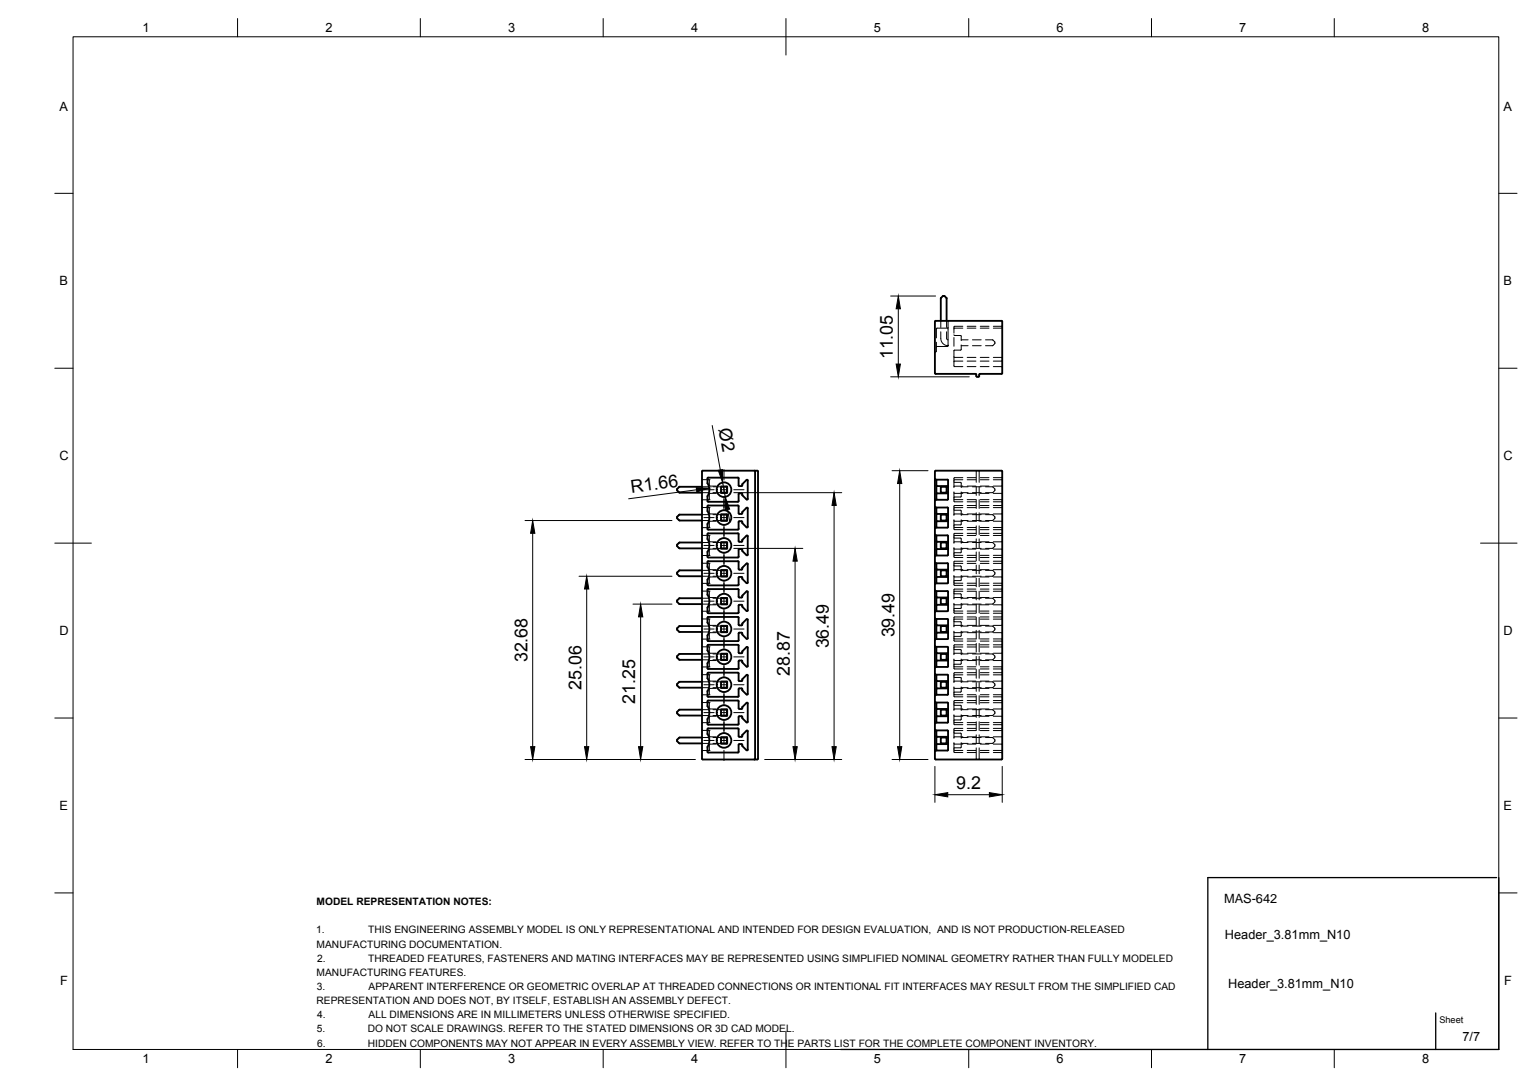
ISO-10303-21;
HEADER;
FILE_DESCRIPTION((''),'2;1');
FILE_NAME('Header_3.81mm_N10.step','2026-10-09T09:51:33-07:00',(''),(''),'','','');
FILE_SCHEMA (('AUTOMOTIVE_DESIGN { 1 0 10303 214 3 1 1 }'));
ENDSEC;
DATA;
#10=MECHANICAL_DESIGN_GEOMETRIC_PRESENTATION_REPRESENTATION('',(#1939,#1940,#1941,#1942,#1943,#1944,#1945,#1946,#1947,#1948,#1949,#1950,#1951,#1952,#1953,#1954,#1955,#1956,#1957,#1958,#1959,#1960,#1961,#1962,#1963,#1964,#1965,#1966,#1967,#1968,#1969,#1970,#1971,#1972,#1973,#1974,#1975,#1976,#1977,#1978,#1979,#1980,#1981,#1982,#1983,#1984,#1985,#1986,#1987,#1988,#1989,#1990,#1991,#1992,#1993,#1994,#1995,#1996,#1997,#1998,#1999,#2000,#2001,#2002,#2003,#2004,#2005,#2006,#2007,#2008,#2009,#2010,#2011,#2012,#2013,#2014,#2015,#2016,#2017,#2018,#2019,#2020,#2021,#2022,#2023,#2024,#2025,#2026,#2027,#2028,#2029,#2030,#2031,#2032,#2033,#2034,#2035,#2036,#2037,#2038,#2039,#2040,#2041,#2042,#2043,#2044,#2045,#2046,#2047,#2048,#2049,#2050,#2051,#2052,#2053,#2054,#2055,#2056,#2057,#2058,#2059,#2060,#2061,#2062,#2063,#2064,#2065,#2066,#2067,#2068,#2069,#2070,#2071,#2072,#2073,#2074,#2075,#2076,#2077,#2078,#2079,#2080,#2081,#2082,#2083,#2084,#2085,#2086,#2087,#2088,#2089,#2090,#2091,#2092,#2093,#2094,#2095,#2096,#2097,#2098,#2099,#2100,#2101,#2102,#2103,#2104,#2105,#2106,#2107,#2108,#2109,#2110,#2111,#2112,#2113,#2114,#2115,#2116,#2117,#2118,#2119,#2120,#2121,#2122,#2123,#2124,#2125,#2126,#2127,#2128,#2129,#2130,#2131,#2132,#2133,#2134,#2135,#2136,#2137,#2138,#2139,#2140,#2141,#2142,#2143,#2144,#2145,#2146,#2147,#2148,#2149,#2150,#2151,#2152,#2153,#2154,#2155,#2156,#2157,#2158,#2159,#2160,#2161,#2162,#2163,#2164,#2165,#2166,#2167,#2168,#2169,#2170,#2171,#2172,#2173,#2174,#2175,#2176,#2177,#2178,#2179,#2180,#2181,#2182,#2183,#2184,#2185,#2186,#2187,#2188,#2189,#2190,#2191,#2192,#2193,#2194,#2195,#2196,#2197,#2198,#2199,#2200,#2201,#2202,#2203,#2204,#2205,#2206,#2207,#2208,#2209,#2210,#2211,#2212,#2213,#2214,#2215,#2216,#2217,#2218,#2219,#2220,#2221,#2222,#2223,#2224,#2225,#2226,#2227,#2228,#2229,#2230,#2231,#2232,#2233,#2234,#2235,#2236,#2237,#2238,#2239,#2240,#2241,#2242,#2243,#2244,#2245,#2246,#2247,#2248,#2249,#2250,#2251,#2252,#2253,#2254,#2255,#2256,#2257,#2258,#2259,#2260,#2261,#2262,#2263,#2264,#2265,#2266,#2267,#2268,#2269,#2270,#2271,#2272,#2273,#2274,#2275,#2276,#2277,#2278,#2279,#2280,#2281,#2282,#2283,#2284,#2285,#2286,#2287,#2288,#2289,#2290,#2291,#2292,#2293,#2294,#2295,#2296,#2297,#2298,#2299,#2300,#2301,#2302,#2303,#2304,#2305,#2306,#2307,#2308,#2309,#2310,#2311,#2312,#2313,#2314,#2315,#2316,#2317,#2318,#2319,#2320,#2321,#2322,#2323,#2324,#2325,#2326,#2327,#2328,#2329,#2330,#2331,#2332,#2333,#2334,#2335,#2336,#2337,#2338,#2339,#2340,#2341,#2342,#2343,#2344,#2345,#2346,#2347,#2348,#2349,#2350,#2351,#2352,#2353,#2354,#2355,#2356,#2357,#2358,#2359,#2360,#2361,#2362,#2363,#2364,#2365,#2366,#2367,#2368,#2369,#2370,#2371,#2372,#2373,#2374,#2375,#2376,#2377,#2378,#2379,#2380,#2381,#2382,#2383,#2384,#2385,#2386,#2387,#2388,#2389,#2390,#2391,#2392,#2393,#2394,#2395,#2396,#2397,#2398,#2399,#2400,#2401,#2402,#2403,#2404,#2405,#2406,#2407,#2408,#2409,#2410,#2411,#2412,#2413,#2414,#2415,#2416,#2417,#2418,#2419,#2420,#2421,#2422,#2423,#2424,#2425,#2426,#2427,#2428,#2429,#2430,#2431,#2432,#2433,#2434,#2435,#2436,#2437,#2438,#2439,#2440,#2441,#2442,#2443,#2444,#2445,#2446,#2447,#2448,#2449,#2450,#2451,#2452,#2453,#2454,#2455,#2456,#2457,#2458,#2459,#2460,#2461,#2462,#2463,#2464,#2465,#2466,#2467,#2468,#2469,#2470,#2471,#2472,#2473,#2474,#2475,#2476,#2477,#2478,#2479,#2480,#2481,#2482,#2483,#2484,#2485,#2486,#2487,#2488,#2489,#2490,#2491,#2492,#2493,#2494,#2495,#2496,#2497,#2498,#2499,#2500,#2501,#2502,#2503,#2504,#2505,#2506,#2507,#2508,#2509,#2510,#2511,#2512,#2513,#2514,#2515,#2516,#2517,#2518,#2519,#2520,#2521,#2522,#2523,#2524,#2525,#2526,#2527,#2528,#2529,#2530,#2531,#2532,#2533,#2534,#2535,#2536,#2537,#2538,#2539,#2540,#2541,#2542,#2543,#2544,#2545,#2546,#2547,#2548,#2549,#2550,#2551,#2552,#2553,#2554,#2555,#2556,#2557,#2558,#2559,#2560,#2561,#2562,#2563,#2564,#2565,#2566,#2567,#2568,#2569,#2570,#2571,#2572,#2573,#2574,#2575,#2576,#2577,#2578,#2579,#2580,#2581,#2582,#2583,#2584,#2585,#2586,#2587,#2588,#2589,#2590,#2591,#2592,#2593,#2594,#2595,#2596,#2597,#2598,#2599,#2600,#2601,#2602,#2603,#2604,#2605,#2606,#2607,#2608,#2609,#2610,#2611,#2612,#2613,#2614,#2615,#2616,#2617,#2618,#2619,#2620,#2621,#2622,#2623,#2624,#2625,#2626,#2627,#2628,#2629,#2630,#2631,#2632,#2633,#2634,#2635,#2636,#2637,#2638,#2639,#2640,#2641,#2642,#2643,#2644,#2645,#2646,#2647,#2648,#2649,#2650,#2651,#2652,#2653,#2654,#2655,#2656,#2657,#2658,#2659,#2660,#2661,#2662,#2663,#2664,#2665,#2666,#2667,#2668,#2669,#2670,#2671,#2672,#2673,#2674,#2675,#2676,#2677,#2678,#2679,#2680,#2681,#2682,#2683,#2684,#2685,#2686,#2687,#2688,#2689,#2690,#2691,#2692,#2693,#2694,#2695,#2696,#2697,#2698,#2699,#2700,#2701,#2702,#2703,#2704,#2705,#2706,#2707,#2708,#2709,#2710,#2711,#2712,#2713,#2714,#2715,#2716,#2717,#2718,#2719,#2720,#2721,#2722,#2723,#2724,#2725,#2726,#2727,#2728,#2729,#2730,#2731,#2732,#2733,#2734,#2735,#2736,#2737,#2738,#2739,#2740,#2741,#2742,#2743,#2744,#2745,#2746,#2747,#2748,#2749,#2750,#2751,#2752,#2753,#2754,#2755,#2756,#2757,#2758,#2759,#2760,#2761,#2762,#2763,#2764,#2765,#2766,#2767,#2768,#2769,#2770,#2771,#2772,#2773,#2774,#2775,#2776,#2777,#2778,#2779,#2780,#2781,#2782,#2783,#2784,#2785,#2786,#2787,#2788,#2789,#2790,#2791,#2792,#2793,#2794,#2795,#2796,#2797,#2798,#2799,#2800,#2801,#2802,#2803,#2804,#2805,#2806,#2807,#2808,#2809,#2810,#2811,#2812,#2813,#2814,#2815,#2816,#2817,#2818,#2819,#2820,#2821,#2822,#2823,#2824,#2825,#2826,#2827,#2828,#2829,#2830,#2831,#2832,#2833,#2834,#2835,#2836,#2837,#2838,#2839,#2840,#2841,#2842,#2843,#2844,#2845,#2846,#2847,#2848,#2849,#2850,#2851,#2852,#2853,#2854,#2855,#2856,#2857,#2858,#2859,#2860,#2861,#2862,#2863,#2864,#2865,#2866,#2867,#2868,#2869,#2870,#2871,#2872,#2873,#2874,#2875,#2876,#2877,#2878,#2879,#2880,#2881,#2882,#2883,#2884,#2885,#2886,#2887,#2888,#2889,#2890,#2891,#2892,#2893,#2894,#2895,#2896,#2897,#2898,#2899,#2900,#2901,#2902,#2903,#2904,#2905,#2906,#2907,#2908,#2909,#2910,#2911,#2912,#2913,#2914,#2915,#2916,#2917,#2918,#2919,#2920,#2921,#2922,#2923,#2924,#2925,#2926,#2927,#2928,#2929,#2930,#2931,#2932,#2933,#2934,#2935,#2936,#2937,#2938,#2939,#2940,#2941,#2942,#2943,#2944,#2945,#2946,#2947,#2948,#2949,#2950,#2951,#2952,#2953,#2954,#2955,#2956,#2957,#2958,#2959,#2960,#2961,#2962,#2963,#2964,#2965,#2966,#2967,#2968,#2969,#2970,#2971,#2972,#2973,#2974,#2975,#2976,#2977,#2978,#2979,#2980,#2981,#2982,#2983,#2984,#2985,#2986,#2987,#2988,#2989,#2990,#2991,#2992,#2993,#2994,#2995,#2996,#2997,#2998,#2999,#3000,#3001,#3002,#3003,#3004,#3005,#3006,#3007,#3008,#3009,#3010,#3011,#3012,#3013,#3014,#3015,#3016,#3017,#3018,#3019,#3020,#3021,#3022,#3023,#3024,#3025,#3026,#3027,#3028,#3029,#3030,#3031,#3032,#3033,#3034,#3035,#3036,#3037,#3038,#3039,#3040,#3041,#3042,#3043,#3044,#3045,#3046,#3047,#3048,#3049,#3050,#3051,#3052,#3053,#3054,#3055,#3056,#3057,#3058,#3059,#3060,#3061,#3062,#3063,#3064,#3065,#3066,#3067,#3068,#3069,#3070,#3071,#3072,#3073,#3074,#3075,#3076,#3077,#3078,#3079,#3080,#3081,#3082,#3083,#3084,#3085,#3086,#3087,#3088,#3089,#3090,#3091,#3092,#3093,#3094,#3095,#3096,#3097,#3098,#3099,#3100,#3101,#3102,#3103,#3104,#3105,#3106,#3107,#3108,#3109,#3110,#3111,#3112,#3113,#3114,#3115,#3116,#3117,#3118,#3119,#3120,#3121,#3122,#3123,#3124,#3125,#3126,#3127,#3128,#3129,#3130,#3131,#3132,#3133,#3134,#3135,#3136,#3137,#3138,#3139,#3140,#3141,#3142,#3143,#3144,#3145,#3146,#3147,#3148,#3149,#3150,#3151,#3152,#3153,#3154,#3155,#3156,#3157,#3158,#3159,#3160,#3161,#3162,#3163,#3164,#3165,#3166,#3167,#3168,#3169,#3170,#3171,#3172,#3173,#3174,#3175,#3176,#3177,#3178,#3179,#3180,#3181,#3182,#3183,#3184,#3185,#3186,#3187,#3188,#3189,#3190,#3191,#3192,#3193,#3194,#3195,#3196,#3197,#3198,#3199,#3200,#3201,#3202,#3203,#3204,#3205,#3206,#3207,#3208,#3209,#3210,#3211,#3212,#3213,#3214,#3215,#3216,#3217,#3218,#3219,#3220,#3221,#3222,#3223,#3224,#3225,#3226,#3227,#3228,#3229,#3230,#3231,#3232,#3233,#3234,#3235,#3236,#3237,#3238,#3239,#3240,#3241,#3242,#3243,#3244,#3245,#3246,#3247,#3248,#3249,#3250,#3251,#3252,#3253,#3254,#3255,#3256,#3257,#3258,#3259,#3260,#3261,#3262,#3263,#3264,#3265,#3266,#3267,#3268,#3269,#3270,#3271,#3272,#3273,#3274,#3275,#3276,#3277,#3278,#3279,#3280,#3281,#3282,#3283,#3284,#3285,#3286,#3287,#3288,#3289,#3290,#3291,#3292,#3293,#3294,#3295,#3296,#3297,#3298,#3299,#3300,#3301,#3302,#3303,#3304,#3305,#3306,#3307,#3308,#3309,#3310,#3311,#3312,#3313,#3314,#3315,#3316,#3317,#3318,#3319,#3320,#3321,#3322,#3323,#3324,#3325,#3326,#3327,#3328,#3329,#3330,#3331,#3332,#3333,#3334,#3335,#3336,#3337,#3338,#3339,#3340,#3341,#3342,#3343,#3344,#3345,#3346,#3347,#3348,#3349,#3350,#3351,#3352,#3353,#3354,#3355,#3356,#3357,#3358,#3359,#3360,#3361,#3362,#3363,#3364,#3365,#3366,#3367,#3368,#3369,#3370,#3371,#3372,#3373,#3374,#3375,#3376,#3377,#3378,#3379,#3380,#3381,#3382,#3383,#3384,#3385,#3386,#3387,#3388,#3389,#3390,#3391,#3392,#3393,#3394,#3395,#3396,#3397,#3398,#3399,#3400,#3401,#3402,#3403,#3404,#3405,#3406,#3407,#3408,#3409,#3410,#3411,#3412,#3413,#3414,#3415,#3416,#3417,#3418,#3419,#3420,#3421,#3422,#3423,#3424,#3425,#3426,#3427,#3428,#3429,#3430,#3431,#3432,#3433,#3434,#3435,#3436,#3437,#3438,#3439,#3440,#3441,#3442,#3443,#3444,#3445,#3446,#3447,#3448,#3449,#3450,#3451,#3452,#3453,#3454,#3455,#3456,#3457,#3458,#3459,#3460,#3461,#3462,#3463,#3464,#3465,#3466,#3467,#3468,#3469,#3470,#3471,#3472,#3473,#3474,#3475,#3476,#3477,#3478,#3479,#3480,#3481,#3482,#3483,#3484,#3485,#3486,#3487,#3488,#3489,#3490,#3491,#3492,#3493,#3494,#3495,#3496,#3497,#3498,#3499,#3500,#3501,#3502,#3503,#3504,#3505,#3506,#3507,#3508,#3509,#3510,#3511,#3512,#3513,#3514,#3515,#3516,#3517,#3518,#3519,#3520,#3521,#3522,#3523,#3524,#3525,#3526,#3527,#3528,#3529,#3530,#3531,#3532,#3533,#3534,#3535,#3536,#3537,#3538,#3539,#3540,#3541,#3542,#3543,#3544,#3545,#3546,#3547,#3548,#3549,#3550,#3551,#3552,#3553,#3554,#3555,#3556,#3557,#3558,#3559,#3560,#3561,#3562,#3563,#3564,#3565,#3566,#3567,#3568,#3569,#3570,#3571,#3572,#3573,#3574,#3575,#3576,#3577,#3578,#3579,#3580,#3581,#3582,#3583,#3584,#3585,#3586,#3587,#3588,#3589,#3590,#3591,#3592,#3593,#3594,#3595,#3596,#3597,#3598,#3599,#3600,#3601,#3602,#3603,#3604,#3605,#3606,#3607,#3608,#3609,#3610,#3611,#3612,#3613,#3614,#3615,#3616,#3617,#3618,#3619,#3620,#3621,#3622,#3623,#3624,#3625,#3626,#3627,#3628,#3629,#3630,#3631,#3632,#3633,#3634,#3635,#3636,#3637,#3638,#3639,#3640,#3641,#3642,#3643,#3644,#3645,#3646,#3647,#3648,#3649,#3650,#3651,#3652,#3653,#3654,#3655,#3656,#3657,#3658,#3659,#3660,#3661,#3662,#3663,#3664,#3665,#3666,#3667,#3668,#3669,#3670,#3671,#3672,#3673,#3674,#3675,#3676,#3677,#3678,#3679,#3680,#3681,#3682,#3683,#3684,#3685,#3686,#3687,#3688,#3689,#3690,#3691,#3692,#3693,#3694,#3695,#3696,#3697,#3698,#3699,#3700,#3701,#3702,#3703,#3704,#3705,#3706,#3707,#3708,#3709,#3710,#3711,#3712,#3713,#3714,#3715,#3716,#3717,#3718,#3719,#3720,#3721,#3722,#3723,#3724,#3725,#3726,#3727,#3728,#3729,#3730,#3731,#3732,#3733,#3734,#3735,#3736,#3737,#3738,#3739,#3740,#3741,#3742,#3743,#3744,#3745,#3746,#3747,#3748,#3749,#3750,#3751,#3752,#3753,#3754,#3755,#3756,#3757,#3758,#3759,#3760,#3761,#3762,#3763,#3764,#3765,#3766,#3767,#3768,#3769,#3770,#3771,#3772,#3773,#3774,#3775,#3776,#3777,#3778,#3779,#3780,#3781,#3782,#3783,#3784,#3785,#3786,#3787,#3788,#3789,#3790,#3791,#3792,#3793,#3794,#3795,#3796,#3797,#3798,#3799,#3800,#3801,#3802,#3803,#3804,#3805,#3806,#3807,#3808,#3809,#3810,#3811,#3812,#3813,#3814,#3815,#3816,#3817,#3818,#3819,#3820,#3821,#3822,#3823,#3824,#3825,#3826,#3827,#3828,#3829,#3830,#3831,#3832,#3833,#3834,#3835,#3836,#3837,#3838,#3839,#3840,#3841,#3842,#3843,#3844,#3845,#3846,#3847,#3848,#3849,#3850,#3851,#3852,#3853,#3854,#3855,#3856,#3857,#3858,#3859,#3860,#3861,#3862,#3863,#3864,#3865,#3866,#3867,#3868,#3869,#3870,#3871,#3872,#3873,#3874,#3875,#3876,#3877,#3878,#3879,#3880,#3881,#3882,#3883,#3884,#3885,#3886,#3887,#3888,#3889,#3890,#3891,#3892,#3893,#3894,#3895,#3896,#3897,#3898,#3899,#3900,#3901,#3902,#3903,#3904,#3905,#3906,#3907,#3908,#3909,#3910,#3911,#3912,#3913,#3914,#3915,#3916,#3917,#3918,#3919,#3920,#3921,#3922,#3923,#3924,#3925,#3926,#3927,#3928,#3929,#3930,#3931,#3932,#3933,#3934,#3935,#3936,#3937,#3938,#3939,#3940,#3941,#3942,#3943,#3944,#3945,#3946,#3947,#3948,#3949,#3950,#3951,#3952,#3953,#3954,#3955,#3956,#3957,#3958,#3959,#3960,#3961,#3962,#3963,#3964,#3965,#3966,#3967,#3968,#3969,#3970,#3971,#3972,#3973,#3974,#3975,#3976,#3977,#3978,#3979,#3980,#3981,#3982,#3983,#3984,#3985,#3986,#3987,#3988,#3989,#3990,#3991,#3992,#3993,#3994,#3995,#3996,#3997,#3998,#3999,#4000,#4001,#4002,#4003,#4004,#4005,#4006,#4007,#4008,#4009,#4010,#4011,#4012,#4013,#4014,#4015,#4016,#4017,#4018,#4019,#4020,#4021,#4022,#4023,#4024,#4025,#4026,#4027,#4028,#4029,#4030,#4031,#4032,#4033,#4034,#4035,#4036,#4037,#4038,#4039,#4040,#4041,#4042,#4043,#4044,#4045,#4046,#4047,#4048,#4049,#4050,#4051,#4052,#4053,#4054,#4055,#4056,#4057,#4058,#4059,#4060,#4061,#4062,#4063,#4064,#4065,#4066,#4067,#4068,#4069,#4070,#4071,#4072,#4073,#4074,#4075,#4076,#4077,#4078,#4079,#4080,#4081,#4082,#4083,#4084,#4085,#4086,#4087,#4088,#4089,#4090,#4091,#4092,#4093,#4094,#4095,#4096,#4097,#4098,#4099,#4100,#4101,#4102,#4103,#4104,#4105,#4106,#4107,#4108,#4109,#4110,#4111,#4112,#4113,#4114,#4115,#4116,#4117,#4118,#4119,#4120,#4121,#4122,#4123,#4124,#4125,#4126,#4127,#4128,#4129,#4130,#4131,#4132,#4133,#4134,#4135,#4136,#4137,#4138,#4139,#4140,#4141,#4142,#4143,#4144,#4145,#4146,#4147,#4148,#4149,#4150,#4151,#4152,#4153,#4154,#4155,#4156,#4157,#4158,#4159,#4160,#4161,#4162,#4163,#4164,#4165,#4166,#4167,#4168,#4169),#126571);
#290=B_SPLINE_CURVE_WITH_KNOTS('',3,(#113894,#113895,#113896,#113897,#113898,
#113899,#113900,#113901),.UNSPECIFIED.,.F.,.F.,(4,2,2,4),(-0.0212593174733862,
-0.0176486602253693,-0.0143243289552082,-0.0134403252720105),
 .UNSPECIFIED.) ;
#291=B_SPLINE_CURVE_WITH_KNOTS('',3,(#113937,#113938,#113939,#113940,#113941,
#113942,#113943,#113944),.UNSPECIFIED.,.F.,.F.,(4,2,2,4),(-0.021259317482921,
-0.0176486602328459,-0.0143243289609224,-0.0134403252772803),
 .UNSPECIFIED.) ;
#292=B_SPLINE_CURVE_WITH_KNOTS('',3,(#113980,#113981,#113982,#113983,#113984,
#113985,#113986,#113987),.UNSPECIFIED.,.F.,.F.,(4,2,2,4),(-0.0212593174877944,
-0.0176486602368674,-0.0143243289641644,-0.0134403252803157),
 .UNSPECIFIED.) ;
#293=B_SPLINE_CURVE_WITH_KNOTS('',3,(#114023,#114024,#114025,#114026,#114027,
#114028,#114029,#114030),.UNSPECIFIED.,.F.,.F.,(4,2,2,4),(-0.0212593174829433,
-0.0176486602328601,-0.014324328960934,-0.0134403252772914),
 .UNSPECIFIED.) ;
#294=B_SPLINE_CURVE_WITH_KNOTS('',3,(#114066,#114067,#114068,#114069,#114070,
#114071,#114072,#114073),.UNSPECIFIED.,.F.,.F.,(4,2,2,4),(-0.0212593174732112,
-0.0176486602254681,-0.0143243289554829,-0.0134403252723181),
 .UNSPECIFIED.) ;
#295=B_SPLINE_CURVE_WITH_KNOTS('',3,(#114109,#114110,#114111,#114112,#114113,
#114114,#114115,#114116),.UNSPECIFIED.,.F.,.F.,(4,2,2,4),(-0.0212593174781932,
-0.0176486602293651,-0.0143243289584549,-0.0134403252750573),
 .UNSPECIFIED.) ;
#296=B_SPLINE_CURVE_WITH_KNOTS('',3,(#114152,#114153,#114154,#114155,#114156,
#114157,#114158,#114159),.UNSPECIFIED.,.F.,.F.,(4,2,2,4),(-0.0212593174830444,
-0.0176486602331658,-0.0143243289613579,-0.0134403252777338),
 .UNSPECIFIED.) ;
#297=B_SPLINE_CURVE_WITH_KNOTS('',3,(#114195,#114196,#114197,#114198,#114199,
#114200,#114201,#114202),.UNSPECIFIED.,.F.,.F.,(4,2,2,4),(-0.021259317485983,
-0.017648660235379,-0.0143243289629727,-0.0134403252792024),
 .UNSPECIFIED.) ;
#298=B_SPLINE_CURVE_WITH_KNOTS('',3,(#114319,#114320,#114321,#114322,#114323,
#114324,#114325,#114326),.UNSPECIFIED.,.F.,.F.,(4,2,2,4),(-0.0212593174838741,
-0.0176486602337396,-0.0143243289617316,-0.0134403252780616),
 .UNSPECIFIED.) ;
#299=B_SPLINE_CURVE_WITH_KNOTS('',3,(#114443,#114444,#114445,#114446,#114447,
#114448,#114449,#114450),.UNSPECIFIED.,.F.,.F.,(4,2,2,4),(-0.021259317485706,
-0.0176486602351398,-0.0143243289627718,-0.013440325279013),
 .UNSPECIFIED.) ;
#300=B_SPLINE_CURVE_WITH_KNOTS('',3,(#116047,#116048,#116049,#116050,#116051,
#116052,#116053,#116054),.UNSPECIFIED.,.F.,.F.,(4,2,2,4),(-0.052701717162025,
-0.0518504523811948,-0.0480303917439054,-0.04467544736819),
 .UNSPECIFIED.) ;
#301=B_SPLINE_CURVE_WITH_KNOTS('',3,(#116058,#116059,#116060,#116061,#116062,
#116063,#116064,#116065,#116066,#116067,#116068,#116069,#116070,#116071,
#116072,#116073,#116074,#116075,#116076,#116077,#116078,#116079,#116080,
#116081,#116082,#116083,#116084,#116085,#116086,#116087,#116088),
 .UNSPECIFIED.,.F.,.F.,(4,3,3,3,3,3,3,3,3,3,4),(0.,1.7911486298437E-5,3.35636550441565E-5,
5.14128838689559E-5,6.71346369544057E-5,8.50076921954425E-5,0.000100614915215922,
0.000118595988596762,0.000134133865285036,0.000151845157316713,0.0001565184788544),
 .UNSPECIFIED.) ;
#302=B_SPLINE_CURVE_WITH_KNOTS('',3,(#116090,#116091,#116092,#116093,#116094,
#116095,#116096,#116097,#116098,#116099,#116100,#116101,#116102,#116103,
#116104,#116105,#116106,#116107,#116108,#116109,#116110,#116111),
 .UNSPECIFIED.,.F.,.F.,(4,2,2,2,2,2,2,2,2,2,4),(-0.0842935807175857,-0.0841564124762399,
-0.0836958438579189,-0.0829341784875174,-0.0805923611130053,-0.0773601159115686,
-0.0742136752654363,-0.071123820447877,-0.0675672289498007,-0.0637829215046486,
-0.0629274139192696),.UNSPECIFIED.) ;
#303=B_SPLINE_CURVE_WITH_KNOTS('',3,(#119109,#119110,#119111,#119112,#119113,
#119114,#119115,#119116),.UNSPECIFIED.,.F.,.F.,(4,2,2,4),(-0.0527017171620382,
-0.0518504523812081,-0.0480303917439178,-0.0446754473682008),
 .UNSPECIFIED.) ;
#304=B_SPLINE_CURVE_WITH_KNOTS('',3,(#119120,#119121,#119122,#119123,#119124,
#119125,#119126,#119127,#119128,#119129,#119130,#119131,#119132,#119133,
#119134,#119135,#119136,#119137,#119138,#119139,#119140,#119141,#119142,
#119143,#119144,#119145,#119146,#119147,#119148,#119149,#119150),
 .UNSPECIFIED.,.F.,.F.,(4,3,3,3,3,3,3,3,3,3,4),(0.,1.79114862984415E-5,
3.35636550441565E-5,5.14128838689557E-5,6.7134636954406E-5,8.50076921954395E-5,
0.000100614915215921,0.000118595988596772,0.000134133865285036,0.000151845157316653,
0.0001565184788544),.UNSPECIFIED.) ;
#305=B_SPLINE_CURVE_WITH_KNOTS('',3,(#119152,#119153,#119154,#119155,#119156,
#119157,#119158,#119159,#119160,#119161,#119162,#119163,#119164,#119165,
#119166,#119167,#119168,#119169,#119170,#119171,#119172,#119173),
 .UNSPECIFIED.,.F.,.F.,(4,2,2,2,2,2,2,2,2,2,4),(-0.0842935807153196,-0.0841564124739783,
-0.0836958438556783,-0.0829341784853091,-0.0805923611108952,-0.0773601159095917,
-0.0742136752635866,-0.0711238204461505,-0.0675672289482145,-0.0637829215032092,
-0.062927413917864),.UNSPECIFIED.) ;
#306=B_SPLINE_CURVE_WITH_KNOTS('',3,(#119813,#119814,#119815,#119816,#119817,
#119818,#119819,#119820),.UNSPECIFIED.,.F.,.F.,(4,2,2,4),(-0.0527017171621304,
-0.0518504523813015,-0.0480303917440028,-0.0446754473682719),
 .UNSPECIFIED.) ;
#307=B_SPLINE_CURVE_WITH_KNOTS('',3,(#119824,#119825,#119826,#119827,#119828,
#119829,#119830,#119831,#119832,#119833,#119834,#119835,#119836,#119837,
#119838,#119839,#119840,#119841,#119842,#119843,#119844,#119845,#119846,
#119847,#119848,#119849,#119850,#119851,#119852,#119853,#119854),
 .UNSPECIFIED.,.F.,.F.,(4,3,3,3,3,3,3,3,3,3,4),(0.,1.79114862984384E-5,
3.35636550441566E-5,5.14128838689606E-5,6.7134636954406E-5,8.50076921954722E-5,
0.000100614915215922,0.000118595988596755,0.000134133865285036,0.00015184515731678,
0.0001565184788544),.UNSPECIFIED.) ;
#308=B_SPLINE_CURVE_WITH_KNOTS('',3,(#119856,#119857,#119858,#119859,#119860,
#119861,#119862,#119863,#119864,#119865,#119866,#119867,#119868,#119869,
#119870,#119871,#119872,#119873,#119874,#119875,#119876,#119877),
 .UNSPECIFIED.,.F.,.F.,(4,2,2,2,2,2,2,2,2,2,4),(-0.0842935807419127,-0.0841564125005222,
-0.0836958438819682,-0.082934178511186,-0.0805923611355419,-0.0773601159325885,
-0.0742136752850249,-0.0711238204661043,-0.0675672289665108,-0.0637829215197928,
-0.0629274139340661),.UNSPECIFIED.) ;
#309=B_SPLINE_CURVE_WITH_KNOTS('',3,(#120040,#120041,#120042,#120043,#120044,
#120045,#120046,#120047),.UNSPECIFIED.,.F.,.F.,(4,2,2,4),(-0.0527017171621393,
-0.0518504523813096,-0.0480303917440155,-0.0446754473682944),
 .UNSPECIFIED.) ;
#310=B_SPLINE_CURVE_WITH_KNOTS('',3,(#120051,#120052,#120053,#120054,#120055,
#120056,#120057,#120058,#120059,#120060,#120061,#120062,#120063,#120064,
#120065,#120066,#120067,#120068,#120069,#120070,#120071,#120072,#120073,
#120074,#120075,#120076,#120077,#120078,#120079,#120080,#120081),
 .UNSPECIFIED.,.F.,.F.,(4,3,3,3,3,3,3,3,3,3,4),(0.,1.7911486298444E-5,3.35636550441567E-5,
5.14128838689174E-5,6.71346369544062E-5,8.50076921954515E-5,0.000100614915215921,
0.000118595988596814,0.000134133865285036,0.000151845157316771,0.0001565184788544),
 .UNSPECIFIED.) ;
#311=B_SPLINE_CURVE_WITH_KNOTS('',3,(#120083,#120084,#120085,#120086,#120087,
#120088,#120089,#120090,#120091,#120092,#120093,#120094,#120095,#120096,
#120097,#120098,#120099,#120100,#120101,#120102,#120103,#120104),
 .UNSPECIFIED.,.F.,.F.,(4,2,2,2,2,2,2,2,2,2,4),(-0.0842935808351552,-0.0841564125935704,
-0.0836958439740798,-0.0829341786018125,-0.0805923612217205,-0.077360116012801,
-0.0742136753596006,-0.0711238205353107,-0.0675672290297288,-0.0637829215768355,
-0.0629274139897445),.UNSPECIFIED.) ;
#312=B_SPLINE_CURVE_WITH_KNOTS('',3,(#120267,#120268,#120269,#120270,#120271,
#120272,#120273,#120274),.UNSPECIFIED.,.F.,.F.,(4,2,2,4),(-0.0527017171620452,
-0.0518504523812172,-0.0480303917439374,-0.04467544736823),
 .UNSPECIFIED.) ;
#313=B_SPLINE_CURVE_WITH_KNOTS('',3,(#120278,#120279,#120280,#120281,#120282,
#120283,#120284,#120285,#120286,#120287,#120288,#120289,#120290,#120291,
#120292,#120293,#120294,#120295,#120296,#120297,#120298,#120299,#120300,
#120301,#120302,#120303,#120304,#120305,#120306,#120307,#120308),
 .UNSPECIFIED.,.F.,.F.,(4,3,3,3,3,3,3,3,3,3,4),(0.,1.79114862984569E-5,
3.35636550441567E-5,5.14128838689565E-5,6.71346369544062E-5,8.50076921954284E-5,
0.000100614915215921,0.000118595988596684,0.000134133865285036,0.000151845157316633,
0.0001565184788544),.UNSPECIFIED.) ;
#314=B_SPLINE_CURVE_WITH_KNOTS('',3,(#120310,#120311,#120312,#120313,#120314,
#120315,#120316,#120317,#120318,#120319,#120320,#120321,#120322,#120323,
#120324,#120325,#120326,#120327,#120328,#120329,#120330,#120331),
 .UNSPECIFIED.,.F.,.F.,(4,2,2,2,2,2,2,2,2,2,4),(-0.0842935807861705,-0.0841564125446822,
-0.08369584392567,-0.0829341785541707,-0.0805923611763772,-0.0773601159705437,
-0.0742136753202586,-0.0711238204987475,-0.0675672289962676,-0.0637829215465878,
-0.0629274139602073),.UNSPECIFIED.) ;
#315=B_SPLINE_CURVE_WITH_KNOTS('',3,(#120494,#120495,#120496,#120497,#120498,
#120499,#120500,#120501),.UNSPECIFIED.,.F.,.F.,(4,2,2,4),(-0.0527017171621833,
-0.0518504523813524,-0.0480303917440445,-0.044675447368305),
 .UNSPECIFIED.) ;
#316=B_SPLINE_CURVE_WITH_KNOTS('',3,(#120505,#120506,#120507,#120508,#120509,
#120510,#120511,#120512,#120513,#120514,#120515,#120516,#120517,#120518,
#120519,#120520,#120521,#120522,#120523,#120524,#120525,#120526,#120527,
#120528,#120529,#120530,#120531,#120532,#120533,#120534,#120535),
 .UNSPECIFIED.,.F.,.F.,(4,3,3,3,3,3,3,3,3,3,4),(0.,1.791148629847E-5,3.35636550441561E-5,
5.14128838689644E-5,6.71346369544058E-5,8.50076921954764E-5,0.000100614915215921,
0.000118595988596817,0.000134133865285032,0.000151845157316703,0.000156518478854398),
 .UNSPECIFIED.) ;
#317=B_SPLINE_CURVE_WITH_KNOTS('',3,(#120537,#120538,#120539,#120540,#120541,
#120542,#120543,#120544,#120545,#120546,#120547,#120548,#120549,#120550,
#120551,#120552,#120553,#120554,#120555,#120556,#120557,#120558),
 .UNSPECIFIED.,.F.,.F.,(4,2,2,2,2,2,2,2,2,2,4),(-0.0842935807861705,-0.0841564125446822,
-0.08369584392567,-0.0829341785541707,-0.0805923611763772,-0.0773601159705437,
-0.0742136753202586,-0.0711238204987475,-0.0675672289962676,-0.0637829215465878,
-0.0629274139602073),.UNSPECIFIED.) ;
#318=B_SPLINE_CURVE_WITH_KNOTS('',3,(#120721,#120722,#120723,#120724,#120725,
#120726,#120727,#120728),.UNSPECIFIED.,.F.,.F.,(4,2,2,4),(-0.0527017171619057,
-0.0518504523810739,-0.0480303917437878,-0.0446754473680843),
 .UNSPECIFIED.) ;
#319=B_SPLINE_CURVE_WITH_KNOTS('',3,(#120732,#120733,#120734,#120735,#120736,
#120737,#120738,#120739,#120740,#120741,#120742,#120743,#120744,#120745,
#120746,#120747,#120748,#120749,#120750,#120751,#120752,#120753,#120754,
#120755,#120756,#120757,#120758,#120759,#120760,#120761,#120762),
 .UNSPECIFIED.,.F.,.F.,(4,3,3,3,3,3,3,3,3,3,4),(0.,1.79114862984022E-5,
3.35636550441561E-5,5.14128838690747E-5,6.71346369544058E-5,8.50076921955029E-5,
0.000100614915215921,0.000118595988596949,0.000134133865285032,0.000151845157316721,
0.000156518478854398),.UNSPECIFIED.) ;
#320=B_SPLINE_CURVE_WITH_KNOTS('',3,(#120764,#120765,#120766,#120767,#120768,
#120769,#120770,#120771,#120772,#120773,#120774,#120775,#120776,#120777,
#120778,#120779,#120780,#120781,#120782,#120783,#120784,#120785),
 .UNSPECIFIED.,.F.,.F.,(4,2,2,2,2,2,2,2,2,2,4),(-0.0842935806846017,-0.0841564124433096,
-0.0836958438252493,-0.0829341784552694,-0.0805923610820353,-0.0773601158823278,
-0.0742136752378489,-0.07112382042188,-0.0675672289255957,-0.0637829214823062,
-0.0629274138973503),.UNSPECIFIED.) ;
#321=B_SPLINE_CURVE_WITH_KNOTS('',3,(#120948,#120949,#120950,#120951,#120952,
#120953,#120954,#120955),.UNSPECIFIED.,.F.,.F.,(4,2,2,4),(-0.0527017171620534,
-0.0518504523812236,-0.0480303917439217,-0.0446754473681886),
 .UNSPECIFIED.) ;
#322=B_SPLINE_CURVE_WITH_KNOTS('',3,(#120959,#120960,#120961,#120962,#120963,
#120964,#120965,#120966,#120967,#120968,#120969,#120970,#120971,#120972,
#120973,#120974,#120975,#120976,#120977,#120978,#120979,#120980,#120981,
#120982,#120983,#120984,#120985,#120986,#120987,#120988,#120989),
 .UNSPECIFIED.,.F.,.F.,(4,3,3,3,3,3,3,3,3,3,4),(0.,1.79114862984111E-5,
3.35636550441561E-5,5.1412883869035E-5,6.71346369544058E-5,8.50076921954072E-5,
0.000100614915215921,0.000118595988596959,0.000134133865285032,0.000151845157317271,
0.000156518478854398),.UNSPECIFIED.) ;
#323=B_SPLINE_CURVE_WITH_KNOTS('',3,(#120991,#120992,#120993,#120994,#120995,
#120996,#120997,#120998,#120999,#121000,#121001,#121002,#121003,#121004,
#121005,#121006,#121007,#121008,#121009,#121010,#121011,#121012),
 .UNSPECIFIED.,.F.,.F.,(4,2,2,2,2,2,2,2,2,2,4),(-0.0842935807784001,-0.0841564125369118,
-0.0836958439179285,-0.0829341785465007,-0.080592361168928,-0.0773601159633862,
-0.0742136753133782,-0.071123820492143,-0.0675672289899856,-0.063782921540619,
-0.0629274139542864),.UNSPECIFIED.) ;
#324=B_SPLINE_CURVE_WITH_KNOTS('',3,(#121175,#121176,#121177,#121178,#121179,
#121180,#121181,#121182),.UNSPECIFIED.,.F.,.F.,(4,2,2,4),(-0.0527017171619366,
-0.0518504523811075,-0.0480303917438238,-0.0446754473681228),
 .UNSPECIFIED.) ;
#325=B_SPLINE_CURVE_WITH_KNOTS('',3,(#121186,#121187,#121188,#121189,#121190,
#121191,#121192,#121193,#121194,#121195,#121196,#121197,#121198,#121199,
#121200,#121201,#121202,#121203,#121204,#121205,#121206,#121207,#121208,
#121209,#121210,#121211,#121212,#121213,#121214,#121215,#121216),
 .UNSPECIFIED.,.F.,.F.,(4,3,3,3,3,3,3,3,3,3,4),(0.,1.7911486298388E-5,3.35636550441561E-5,
5.14128838690249E-5,6.71346369544058E-5,8.50076921954834E-5,0.000100614915215921,
0.000118595988596784,0.000134133865285032,0.000151845157317113,0.000156518478854398),
 .UNSPECIFIED.) ;
#326=B_SPLINE_CURVE_WITH_KNOTS('',3,(#121218,#121219,#121220,#121221,#121222,
#121223,#121224,#121225,#121226,#121227,#121228,#121229,#121230,#121231,
#121232,#121233,#121234,#121235,#121236,#121237,#121238,#121239),
 .UNSPECIFIED.,.F.,.F.,(4,2,2,2,2,2,2,2,2,2,4),(-0.0842935807784001,-0.0841564125369118,
-0.0836958439179285,-0.0829341785465007,-0.080592361168928,-0.0773601159633862,
-0.0742136753133782,-0.071123820492143,-0.0675672289899856,-0.063782921540619,
-0.0629274139542864),.UNSPECIFIED.) ;
#327=B_SPLINE_CURVE_WITH_KNOTS('',3,(#121402,#121403,#121404,#121405,#121406,
#121407,#121408,#121409),.UNSPECIFIED.,.F.,.F.,(4,2,2,4),(-0.0527017171617456,
-0.0518504523809185,-0.0480303917436524,-0.0446754473679689),
 .UNSPECIFIED.) ;
#328=B_SPLINE_CURVE_WITH_KNOTS('',3,(#121413,#121414,#121415,#121416,#121417,
#121418,#121419,#121420,#121421,#121422,#121423,#121424,#121425,#121426,
#121427,#121428,#121429,#121430,#121431,#121432,#121433,#121434,#121435,
#121436,#121437,#121438,#121439,#121440,#121441,#121442,#121443),
 .UNSPECIFIED.,.F.,.F.,(4,3,3,3,3,3,3,3,3,3,4),(0.,1.79114862983986E-5,
3.35636550441583E-5,5.14128838688763E-5,6.71346369544075E-5,8.5007692195462E-5,
0.000100614915215918,0.000118595988596873,0.000134133865285036,0.000151845157315814,
0.000156518478854401),.UNSPECIFIED.) ;
#329=B_SPLINE_CURVE_WITH_KNOTS('',3,(#121445,#121446,#121447,#121448,#121449,
#121450,#121451,#121452,#121453,#121454,#121455,#121456,#121457,#121458,
#121459,#121460,#121461,#121462,#121463,#121464,#121465,#121466),
 .UNSPECIFIED.,.F.,.F.,(4,2,2,2,2,2,2,2,2,2,4),(-0.0842935807784001,-0.0841564125369118,
-0.0836958439179285,-0.0829341785465007,-0.080592361168928,-0.0773601159633862,
-0.0742136753133782,-0.071123820492143,-0.0675672289899856,-0.063782921540619,
-0.0629274139542864),.UNSPECIFIED.) ;
#472=SHAPE_REPRESENTATION_RELATIONSHIP('SRR','None',#126602,#478) ;
#478=ADVANCED_BREP_SHAPE_REPRESENTATION('',(#4179),#126568) ;
#1939=STYLED_ITEM('',(#126640),#65362) ;
#1940=STYLED_ITEM('',(#126640),#65363) ;
#1941=STYLED_ITEM('',(#126640),#65364) ;
#1942=STYLED_ITEM('',(#126640),#65365) ;
#1943=STYLED_ITEM('',(#126640),#65366) ;
#1944=STYLED_ITEM('',(#126640),#65367) ;
#1945=STYLED_ITEM('',(#126640),#65368) ;
#1946=STYLED_ITEM('',(#126640),#65369) ;
#1947=STYLED_ITEM('',(#126640),#65370) ;
#1948=STYLED_ITEM('',(#126640),#65371) ;
#1949=STYLED_ITEM('',(#126640),#65372) ;
#1950=STYLED_ITEM('',(#126640),#65373) ;
#1951=STYLED_ITEM('',(#126640),#65374) ;
#1952=STYLED_ITEM('',(#126640),#65375) ;
#1953=STYLED_ITEM('',(#126640),#65376) ;
#1954=STYLED_ITEM('',(#126640),#65377) ;
#1955=STYLED_ITEM('',(#126640),#65378) ;
#1956=STYLED_ITEM('',(#126640),#65379) ;
#1957=STYLED_ITEM('',(#126640),#65380) ;
#1958=STYLED_ITEM('',(#126640),#65381) ;
#1959=STYLED_ITEM('',(#126640),#65382) ;
#1960=STYLED_ITEM('',(#126640),#65383) ;
#1961=STYLED_ITEM('',(#126640),#65384) ;
#1962=STYLED_ITEM('',(#126640),#65385) ;
#1963=STYLED_ITEM('',(#126640),#65386) ;
#1964=STYLED_ITEM('',(#126640),#65387) ;
#1965=STYLED_ITEM('',(#126640),#65388) ;
#1966=STYLED_ITEM('',(#126640),#65389) ;
#1967=STYLED_ITEM('',(#126640),#65390) ;
#1968=STYLED_ITEM('',(#126640),#65391) ;
#1969=STYLED_ITEM('',(#126640),#65392) ;
#1970=STYLED_ITEM('',(#126640),#65393) ;
#1971=STYLED_ITEM('',(#126640),#65394) ;
#1972=STYLED_ITEM('',(#126640),#65395) ;
#1973=STYLED_ITEM('',(#126640),#65396) ;
#1974=STYLED_ITEM('',(#126640),#65397) ;
#1975=STYLED_ITEM('',(#126640),#65398) ;
#1976=STYLED_ITEM('',(#126640),#65399) ;
#1977=STYLED_ITEM('',(#126640),#65400) ;
#1978=STYLED_ITEM('',(#126640),#65401) ;
#1979=STYLED_ITEM('',(#126640),#65402) ;
#1980=STYLED_ITEM('',(#126640),#65403) ;
#1981=STYLED_ITEM('',(#126640),#65404) ;
#1982=STYLED_ITEM('',(#126640),#65405) ;
#1983=STYLED_ITEM('',(#126640),#65406) ;
#1984=STYLED_ITEM('',(#126640),#65407) ;
#1985=STYLED_ITEM('',(#126640),#65408) ;
#1986=STYLED_ITEM('',(#126640),#65409) ;
#1987=STYLED_ITEM('',(#126640),#65410) ;
#1988=STYLED_ITEM('',(#126640),#65411) ;
#1989=STYLED_ITEM('',(#126640),#65412) ;
#1990=STYLED_ITEM('',(#126640),#65413) ;
#1991=STYLED_ITEM('',(#126640),#65414) ;
#1992=STYLED_ITEM('',(#126640),#65415) ;
#1993=STYLED_ITEM('',(#126640),#65416) ;
#1994=STYLED_ITEM('',(#126640),#65417) ;
#1995=STYLED_ITEM('',(#126640),#65418) ;
#1996=STYLED_ITEM('',(#126640),#65419) ;
#1997=STYLED_ITEM('',(#126640),#65420) ;
#1998=STYLED_ITEM('',(#126640),#65421) ;
#1999=STYLED_ITEM('',(#126640),#65422) ;
#2000=STYLED_ITEM('',(#126640),#65423) ;
#2001=STYLED_ITEM('',(#126640),#65424) ;
#2002=STYLED_ITEM('',(#126640),#65425) ;
#2003=STYLED_ITEM('',(#126640),#65426) ;
#2004=STYLED_ITEM('',(#126640),#65427) ;
#2005=STYLED_ITEM('',(#126640),#65428) ;
#2006=STYLED_ITEM('',(#126640),#65429) ;
#2007=STYLED_ITEM('',(#126640),#65430) ;
#2008=STYLED_ITEM('',(#126640),#65431) ;
#2009=STYLED_ITEM('',(#126640),#65432) ;
#2010=STYLED_ITEM('',(#126640),#65433) ;
#2011=STYLED_ITEM('',(#126640),#65434) ;
#2012=STYLED_ITEM('',(#126640),#65435) ;
#2013=STYLED_ITEM('',(#126640),#65436) ;
#2014=STYLED_ITEM('',(#126640),#65437) ;
#2015=STYLED_ITEM('',(#126640),#65438) ;
#2016=STYLED_ITEM('',(#126640),#65439) ;
#2017=STYLED_ITEM('',(#126640),#65440) ;
#2018=STYLED_ITEM('',(#126640),#65441) ;
#2019=STYLED_ITEM('',(#126640),#65442) ;
#2020=STYLED_ITEM('',(#126640),#65443) ;
#2021=STYLED_ITEM('',(#126640),#65444) ;
#2022=STYLED_ITEM('',(#126640),#65445) ;
#2023=STYLED_ITEM('',(#126640),#65446) ;
#2024=STYLED_ITEM('',(#126640),#65447) ;
#2025=STYLED_ITEM('',(#126640),#65448) ;
#2026=STYLED_ITEM('',(#126640),#65449) ;
#2027=STYLED_ITEM('',(#126640),#65450) ;
#2028=STYLED_ITEM('',(#126640),#65451) ;
#2029=STYLED_ITEM('',(#126640),#65452) ;
#2030=STYLED_ITEM('',(#126640),#65453) ;
#2031=STYLED_ITEM('',(#126640),#65454) ;
#2032=STYLED_ITEM('',(#126640),#65455) ;
#2033=STYLED_ITEM('',(#126640),#65456) ;
#2034=STYLED_ITEM('',(#126640),#65457) ;
#2035=STYLED_ITEM('',(#126640),#65458) ;
#2036=STYLED_ITEM('',(#126640),#65459) ;
#2037=STYLED_ITEM('',(#126640),#65460) ;
#2038=STYLED_ITEM('',(#126640),#65461) ;
#2039=STYLED_ITEM('',(#126640),#65462) ;
#2040=STYLED_ITEM('',(#126640),#65463) ;
#2041=STYLED_ITEM('',(#126640),#65464) ;
#2042=STYLED_ITEM('',(#126640),#65465) ;
#2043=STYLED_ITEM('',(#126640),#65466) ;
#2044=STYLED_ITEM('',(#126640),#65467) ;
#2045=STYLED_ITEM('',(#126640),#65468) ;
#2046=STYLED_ITEM('',(#126640),#65469) ;
#2047=STYLED_ITEM('',(#126640),#65470) ;
#2048=STYLED_ITEM('',(#126640),#65471) ;
#2049=STYLED_ITEM('',(#126640),#65472) ;
#2050=STYLED_ITEM('',(#126640),#65473) ;
#2051=STYLED_ITEM('',(#126640),#65474) ;
#2052=STYLED_ITEM('',(#126640),#65475) ;
#2053=STYLED_ITEM('',(#126640),#65476) ;
#2054=STYLED_ITEM('',(#126640),#65477) ;
#2055=STYLED_ITEM('',(#126640),#65478) ;
#2056=STYLED_ITEM('',(#126640),#65479) ;
#2057=STYLED_ITEM('',(#126640),#65480) ;
#2058=STYLED_ITEM('',(#126640),#65481) ;
#2059=STYLED_ITEM('',(#126640),#65482) ;
#2060=STYLED_ITEM('',(#126640),#65483) ;
#2061=STYLED_ITEM('',(#126640),#65484) ;
#2062=STYLED_ITEM('',(#126640),#65485) ;
#2063=STYLED_ITEM('',(#126640),#65486) ;
#2064=STYLED_ITEM('',(#126640),#65487) ;
#2065=STYLED_ITEM('',(#126640),#65488) ;
#2066=STYLED_ITEM('',(#126640),#65489) ;
#2067=STYLED_ITEM('',(#126640),#65490) ;
#2068=STYLED_ITEM('',(#126640),#65491) ;
#2069=STYLED_ITEM('',(#126640),#65492) ;
#2070=STYLED_ITEM('',(#126640),#65493) ;
#2071=STYLED_ITEM('',(#126640),#65494) ;
#2072=STYLED_ITEM('',(#126640),#65495) ;
#2073=STYLED_ITEM('',(#126640),#65496) ;
#2074=STYLED_ITEM('',(#126640),#65497) ;
#2075=STYLED_ITEM('',(#126640),#65498) ;
#2076=STYLED_ITEM('',(#126640),#65499) ;
#2077=STYLED_ITEM('',(#126640),#65500) ;
#2078=STYLED_ITEM('',(#126640),#65501) ;
#2079=STYLED_ITEM('',(#126640),#65502) ;
#2080=STYLED_ITEM('',(#126640),#65503) ;
#2081=STYLED_ITEM('',(#126640),#65504) ;
#2082=STYLED_ITEM('',(#126640),#65505) ;
#2083=STYLED_ITEM('',(#126640),#65506) ;
#2084=STYLED_ITEM('',(#126640),#65507) ;
#2085=STYLED_ITEM('',(#126640),#65508) ;
#2086=STYLED_ITEM('',(#126640),#65509) ;
#2087=STYLED_ITEM('',(#126640),#65510) ;
#2088=STYLED_ITEM('',(#126640),#65511) ;
#2089=STYLED_ITEM('',(#126640),#65512) ;
#2090=STYLED_ITEM('',(#126640),#65513) ;
#2091=STYLED_ITEM('',(#126640),#65514) ;
#2092=STYLED_ITEM('',(#126640),#65515) ;
#2093=STYLED_ITEM('',(#126640),#65516) ;
#2094=STYLED_ITEM('',(#126640),#65517) ;
#2095=STYLED_ITEM('',(#126640),#65518) ;
#2096=STYLED_ITEM('',(#126640),#65519) ;
#2097=STYLED_ITEM('',(#126640),#65520) ;
#2098=STYLED_ITEM('',(#126640),#65521) ;
#2099=STYLED_ITEM('',(#126640),#65522) ;
#2100=STYLED_ITEM('',(#126640),#65523) ;
#2101=STYLED_ITEM('',(#126640),#65524) ;
#2102=STYLED_ITEM('',(#126640),#65525) ;
#2103=STYLED_ITEM('',(#126640),#65526) ;
#2104=STYLED_ITEM('',(#126640),#65527) ;
#2105=STYLED_ITEM('',(#126640),#65528) ;
#2106=STYLED_ITEM('',(#126640),#65529) ;
#2107=STYLED_ITEM('',(#126640),#65530) ;
#2108=STYLED_ITEM('',(#126640),#65531) ;
#2109=STYLED_ITEM('',(#126640),#65532) ;
#2110=STYLED_ITEM('',(#126640),#65533) ;
#2111=STYLED_ITEM('',(#126640),#65534) ;
#2112=STYLED_ITEM('',(#126640),#65535) ;
#2113=STYLED_ITEM('',(#126640),#65536) ;
#2114=STYLED_ITEM('',(#126640),#65537) ;
#2115=STYLED_ITEM('',(#126640),#65538) ;
#2116=STYLED_ITEM('',(#126640),#65539) ;
#2117=STYLED_ITEM('',(#126640),#65540) ;
#2118=STYLED_ITEM('',(#126640),#65541) ;
#2119=STYLED_ITEM('',(#126640),#65542) ;
#2120=STYLED_ITEM('',(#126640),#65543) ;
#2121=STYLED_ITEM('',(#126640),#65544) ;
#2122=STYLED_ITEM('',(#126640),#65545) ;
#2123=STYLED_ITEM('',(#126640),#65546) ;
#2124=STYLED_ITEM('',(#126640),#65547) ;
#2125=STYLED_ITEM('',(#126640),#65548) ;
#2126=STYLED_ITEM('',(#126640),#65549) ;
#2127=STYLED_ITEM('',(#126640),#65550) ;
#2128=STYLED_ITEM('',(#126640),#65551) ;
#2129=STYLED_ITEM('',(#126640),#65552) ;
#2130=STYLED_ITEM('',(#126640),#65553) ;
#2131=STYLED_ITEM('',(#126640),#65554) ;
#2132=STYLED_ITEM('',(#126640),#65555) ;
#2133=STYLED_ITEM('',(#126640),#65556) ;
#2134=STYLED_ITEM('',(#126640),#65557) ;
#2135=STYLED_ITEM('',(#126640),#65558) ;
#2136=STYLED_ITEM('',(#126640),#65559) ;
#2137=STYLED_ITEM('',(#126640),#65560) ;
#2138=STYLED_ITEM('',(#126640),#65561) ;
#2139=STYLED_ITEM('',(#126640),#65562) ;
#2140=STYLED_ITEM('',(#126640),#65563) ;
#2141=STYLED_ITEM('',(#126640),#65564) ;
#2142=STYLED_ITEM('',(#126640),#65565) ;
#2143=STYLED_ITEM('',(#126640),#65566) ;
#2144=STYLED_ITEM('',(#126640),#65567) ;
#2145=STYLED_ITEM('',(#126640),#65568) ;
#2146=STYLED_ITEM('',(#126640),#65569) ;
#2147=STYLED_ITEM('',(#126640),#65570) ;
#2148=STYLED_ITEM('',(#126640),#65571) ;
#2149=STYLED_ITEM('',(#126640),#65572) ;
#2150=STYLED_ITEM('',(#126640),#65573) ;
#2151=STYLED_ITEM('',(#126640),#65574) ;
#2152=STYLED_ITEM('',(#126640),#65575) ;
#2153=STYLED_ITEM('',(#126640),#65576) ;
#2154=STYLED_ITEM('',(#126640),#65577) ;
#2155=STYLED_ITEM('',(#126640),#65578) ;
#2156=STYLED_ITEM('',(#126640),#65579) ;
#2157=STYLED_ITEM('',(#126640),#65580) ;
#2158=STYLED_ITEM('',(#126640),#65581) ;
#2159=STYLED_ITEM('',(#126640),#65582) ;
#2160=STYLED_ITEM('',(#126640),#65583) ;
#2161=STYLED_ITEM('',(#126640),#65584) ;
#2162=STYLED_ITEM('',(#126640),#65585) ;
#2163=STYLED_ITEM('',(#126640),#65586) ;
#2164=STYLED_ITEM('',(#126640),#65587) ;
#2165=STYLED_ITEM('',(#126640),#65588) ;
#2166=STYLED_ITEM('',(#126640),#65589) ;
#2167=STYLED_ITEM('',(#126640),#65590) ;
#2168=STYLED_ITEM('',(#126640),#65591) ;
#2169=STYLED_ITEM('',(#126640),#65592) ;
#2170=STYLED_ITEM('',(#126640),#65593) ;
#2171=STYLED_ITEM('',(#126640),#65594) ;
#2172=STYLED_ITEM('',(#126640),#65595) ;
#2173=STYLED_ITEM('',(#126640),#65596) ;
#2174=STYLED_ITEM('',(#126640),#65597) ;
#2175=STYLED_ITEM('',(#126640),#65598) ;
#2176=STYLED_ITEM('',(#126640),#65599) ;
#2177=STYLED_ITEM('',(#126640),#65600) ;
#2178=STYLED_ITEM('',(#126640),#65601) ;
#2179=STYLED_ITEM('',(#126640),#65602) ;
#2180=STYLED_ITEM('',(#126640),#65603) ;
#2181=STYLED_ITEM('',(#126640),#65604) ;
#2182=STYLED_ITEM('',(#126640),#65605) ;
#2183=STYLED_ITEM('',(#126640),#65606) ;
#2184=STYLED_ITEM('',(#126640),#65607) ;
#2185=STYLED_ITEM('',(#126640),#65608) ;
#2186=STYLED_ITEM('',(#126640),#65609) ;
#2187=STYLED_ITEM('',(#126640),#65610) ;
#2188=STYLED_ITEM('',(#126640),#65611) ;
#2189=STYLED_ITEM('',(#126640),#65612) ;
#2190=STYLED_ITEM('',(#126640),#65613) ;
#2191=STYLED_ITEM('',(#126640),#65614) ;
#2192=STYLED_ITEM('',(#126640),#65615) ;
#2193=STYLED_ITEM('',(#126640),#65616) ;
#2194=STYLED_ITEM('',(#126640),#65617) ;
#2195=STYLED_ITEM('',(#126640),#65618) ;
#2196=STYLED_ITEM('',(#126640),#65619) ;
#2197=STYLED_ITEM('',(#126640),#65620) ;
#2198=STYLED_ITEM('',(#126640),#65621) ;
#2199=STYLED_ITEM('',(#126640),#65622) ;
#2200=STYLED_ITEM('',(#126640),#65623) ;
#2201=STYLED_ITEM('',(#126640),#65624) ;
#2202=STYLED_ITEM('',(#126640),#65625) ;
#2203=STYLED_ITEM('',(#126640),#65626) ;
#2204=STYLED_ITEM('',(#126640),#65627) ;
#2205=STYLED_ITEM('',(#126640),#65628) ;
#2206=STYLED_ITEM('',(#126640),#65629) ;
#2207=STYLED_ITEM('',(#126640),#65630) ;
#2208=STYLED_ITEM('',(#126640),#65631) ;
#2209=STYLED_ITEM('',(#126640),#65632) ;
#2210=STYLED_ITEM('',(#126640),#65633) ;
#2211=STYLED_ITEM('',(#126640),#65634) ;
#2212=STYLED_ITEM('',(#126640),#65635) ;
#2213=STYLED_ITEM('',(#126640),#65636) ;
#2214=STYLED_ITEM('',(#126640),#65637) ;
#2215=STYLED_ITEM('',(#126640),#65638) ;
#2216=STYLED_ITEM('',(#126640),#65639) ;
#2217=STYLED_ITEM('',(#126640),#65640) ;
#2218=STYLED_ITEM('',(#126640),#65641) ;
#2219=STYLED_ITEM('',(#126640),#65642) ;
#2220=STYLED_ITEM('',(#126640),#65643) ;
#2221=STYLED_ITEM('',(#126640),#65644) ;
#2222=STYLED_ITEM('',(#126640),#65645) ;
#2223=STYLED_ITEM('',(#126640),#65646) ;
#2224=STYLED_ITEM('',(#126640),#65647) ;
#2225=STYLED_ITEM('',(#126640),#65648) ;
#2226=STYLED_ITEM('',(#126640),#65649) ;
#2227=STYLED_ITEM('',(#126640),#65650) ;
#2228=STYLED_ITEM('',(#126640),#65651) ;
#2229=STYLED_ITEM('',(#126640),#65652) ;
#2230=STYLED_ITEM('',(#126640),#65653) ;
#2231=STYLED_ITEM('',(#126640),#65654) ;
#2232=STYLED_ITEM('',(#126640),#65655) ;
#2233=STYLED_ITEM('',(#126640),#65656) ;
#2234=STYLED_ITEM('',(#126641),#65657) ;
#2235=STYLED_ITEM('',(#126641),#65658) ;
#2236=STYLED_ITEM('',(#126641),#65659) ;
#2237=STYLED_ITEM('',(#126641),#65660) ;
#2238=STYLED_ITEM('',(#126641),#65661) ;
#2239=STYLED_ITEM('',(#126641),#65662) ;
#2240=STYLED_ITEM('',(#126641),#65663) ;
#2241=STYLED_ITEM('',(#126641),#65664) ;
#2242=STYLED_ITEM('',(#126641),#65665) ;
#2243=STYLED_ITEM('',(#126641),#65666) ;
#2244=STYLED_ITEM('',(#126641),#65667) ;
#2245=STYLED_ITEM('',(#126641),#65668) ;
#2246=STYLED_ITEM('',(#126641),#65669) ;
#2247=STYLED_ITEM('',(#126641),#65670) ;
#2248=STYLED_ITEM('',(#126641),#65671) ;
#2249=STYLED_ITEM('',(#126641),#65672) ;
#2250=STYLED_ITEM('',(#126641),#65673) ;
#2251=STYLED_ITEM('',(#126641),#65674) ;
#2252=STYLED_ITEM('',(#126641),#65675) ;
#2253=STYLED_ITEM('',(#126641),#65676) ;
#2254=STYLED_ITEM('',(#126641),#65677) ;
#2255=STYLED_ITEM('',(#126641),#65678) ;
#2256=STYLED_ITEM('',(#126641),#65679) ;
#2257=STYLED_ITEM('',(#126641),#65680) ;
#2258=STYLED_ITEM('',(#126641),#65681) ;
#2259=STYLED_ITEM('',(#126641),#65682) ;
#2260=STYLED_ITEM('',(#126641),#65683) ;
#2261=STYLED_ITEM('',(#126641),#65684) ;
#2262=STYLED_ITEM('',(#126641),#65685) ;
#2263=STYLED_ITEM('',(#126641),#65686) ;
#2264=STYLED_ITEM('',(#126641),#65687) ;
#2265=STYLED_ITEM('',(#126641),#65688) ;
#2266=STYLED_ITEM('',(#126641),#65689) ;
#2267=STYLED_ITEM('',(#126641),#65690) ;
#2268=STYLED_ITEM('',(#126641),#65691) ;
#2269=STYLED_ITEM('',(#126641),#65692) ;
#2270=STYLED_ITEM('',(#126641),#65693) ;
#2271=STYLED_ITEM('',(#126641),#65694) ;
#2272=STYLED_ITEM('',(#126641),#65695) ;
#2273=STYLED_ITEM('',(#126641),#65696) ;
#2274=STYLED_ITEM('',(#126641),#65697) ;
#2275=STYLED_ITEM('',(#126641),#65698) ;
#2276=STYLED_ITEM('',(#126641),#65699) ;
#2277=STYLED_ITEM('',(#126641),#65700) ;
#2278=STYLED_ITEM('',(#126641),#65701) ;
#2279=STYLED_ITEM('',(#126641),#65702) ;
#2280=STYLED_ITEM('',(#126641),#65703) ;
#2281=STYLED_ITEM('',(#126641),#65704) ;
#2282=STYLED_ITEM('',(#126641),#65705) ;
#2283=STYLED_ITEM('',(#126641),#65706) ;
#2284=STYLED_ITEM('',(#126641),#65707) ;
#2285=STYLED_ITEM('',(#126641),#65708) ;
#2286=STYLED_ITEM('',(#126641),#65709) ;
#2287=STYLED_ITEM('',(#126641),#65710) ;
#2288=STYLED_ITEM('',(#126641),#65711) ;
#2289=STYLED_ITEM('',(#126641),#65712) ;
#2290=STYLED_ITEM('',(#126641),#65713) ;
#2291=STYLED_ITEM('',(#126641),#65714) ;
#2292=STYLED_ITEM('',(#126641),#65715) ;
#2293=STYLED_ITEM('',(#126641),#65716) ;
#2294=STYLED_ITEM('',(#126641),#65717) ;
#2295=STYLED_ITEM('',(#126641),#65718) ;
#2296=STYLED_ITEM('',(#126641),#65719) ;
#2297=STYLED_ITEM('',(#126641),#65720) ;
#2298=STYLED_ITEM('',(#126641),#65721) ;
#2299=STYLED_ITEM('',(#126641),#65722) ;
#2300=STYLED_ITEM('',(#126641),#65723) ;
#2301=STYLED_ITEM('',(#126641),#65724) ;
#2302=STYLED_ITEM('',(#126641),#65725) ;
#2303=STYLED_ITEM('',(#126641),#65726) ;
#2304=STYLED_ITEM('',(#126641),#65727) ;
#2305=STYLED_ITEM('',(#126641),#65728) ;
#2306=STYLED_ITEM('',(#126640),#65729) ;
#2307=STYLED_ITEM('',(#126640),#65730) ;
#2308=STYLED_ITEM('',(#126640),#65731) ;
#2309=STYLED_ITEM('',(#126640),#65732) ;
#2310=STYLED_ITEM('',(#126640),#65733) ;
#2311=STYLED_ITEM('',(#126640),#65734) ;
#2312=STYLED_ITEM('',(#126640),#65735) ;
#2313=STYLED_ITEM('',(#126640),#65736) ;
#2314=STYLED_ITEM('',(#126640),#65737) ;
#2315=STYLED_ITEM('',(#126640),#65738) ;
#2316=STYLED_ITEM('',(#126640),#65739) ;
#2317=STYLED_ITEM('',(#126640),#65740) ;
#2318=STYLED_ITEM('',(#126640),#65741) ;
#2319=STYLED_ITEM('',(#126640),#65742) ;
#2320=STYLED_ITEM('',(#126640),#65743) ;
#2321=STYLED_ITEM('',(#126640),#65744) ;
#2322=STYLED_ITEM('',(#126640),#65745) ;
#2323=STYLED_ITEM('',(#126640),#65746) ;
#2324=STYLED_ITEM('',(#126640),#65747) ;
#2325=STYLED_ITEM('',(#126640),#65748) ;
#2326=STYLED_ITEM('',(#126640),#65749) ;
#2327=STYLED_ITEM('',(#126640),#65750) ;
#2328=STYLED_ITEM('',(#126640),#65751) ;
#2329=STYLED_ITEM('',(#126640),#65752) ;
#2330=STYLED_ITEM('',(#126640),#65753) ;
#2331=STYLED_ITEM('',(#126640),#65754) ;
#2332=STYLED_ITEM('',(#126640),#65755) ;
#2333=STYLED_ITEM('',(#126640),#65756) ;
#2334=STYLED_ITEM('',(#126640),#65757) ;
#2335=STYLED_ITEM('',(#126640),#65758) ;
#2336=STYLED_ITEM('',(#126640),#65759) ;
#2337=STYLED_ITEM('',(#126640),#65760) ;
#2338=STYLED_ITEM('',(#126640),#65761) ;
#2339=STYLED_ITEM('',(#126640),#65762) ;
#2340=STYLED_ITEM('',(#126640),#65763) ;
#2341=STYLED_ITEM('',(#126640),#65764) ;
#2342=STYLED_ITEM('',(#126640),#65765) ;
#2343=STYLED_ITEM('',(#126640),#65766) ;
#2344=STYLED_ITEM('',(#126640),#65767) ;
#2345=STYLED_ITEM('',(#126640),#65768) ;
#2346=STYLED_ITEM('',(#126640),#65769) ;
#2347=STYLED_ITEM('',(#126640),#65770) ;
#2348=STYLED_ITEM('',(#126640),#65771) ;
#2349=STYLED_ITEM('',(#126640),#65772) ;
#2350=STYLED_ITEM('',(#126640),#65773) ;
#2351=STYLED_ITEM('',(#126640),#65774) ;
#2352=STYLED_ITEM('',(#126640),#65775) ;
#2353=STYLED_ITEM('',(#126640),#65776) ;
#2354=STYLED_ITEM('',(#126640),#65777) ;
#2355=STYLED_ITEM('',(#126640),#65778) ;
#2356=STYLED_ITEM('',(#126640),#65779) ;
#2357=STYLED_ITEM('',(#126640),#65780) ;
#2358=STYLED_ITEM('',(#126640),#65781) ;
#2359=STYLED_ITEM('',(#126640),#65782) ;
#2360=STYLED_ITEM('',(#126640),#65783) ;
#2361=STYLED_ITEM('',(#126640),#65784) ;
#2362=STYLED_ITEM('',(#126640),#65785) ;
#2363=STYLED_ITEM('',(#126640),#65786) ;
#2364=STYLED_ITEM('',(#126640),#65787) ;
#2365=STYLED_ITEM('',(#126640),#65788) ;
#2366=STYLED_ITEM('',(#126640),#65789) ;
#2367=STYLED_ITEM('',(#126640),#65790) ;
#2368=STYLED_ITEM('',(#126640),#65791) ;
#2369=STYLED_ITEM('',(#126640),#65792) ;
#2370=STYLED_ITEM('',(#126640),#65793) ;
#2371=STYLED_ITEM('',(#126640),#65794) ;
#2372=STYLED_ITEM('',(#126640),#65795) ;
#2373=STYLED_ITEM('',(#126640),#65796) ;
#2374=STYLED_ITEM('',(#126640),#65797) ;
#2375=STYLED_ITEM('',(#126640),#65798) ;
#2376=STYLED_ITEM('',(#126640),#65799) ;
#2377=STYLED_ITEM('',(#126640),#65800) ;
#2378=STYLED_ITEM('',(#126640),#65801) ;
#2379=STYLED_ITEM('',(#126640),#65802) ;
#2380=STYLED_ITEM('',(#126640),#65803) ;
#2381=STYLED_ITEM('',(#126640),#65804) ;
#2382=STYLED_ITEM('',(#126640),#65805) ;
#2383=STYLED_ITEM('',(#126640),#65806) ;
#2384=STYLED_ITEM('',(#126640),#65807) ;
#2385=STYLED_ITEM('',(#126640),#65808) ;
#2386=STYLED_ITEM('',(#126640),#65809) ;
#2387=STYLED_ITEM('',(#126640),#65810) ;
#2388=STYLED_ITEM('',(#126640),#65811) ;
#2389=STYLED_ITEM('',(#126640),#65812) ;
#2390=STYLED_ITEM('',(#126640),#65813) ;
#2391=STYLED_ITEM('',(#126640),#65814) ;
#2392=STYLED_ITEM('',(#126640),#65815) ;
#2393=STYLED_ITEM('',(#126640),#65816) ;
#2394=STYLED_ITEM('',(#126640),#65817) ;
#2395=STYLED_ITEM('',(#126640),#65818) ;
#2396=STYLED_ITEM('',(#126640),#65819) ;
#2397=STYLED_ITEM('',(#126640),#65820) ;
#2398=STYLED_ITEM('',(#126640),#65821) ;
#2399=STYLED_ITEM('',(#126640),#65822) ;
#2400=STYLED_ITEM('',(#126640),#65823) ;
#2401=STYLED_ITEM('',(#126640),#65824) ;
#2402=STYLED_ITEM('',(#126640),#65825) ;
#2403=STYLED_ITEM('',(#126640),#65826) ;
#2404=STYLED_ITEM('',(#126640),#65827) ;
#2405=STYLED_ITEM('',(#126640),#65828) ;
#2406=STYLED_ITEM('',(#126640),#65829) ;
#2407=STYLED_ITEM('',(#126640),#65830) ;
#2408=STYLED_ITEM('',(#126640),#65831) ;
#2409=STYLED_ITEM('',(#126640),#65832) ;
#2410=STYLED_ITEM('',(#126640),#65833) ;
#2411=STYLED_ITEM('',(#126640),#65834) ;
#2412=STYLED_ITEM('',(#126640),#65835) ;
#2413=STYLED_ITEM('',(#126640),#65836) ;
#2414=STYLED_ITEM('',(#126640),#65837) ;
#2415=STYLED_ITEM('',(#126640),#65838) ;
#2416=STYLED_ITEM('',(#126640),#65839) ;
#2417=STYLED_ITEM('',(#126640),#65840) ;
#2418=STYLED_ITEM('',(#126640),#65841) ;
#2419=STYLED_ITEM('',(#126640),#65842) ;
#2420=STYLED_ITEM('',(#126640),#65843) ;
#2421=STYLED_ITEM('',(#126640),#65844) ;
#2422=STYLED_ITEM('',(#126640),#65845) ;
#2423=STYLED_ITEM('',(#126640),#65846) ;
#2424=STYLED_ITEM('',(#126640),#65847) ;
#2425=STYLED_ITEM('',(#126640),#65848) ;
#2426=STYLED_ITEM('',(#126640),#65849) ;
#2427=STYLED_ITEM('',(#126640),#65850) ;
#2428=STYLED_ITEM('',(#126640),#65851) ;
#2429=STYLED_ITEM('',(#126640),#65852) ;
#2430=STYLED_ITEM('',(#126640),#65853) ;
#2431=STYLED_ITEM('',(#126640),#65854) ;
#2432=STYLED_ITEM('',(#126640),#65855) ;
#2433=STYLED_ITEM('',(#126640),#65856) ;
#2434=STYLED_ITEM('',(#126640),#65857) ;
#2435=STYLED_ITEM('',(#126640),#65858) ;
#2436=STYLED_ITEM('',(#126640),#65859) ;
#2437=STYLED_ITEM('',(#126640),#65860) ;
#2438=STYLED_ITEM('',(#126640),#65861) ;
#2439=STYLED_ITEM('',(#126640),#65862) ;
#2440=STYLED_ITEM('',(#126640),#65863) ;
#2441=STYLED_ITEM('',(#126640),#65864) ;
#2442=STYLED_ITEM('',(#126640),#65865) ;
#2443=STYLED_ITEM('',(#126640),#65866) ;
#2444=STYLED_ITEM('',(#126640),#65867) ;
#2445=STYLED_ITEM('',(#126640),#65868) ;
#2446=STYLED_ITEM('',(#126640),#65869) ;
#2447=STYLED_ITEM('',(#126640),#65870) ;
#2448=STYLED_ITEM('',(#126640),#65871) ;
#2449=STYLED_ITEM('',(#126640),#65872) ;
#2450=STYLED_ITEM('',(#126640),#65873) ;
#2451=STYLED_ITEM('',(#126640),#65874) ;
#2452=STYLED_ITEM('',(#126640),#65875) ;
#2453=STYLED_ITEM('',(#126640),#65876) ;
#2454=STYLED_ITEM('',(#126640),#65877) ;
#2455=STYLED_ITEM('',(#126640),#65878) ;
#2456=STYLED_ITEM('',(#126640),#65879) ;
#2457=STYLED_ITEM('',(#126640),#65880) ;
#2458=STYLED_ITEM('',(#126640),#65881) ;
#2459=STYLED_ITEM('',(#126640),#65882) ;
#2460=STYLED_ITEM('',(#126640),#65883) ;
#2461=STYLED_ITEM('',(#126640),#65884) ;
#2462=STYLED_ITEM('',(#126640),#65885) ;
#2463=STYLED_ITEM('',(#126640),#65886) ;
#2464=STYLED_ITEM('',(#126640),#65887) ;
#2465=STYLED_ITEM('',(#126640),#65888) ;
#2466=STYLED_ITEM('',(#126640),#65889) ;
#2467=STYLED_ITEM('',(#126640),#65890) ;
#2468=STYLED_ITEM('',(#126640),#65891) ;
#2469=STYLED_ITEM('',(#126640),#65892) ;
#2470=STYLED_ITEM('',(#126640),#65893) ;
#2471=STYLED_ITEM('',(#126640),#65894) ;
#2472=STYLED_ITEM('',(#126640),#65895) ;
#2473=STYLED_ITEM('',(#126640),#65896) ;
#2474=STYLED_ITEM('',(#126640),#65897) ;
#2475=STYLED_ITEM('',(#126640),#65898) ;
#2476=STYLED_ITEM('',(#126640),#65899) ;
#2477=STYLED_ITEM('',(#126640),#65900) ;
#2478=STYLED_ITEM('',(#126640),#65901) ;
#2479=STYLED_ITEM('',(#126640),#65902) ;
#2480=STYLED_ITEM('',(#126640),#65903) ;
#2481=STYLED_ITEM('',(#126640),#65904) ;
#2482=STYLED_ITEM('',(#126640),#65905) ;
#2483=STYLED_ITEM('',(#126640),#65906) ;
#2484=STYLED_ITEM('',(#126640),#65907) ;
#2485=STYLED_ITEM('',(#126640),#65908) ;
#2486=STYLED_ITEM('',(#126640),#65909) ;
#2487=STYLED_ITEM('',(#126640),#65910) ;
#2488=STYLED_ITEM('',(#126640),#65911) ;
#2489=STYLED_ITEM('',(#126640),#65912) ;
#2490=STYLED_ITEM('',(#126640),#65913) ;
#2491=STYLED_ITEM('',(#126640),#65914) ;
#2492=STYLED_ITEM('',(#126640),#65915) ;
#2493=STYLED_ITEM('',(#126640),#65916) ;
#2494=STYLED_ITEM('',(#126640),#65917) ;
#2495=STYLED_ITEM('',(#126640),#65918) ;
#2496=STYLED_ITEM('',(#126640),#65919) ;
#2497=STYLED_ITEM('',(#126640),#65920) ;
#2498=STYLED_ITEM('',(#126640),#65921) ;
#2499=STYLED_ITEM('',(#126640),#65922) ;
#2500=STYLED_ITEM('',(#126640),#65923) ;
#2501=STYLED_ITEM('',(#126640),#65924) ;
#2502=STYLED_ITEM('',(#126640),#65925) ;
#2503=STYLED_ITEM('',(#126640),#65926) ;
#2504=STYLED_ITEM('',(#126640),#65927) ;
#2505=STYLED_ITEM('',(#126640),#65928) ;
#2506=STYLED_ITEM('',(#126640),#65929) ;
#2507=STYLED_ITEM('',(#126640),#65930) ;
#2508=STYLED_ITEM('',(#126640),#65931) ;
#2509=STYLED_ITEM('',(#126640),#65932) ;
#2510=STYLED_ITEM('',(#126640),#65933) ;
#2511=STYLED_ITEM('',(#126640),#65934) ;
#2512=STYLED_ITEM('',(#126640),#65935) ;
#2513=STYLED_ITEM('',(#126640),#65936) ;
#2514=STYLED_ITEM('',(#126640),#65937) ;
#2515=STYLED_ITEM('',(#126640),#65938) ;
#2516=STYLED_ITEM('',(#126640),#65939) ;
#2517=STYLED_ITEM('',(#126640),#65940) ;
#2518=STYLED_ITEM('',(#126640),#65941) ;
#2519=STYLED_ITEM('',(#126640),#65942) ;
#2520=STYLED_ITEM('',(#126640),#65943) ;
#2521=STYLED_ITEM('',(#126640),#65944) ;
#2522=STYLED_ITEM('',(#126640),#65945) ;
#2523=STYLED_ITEM('',(#126640),#65946) ;
#2524=STYLED_ITEM('',(#126640),#65947) ;
#2525=STYLED_ITEM('',(#126640),#65948) ;
#2526=STYLED_ITEM('',(#126640),#65949) ;
#2527=STYLED_ITEM('',(#126640),#65950) ;
#2528=STYLED_ITEM('',(#126640),#65951) ;
#2529=STYLED_ITEM('',(#126640),#65952) ;
#2530=STYLED_ITEM('',(#126640),#65953) ;
#2531=STYLED_ITEM('',(#126640),#65954) ;
#2532=STYLED_ITEM('',(#126640),#65955) ;
#2533=STYLED_ITEM('',(#126640),#65956) ;
#2534=STYLED_ITEM('',(#126640),#65957) ;
#2535=STYLED_ITEM('',(#126640),#65958) ;
#2536=STYLED_ITEM('',(#126640),#65959) ;
#2537=STYLED_ITEM('',(#126640),#65960) ;
#2538=STYLED_ITEM('',(#126640),#65961) ;
#2539=STYLED_ITEM('',(#126640),#65962) ;
#2540=STYLED_ITEM('',(#126640),#65963) ;
#2541=STYLED_ITEM('',(#126640),#65964) ;
#2542=STYLED_ITEM('',(#126640),#65965) ;
#2543=STYLED_ITEM('',(#126640),#65966) ;
#2544=STYLED_ITEM('',(#126640),#65967) ;
#2545=STYLED_ITEM('',(#126640),#65968) ;
#2546=STYLED_ITEM('',(#126640),#65969) ;
#2547=STYLED_ITEM('',(#126640),#65970) ;
#2548=STYLED_ITEM('',(#126640),#65971) ;
#2549=STYLED_ITEM('',(#126640),#65972) ;
#2550=STYLED_ITEM('',(#126640),#65973) ;
#2551=STYLED_ITEM('',(#126640),#65974) ;
#2552=STYLED_ITEM('',(#126640),#65975) ;
#2553=STYLED_ITEM('',(#126640),#65976) ;
#2554=STYLED_ITEM('',(#126640),#65977) ;
#2555=STYLED_ITEM('',(#126640),#65978) ;
#2556=STYLED_ITEM('',(#126640),#65979) ;
#2557=STYLED_ITEM('',(#126640),#65980) ;
#2558=STYLED_ITEM('',(#126640),#65981) ;
#2559=STYLED_ITEM('',(#126640),#65982) ;
#2560=STYLED_ITEM('',(#126640),#65983) ;
#2561=STYLED_ITEM('',(#126640),#65984) ;
#2562=STYLED_ITEM('',(#126640),#65985) ;
#2563=STYLED_ITEM('',(#126640),#65986) ;
#2564=STYLED_ITEM('',(#126640),#65987) ;
#2565=STYLED_ITEM('',(#126640),#65988) ;
#2566=STYLED_ITEM('',(#126640),#65989) ;
#2567=STYLED_ITEM('',(#126640),#65990) ;
#2568=STYLED_ITEM('',(#126640),#65991) ;
#2569=STYLED_ITEM('',(#126640),#65992) ;
#2570=STYLED_ITEM('',(#126640),#65993) ;
#2571=STYLED_ITEM('',(#126640),#65994) ;
#2572=STYLED_ITEM('',(#126640),#65995) ;
#2573=STYLED_ITEM('',(#126640),#65996) ;
#2574=STYLED_ITEM('',(#126640),#65997) ;
#2575=STYLED_ITEM('',(#126640),#65998) ;
#2576=STYLED_ITEM('',(#126640),#65999) ;
#2577=STYLED_ITEM('',(#126640),#66000) ;
#2578=STYLED_ITEM('',(#126640),#66001) ;
#2579=STYLED_ITEM('',(#126640),#66002) ;
#2580=STYLED_ITEM('',(#126640),#66003) ;
#2581=STYLED_ITEM('',(#126640),#66004) ;
#2582=STYLED_ITEM('',(#126640),#66005) ;
#2583=STYLED_ITEM('',(#126640),#66006) ;
#2584=STYLED_ITEM('',(#126640),#66007) ;
#2585=STYLED_ITEM('',(#126640),#66008) ;
#2586=STYLED_ITEM('',(#126640),#66009) ;
#2587=STYLED_ITEM('',(#126640),#66010) ;
#2588=STYLED_ITEM('',(#126640),#66011) ;
#2589=STYLED_ITEM('',(#126640),#66012) ;
#2590=STYLED_ITEM('',(#126640),#66013) ;
#2591=STYLED_ITEM('',(#126640),#66014) ;
#2592=STYLED_ITEM('',(#126640),#66015) ;
#2593=STYLED_ITEM('',(#126640),#66016) ;
#2594=STYLED_ITEM('',(#126640),#66017) ;
#2595=STYLED_ITEM('',(#126640),#66018) ;
#2596=STYLED_ITEM('',(#126640),#66019) ;
#2597=STYLED_ITEM('',(#126640),#66020) ;
#2598=STYLED_ITEM('',(#126640),#66021) ;
#2599=STYLED_ITEM('',(#126640),#66022) ;
#2600=STYLED_ITEM('',(#126640),#66023) ;
#2601=STYLED_ITEM('',(#126640),#66024) ;
#2602=STYLED_ITEM('',(#126640),#66025) ;
#2603=STYLED_ITEM('',(#126640),#66026) ;
#2604=STYLED_ITEM('',(#126640),#66027) ;
#2605=STYLED_ITEM('',(#126640),#66028) ;
#2606=STYLED_ITEM('',(#126640),#66029) ;
#2607=STYLED_ITEM('',(#126640),#66030) ;
#2608=STYLED_ITEM('',(#126640),#66031) ;
#2609=STYLED_ITEM('',(#126640),#66032) ;
#2610=STYLED_ITEM('',(#126640),#66033) ;
#2611=STYLED_ITEM('',(#126640),#66034) ;
#2612=STYLED_ITEM('',(#126640),#66035) ;
#2613=STYLED_ITEM('',(#126640),#66036) ;
#2614=STYLED_ITEM('',(#126640),#66037) ;
#2615=STYLED_ITEM('',(#126640),#66038) ;
#2616=STYLED_ITEM('',(#126640),#66039) ;
#2617=STYLED_ITEM('',(#126640),#66040) ;
#2618=STYLED_ITEM('',(#126640),#66041) ;
#2619=STYLED_ITEM('',(#126640),#66042) ;
#2620=STYLED_ITEM('',(#126640),#66043) ;
#2621=STYLED_ITEM('',(#126640),#66044) ;
#2622=STYLED_ITEM('',(#126640),#66045) ;
#2623=STYLED_ITEM('',(#126640),#66046) ;
#2624=STYLED_ITEM('',(#126640),#66047) ;
#2625=STYLED_ITEM('',(#126640),#66048) ;
#2626=STYLED_ITEM('',(#126640),#66049) ;
#2627=STYLED_ITEM('',(#126640),#66050) ;
#2628=STYLED_ITEM('',(#126640),#66051) ;
#2629=STYLED_ITEM('',(#126640),#66052) ;
#2630=STYLED_ITEM('',(#126640),#66053) ;
#2631=STYLED_ITEM('',(#126640),#66054) ;
#2632=STYLED_ITEM('',(#126640),#66055) ;
#2633=STYLED_ITEM('',(#126640),#66056) ;
#2634=STYLED_ITEM('',(#126640),#66057) ;
#2635=STYLED_ITEM('',(#126640),#66058) ;
#2636=STYLED_ITEM('',(#126640),#66059) ;
#2637=STYLED_ITEM('',(#126640),#66060) ;
#2638=STYLED_ITEM('',(#126640),#66061) ;
#2639=STYLED_ITEM('',(#126640),#66062) ;
#2640=STYLED_ITEM('',(#126640),#66063) ;
#2641=STYLED_ITEM('',(#126640),#66064) ;
#2642=STYLED_ITEM('',(#126640),#66065) ;
#2643=STYLED_ITEM('',(#126640),#66066) ;
#2644=STYLED_ITEM('',(#126640),#66067) ;
#2645=STYLED_ITEM('',(#126640),#66068) ;
#2646=STYLED_ITEM('',(#126640),#66069) ;
#2647=STYLED_ITEM('',(#126640),#66070) ;
#2648=STYLED_ITEM('',(#126640),#66071) ;
#2649=STYLED_ITEM('',(#126640),#66072) ;
#2650=STYLED_ITEM('',(#126640),#66073) ;
#2651=STYLED_ITEM('',(#126640),#66074) ;
#2652=STYLED_ITEM('',(#126640),#66075) ;
#2653=STYLED_ITEM('',(#126640),#66076) ;
#2654=STYLED_ITEM('',(#126640),#66077) ;
#2655=STYLED_ITEM('',(#126640),#66078) ;
#2656=STYLED_ITEM('',(#126640),#66079) ;
#2657=STYLED_ITEM('',(#126640),#66080) ;
#2658=STYLED_ITEM('',(#126640),#66081) ;
#2659=STYLED_ITEM('',(#126640),#66082) ;
#2660=STYLED_ITEM('',(#126640),#66083) ;
#2661=STYLED_ITEM('',(#126640),#66084) ;
#2662=STYLED_ITEM('',(#126640),#66085) ;
#2663=STYLED_ITEM('',(#126640),#66086) ;
#2664=STYLED_ITEM('',(#126640),#66087) ;
#2665=STYLED_ITEM('',(#126640),#66088) ;
#2666=STYLED_ITEM('',(#126640),#66089) ;
#2667=STYLED_ITEM('',(#126640),#66090) ;
#2668=STYLED_ITEM('',(#126640),#66091) ;
#2669=STYLED_ITEM('',(#126640),#66092) ;
#2670=STYLED_ITEM('',(#126640),#66093) ;
#2671=STYLED_ITEM('',(#126640),#66094) ;
#2672=STYLED_ITEM('',(#126640),#66095) ;
#2673=STYLED_ITEM('',(#126640),#66096) ;
#2674=STYLED_ITEM('',(#126640),#66097) ;
#2675=STYLED_ITEM('',(#126640),#66098) ;
#2676=STYLED_ITEM('',(#126640),#66099) ;
#2677=STYLED_ITEM('',(#126640),#66100) ;
#2678=STYLED_ITEM('',(#126640),#66101) ;
#2679=STYLED_ITEM('',(#126640),#66102) ;
#2680=STYLED_ITEM('',(#126640),#66103) ;
#2681=STYLED_ITEM('',(#126640),#66104) ;
#2682=STYLED_ITEM('',(#126640),#66105) ;
#2683=STYLED_ITEM('',(#126640),#66106) ;
#2684=STYLED_ITEM('',(#126640),#66107) ;
#2685=STYLED_ITEM('',(#126640),#66108) ;
#2686=STYLED_ITEM('',(#126640),#66109) ;
#2687=STYLED_ITEM('',(#126640),#66110) ;
#2688=STYLED_ITEM('',(#126640),#66111) ;
#2689=STYLED_ITEM('',(#126640),#66112) ;
#2690=STYLED_ITEM('',(#126640),#66113) ;
#2691=STYLED_ITEM('',(#126640),#66114) ;
#2692=STYLED_ITEM('',(#126640),#66115) ;
#2693=STYLED_ITEM('',(#126640),#66116) ;
#2694=STYLED_ITEM('',(#126640),#66117) ;
#2695=STYLED_ITEM('',(#126640),#66118) ;
#2696=STYLED_ITEM('',(#126640),#66119) ;
#2697=STYLED_ITEM('',(#126640),#66120) ;
#2698=STYLED_ITEM('',(#126640),#66121) ;
#2699=STYLED_ITEM('',(#126640),#66122) ;
#2700=STYLED_ITEM('',(#126640),#66123) ;
#2701=STYLED_ITEM('',(#126640),#66124) ;
#2702=STYLED_ITEM('',(#126640),#66125) ;
#2703=STYLED_ITEM('',(#126640),#66126) ;
#2704=STYLED_ITEM('',(#126640),#66127) ;
#2705=STYLED_ITEM('',(#126640),#66128) ;
#2706=STYLED_ITEM('',(#126640),#66129) ;
#2707=STYLED_ITEM('',(#126640),#66130) ;
#2708=STYLED_ITEM('',(#126640),#66131) ;
#2709=STYLED_ITEM('',(#126640),#66132) ;
#2710=STYLED_ITEM('',(#126640),#66133) ;
#2711=STYLED_ITEM('',(#126640),#66134) ;
#2712=STYLED_ITEM('',(#126640),#66135) ;
#2713=STYLED_ITEM('',(#126640),#66136) ;
#2714=STYLED_ITEM('',(#126640),#66137) ;
#2715=STYLED_ITEM('',(#126640),#66138) ;
#2716=STYLED_ITEM('',(#126640),#66139) ;
#2717=STYLED_ITEM('',(#126640),#66140) ;
#2718=STYLED_ITEM('',(#126640),#66141) ;
#2719=STYLED_ITEM('',(#126640),#66142) ;
#2720=STYLED_ITEM('',(#126640),#66143) ;
#2721=STYLED_ITEM('',(#126640),#66144) ;
#2722=STYLED_ITEM('',(#126640),#66145) ;
#2723=STYLED_ITEM('',(#126640),#66146) ;
#2724=STYLED_ITEM('',(#126640),#66147) ;
#2725=STYLED_ITEM('',(#126640),#66148) ;
#2726=STYLED_ITEM('',(#126640),#66149) ;
#2727=STYLED_ITEM('',(#126640),#66150) ;
#2728=STYLED_ITEM('',(#126640),#66151) ;
#2729=STYLED_ITEM('',(#126640),#66152) ;
#2730=STYLED_ITEM('',(#126640),#66153) ;
#2731=STYLED_ITEM('',(#126640),#66154) ;
#2732=STYLED_ITEM('',(#126640),#66155) ;
#2733=STYLED_ITEM('',(#126640),#66156) ;
#2734=STYLED_ITEM('',(#126640),#66157) ;
#2735=STYLED_ITEM('',(#126640),#66158) ;
#2736=STYLED_ITEM('',(#126640),#66159) ;
#2737=STYLED_ITEM('',(#126640),#66160) ;
#2738=STYLED_ITEM('',(#126640),#66161) ;
#2739=STYLED_ITEM('',(#126640),#66162) ;
#2740=STYLED_ITEM('',(#126640),#66163) ;
#2741=STYLED_ITEM('',(#126640),#66164) ;
#2742=STYLED_ITEM('',(#126640),#66165) ;
#2743=STYLED_ITEM('',(#126640),#66166) ;
#2744=STYLED_ITEM('',(#126640),#66167) ;
#2745=STYLED_ITEM('',(#126640),#66168) ;
#2746=STYLED_ITEM('',(#126640),#66169) ;
#2747=STYLED_ITEM('',(#126640),#66170) ;
#2748=STYLED_ITEM('',(#126640),#66171) ;
#2749=STYLED_ITEM('',(#126640),#66172) ;
#2750=STYLED_ITEM('',(#126640),#66173) ;
#2751=STYLED_ITEM('',(#126640),#66174) ;
#2752=STYLED_ITEM('',(#126640),#66175) ;
#2753=STYLED_ITEM('',(#126640),#66176) ;
#2754=STYLED_ITEM('',(#126640),#66177) ;
#2755=STYLED_ITEM('',(#126640),#66178) ;
#2756=STYLED_ITEM('',(#126640),#66179) ;
#2757=STYLED_ITEM('',(#126640),#66180) ;
#2758=STYLED_ITEM('',(#126640),#66181) ;
#2759=STYLED_ITEM('',(#126640),#66182) ;
#2760=STYLED_ITEM('',(#126640),#66183) ;
#2761=STYLED_ITEM('',(#126640),#66184) ;
#2762=STYLED_ITEM('',(#126640),#66185) ;
#2763=STYLED_ITEM('',(#126640),#66186) ;
#2764=STYLED_ITEM('',(#126640),#66187) ;
#2765=STYLED_ITEM('',(#126640),#66188) ;
#2766=STYLED_ITEM('',(#126640),#66189) ;
#2767=STYLED_ITEM('',(#126640),#66190) ;
#2768=STYLED_ITEM('',(#126640),#66191) ;
#2769=STYLED_ITEM('',(#126640),#66192) ;
#2770=STYLED_ITEM('',(#126640),#66193) ;
#2771=STYLED_ITEM('',(#126640),#66194) ;
#2772=STYLED_ITEM('',(#126640),#66195) ;
#2773=STYLED_ITEM('',(#126640),#66196) ;
#2774=STYLED_ITEM('',(#126640),#66197) ;
#2775=STYLED_ITEM('',(#126640),#66198) ;
#2776=STYLED_ITEM('',(#126640),#66199) ;
#2777=STYLED_ITEM('',(#126640),#66200) ;
#2778=STYLED_ITEM('',(#126640),#66201) ;
#2779=STYLED_ITEM('',(#126640),#66202) ;
#2780=STYLED_ITEM('',(#126640),#66203) ;
#2781=STYLED_ITEM('',(#126640),#66204) ;
#2782=STYLED_ITEM('',(#126640),#66205) ;
#2783=STYLED_ITEM('',(#126640),#66206) ;
#2784=STYLED_ITEM('',(#126640),#66207) ;
#2785=STYLED_ITEM('',(#126640),#66208) ;
#2786=STYLED_ITEM('',(#126640),#66209) ;
#2787=STYLED_ITEM('',(#126640),#66210) ;
#2788=STYLED_ITEM('',(#126640),#66211) ;
#2789=STYLED_ITEM('',(#126640),#66212) ;
#2790=STYLED_ITEM('',(#126640),#66213) ;
#2791=STYLED_ITEM('',(#126640),#66214) ;
#2792=STYLED_ITEM('',(#126640),#66215) ;
#2793=STYLED_ITEM('',(#126640),#66216) ;
#2794=STYLED_ITEM('',(#126640),#66217) ;
#2795=STYLED_ITEM('',(#126640),#66218) ;
#2796=STYLED_ITEM('',(#126640),#66219) ;
#2797=STYLED_ITEM('',(#126640),#66220) ;
#2798=STYLED_ITEM('',(#126640),#66221) ;
#2799=STYLED_ITEM('',(#126640),#66222) ;
#2800=STYLED_ITEM('',(#126640),#66223) ;
#2801=STYLED_ITEM('',(#126640),#66224) ;
#2802=STYLED_ITEM('',(#126640),#66225) ;
#2803=STYLED_ITEM('',(#126640),#66226) ;
#2804=STYLED_ITEM('',(#126640),#66227) ;
#2805=STYLED_ITEM('',(#126640),#66228) ;
#2806=STYLED_ITEM('',(#126640),#66229) ;
#2807=STYLED_ITEM('',(#126640),#66230) ;
#2808=STYLED_ITEM('',(#126640),#66231) ;
#2809=STYLED_ITEM('',(#126640),#66232) ;
#2810=STYLED_ITEM('',(#126640),#66233) ;
#2811=STYLED_ITEM('',(#126640),#66234) ;
#2812=STYLED_ITEM('',(#126640),#66235) ;
#2813=STYLED_ITEM('',(#126640),#66236) ;
#2814=STYLED_ITEM('',(#126640),#66237) ;
#2815=STYLED_ITEM('',(#126640),#66238) ;
#2816=STYLED_ITEM('',(#126640),#66239) ;
#2817=STYLED_ITEM('',(#126640),#66240) ;
#2818=STYLED_ITEM('',(#126640),#66241) ;
#2819=STYLED_ITEM('',(#126640),#66242) ;
#2820=STYLED_ITEM('',(#126640),#66243) ;
#2821=STYLED_ITEM('',(#126640),#66244) ;
#2822=STYLED_ITEM('',(#126640),#66245) ;
#2823=STYLED_ITEM('',(#126640),#66246) ;
#2824=STYLED_ITEM('',(#126640),#66247) ;
#2825=STYLED_ITEM('',(#126640),#66248) ;
#2826=STYLED_ITEM('',(#126640),#66249) ;
#2827=STYLED_ITEM('',(#126640),#66250) ;
#2828=STYLED_ITEM('',(#126640),#66251) ;
#2829=STYLED_ITEM('',(#126640),#66252) ;
#2830=STYLED_ITEM('',(#126640),#66253) ;
#2831=STYLED_ITEM('',(#126640),#66254) ;
#2832=STYLED_ITEM('',(#126640),#66255) ;
#2833=STYLED_ITEM('',(#126640),#66256) ;
#2834=STYLED_ITEM('',(#126640),#66257) ;
#2835=STYLED_ITEM('',(#126640),#66258) ;
#2836=STYLED_ITEM('',(#126640),#66259) ;
#2837=STYLED_ITEM('',(#126640),#66260) ;
#2838=STYLED_ITEM('',(#126640),#66261) ;
#2839=STYLED_ITEM('',(#126640),#66262) ;
#2840=STYLED_ITEM('',(#126640),#66263) ;
#2841=STYLED_ITEM('',(#126640),#66264) ;
#2842=STYLED_ITEM('',(#126640),#66265) ;
#2843=STYLED_ITEM('',(#126640),#66266) ;
#2844=STYLED_ITEM('',(#126640),#66267) ;
#2845=STYLED_ITEM('',(#126640),#66268) ;
#2846=STYLED_ITEM('',(#126640),#66269) ;
#2847=STYLED_ITEM('',(#126640),#66270) ;
#2848=STYLED_ITEM('',(#126640),#66271) ;
#2849=STYLED_ITEM('',(#126640),#66272) ;
#2850=STYLED_ITEM('',(#126640),#66273) ;
#2851=STYLED_ITEM('',(#126640),#66274) ;
#2852=STYLED_ITEM('',(#126640),#66275) ;
#2853=STYLED_ITEM('',(#126640),#66276) ;
#2854=STYLED_ITEM('',(#126640),#66277) ;
#2855=STYLED_ITEM('',(#126640),#66278) ;
#2856=STYLED_ITEM('',(#126640),#66279) ;
#2857=STYLED_ITEM('',(#126640),#66280) ;
#2858=STYLED_ITEM('',(#126640),#66281) ;
#2859=STYLED_ITEM('',(#126640),#66282) ;
#2860=STYLED_ITEM('',(#126640),#66283) ;
#2861=STYLED_ITEM('',(#126640),#66284) ;
#2862=STYLED_ITEM('',(#126640),#66285) ;
#2863=STYLED_ITEM('',(#126640),#66286) ;
#2864=STYLED_ITEM('',(#126640),#66287) ;
#2865=STYLED_ITEM('',(#126640),#66288) ;
#2866=STYLED_ITEM('',(#126640),#66289) ;
#2867=STYLED_ITEM('',(#126640),#66290) ;
#2868=STYLED_ITEM('',(#126640),#66291) ;
#2869=STYLED_ITEM('',(#126640),#66292) ;
#2870=STYLED_ITEM('',(#126640),#66293) ;
#2871=STYLED_ITEM('',(#126640),#66294) ;
#2872=STYLED_ITEM('',(#126640),#66295) ;
#2873=STYLED_ITEM('',(#126640),#66296) ;
#2874=STYLED_ITEM('',(#126640),#66297) ;
#2875=STYLED_ITEM('',(#126640),#66298) ;
#2876=STYLED_ITEM('',(#126640),#66299) ;
#2877=STYLED_ITEM('',(#126640),#66300) ;
#2878=STYLED_ITEM('',(#126640),#66301) ;
#2879=STYLED_ITEM('',(#126640),#66302) ;
#2880=STYLED_ITEM('',(#126640),#66303) ;
#2881=STYLED_ITEM('',(#126640),#66304) ;
#2882=STYLED_ITEM('',(#126640),#66305) ;
#2883=STYLED_ITEM('',(#126640),#66306) ;
#2884=STYLED_ITEM('',(#126640),#66307) ;
#2885=STYLED_ITEM('',(#126640),#66308) ;
#2886=STYLED_ITEM('',(#126640),#66309) ;
#2887=STYLED_ITEM('',(#126640),#66310) ;
#2888=STYLED_ITEM('',(#126640),#66311) ;
#2889=STYLED_ITEM('',(#126640),#66312) ;
#2890=STYLED_ITEM('',(#126640),#66313) ;
#2891=STYLED_ITEM('',(#126640),#66314) ;
#2892=STYLED_ITEM('',(#126640),#66315) ;
#2893=STYLED_ITEM('',(#126640),#66316) ;
#2894=STYLED_ITEM('',(#126640),#66317) ;
#2895=STYLED_ITEM('',(#126640),#66318) ;
#2896=STYLED_ITEM('',(#126640),#66319) ;
#2897=STYLED_ITEM('',(#126640),#66320) ;
#2898=STYLED_ITEM('',(#126640),#66321) ;
#2899=STYLED_ITEM('',(#126640),#66322) ;
#2900=STYLED_ITEM('',(#126640),#66323) ;
#2901=STYLED_ITEM('',(#126640),#66324) ;
#2902=STYLED_ITEM('',(#126640),#66325) ;
#2903=STYLED_ITEM('',(#126640),#66326) ;
#2904=STYLED_ITEM('',(#126640),#66327) ;
#2905=STYLED_ITEM('',(#126640),#66328) ;
#2906=STYLED_ITEM('',(#126640),#66329) ;
#2907=STYLED_ITEM('',(#126640),#66330) ;
#2908=STYLED_ITEM('',(#126640),#66331) ;
#2909=STYLED_ITEM('',(#126640),#66332) ;
#2910=STYLED_ITEM('',(#126640),#66333) ;
#2911=STYLED_ITEM('',(#126640),#66334) ;
#2912=STYLED_ITEM('',(#126640),#66335) ;
#2913=STYLED_ITEM('',(#126640),#66336) ;
#2914=STYLED_ITEM('',(#126640),#66337) ;
#2915=STYLED_ITEM('',(#126640),#66338) ;
#2916=STYLED_ITEM('',(#126640),#66339) ;
#2917=STYLED_ITEM('',(#126640),#66340) ;
#2918=STYLED_ITEM('',(#126640),#66341) ;
#2919=STYLED_ITEM('',(#126640),#66342) ;
#2920=STYLED_ITEM('',(#126640),#66343) ;
#2921=STYLED_ITEM('',(#126640),#66344) ;
#2922=STYLED_ITEM('',(#126640),#66345) ;
#2923=STYLED_ITEM('',(#126640),#66346) ;
#2924=STYLED_ITEM('',(#126640),#66347) ;
#2925=STYLED_ITEM('',(#126640),#66348) ;
#2926=STYLED_ITEM('',(#126640),#66349) ;
#2927=STYLED_ITEM('',(#126640),#66350) ;
#2928=STYLED_ITEM('',(#126640),#66351) ;
#2929=STYLED_ITEM('',(#126640),#66352) ;
#2930=STYLED_ITEM('',(#126640),#66353) ;
#2931=STYLED_ITEM('',(#126640),#66354) ;
#2932=STYLED_ITEM('',(#126640),#66355) ;
#2933=STYLED_ITEM('',(#126640),#66356) ;
#2934=STYLED_ITEM('',(#126640),#66357) ;
#2935=STYLED_ITEM('',(#126640),#66358) ;
#2936=STYLED_ITEM('',(#126640),#66359) ;
#2937=STYLED_ITEM('',(#126640),#66360) ;
#2938=STYLED_ITEM('',(#126640),#66361) ;
#2939=STYLED_ITEM('',(#126640),#66362) ;
#2940=STYLED_ITEM('',(#126640),#66363) ;
#2941=STYLED_ITEM('',(#126640),#66364) ;
#2942=STYLED_ITEM('',(#126640),#66365) ;
#2943=STYLED_ITEM('',(#126640),#66366) ;
#2944=STYLED_ITEM('',(#126640),#66367) ;
#2945=STYLED_ITEM('',(#126640),#66368) ;
#2946=STYLED_ITEM('',(#126640),#66369) ;
#2947=STYLED_ITEM('',(#126640),#66370) ;
#2948=STYLED_ITEM('',(#126640),#66371) ;
#2949=STYLED_ITEM('',(#126640),#66372) ;
#2950=STYLED_ITEM('',(#126640),#66373) ;
#2951=STYLED_ITEM('',(#126640),#66374) ;
#2952=STYLED_ITEM('',(#126640),#66375) ;
#2953=STYLED_ITEM('',(#126640),#66376) ;
#2954=STYLED_ITEM('',(#126640),#66377) ;
#2955=STYLED_ITEM('',(#126640),#66378) ;
#2956=STYLED_ITEM('',(#126640),#66379) ;
#2957=STYLED_ITEM('',(#126640),#66380) ;
#2958=STYLED_ITEM('',(#126640),#66381) ;
#2959=STYLED_ITEM('',(#126640),#66382) ;
#2960=STYLED_ITEM('',(#126640),#66383) ;
#2961=STYLED_ITEM('',(#126640),#66384) ;
#2962=STYLED_ITEM('',(#126640),#66385) ;
#2963=STYLED_ITEM('',(#126640),#66386) ;
#2964=STYLED_ITEM('',(#126640),#66387) ;
#2965=STYLED_ITEM('',(#126640),#66388) ;
#2966=STYLED_ITEM('',(#126640),#66389) ;
#2967=STYLED_ITEM('',(#126640),#66390) ;
#2968=STYLED_ITEM('',(#126640),#66391) ;
#2969=STYLED_ITEM('',(#126640),#66392) ;
#2970=STYLED_ITEM('',(#126640),#66393) ;
#2971=STYLED_ITEM('',(#126640),#66394) ;
#2972=STYLED_ITEM('',(#126640),#66395) ;
#2973=STYLED_ITEM('',(#126640),#66396) ;
#2974=STYLED_ITEM('',(#126640),#66397) ;
#2975=STYLED_ITEM('',(#126640),#66398) ;
#2976=STYLED_ITEM('',(#126640),#66399) ;
#2977=STYLED_ITEM('',(#126640),#66400) ;
#2978=STYLED_ITEM('',(#126640),#66401) ;
#2979=STYLED_ITEM('',(#126640),#66402) ;
#2980=STYLED_ITEM('',(#126640),#66403) ;
#2981=STYLED_ITEM('',(#126640),#66404) ;
#2982=STYLED_ITEM('',(#126640),#66405) ;
#2983=STYLED_ITEM('',(#126640),#66406) ;
#2984=STYLED_ITEM('',(#126640),#66407) ;
#2985=STYLED_ITEM('',(#126640),#66408) ;
#2986=STYLED_ITEM('',(#126640),#66409) ;
#2987=STYLED_ITEM('',(#126640),#66410) ;
#2988=STYLED_ITEM('',(#126640),#66411) ;
#2989=STYLED_ITEM('',(#126640),#66412) ;
#2990=STYLED_ITEM('',(#126640),#66413) ;
#2991=STYLED_ITEM('',(#126640),#66414) ;
#2992=STYLED_ITEM('',(#126640),#66415) ;
#2993=STYLED_ITEM('',(#126640),#66416) ;
#2994=STYLED_ITEM('',(#126640),#66417) ;
#2995=STYLED_ITEM('',(#126640),#66418) ;
#2996=STYLED_ITEM('',(#126640),#66419) ;
#2997=STYLED_ITEM('',(#126640),#66420) ;
#2998=STYLED_ITEM('',(#126640),#66421) ;
#2999=STYLED_ITEM('',(#126640),#66422) ;
#3000=STYLED_ITEM('',(#126640),#66423) ;
#3001=STYLED_ITEM('',(#126640),#66424) ;
#3002=STYLED_ITEM('',(#126640),#66425) ;
#3003=STYLED_ITEM('',(#126640),#66426) ;
#3004=STYLED_ITEM('',(#126640),#66427) ;
#3005=STYLED_ITEM('',(#126640),#66428) ;
#3006=STYLED_ITEM('',(#126640),#66429) ;
#3007=STYLED_ITEM('',(#126640),#66430) ;
#3008=STYLED_ITEM('',(#126640),#66431) ;
#3009=STYLED_ITEM('',(#126640),#66432) ;
#3010=STYLED_ITEM('',(#126640),#66433) ;
#3011=STYLED_ITEM('',(#126640),#66434) ;
#3012=STYLED_ITEM('',(#126640),#66435) ;
#3013=STYLED_ITEM('',(#126640),#66436) ;
#3014=STYLED_ITEM('',(#126640),#66437) ;
#3015=STYLED_ITEM('',(#126640),#66438) ;
#3016=STYLED_ITEM('',(#126640),#66439) ;
#3017=STYLED_ITEM('',(#126640),#66440) ;
#3018=STYLED_ITEM('',(#126640),#66441) ;
#3019=STYLED_ITEM('',(#126640),#66442) ;
#3020=STYLED_ITEM('',(#126640),#66443) ;
#3021=STYLED_ITEM('',(#126640),#66444) ;
#3022=STYLED_ITEM('',(#126640),#66445) ;
#3023=STYLED_ITEM('',(#126640),#66446) ;
#3024=STYLED_ITEM('',(#126640),#66447) ;
#3025=STYLED_ITEM('',(#126640),#66448) ;
#3026=STYLED_ITEM('',(#126640),#66449) ;
#3027=STYLED_ITEM('',(#126640),#66450) ;
#3028=STYLED_ITEM('',(#126640),#66451) ;
#3029=STYLED_ITEM('',(#126640),#66452) ;
#3030=STYLED_ITEM('',(#126640),#66453) ;
#3031=STYLED_ITEM('',(#126640),#66454) ;
#3032=STYLED_ITEM('',(#126640),#66455) ;
#3033=STYLED_ITEM('',(#126640),#66456) ;
#3034=STYLED_ITEM('',(#126640),#66457) ;
#3035=STYLED_ITEM('',(#126640),#66458) ;
#3036=STYLED_ITEM('',(#126640),#66459) ;
#3037=STYLED_ITEM('',(#126640),#66460) ;
#3038=STYLED_ITEM('',(#126640),#66461) ;
#3039=STYLED_ITEM('',(#126640),#66462) ;
#3040=STYLED_ITEM('',(#126640),#66463) ;
#3041=STYLED_ITEM('',(#126640),#66464) ;
#3042=STYLED_ITEM('',(#126640),#66465) ;
#3043=STYLED_ITEM('',(#126640),#66466) ;
#3044=STYLED_ITEM('',(#126640),#66467) ;
#3045=STYLED_ITEM('',(#126640),#66468) ;
#3046=STYLED_ITEM('',(#126640),#66469) ;
#3047=STYLED_ITEM('',(#126640),#66470) ;
#3048=STYLED_ITEM('',(#126640),#66471) ;
#3049=STYLED_ITEM('',(#126640),#66472) ;
#3050=STYLED_ITEM('',(#126640),#66473) ;
#3051=STYLED_ITEM('',(#126640),#66474) ;
#3052=STYLED_ITEM('',(#126640),#66475) ;
#3053=STYLED_ITEM('',(#126640),#66476) ;
#3054=STYLED_ITEM('',(#126640),#66477) ;
#3055=STYLED_ITEM('',(#126640),#66478) ;
#3056=STYLED_ITEM('',(#126640),#66479) ;
#3057=STYLED_ITEM('',(#126640),#66480) ;
#3058=STYLED_ITEM('',(#126640),#66481) ;
#3059=STYLED_ITEM('',(#126640),#66482) ;
#3060=STYLED_ITEM('',(#126640),#66483) ;
#3061=STYLED_ITEM('',(#126640),#66484) ;
#3062=STYLED_ITEM('',(#126640),#66485) ;
#3063=STYLED_ITEM('',(#126640),#66486) ;
#3064=STYLED_ITEM('',(#126640),#66487) ;
#3065=STYLED_ITEM('',(#126640),#66488) ;
#3066=STYLED_ITEM('',(#126640),#66489) ;
#3067=STYLED_ITEM('',(#126640),#66490) ;
#3068=STYLED_ITEM('',(#126640),#66491) ;
#3069=STYLED_ITEM('',(#126640),#66492) ;
#3070=STYLED_ITEM('',(#126640),#66493) ;
#3071=STYLED_ITEM('',(#126640),#66494) ;
#3072=STYLED_ITEM('',(#126640),#66495) ;
#3073=STYLED_ITEM('',(#126640),#66496) ;
#3074=STYLED_ITEM('',(#126640),#66497) ;
#3075=STYLED_ITEM('',(#126640),#66498) ;
#3076=STYLED_ITEM('',(#126640),#66499) ;
#3077=STYLED_ITEM('',(#126640),#66500) ;
#3078=STYLED_ITEM('',(#126640),#66501) ;
#3079=STYLED_ITEM('',(#126640),#66502) ;
#3080=STYLED_ITEM('',(#126640),#66503) ;
#3081=STYLED_ITEM('',(#126640),#66504) ;
#3082=STYLED_ITEM('',(#126640),#66505) ;
#3083=STYLED_ITEM('',(#126640),#66506) ;
#3084=STYLED_ITEM('',(#126640),#66507) ;
#3085=STYLED_ITEM('',(#126640),#66508) ;
#3086=STYLED_ITEM('',(#126640),#66509) ;
#3087=STYLED_ITEM('',(#126640),#66510) ;
#3088=STYLED_ITEM('',(#126640),#66511) ;
#3089=STYLED_ITEM('',(#126640),#66512) ;
#3090=STYLED_ITEM('',(#126640),#66513) ;
#3091=STYLED_ITEM('',(#126640),#66514) ;
#3092=STYLED_ITEM('',(#126640),#66515) ;
#3093=STYLED_ITEM('',(#126640),#66516) ;
#3094=STYLED_ITEM('',(#126640),#66517) ;
#3095=STYLED_ITEM('',(#126640),#66518) ;
#3096=STYLED_ITEM('',(#126640),#66519) ;
#3097=STYLED_ITEM('',(#126640),#66520) ;
#3098=STYLED_ITEM('',(#126640),#66521) ;
#3099=STYLED_ITEM('',(#126640),#66522) ;
#3100=STYLED_ITEM('',(#126640),#66523) ;
#3101=STYLED_ITEM('',(#126640),#66524) ;
#3102=STYLED_ITEM('',(#126640),#66525) ;
#3103=STYLED_ITEM('',(#126640),#66526) ;
#3104=STYLED_ITEM('',(#126640),#66527) ;
#3105=STYLED_ITEM('',(#126640),#66528) ;
#3106=STYLED_ITEM('',(#126640),#66529) ;
#3107=STYLED_ITEM('',(#126640),#66530) ;
#3108=STYLED_ITEM('',(#126640),#66531) ;
#3109=STYLED_ITEM('',(#126640),#66532) ;
#3110=STYLED_ITEM('',(#126640),#66533) ;
#3111=STYLED_ITEM('',(#126640),#66534) ;
#3112=STYLED_ITEM('',(#126640),#66535) ;
#3113=STYLED_ITEM('',(#126640),#66536) ;
#3114=STYLED_ITEM('',(#126640),#66537) ;
#3115=STYLED_ITEM('',(#126640),#66538) ;
#3116=STYLED_ITEM('',(#126640),#66539) ;
#3117=STYLED_ITEM('',(#126640),#66540) ;
#3118=STYLED_ITEM('',(#126640),#66541) ;
#3119=STYLED_ITEM('',(#126640),#66542) ;
#3120=STYLED_ITEM('',(#126640),#66543) ;
#3121=STYLED_ITEM('',(#126640),#66544) ;
#3122=STYLED_ITEM('',(#126640),#66545) ;
#3123=STYLED_ITEM('',(#126640),#66546) ;
#3124=STYLED_ITEM('',(#126640),#66547) ;
#3125=STYLED_ITEM('',(#126640),#66548) ;
#3126=STYLED_ITEM('',(#126640),#66549) ;
#3127=STYLED_ITEM('',(#126640),#66550) ;
#3128=STYLED_ITEM('',(#126640),#66551) ;
#3129=STYLED_ITEM('',(#126640),#66552) ;
#3130=STYLED_ITEM('',(#126640),#66553) ;
#3131=STYLED_ITEM('',(#126640),#66554) ;
#3132=STYLED_ITEM('',(#126640),#66555) ;
#3133=STYLED_ITEM('',(#126640),#66556) ;
#3134=STYLED_ITEM('',(#126640),#66557) ;
#3135=STYLED_ITEM('',(#126640),#66558) ;
#3136=STYLED_ITEM('',(#126640),#66559) ;
#3137=STYLED_ITEM('',(#126640),#66560) ;
#3138=STYLED_ITEM('',(#126640),#66561) ;
#3139=STYLED_ITEM('',(#126640),#66562) ;
#3140=STYLED_ITEM('',(#126640),#66563) ;
#3141=STYLED_ITEM('',(#126640),#66564) ;
#3142=STYLED_ITEM('',(#126640),#66565) ;
#3143=STYLED_ITEM('',(#126640),#66566) ;
#3144=STYLED_ITEM('',(#126640),#66567) ;
#3145=STYLED_ITEM('',(#126640),#66568) ;
#3146=STYLED_ITEM('',(#126640),#66569) ;
#3147=STYLED_ITEM('',(#126640),#66570) ;
#3148=STYLED_ITEM('',(#126640),#66571) ;
#3149=STYLED_ITEM('',(#126640),#66572) ;
#3150=STYLED_ITEM('',(#126640),#66573) ;
#3151=STYLED_ITEM('',(#126640),#66574) ;
#3152=STYLED_ITEM('',(#126640),#66575) ;
#3153=STYLED_ITEM('',(#126640),#66576) ;
#3154=STYLED_ITEM('',(#126640),#66577) ;
#3155=STYLED_ITEM('',(#126640),#66578) ;
#3156=STYLED_ITEM('',(#126640),#66579) ;
#3157=STYLED_ITEM('',(#126640),#66580) ;
#3158=STYLED_ITEM('',(#126640),#66581) ;
#3159=STYLED_ITEM('',(#126640),#66582) ;
#3160=STYLED_ITEM('',(#126640),#66583) ;
#3161=STYLED_ITEM('',(#126640),#66584) ;
#3162=STYLED_ITEM('',(#126640),#66585) ;
#3163=STYLED_ITEM('',(#126640),#66586) ;
#3164=STYLED_ITEM('',(#126640),#66587) ;
#3165=STYLED_ITEM('',(#126640),#66588) ;
#3166=STYLED_ITEM('',(#126640),#66589) ;
#3167=STYLED_ITEM('',(#126640),#66590) ;
#3168=STYLED_ITEM('',(#126640),#66591) ;
#3169=STYLED_ITEM('',(#126640),#66592) ;
#3170=STYLED_ITEM('',(#126640),#66593) ;
#3171=STYLED_ITEM('',(#126640),#66594) ;
#3172=STYLED_ITEM('',(#126640),#66595) ;
#3173=STYLED_ITEM('',(#126640),#66596) ;
#3174=STYLED_ITEM('',(#126640),#66597) ;
#3175=STYLED_ITEM('',(#126640),#66598) ;
#3176=STYLED_ITEM('',(#126640),#66599) ;
#3177=STYLED_ITEM('',(#126640),#66600) ;
#3178=STYLED_ITEM('',(#126640),#66601) ;
#3179=STYLED_ITEM('',(#126640),#66602) ;
#3180=STYLED_ITEM('',(#126640),#66603) ;
#3181=STYLED_ITEM('',(#126640),#66604) ;
#3182=STYLED_ITEM('',(#126640),#66605) ;
#3183=STYLED_ITEM('',(#126640),#66606) ;
#3184=STYLED_ITEM('',(#126640),#66607) ;
#3185=STYLED_ITEM('',(#126640),#66608) ;
#3186=STYLED_ITEM('',(#126640),#66609) ;
#3187=STYLED_ITEM('',(#126640),#66610) ;
#3188=STYLED_ITEM('',(#126640),#66611) ;
#3189=STYLED_ITEM('',(#126640),#66612) ;
#3190=STYLED_ITEM('',(#126640),#66613) ;
#3191=STYLED_ITEM('',(#126640),#66614) ;
#3192=STYLED_ITEM('',(#126640),#66615) ;
#3193=STYLED_ITEM('',(#126640),#66616) ;
#3194=STYLED_ITEM('',(#126640),#66617) ;
#3195=STYLED_ITEM('',(#126640),#66618) ;
#3196=STYLED_ITEM('',(#126640),#66619) ;
#3197=STYLED_ITEM('',(#126640),#66620) ;
#3198=STYLED_ITEM('',(#126640),#66621) ;
#3199=STYLED_ITEM('',(#126640),#66622) ;
#3200=STYLED_ITEM('',(#126640),#66623) ;
#3201=STYLED_ITEM('',(#126640),#66624) ;
#3202=STYLED_ITEM('',(#126640),#66625) ;
#3203=STYLED_ITEM('',(#126640),#66626) ;
#3204=STYLED_ITEM('',(#126640),#66627) ;
#3205=STYLED_ITEM('',(#126640),#66628) ;
#3206=STYLED_ITEM('',(#126640),#66629) ;
#3207=STYLED_ITEM('',(#126640),#66630) ;
#3208=STYLED_ITEM('',(#126640),#66631) ;
#3209=STYLED_ITEM('',(#126640),#66632) ;
#3210=STYLED_ITEM('',(#126640),#66633) ;
#3211=STYLED_ITEM('',(#126640),#66634) ;
#3212=STYLED_ITEM('',(#126640),#66635) ;
#3213=STYLED_ITEM('',(#126640),#66636) ;
#3214=STYLED_ITEM('',(#126640),#66637) ;
#3215=STYLED_ITEM('',(#126640),#66638) ;
#3216=STYLED_ITEM('',(#126640),#66639) ;
#3217=STYLED_ITEM('',(#126640),#66640) ;
#3218=STYLED_ITEM('',(#126640),#66641) ;
#3219=STYLED_ITEM('',(#126640),#66642) ;
#3220=STYLED_ITEM('',(#126640),#66643) ;
#3221=STYLED_ITEM('',(#126640),#66644) ;
#3222=STYLED_ITEM('',(#126640),#66645) ;
#3223=STYLED_ITEM('',(#126640),#66646) ;
#3224=STYLED_ITEM('',(#126640),#66647) ;
#3225=STYLED_ITEM('',(#126640),#66648) ;
#3226=STYLED_ITEM('',(#126640),#66649) ;
#3227=STYLED_ITEM('',(#126640),#66650) ;
#3228=STYLED_ITEM('',(#126640),#66651) ;
#3229=STYLED_ITEM('',(#126640),#66652) ;
#3230=STYLED_ITEM('',(#126640),#66653) ;
#3231=STYLED_ITEM('',(#126640),#66654) ;
#3232=STYLED_ITEM('',(#126640),#66655) ;
#3233=STYLED_ITEM('',(#126640),#66656) ;
#3234=STYLED_ITEM('',(#126640),#66657) ;
#3235=STYLED_ITEM('',(#126640),#66658) ;
#3236=STYLED_ITEM('',(#126640),#66659) ;
#3237=STYLED_ITEM('',(#126640),#66660) ;
#3238=STYLED_ITEM('',(#126640),#66661) ;
#3239=STYLED_ITEM('',(#126640),#66662) ;
#3240=STYLED_ITEM('',(#126640),#66663) ;
#3241=STYLED_ITEM('',(#126640),#66664) ;
#3242=STYLED_ITEM('',(#126640),#66665) ;
#3243=STYLED_ITEM('',(#126640),#66666) ;
#3244=STYLED_ITEM('',(#126640),#66667) ;
#3245=STYLED_ITEM('',(#126640),#66668) ;
#3246=STYLED_ITEM('',(#126640),#66669) ;
#3247=STYLED_ITEM('',(#126640),#66670) ;
#3248=STYLED_ITEM('',(#126640),#66671) ;
#3249=STYLED_ITEM('',(#126640),#66672) ;
#3250=STYLED_ITEM('',(#126640),#66673) ;
#3251=STYLED_ITEM('',(#126640),#66674) ;
#3252=STYLED_ITEM('',(#126640),#66675) ;
#3253=STYLED_ITEM('',(#126640),#66676) ;
#3254=STYLED_ITEM('',(#126640),#66677) ;
#3255=STYLED_ITEM('',(#126640),#66678) ;
#3256=STYLED_ITEM('',(#126640),#66679) ;
#3257=STYLED_ITEM('',(#126640),#66680) ;
#3258=STYLED_ITEM('',(#126640),#66681) ;
#3259=STYLED_ITEM('',(#126640),#66682) ;
#3260=STYLED_ITEM('',(#126640),#66683) ;
#3261=STYLED_ITEM('',(#126640),#66684) ;
#3262=STYLED_ITEM('',(#126640),#66685) ;
#3263=STYLED_ITEM('',(#126640),#66686) ;
#3264=STYLED_ITEM('',(#126640),#66687) ;
#3265=STYLED_ITEM('',(#126640),#66688) ;
#3266=STYLED_ITEM('',(#126640),#66689) ;
#3267=STYLED_ITEM('',(#126640),#66690) ;
#3268=STYLED_ITEM('',(#126640),#66691) ;
#3269=STYLED_ITEM('',(#126640),#66692) ;
#3270=STYLED_ITEM('',(#126640),#66693) ;
#3271=STYLED_ITEM('',(#126640),#66694) ;
#3272=STYLED_ITEM('',(#126640),#66695) ;
#3273=STYLED_ITEM('',(#126640),#66696) ;
#3274=STYLED_ITEM('',(#126640),#66697) ;
#3275=STYLED_ITEM('',(#126640),#66698) ;
#3276=STYLED_ITEM('',(#126640),#66699) ;
#3277=STYLED_ITEM('',(#126640),#66700) ;
#3278=STYLED_ITEM('',(#126640),#66701) ;
#3279=STYLED_ITEM('',(#126640),#66702) ;
#3280=STYLED_ITEM('',(#126640),#66703) ;
#3281=STYLED_ITEM('',(#126640),#66704) ;
#3282=STYLED_ITEM('',(#126640),#66705) ;
#3283=STYLED_ITEM('',(#126640),#66706) ;
#3284=STYLED_ITEM('',(#126640),#66707) ;
#3285=STYLED_ITEM('',(#126640),#66708) ;
#3286=STYLED_ITEM('',(#126640),#66709) ;
#3287=STYLED_ITEM('',(#126640),#66710) ;
#3288=STYLED_ITEM('',(#126640),#66711) ;
#3289=STYLED_ITEM('',(#126640),#66712) ;
#3290=STYLED_ITEM('',(#126640),#66713) ;
#3291=STYLED_ITEM('',(#126640),#66714) ;
#3292=STYLED_ITEM('',(#126640),#66715) ;
#3293=STYLED_ITEM('',(#126640),#66716) ;
#3294=STYLED_ITEM('',(#126640),#66717) ;
#3295=STYLED_ITEM('',(#126640),#66718) ;
#3296=STYLED_ITEM('',(#126640),#66719) ;
#3297=STYLED_ITEM('',(#126640),#66720) ;
#3298=STYLED_ITEM('',(#126640),#66721) ;
#3299=STYLED_ITEM('',(#126640),#66722) ;
#3300=STYLED_ITEM('',(#126640),#66723) ;
#3301=STYLED_ITEM('',(#126640),#66724) ;
#3302=STYLED_ITEM('',(#126640),#66725) ;
#3303=STYLED_ITEM('',(#126640),#66726) ;
#3304=STYLED_ITEM('',(#126640),#66727) ;
#3305=STYLED_ITEM('',(#126640),#66728) ;
#3306=STYLED_ITEM('',(#126640),#66729) ;
#3307=STYLED_ITEM('',(#126640),#66730) ;
#3308=STYLED_ITEM('',(#126640),#66731) ;
#3309=STYLED_ITEM('',(#126640),#66732) ;
#3310=STYLED_ITEM('',(#126640),#66733) ;
#3311=STYLED_ITEM('',(#126640),#66734) ;
#3312=STYLED_ITEM('',(#126640),#66735) ;
#3313=STYLED_ITEM('',(#126640),#66736) ;
#3314=STYLED_ITEM('',(#126640),#66737) ;
#3315=STYLED_ITEM('',(#126640),#66738) ;
#3316=STYLED_ITEM('',(#126640),#66739) ;
#3317=STYLED_ITEM('',(#126640),#66740) ;
#3318=STYLED_ITEM('',(#126640),#66741) ;
#3319=STYLED_ITEM('',(#126640),#66742) ;
#3320=STYLED_ITEM('',(#126640),#66743) ;
#3321=STYLED_ITEM('',(#126640),#66744) ;
#3322=STYLED_ITEM('',(#126640),#66745) ;
#3323=STYLED_ITEM('',(#126640),#66746) ;
#3324=STYLED_ITEM('',(#126640),#66747) ;
#3325=STYLED_ITEM('',(#126640),#66748) ;
#3326=STYLED_ITEM('',(#126640),#66749) ;
#3327=STYLED_ITEM('',(#126640),#66750) ;
#3328=STYLED_ITEM('',(#126640),#66751) ;
#3329=STYLED_ITEM('',(#126640),#66752) ;
#3330=STYLED_ITEM('',(#126640),#66753) ;
#3331=STYLED_ITEM('',(#126640),#66754) ;
#3332=STYLED_ITEM('',(#126640),#66755) ;
#3333=STYLED_ITEM('',(#126640),#66756) ;
#3334=STYLED_ITEM('',(#126640),#66757) ;
#3335=STYLED_ITEM('',(#126640),#66758) ;
#3336=STYLED_ITEM('',(#126640),#66759) ;
#3337=STYLED_ITEM('',(#126640),#66760) ;
#3338=STYLED_ITEM('',(#126640),#66761) ;
#3339=STYLED_ITEM('',(#126640),#66762) ;
#3340=STYLED_ITEM('',(#126640),#66763) ;
#3341=STYLED_ITEM('',(#126640),#66764) ;
#3342=STYLED_ITEM('',(#126640),#66765) ;
#3343=STYLED_ITEM('',(#126640),#66766) ;
#3344=STYLED_ITEM('',(#126640),#66767) ;
#3345=STYLED_ITEM('',(#126640),#66768) ;
#3346=STYLED_ITEM('',(#126640),#66769) ;
#3347=STYLED_ITEM('',(#126640),#66770) ;
#3348=STYLED_ITEM('',(#126640),#66771) ;
#3349=STYLED_ITEM('',(#126640),#66772) ;
#3350=STYLED_ITEM('',(#126640),#66773) ;
#3351=STYLED_ITEM('',(#126640),#66774) ;
#3352=STYLED_ITEM('',(#126640),#66775) ;
#3353=STYLED_ITEM('',(#126640),#66776) ;
#3354=STYLED_ITEM('',(#126640),#66777) ;
#3355=STYLED_ITEM('',(#126640),#66778) ;
#3356=STYLED_ITEM('',(#126640),#66779) ;
#3357=STYLED_ITEM('',(#126640),#66780) ;
#3358=STYLED_ITEM('',(#126640),#66781) ;
#3359=STYLED_ITEM('',(#126640),#66782) ;
#3360=STYLED_ITEM('',(#126640),#66783) ;
#3361=STYLED_ITEM('',(#126640),#66784) ;
#3362=STYLED_ITEM('',(#126640),#66785) ;
#3363=STYLED_ITEM('',(#126640),#66786) ;
#3364=STYLED_ITEM('',(#126640),#66787) ;
#3365=STYLED_ITEM('',(#126640),#66788) ;
#3366=STYLED_ITEM('',(#126640),#66789) ;
#3367=STYLED_ITEM('',(#126640),#66790) ;
#3368=STYLED_ITEM('',(#126640),#66791) ;
#3369=STYLED_ITEM('',(#126640),#66792) ;
#3370=STYLED_ITEM('',(#126640),#66793) ;
#3371=STYLED_ITEM('',(#126640),#66794) ;
#3372=STYLED_ITEM('',(#126640),#66795) ;
#3373=STYLED_ITEM('',(#126640),#66796) ;
#3374=STYLED_ITEM('',(#126640),#66797) ;
#3375=STYLED_ITEM('',(#126640),#66798) ;
#3376=STYLED_ITEM('',(#126640),#66799) ;
#3377=STYLED_ITEM('',(#126640),#66800) ;
#3378=STYLED_ITEM('',(#126640),#66801) ;
#3379=STYLED_ITEM('',(#126640),#66802) ;
#3380=STYLED_ITEM('',(#126640),#66803) ;
#3381=STYLED_ITEM('',(#126640),#66804) ;
#3382=STYLED_ITEM('',(#126640),#66805) ;
#3383=STYLED_ITEM('',(#126640),#66806) ;
#3384=STYLED_ITEM('',(#126640),#66807) ;
#3385=STYLED_ITEM('',(#126640),#66808) ;
#3386=STYLED_ITEM('',(#126640),#66809) ;
#3387=STYLED_ITEM('',(#126640),#66810) ;
#3388=STYLED_ITEM('',(#126640),#66811) ;
#3389=STYLED_ITEM('',(#126640),#66812) ;
#3390=STYLED_ITEM('',(#126640),#66813) ;
#3391=STYLED_ITEM('',(#126640),#66814) ;
#3392=STYLED_ITEM('',(#126640),#66815) ;
#3393=STYLED_ITEM('',(#126640),#66816) ;
#3394=STYLED_ITEM('',(#126640),#66817) ;
#3395=STYLED_ITEM('',(#126640),#66818) ;
#3396=STYLED_ITEM('',(#126640),#66819) ;
#3397=STYLED_ITEM('',(#126640),#66820) ;
#3398=STYLED_ITEM('',(#126640),#66821) ;
#3399=STYLED_ITEM('',(#126640),#66822) ;
#3400=STYLED_ITEM('',(#126640),#66823) ;
#3401=STYLED_ITEM('',(#126640),#66824) ;
#3402=STYLED_ITEM('',(#126640),#66825) ;
#3403=STYLED_ITEM('',(#126640),#66826) ;
#3404=STYLED_ITEM('',(#126640),#66827) ;
#3405=STYLED_ITEM('',(#126640),#66828) ;
#3406=STYLED_ITEM('',(#126640),#66829) ;
#3407=STYLED_ITEM('',(#126640),#66830) ;
#3408=STYLED_ITEM('',(#126640),#66831) ;
#3409=STYLED_ITEM('',(#126640),#66832) ;
#3410=STYLED_ITEM('',(#126640),#66833) ;
#3411=STYLED_ITEM('',(#126640),#66834) ;
#3412=STYLED_ITEM('',(#126640),#66835) ;
#3413=STYLED_ITEM('',(#126640),#66836) ;
#3414=STYLED_ITEM('',(#126640),#66837) ;
#3415=STYLED_ITEM('',(#126640),#66838) ;
#3416=STYLED_ITEM('',(#126640),#66839) ;
#3417=STYLED_ITEM('',(#126640),#66840) ;
#3418=STYLED_ITEM('',(#126640),#66841) ;
#3419=STYLED_ITEM('',(#126640),#66842) ;
#3420=STYLED_ITEM('',(#126640),#66843) ;
#3421=STYLED_ITEM('',(#126640),#66844) ;
#3422=STYLED_ITEM('',(#126640),#66845) ;
#3423=STYLED_ITEM('',(#126640),#66846) ;
#3424=STYLED_ITEM('',(#126640),#66847) ;
#3425=STYLED_ITEM('',(#126640),#66848) ;
#3426=STYLED_ITEM('',(#126640),#66849) ;
#3427=STYLED_ITEM('',(#126640),#66850) ;
#3428=STYLED_ITEM('',(#126640),#66851) ;
#3429=STYLED_ITEM('',(#126640),#66852) ;
#3430=STYLED_ITEM('',(#126640),#66853) ;
#3431=STYLED_ITEM('',(#126640),#66854) ;
#3432=STYLED_ITEM('',(#126640),#66855) ;
#3433=STYLED_ITEM('',(#126640),#66856) ;
#3434=STYLED_ITEM('',(#126640),#66857) ;
#3435=STYLED_ITEM('',(#126640),#66858) ;
#3436=STYLED_ITEM('',(#126640),#66859) ;
#3437=STYLED_ITEM('',(#126640),#66860) ;
#3438=STYLED_ITEM('',(#126640),#66861) ;
#3439=STYLED_ITEM('',(#126640),#66862) ;
#3440=STYLED_ITEM('',(#126640),#66863) ;
#3441=STYLED_ITEM('',(#126640),#66864) ;
#3442=STYLED_ITEM('',(#126640),#66865) ;
#3443=STYLED_ITEM('',(#126640),#66866) ;
#3444=STYLED_ITEM('',(#126640),#66867) ;
#3445=STYLED_ITEM('',(#126640),#66868) ;
#3446=STYLED_ITEM('',(#126640),#66869) ;
#3447=STYLED_ITEM('',(#126640),#66870) ;
#3448=STYLED_ITEM('',(#126640),#66871) ;
#3449=STYLED_ITEM('',(#126640),#66872) ;
#3450=STYLED_ITEM('',(#126640),#66873) ;
#3451=STYLED_ITEM('',(#126640),#66874) ;
#3452=STYLED_ITEM('',(#126640),#66875) ;
#3453=STYLED_ITEM('',(#126640),#66876) ;
#3454=STYLED_ITEM('',(#126640),#66877) ;
#3455=STYLED_ITEM('',(#126640),#66878) ;
#3456=STYLED_ITEM('',(#126640),#66879) ;
#3457=STYLED_ITEM('',(#126640),#66880) ;
#3458=STYLED_ITEM('',(#126640),#66881) ;
#3459=STYLED_ITEM('',(#126640),#66882) ;
#3460=STYLED_ITEM('',(#126640),#66883) ;
#3461=STYLED_ITEM('',(#126640),#66884) ;
#3462=STYLED_ITEM('',(#126640),#66885) ;
#3463=STYLED_ITEM('',(#126640),#66886) ;
#3464=STYLED_ITEM('',(#126640),#66887) ;
#3465=STYLED_ITEM('',(#126640),#66888) ;
#3466=STYLED_ITEM('',(#126640),#66889) ;
#3467=STYLED_ITEM('',(#126640),#66890) ;
#3468=STYLED_ITEM('',(#126640),#66891) ;
#3469=STYLED_ITEM('',(#126640),#66892) ;
#3470=STYLED_ITEM('',(#126640),#66893) ;
#3471=STYLED_ITEM('',(#126640),#66894) ;
#3472=STYLED_ITEM('',(#126640),#66895) ;
#3473=STYLED_ITEM('',(#126640),#66896) ;
#3474=STYLED_ITEM('',(#126640),#66897) ;
#3475=STYLED_ITEM('',(#126640),#66898) ;
#3476=STYLED_ITEM('',(#126640),#66899) ;
#3477=STYLED_ITEM('',(#126640),#66900) ;
#3478=STYLED_ITEM('',(#126640),#66901) ;
#3479=STYLED_ITEM('',(#126640),#66902) ;
#3480=STYLED_ITEM('',(#126640),#66903) ;
#3481=STYLED_ITEM('',(#126640),#66904) ;
#3482=STYLED_ITEM('',(#126640),#66905) ;
#3483=STYLED_ITEM('',(#126640),#66906) ;
#3484=STYLED_ITEM('',(#126640),#66907) ;
#3485=STYLED_ITEM('',(#126640),#66908) ;
#3486=STYLED_ITEM('',(#126640),#66909) ;
#3487=STYLED_ITEM('',(#126640),#66910) ;
#3488=STYLED_ITEM('',(#126640),#66911) ;
#3489=STYLED_ITEM('',(#126640),#66912) ;
#3490=STYLED_ITEM('',(#126640),#66913) ;
#3491=STYLED_ITEM('',(#126640),#66914) ;
#3492=STYLED_ITEM('',(#126640),#66915) ;
#3493=STYLED_ITEM('',(#126640),#66916) ;
#3494=STYLED_ITEM('',(#126640),#66917) ;
#3495=STYLED_ITEM('',(#126640),#66918) ;
#3496=STYLED_ITEM('',(#126640),#66919) ;
#3497=STYLED_ITEM('',(#126640),#66920) ;
#3498=STYLED_ITEM('',(#126640),#66921) ;
#3499=STYLED_ITEM('',(#126640),#66922) ;
#3500=STYLED_ITEM('',(#126640),#66923) ;
#3501=STYLED_ITEM('',(#126640),#66924) ;
#3502=STYLED_ITEM('',(#126640),#66925) ;
#3503=STYLED_ITEM('',(#126640),#66926) ;
#3504=STYLED_ITEM('',(#126640),#66927) ;
#3505=STYLED_ITEM('',(#126640),#66928) ;
#3506=STYLED_ITEM('',(#126640),#66929) ;
#3507=STYLED_ITEM('',(#126640),#66930) ;
#3508=STYLED_ITEM('',(#126640),#66931) ;
#3509=STYLED_ITEM('',(#126640),#66932) ;
#3510=STYLED_ITEM('',(#126640),#66933) ;
#3511=STYLED_ITEM('',(#126640),#66934) ;
#3512=STYLED_ITEM('',(#126640),#66935) ;
#3513=STYLED_ITEM('',(#126640),#66936) ;
#3514=STYLED_ITEM('',(#126640),#66937) ;
#3515=STYLED_ITEM('',(#126640),#66938) ;
#3516=STYLED_ITEM('',(#126640),#66939) ;
#3517=STYLED_ITEM('',(#126640),#66940) ;
#3518=STYLED_ITEM('',(#126640),#66941) ;
#3519=STYLED_ITEM('',(#126640),#66942) ;
#3520=STYLED_ITEM('',(#126640),#66943) ;
#3521=STYLED_ITEM('',(#126641),#66944) ;
#3522=STYLED_ITEM('',(#126641),#66945) ;
#3523=STYLED_ITEM('',(#126641),#66946) ;
#3524=STYLED_ITEM('',(#126641),#66947) ;
#3525=STYLED_ITEM('',(#126641),#66948) ;
#3526=STYLED_ITEM('',(#126641),#66949) ;
#3527=STYLED_ITEM('',(#126641),#66950) ;
#3528=STYLED_ITEM('',(#126641),#66951) ;
#3529=STYLED_ITEM('',(#126641),#66952) ;
#3530=STYLED_ITEM('',(#126641),#66953) ;
#3531=STYLED_ITEM('',(#126641),#66954) ;
#3532=STYLED_ITEM('',(#126641),#66955) ;
#3533=STYLED_ITEM('',(#126641),#66956) ;
#3534=STYLED_ITEM('',(#126641),#66957) ;
#3535=STYLED_ITEM('',(#126641),#66958) ;
#3536=STYLED_ITEM('',(#126641),#66959) ;
#3537=STYLED_ITEM('',(#126641),#66960) ;
#3538=STYLED_ITEM('',(#126641),#66961) ;
#3539=STYLED_ITEM('',(#126641),#66962) ;
#3540=STYLED_ITEM('',(#126641),#66963) ;
#3541=STYLED_ITEM('',(#126641),#66964) ;
#3542=STYLED_ITEM('',(#126641),#66965) ;
#3543=STYLED_ITEM('',(#126641),#66966) ;
#3544=STYLED_ITEM('',(#126641),#66967) ;
#3545=STYLED_ITEM('',(#126641),#66968) ;
#3546=STYLED_ITEM('',(#126641),#66969) ;
#3547=STYLED_ITEM('',(#126641),#66970) ;
#3548=STYLED_ITEM('',(#126641),#66971) ;
#3549=STYLED_ITEM('',(#126641),#66972) ;
#3550=STYLED_ITEM('',(#126641),#66973) ;
#3551=STYLED_ITEM('',(#126641),#66974) ;
#3552=STYLED_ITEM('',(#126641),#66975) ;
#3553=STYLED_ITEM('',(#126641),#66976) ;
#3554=STYLED_ITEM('',(#126641),#66977) ;
#3555=STYLED_ITEM('',(#126641),#66978) ;
#3556=STYLED_ITEM('',(#126641),#66979) ;
#3557=STYLED_ITEM('',(#126641),#66980) ;
#3558=STYLED_ITEM('',(#126641),#66981) ;
#3559=STYLED_ITEM('',(#126641),#66982) ;
#3560=STYLED_ITEM('',(#126641),#66983) ;
#3561=STYLED_ITEM('',(#126641),#66984) ;
#3562=STYLED_ITEM('',(#126641),#66985) ;
#3563=STYLED_ITEM('',(#126641),#66986) ;
#3564=STYLED_ITEM('',(#126641),#66987) ;
#3565=STYLED_ITEM('',(#126641),#66988) ;
#3566=STYLED_ITEM('',(#126641),#66989) ;
#3567=STYLED_ITEM('',(#126641),#66990) ;
#3568=STYLED_ITEM('',(#126641),#66991) ;
#3569=STYLED_ITEM('',(#126641),#66992) ;
#3570=STYLED_ITEM('',(#126641),#66993) ;
#3571=STYLED_ITEM('',(#126641),#66994) ;
#3572=STYLED_ITEM('',(#126641),#66995) ;
#3573=STYLED_ITEM('',(#126641),#66996) ;
#3574=STYLED_ITEM('',(#126641),#66997) ;
#3575=STYLED_ITEM('',(#126641),#66998) ;
#3576=STYLED_ITEM('',(#126641),#66999) ;
#3577=STYLED_ITEM('',(#126641),#67000) ;
#3578=STYLED_ITEM('',(#126641),#67001) ;
#3579=STYLED_ITEM('',(#126641),#67002) ;
#3580=STYLED_ITEM('',(#126641),#67003) ;
#3581=STYLED_ITEM('',(#126641),#67004) ;
#3582=STYLED_ITEM('',(#126641),#67005) ;
#3583=STYLED_ITEM('',(#126641),#67006) ;
#3584=STYLED_ITEM('',(#126641),#67007) ;
#3585=STYLED_ITEM('',(#126641),#67008) ;
#3586=STYLED_ITEM('',(#126641),#67009) ;
#3587=STYLED_ITEM('',(#126641),#67010) ;
#3588=STYLED_ITEM('',(#126641),#67011) ;
#3589=STYLED_ITEM('',(#126641),#67012) ;
#3590=STYLED_ITEM('',(#126641),#67013) ;
#3591=STYLED_ITEM('',(#126641),#67014) ;
#3592=STYLED_ITEM('',(#126641),#67015) ;
#3593=STYLED_ITEM('',(#126641),#67016) ;
#3594=STYLED_ITEM('',(#126641),#67017) ;
#3595=STYLED_ITEM('',(#126641),#67018) ;
#3596=STYLED_ITEM('',(#126641),#67019) ;
#3597=STYLED_ITEM('',(#126641),#67020) ;
#3598=STYLED_ITEM('',(#126641),#67021) ;
#3599=STYLED_ITEM('',(#126641),#67022) ;
#3600=STYLED_ITEM('',(#126641),#67023) ;
#3601=STYLED_ITEM('',(#126641),#67024) ;
#3602=STYLED_ITEM('',(#126641),#67025) ;
#3603=STYLED_ITEM('',(#126641),#67026) ;
#3604=STYLED_ITEM('',(#126641),#67027) ;
#3605=STYLED_ITEM('',(#126641),#67028) ;
#3606=STYLED_ITEM('',(#126641),#67029) ;
#3607=STYLED_ITEM('',(#126641),#67030) ;
#3608=STYLED_ITEM('',(#126641),#67031) ;
#3609=STYLED_ITEM('',(#126641),#67032) ;
#3610=STYLED_ITEM('',(#126641),#67033) ;
#3611=STYLED_ITEM('',(#126641),#67034) ;
#3612=STYLED_ITEM('',(#126641),#67035) ;
#3613=STYLED_ITEM('',(#126641),#67036) ;
#3614=STYLED_ITEM('',(#126641),#67037) ;
#3615=STYLED_ITEM('',(#126641),#67038) ;
#3616=STYLED_ITEM('',(#126641),#67039) ;
#3617=STYLED_ITEM('',(#126641),#67040) ;
#3618=STYLED_ITEM('',(#126641),#67041) ;
#3619=STYLED_ITEM('',(#126641),#67042) ;
#3620=STYLED_ITEM('',(#126641),#67043) ;
#3621=STYLED_ITEM('',(#126641),#67044) ;
#3622=STYLED_ITEM('',(#126641),#67045) ;
#3623=STYLED_ITEM('',(#126641),#67046) ;
#3624=STYLED_ITEM('',(#126641),#67047) ;
#3625=STYLED_ITEM('',(#126641),#67048) ;
#3626=STYLED_ITEM('',(#126641),#67049) ;
#3627=STYLED_ITEM('',(#126641),#67050) ;
#3628=STYLED_ITEM('',(#126641),#67051) ;
#3629=STYLED_ITEM('',(#126641),#67052) ;
#3630=STYLED_ITEM('',(#126641),#67053) ;
#3631=STYLED_ITEM('',(#126641),#67054) ;
#3632=STYLED_ITEM('',(#126641),#67055) ;
#3633=STYLED_ITEM('',(#126641),#67056) ;
#3634=STYLED_ITEM('',(#126641),#67057) ;
#3635=STYLED_ITEM('',(#126641),#67058) ;
#3636=STYLED_ITEM('',(#126641),#67059) ;
#3637=STYLED_ITEM('',(#126641),#67060) ;
#3638=STYLED_ITEM('',(#126641),#67061) ;
#3639=STYLED_ITEM('',(#126641),#67062) ;
#3640=STYLED_ITEM('',(#126641),#67063) ;
#3641=STYLED_ITEM('',(#126641),#67064) ;
#3642=STYLED_ITEM('',(#126641),#67065) ;
#3643=STYLED_ITEM('',(#126641),#67066) ;
#3644=STYLED_ITEM('',(#126641),#67067) ;
#3645=STYLED_ITEM('',(#126641),#67068) ;
#3646=STYLED_ITEM('',(#126641),#67069) ;
#3647=STYLED_ITEM('',(#126641),#67070) ;
#3648=STYLED_ITEM('',(#126641),#67071) ;
#3649=STYLED_ITEM('',(#126641),#67072) ;
#3650=STYLED_ITEM('',(#126641),#67073) ;
#3651=STYLED_ITEM('',(#126641),#67074) ;
#3652=STYLED_ITEM('',(#126641),#67075) ;
#3653=STYLED_ITEM('',(#126641),#67076) ;
#3654=STYLED_ITEM('',(#126641),#67077) ;
#3655=STYLED_ITEM('',(#126641),#67078) ;
#3656=STYLED_ITEM('',(#126641),#67079) ;
#3657=STYLED_ITEM('',(#126641),#67080) ;
#3658=STYLED_ITEM('',(#126641),#67081) ;
#3659=STYLED_ITEM('',(#126641),#67082) ;
#3660=STYLED_ITEM('',(#126641),#67083) ;
#3661=STYLED_ITEM('',(#126641),#67084) ;
#3662=STYLED_ITEM('',(#126641),#67085) ;
#3663=STYLED_ITEM('',(#126641),#67086) ;
#3664=STYLED_ITEM('',(#126641),#67087) ;
#3665=STYLED_ITEM('',(#126641),#67088) ;
#3666=STYLED_ITEM('',(#126641),#67089) ;
#3667=STYLED_ITEM('',(#126641),#67090) ;
#3668=STYLED_ITEM('',(#126641),#67091) ;
#3669=STYLED_ITEM('',(#126641),#67092) ;
#3670=STYLED_ITEM('',(#126641),#67093) ;
#3671=STYLED_ITEM('',(#126641),#67094) ;
#3672=STYLED_ITEM('',(#126641),#67095) ;
#3673=STYLED_ITEM('',(#126641),#67096) ;
#3674=STYLED_ITEM('',(#126641),#67097) ;
#3675=STYLED_ITEM('',(#126641),#67098) ;
#3676=STYLED_ITEM('',(#126641),#67099) ;
#3677=STYLED_ITEM('',(#126641),#67100) ;
#3678=STYLED_ITEM('',(#126641),#67101) ;
#3679=STYLED_ITEM('',(#126641),#67102) ;
#3680=STYLED_ITEM('',(#126641),#67103) ;
#3681=STYLED_ITEM('',(#126641),#67104) ;
#3682=STYLED_ITEM('',(#126641),#67105) ;
#3683=STYLED_ITEM('',(#126641),#67106) ;
#3684=STYLED_ITEM('',(#126641),#67107) ;
#3685=STYLED_ITEM('',(#126641),#67108) ;
#3686=STYLED_ITEM('',(#126641),#67109) ;
#3687=STYLED_ITEM('',(#126641),#67110) ;
#3688=STYLED_ITEM('',(#126641),#67111) ;
#3689=STYLED_ITEM('',(#126641),#67112) ;
#3690=STYLED_ITEM('',(#126641),#67113) ;
#3691=STYLED_ITEM('',(#126641),#67114) ;
#3692=STYLED_ITEM('',(#126641),#67115) ;
#3693=STYLED_ITEM('',(#126641),#67116) ;
#3694=STYLED_ITEM('',(#126641),#67117) ;
#3695=STYLED_ITEM('',(#126641),#67118) ;
#3696=STYLED_ITEM('',(#126641),#67119) ;
#3697=STYLED_ITEM('',(#126641),#67120) ;
#3698=STYLED_ITEM('',(#126641),#67121) ;
#3699=STYLED_ITEM('',(#126641),#67122) ;
#3700=STYLED_ITEM('',(#126641),#67123) ;
#3701=STYLED_ITEM('',(#126641),#67124) ;
#3702=STYLED_ITEM('',(#126641),#67125) ;
#3703=STYLED_ITEM('',(#126641),#67126) ;
#3704=STYLED_ITEM('',(#126641),#67127) ;
#3705=STYLED_ITEM('',(#126641),#67128) ;
#3706=STYLED_ITEM('',(#126641),#67129) ;
#3707=STYLED_ITEM('',(#126641),#67130) ;
#3708=STYLED_ITEM('',(#126641),#67131) ;
#3709=STYLED_ITEM('',(#126641),#67132) ;
#3710=STYLED_ITEM('',(#126641),#67133) ;
#3711=STYLED_ITEM('',(#126641),#67134) ;
#3712=STYLED_ITEM('',(#126641),#67135) ;
#3713=STYLED_ITEM('',(#126641),#67136) ;
#3714=STYLED_ITEM('',(#126641),#67137) ;
#3715=STYLED_ITEM('',(#126641),#67138) ;
#3716=STYLED_ITEM('',(#126641),#67139) ;
#3717=STYLED_ITEM('',(#126641),#67140) ;
#3718=STYLED_ITEM('',(#126641),#67141) ;
#3719=STYLED_ITEM('',(#126641),#67142) ;
#3720=STYLED_ITEM('',(#126641),#67143) ;
#3721=STYLED_ITEM('',(#126641),#67144) ;
#3722=STYLED_ITEM('',(#126641),#67145) ;
#3723=STYLED_ITEM('',(#126641),#67146) ;
#3724=STYLED_ITEM('',(#126641),#67147) ;
#3725=STYLED_ITEM('',(#126641),#67148) ;
#3726=STYLED_ITEM('',(#126641),#67149) ;
#3727=STYLED_ITEM('',(#126641),#67150) ;
#3728=STYLED_ITEM('',(#126641),#67151) ;
#3729=STYLED_ITEM('',(#126641),#67152) ;
#3730=STYLED_ITEM('',(#126641),#67153) ;
#3731=STYLED_ITEM('',(#126641),#67154) ;
#3732=STYLED_ITEM('',(#126641),#67155) ;
#3733=STYLED_ITEM('',(#126641),#67156) ;
#3734=STYLED_ITEM('',(#126641),#67157) ;
#3735=STYLED_ITEM('',(#126641),#67158) ;
#3736=STYLED_ITEM('',(#126641),#67159) ;
#3737=STYLED_ITEM('',(#126641),#67160) ;
#3738=STYLED_ITEM('',(#126641),#67161) ;
#3739=STYLED_ITEM('',(#126641),#67162) ;
#3740=STYLED_ITEM('',(#126641),#67163) ;
#3741=STYLED_ITEM('',(#126641),#67164) ;
#3742=STYLED_ITEM('',(#126641),#67165) ;
#3743=STYLED_ITEM('',(#126641),#67166) ;
#3744=STYLED_ITEM('',(#126641),#67167) ;
#3745=STYLED_ITEM('',(#126641),#67168) ;
#3746=STYLED_ITEM('',(#126641),#67169) ;
#3747=STYLED_ITEM('',(#126641),#67170) ;
#3748=STYLED_ITEM('',(#126641),#67171) ;
#3749=STYLED_ITEM('',(#126641),#67172) ;
#3750=STYLED_ITEM('',(#126641),#67173) ;
#3751=STYLED_ITEM('',(#126641),#67174) ;
#3752=STYLED_ITEM('',(#126641),#67175) ;
#3753=STYLED_ITEM('',(#126641),#67176) ;
#3754=STYLED_ITEM('',(#126641),#67177) ;
#3755=STYLED_ITEM('',(#126641),#67178) ;
#3756=STYLED_ITEM('',(#126641),#67179) ;
#3757=STYLED_ITEM('',(#126641),#67180) ;
#3758=STYLED_ITEM('',(#126641),#67181) ;
#3759=STYLED_ITEM('',(#126641),#67182) ;
#3760=STYLED_ITEM('',(#126641),#67183) ;
#3761=STYLED_ITEM('',(#126641),#67184) ;
#3762=STYLED_ITEM('',(#126641),#67185) ;
#3763=STYLED_ITEM('',(#126641),#67186) ;
#3764=STYLED_ITEM('',(#126641),#67187) ;
#3765=STYLED_ITEM('',(#126641),#67188) ;
#3766=STYLED_ITEM('',(#126641),#67189) ;
#3767=STYLED_ITEM('',(#126641),#67190) ;
#3768=STYLED_ITEM('',(#126641),#67191) ;
#3769=STYLED_ITEM('',(#126641),#67192) ;
#3770=STYLED_ITEM('',(#126641),#67193) ;
#3771=STYLED_ITEM('',(#126641),#67194) ;
#3772=STYLED_ITEM('',(#126641),#67195) ;
#3773=STYLED_ITEM('',(#126641),#67196) ;
#3774=STYLED_ITEM('',(#126641),#67197) ;
#3775=STYLED_ITEM('',(#126641),#67198) ;
#3776=STYLED_ITEM('',(#126641),#67199) ;
#3777=STYLED_ITEM('',(#126641),#67200) ;
#3778=STYLED_ITEM('',(#126641),#67201) ;
#3779=STYLED_ITEM('',(#126641),#67202) ;
#3780=STYLED_ITEM('',(#126641),#67203) ;
#3781=STYLED_ITEM('',(#126641),#67204) ;
#3782=STYLED_ITEM('',(#126641),#67205) ;
#3783=STYLED_ITEM('',(#126641),#67206) ;
#3784=STYLED_ITEM('',(#126641),#67207) ;
#3785=STYLED_ITEM('',(#126641),#67208) ;
#3786=STYLED_ITEM('',(#126641),#67209) ;
#3787=STYLED_ITEM('',(#126641),#67210) ;
#3788=STYLED_ITEM('',(#126641),#67211) ;
#3789=STYLED_ITEM('',(#126641),#67212) ;
#3790=STYLED_ITEM('',(#126641),#67213) ;
#3791=STYLED_ITEM('',(#126641),#67214) ;
#3792=STYLED_ITEM('',(#126641),#67215) ;
#3793=STYLED_ITEM('',(#126641),#67216) ;
#3794=STYLED_ITEM('',(#126641),#67217) ;
#3795=STYLED_ITEM('',(#126641),#67218) ;
#3796=STYLED_ITEM('',(#126641),#67219) ;
#3797=STYLED_ITEM('',(#126641),#67220) ;
#3798=STYLED_ITEM('',(#126641),#67221) ;
#3799=STYLED_ITEM('',(#126641),#67222) ;
#3800=STYLED_ITEM('',(#126641),#67223) ;
#3801=STYLED_ITEM('',(#126641),#67224) ;
#3802=STYLED_ITEM('',(#126641),#67225) ;
#3803=STYLED_ITEM('',(#126641),#67226) ;
#3804=STYLED_ITEM('',(#126641),#67227) ;
#3805=STYLED_ITEM('',(#126641),#67228) ;
#3806=STYLED_ITEM('',(#126641),#67229) ;
#3807=STYLED_ITEM('',(#126641),#67230) ;
#3808=STYLED_ITEM('',(#126641),#67231) ;
#3809=STYLED_ITEM('',(#126641),#67232) ;
#3810=STYLED_ITEM('',(#126641),#67233) ;
#3811=STYLED_ITEM('',(#126641),#67234) ;
#3812=STYLED_ITEM('',(#126641),#67235) ;
#3813=STYLED_ITEM('',(#126641),#67236) ;
#3814=STYLED_ITEM('',(#126641),#67237) ;
#3815=STYLED_ITEM('',(#126641),#67238) ;
#3816=STYLED_ITEM('',(#126641),#67239) ;
#3817=STYLED_ITEM('',(#126641),#67240) ;
#3818=STYLED_ITEM('',(#126641),#67241) ;
#3819=STYLED_ITEM('',(#126641),#67242) ;
#3820=STYLED_ITEM('',(#126641),#67243) ;
#3821=STYLED_ITEM('',(#126641),#67244) ;
#3822=STYLED_ITEM('',(#126641),#67245) ;
#3823=STYLED_ITEM('',(#126641),#67246) ;
#3824=STYLED_ITEM('',(#126641),#67247) ;
#3825=STYLED_ITEM('',(#126641),#67248) ;
#3826=STYLED_ITEM('',(#126641),#67249) ;
#3827=STYLED_ITEM('',(#126641),#67250) ;
#3828=STYLED_ITEM('',(#126641),#67251) ;
#3829=STYLED_ITEM('',(#126641),#67252) ;
#3830=STYLED_ITEM('',(#126641),#67253) ;
#3831=STYLED_ITEM('',(#126641),#67254) ;
#3832=STYLED_ITEM('',(#126641),#67255) ;
#3833=STYLED_ITEM('',(#126641),#67256) ;
#3834=STYLED_ITEM('',(#126641),#67257) ;
#3835=STYLED_ITEM('',(#126641),#67258) ;
#3836=STYLED_ITEM('',(#126641),#67259) ;
#3837=STYLED_ITEM('',(#126641),#67260) ;
#3838=STYLED_ITEM('',(#126641),#67261) ;
#3839=STYLED_ITEM('',(#126641),#67262) ;
#3840=STYLED_ITEM('',(#126641),#67263) ;
#3841=STYLED_ITEM('',(#126641),#67264) ;
#3842=STYLED_ITEM('',(#126641),#67265) ;
#3843=STYLED_ITEM('',(#126641),#67266) ;
#3844=STYLED_ITEM('',(#126641),#67267) ;
#3845=STYLED_ITEM('',(#126641),#67268) ;
#3846=STYLED_ITEM('',(#126641),#67269) ;
#3847=STYLED_ITEM('',(#126641),#67270) ;
#3848=STYLED_ITEM('',(#126641),#67271) ;
#3849=STYLED_ITEM('',(#126641),#67272) ;
#3850=STYLED_ITEM('',(#126641),#67273) ;
#3851=STYLED_ITEM('',(#126641),#67274) ;
#3852=STYLED_ITEM('',(#126641),#67275) ;
#3853=STYLED_ITEM('',(#126641),#67276) ;
#3854=STYLED_ITEM('',(#126641),#67277) ;
#3855=STYLED_ITEM('',(#126641),#67278) ;
#3856=STYLED_ITEM('',(#126641),#67279) ;
#3857=STYLED_ITEM('',(#126641),#67280) ;
#3858=STYLED_ITEM('',(#126641),#67281) ;
#3859=STYLED_ITEM('',(#126641),#67282) ;
#3860=STYLED_ITEM('',(#126641),#67283) ;
#3861=STYLED_ITEM('',(#126641),#67284) ;
#3862=STYLED_ITEM('',(#126641),#67285) ;
#3863=STYLED_ITEM('',(#126641),#67286) ;
#3864=STYLED_ITEM('',(#126641),#67287) ;
#3865=STYLED_ITEM('',(#126641),#67288) ;
#3866=STYLED_ITEM('',(#126641),#67289) ;
#3867=STYLED_ITEM('',(#126641),#67290) ;
#3868=STYLED_ITEM('',(#126641),#67291) ;
#3869=STYLED_ITEM('',(#126641),#67292) ;
#3870=STYLED_ITEM('',(#126641),#67293) ;
#3871=STYLED_ITEM('',(#126641),#67294) ;
#3872=STYLED_ITEM('',(#126641),#67295) ;
#3873=STYLED_ITEM('',(#126641),#67296) ;
#3874=STYLED_ITEM('',(#126641),#67297) ;
#3875=STYLED_ITEM('',(#126641),#67298) ;
#3876=STYLED_ITEM('',(#126641),#67299) ;
#3877=STYLED_ITEM('',(#126641),#67300) ;
#3878=STYLED_ITEM('',(#126641),#67301) ;
#3879=STYLED_ITEM('',(#126641),#67302) ;
#3880=STYLED_ITEM('',(#126641),#67303) ;
#3881=STYLED_ITEM('',(#126641),#67304) ;
#3882=STYLED_ITEM('',(#126641),#67305) ;
#3883=STYLED_ITEM('',(#126641),#67306) ;
#3884=STYLED_ITEM('',(#126641),#67307) ;
#3885=STYLED_ITEM('',(#126641),#67308) ;
#3886=STYLED_ITEM('',(#126641),#67309) ;
#3887=STYLED_ITEM('',(#126641),#67310) ;
#3888=STYLED_ITEM('',(#126641),#67311) ;
#3889=STYLED_ITEM('',(#126641),#67312) ;
#3890=STYLED_ITEM('',(#126641),#67313) ;
#3891=STYLED_ITEM('',(#126641),#67314) ;
#3892=STYLED_ITEM('',(#126641),#67315) ;
#3893=STYLED_ITEM('',(#126641),#67316) ;
#3894=STYLED_ITEM('',(#126641),#67317) ;
#3895=STYLED_ITEM('',(#126641),#67318) ;
#3896=STYLED_ITEM('',(#126641),#67319) ;
#3897=STYLED_ITEM('',(#126641),#67320) ;
#3898=STYLED_ITEM('',(#126641),#67321) ;
#3899=STYLED_ITEM('',(#126641),#67322) ;
#3900=STYLED_ITEM('',(#126641),#67323) ;
#3901=STYLED_ITEM('',(#126641),#67324) ;
#3902=STYLED_ITEM('',(#126641),#67325) ;
#3903=STYLED_ITEM('',(#126641),#67326) ;
#3904=STYLED_ITEM('',(#126641),#67327) ;
#3905=STYLED_ITEM('',(#126641),#67328) ;
#3906=STYLED_ITEM('',(#126641),#67329) ;
#3907=STYLED_ITEM('',(#126641),#67330) ;
#3908=STYLED_ITEM('',(#126641),#67331) ;
#3909=STYLED_ITEM('',(#126641),#67332) ;
#3910=STYLED_ITEM('',(#126641),#67333) ;
#3911=STYLED_ITEM('',(#126641),#67334) ;
#3912=STYLED_ITEM('',(#126641),#67335) ;
#3913=STYLED_ITEM('',(#126641),#67336) ;
#3914=STYLED_ITEM('',(#126641),#67337) ;
#3915=STYLED_ITEM('',(#126641),#67338) ;
#3916=STYLED_ITEM('',(#126641),#67339) ;
#3917=STYLED_ITEM('',(#126641),#67340) ;
#3918=STYLED_ITEM('',(#126641),#67341) ;
#3919=STYLED_ITEM('',(#126641),#67342) ;
#3920=STYLED_ITEM('',(#126641),#67343) ;
#3921=STYLED_ITEM('',(#126641),#67344) ;
#3922=STYLED_ITEM('',(#126641),#67345) ;
#3923=STYLED_ITEM('',(#126641),#67346) ;
#3924=STYLED_ITEM('',(#126641),#67347) ;
#3925=STYLED_ITEM('',(#126641),#67348) ;
#3926=STYLED_ITEM('',(#126641),#67349) ;
#3927=STYLED_ITEM('',(#126641),#67350) ;
#3928=STYLED_ITEM('',(#126641),#67351) ;
#3929=STYLED_ITEM('',(#126641),#67352) ;
#3930=STYLED_ITEM('',(#126641),#67353) ;
#3931=STYLED_ITEM('',(#126641),#67354) ;
#3932=STYLED_ITEM('',(#126641),#67355) ;
#3933=STYLED_ITEM('',(#126641),#67356) ;
#3934=STYLED_ITEM('',(#126641),#67357) ;
#3935=STYLED_ITEM('',(#126641),#67358) ;
#3936=STYLED_ITEM('',(#126641),#67359) ;
#3937=STYLED_ITEM('',(#126641),#67360) ;
#3938=STYLED_ITEM('',(#126641),#67361) ;
#3939=STYLED_ITEM('',(#126641),#67362) ;
#3940=STYLED_ITEM('',(#126641),#67363) ;
#3941=STYLED_ITEM('',(#126641),#67364) ;
#3942=STYLED_ITEM('',(#126641),#67365) ;
#3943=STYLED_ITEM('',(#126641),#67366) ;
#3944=STYLED_ITEM('',(#126641),#67367) ;
#3945=STYLED_ITEM('',(#126641),#67368) ;
#3946=STYLED_ITEM('',(#126641),#67369) ;
#3947=STYLED_ITEM('',(#126641),#67370) ;
#3948=STYLED_ITEM('',(#126641),#67371) ;
#3949=STYLED_ITEM('',(#126641),#67372) ;
#3950=STYLED_ITEM('',(#126641),#67373) ;
#3951=STYLED_ITEM('',(#126641),#67374) ;
#3952=STYLED_ITEM('',(#126641),#67375) ;
#3953=STYLED_ITEM('',(#126641),#67376) ;
#3954=STYLED_ITEM('',(#126641),#67377) ;
#3955=STYLED_ITEM('',(#126641),#67378) ;
#3956=STYLED_ITEM('',(#126641),#67379) ;
#3957=STYLED_ITEM('',(#126641),#67380) ;
#3958=STYLED_ITEM('',(#126641),#67381) ;
#3959=STYLED_ITEM('',(#126641),#67382) ;
#3960=STYLED_ITEM('',(#126641),#67383) ;
#3961=STYLED_ITEM('',(#126641),#67384) ;
#3962=STYLED_ITEM('',(#126641),#67385) ;
#3963=STYLED_ITEM('',(#126641),#67386) ;
#3964=STYLED_ITEM('',(#126641),#67387) ;
#3965=STYLED_ITEM('',(#126641),#67388) ;
#3966=STYLED_ITEM('',(#126641),#67389) ;
#3967=STYLED_ITEM('',(#126641),#67390) ;
#3968=STYLED_ITEM('',(#126641),#67391) ;
#3969=STYLED_ITEM('',(#126641),#67392) ;
#3970=STYLED_ITEM('',(#126641),#67393) ;
#3971=STYLED_ITEM('',(#126641),#67394) ;
#3972=STYLED_ITEM('',(#126641),#67395) ;
#3973=STYLED_ITEM('',(#126641),#67396) ;
#3974=STYLED_ITEM('',(#126641),#67397) ;
#3975=STYLED_ITEM('',(#126641),#67398) ;
#3976=STYLED_ITEM('',(#126641),#67399) ;
#3977=STYLED_ITEM('',(#126641),#67400) ;
#3978=STYLED_ITEM('',(#126641),#67401) ;
#3979=STYLED_ITEM('',(#126641),#67402) ;
#3980=STYLED_ITEM('',(#126641),#67403) ;
#3981=STYLED_ITEM('',(#126641),#67404) ;
#3982=STYLED_ITEM('',(#126641),#67405) ;
#3983=STYLED_ITEM('',(#126641),#67406) ;
#3984=STYLED_ITEM('',(#126641),#67407) ;
#3985=STYLED_ITEM('',(#126641),#67408) ;
#3986=STYLED_ITEM('',(#126641),#67409) ;
#3987=STYLED_ITEM('',(#126641),#67410) ;
#3988=STYLED_ITEM('',(#126641),#67411) ;
#3989=STYLED_ITEM('',(#126641),#67412) ;
#3990=STYLED_ITEM('',(#126641),#67413) ;
#3991=STYLED_ITEM('',(#126641),#67414) ;
#3992=STYLED_ITEM('',(#126641),#67415) ;
#3993=STYLED_ITEM('',(#126641),#67416) ;
#3994=STYLED_ITEM('',(#126641),#67417) ;
#3995=STYLED_ITEM('',(#126641),#67418) ;
#3996=STYLED_ITEM('',(#126641),#67419) ;
#3997=STYLED_ITEM('',(#126641),#67420) ;
#3998=STYLED_ITEM('',(#126641),#67421) ;
#3999=STYLED_ITEM('',(#126641),#67422) ;
#4000=STYLED_ITEM('',(#126641),#67423) ;
#4001=STYLED_ITEM('',(#126641),#67424) ;
#4002=STYLED_ITEM('',(#126641),#67425) ;
#4003=STYLED_ITEM('',(#126641),#67426) ;
#4004=STYLED_ITEM('',(#126641),#67427) ;
#4005=STYLED_ITEM('',(#126641),#67428) ;
#4006=STYLED_ITEM('',(#126641),#67429) ;
#4007=STYLED_ITEM('',(#126641),#67430) ;
#4008=STYLED_ITEM('',(#126641),#67431) ;
#4009=STYLED_ITEM('',(#126641),#67432) ;
#4010=STYLED_ITEM('',(#126641),#67433) ;
#4011=STYLED_ITEM('',(#126641),#67434) ;
#4012=STYLED_ITEM('',(#126641),#67435) ;
#4013=STYLED_ITEM('',(#126641),#67436) ;
#4014=STYLED_ITEM('',(#126641),#67437) ;
#4015=STYLED_ITEM('',(#126641),#67438) ;
#4016=STYLED_ITEM('',(#126641),#67439) ;
#4017=STYLED_ITEM('',(#126641),#67440) ;
#4018=STYLED_ITEM('',(#126641),#67441) ;
#4019=STYLED_ITEM('',(#126641),#67442) ;
#4020=STYLED_ITEM('',(#126641),#67443) ;
#4021=STYLED_ITEM('',(#126641),#67444) ;
#4022=STYLED_ITEM('',(#126641),#67445) ;
#4023=STYLED_ITEM('',(#126641),#67446) ;
#4024=STYLED_ITEM('',(#126641),#67447) ;
#4025=STYLED_ITEM('',(#126641),#67448) ;
#4026=STYLED_ITEM('',(#126641),#67449) ;
#4027=STYLED_ITEM('',(#126641),#67450) ;
#4028=STYLED_ITEM('',(#126641),#67451) ;
#4029=STYLED_ITEM('',(#126641),#67452) ;
#4030=STYLED_ITEM('',(#126641),#67453) ;
#4031=STYLED_ITEM('',(#126641),#67454) ;
#4032=STYLED_ITEM('',(#126641),#67455) ;
#4033=STYLED_ITEM('',(#126641),#67456) ;
#4034=STYLED_ITEM('',(#126641),#67457) ;
#4035=STYLED_ITEM('',(#126641),#67458) ;
#4036=STYLED_ITEM('',(#126641),#67459) ;
#4037=STYLED_ITEM('',(#126641),#67460) ;
#4038=STYLED_ITEM('',(#126641),#67461) ;
#4039=STYLED_ITEM('',(#126641),#67462) ;
#4040=STYLED_ITEM('',(#126641),#67463) ;
#4041=STYLED_ITEM('',(#126641),#67464) ;
#4042=STYLED_ITEM('',(#126641),#67465) ;
#4043=STYLED_ITEM('',(#126641),#67466) ;
#4044=STYLED_ITEM('',(#126641),#67467) ;
#4045=STYLED_ITEM('',(#126641),#67468) ;
#4046=STYLED_ITEM('',(#126641),#67469) ;
#4047=STYLED_ITEM('',(#126641),#67470) ;
#4048=STYLED_ITEM('',(#126641),#67471) ;
#4049=STYLED_ITEM('',(#126641),#67472) ;
#4050=STYLED_ITEM('',(#126641),#67473) ;
#4051=STYLED_ITEM('',(#126641),#67474) ;
#4052=STYLED_ITEM('',(#126641),#67475) ;
#4053=STYLED_ITEM('',(#126641),#67476) ;
#4054=STYLED_ITEM('',(#126641),#67477) ;
#4055=STYLED_ITEM('',(#126641),#67478) ;
#4056=STYLED_ITEM('',(#126641),#67479) ;
#4057=STYLED_ITEM('',(#126641),#67480) ;
#4058=STYLED_ITEM('',(#126641),#67481) ;
#4059=STYLED_ITEM('',(#126641),#67482) ;
#4060=STYLED_ITEM('',(#126641),#67483) ;
#4061=STYLED_ITEM('',(#126641),#67484) ;
#4062=STYLED_ITEM('',(#126641),#67485) ;
#4063=STYLED_ITEM('',(#126641),#67486) ;
#4064=STYLED_ITEM('',(#126641),#67487) ;
#4065=STYLED_ITEM('',(#126641),#67488) ;
#4066=STYLED_ITEM('',(#126641),#67489) ;
#4067=STYLED_ITEM('',(#126641),#67490) ;
#4068=STYLED_ITEM('',(#126641),#67491) ;
#4069=STYLED_ITEM('',(#126641),#67492) ;
#4070=STYLED_ITEM('',(#126641),#67493) ;
#4071=STYLED_ITEM('',(#126641),#67494) ;
#4072=STYLED_ITEM('',(#126641),#67495) ;
#4073=STYLED_ITEM('',(#126641),#67496) ;
#4074=STYLED_ITEM('',(#126641),#67497) ;
#4075=STYLED_ITEM('',(#126641),#67498) ;
#4076=STYLED_ITEM('',(#126641),#67499) ;
#4077=STYLED_ITEM('',(#126641),#67500) ;
#4078=STYLED_ITEM('',(#126641),#67501) ;
#4079=STYLED_ITEM('',(#126641),#67502) ;
#4080=STYLED_ITEM('',(#126641),#67503) ;
#4081=STYLED_ITEM('',(#126641),#67504) ;
#4082=STYLED_ITEM('',(#126641),#67505) ;
#4083=STYLED_ITEM('',(#126641),#67506) ;
#4084=STYLED_ITEM('',(#126641),#67507) ;
#4085=STYLED_ITEM('',(#126641),#67508) ;
#4086=STYLED_ITEM('',(#126641),#67509) ;
#4087=STYLED_ITEM('',(#126641),#67510) ;
#4088=STYLED_ITEM('',(#126641),#67511) ;
#4089=STYLED_ITEM('',(#126641),#67512) ;
#4090=STYLED_ITEM('',(#126641),#67513) ;
#4091=STYLED_ITEM('',(#126641),#67514) ;
#4092=STYLED_ITEM('',(#126641),#67515) ;
#4093=STYLED_ITEM('',(#126641),#67516) ;
#4094=STYLED_ITEM('',(#126641),#67517) ;
#4095=STYLED_ITEM('',(#126641),#67518) ;
#4096=STYLED_ITEM('',(#126641),#67519) ;
#4097=STYLED_ITEM('',(#126641),#67520) ;
#4098=STYLED_ITEM('',(#126641),#67521) ;
#4099=STYLED_ITEM('',(#126641),#67522) ;
#4100=STYLED_ITEM('',(#126641),#67523) ;
#4101=STYLED_ITEM('',(#126641),#67524) ;
#4102=STYLED_ITEM('',(#126641),#67525) ;
#4103=STYLED_ITEM('',(#126641),#67526) ;
#4104=STYLED_ITEM('',(#126641),#67527) ;
#4105=STYLED_ITEM('',(#126641),#67528) ;
#4106=STYLED_ITEM('',(#126641),#67529) ;
#4107=STYLED_ITEM('',(#126641),#67530) ;
#4108=STYLED_ITEM('',(#126641),#67531) ;
#4109=STYLED_ITEM('',(#126641),#67532) ;
#4110=STYLED_ITEM('',(#126641),#67533) ;
#4111=STYLED_ITEM('',(#126641),#67534) ;
#4112=STYLED_ITEM('',(#126641),#67535) ;
#4113=STYLED_ITEM('',(#126641),#67536) ;
#4114=STYLED_ITEM('',(#126641),#67537) ;
#4115=STYLED_ITEM('',(#126641),#67538) ;
#4116=STYLED_ITEM('',(#126641),#67539) ;
#4117=STYLED_ITEM('',(#126641),#67540) ;
#4118=STYLED_ITEM('',(#126641),#67541) ;
#4119=STYLED_ITEM('',(#126641),#67542) ;
#4120=STYLED_ITEM('',(#126641),#67543) ;
#4121=STYLED_ITEM('',(#126641),#67544) ;
#4122=STYLED_ITEM('',(#126641),#67545) ;
#4123=STYLED_ITEM('',(#126641),#67546) ;
#4124=STYLED_ITEM('',(#126641),#67547) ;
#4125=STYLED_ITEM('',(#126641),#67548) ;
#4126=STYLED_ITEM('',(#126641),#67549) ;
#4127=STYLED_ITEM('',(#126641),#67550) ;
#4128=STYLED_ITEM('',(#126641),#67551) ;
#4129=STYLED_ITEM('',(#126641),#67552) ;
#4130=STYLED_ITEM('',(#126641),#67553) ;
#4131=STYLED_ITEM('',(#126641),#67554) ;
#4132=STYLED_ITEM('',(#126641),#67555) ;
#4133=STYLED_ITEM('',(#126641),#67556) ;
#4134=STYLED_ITEM('',(#126641),#67557) ;
#4135=STYLED_ITEM('',(#126641),#67558) ;
#4136=STYLED_ITEM('',(#126641),#67559) ;
#4137=STYLED_ITEM('',(#126641),#67560) ;
#4138=STYLED_ITEM('',(#126641),#67561) ;
#4139=STYLED_ITEM('',(#126641),#67562) ;
#4140=STYLED_ITEM('',(#126641),#67563) ;
#4141=STYLED_ITEM('',(#126641),#67564) ;
#4142=STYLED_ITEM('',(#126641),#67565) ;
#4143=STYLED_ITEM('',(#126641),#67566) ;
#4144=STYLED_ITEM('',(#126641),#67567) ;
#4145=STYLED_ITEM('',(#126641),#67568) ;
#4146=STYLED_ITEM('',(#126641),#67569) ;
#4147=STYLED_ITEM('',(#126641),#67570) ;
#4148=STYLED_ITEM('',(#126641),#67571) ;
#4149=STYLED_ITEM('',(#126641),#67572) ;
#4150=STYLED_ITEM('',(#126641),#67573) ;
#4151=STYLED_ITEM('',(#126641),#67574) ;
#4152=STYLED_ITEM('',(#126641),#67575) ;
#4153=STYLED_ITEM('',(#126641),#67576) ;
#4154=STYLED_ITEM('',(#126641),#67577) ;
#4155=STYLED_ITEM('',(#126641),#67578) ;
#4156=STYLED_ITEM('',(#126641),#67579) ;
#4157=STYLED_ITEM('',(#126641),#67580) ;
#4158=STYLED_ITEM('',(#126641),#67581) ;
#4159=STYLED_ITEM('',(#126641),#67582) ;
#4160=STYLED_ITEM('',(#126641),#67583) ;
#4161=STYLED_ITEM('',(#126641),#67584) ;
#4162=STYLED_ITEM('',(#126641),#67585) ;
#4163=STYLED_ITEM('',(#126641),#67586) ;
#4164=STYLED_ITEM('',(#126641),#67587) ;
#4165=STYLED_ITEM('',(#126641),#67588) ;
#4166=STYLED_ITEM('',(#126641),#67589) ;
#4167=STYLED_ITEM('',(#126641),#67590) ;
#4168=STYLED_ITEM('',(#126641),#67591) ;
#4169=STYLED_ITEM('',(#126639),#4179) ;
#4179=MANIFOLD_SOLID_BREP('Body1',#67693) ;
#4427=SPHERICAL_SURFACE('',#71876,0.1) ;
#4428=SPHERICAL_SURFACE('',#71893,0.1) ;
#4429=SPHERICAL_SURFACE('',#71910,0.1) ;
#4430=SPHERICAL_SURFACE('',#71927,0.1) ;
#4431=SPHERICAL_SURFACE('',#71944,0.1) ;
#4432=SPHERICAL_SURFACE('',#71961,0.1) ;
#4433=SPHERICAL_SURFACE('',#71978,0.1) ;
#4434=SPHERICAL_SURFACE('',#71995,0.1) ;
#4435=SPHERICAL_SURFACE('',#72057,0.1) ;
#4436=SPHERICAL_SURFACE('',#72106,0.1) ;
#4437=SPHERICAL_SURFACE('',#72494,0.1) ;
#4438=SPHERICAL_SURFACE('',#72497,0.1) ;
#4439=SPHERICAL_SURFACE('',#72515,0.1) ;
#4440=SPHERICAL_SURFACE('',#72536,0.1) ;
#4441=SPHERICAL_SURFACE('',#72538,0.1) ;
#4442=SPHERICAL_SURFACE('',#72543,0.1) ;
#4443=SPHERICAL_SURFACE('',#72546,0.1) ;
#4444=SPHERICAL_SURFACE('',#72563,0.1) ;
#4445=SPHERICAL_SURFACE('',#72569,0.1) ;
#4446=SPHERICAL_SURFACE('',#72587,0.1) ;
#4447=SPHERICAL_SURFACE('',#72588,0.1) ;
#4448=SPHERICAL_SURFACE('',#72597,0.1) ;
#4449=SPHERICAL_SURFACE('',#72603,0.1) ;
#4450=SPHERICAL_SURFACE('',#72611,0.1) ;
#4451=SPHERICAL_SURFACE('',#72613,0.1) ;
#4452=SPHERICAL_SURFACE('',#72619,0.1) ;
#4453=SPHERICAL_SURFACE('',#72620,0.1) ;
#4454=SPHERICAL_SURFACE('',#72629,0.1) ;
#4455=SPHERICAL_SURFACE('',#72635,0.1) ;
#4456=SPHERICAL_SURFACE('',#72643,0.1) ;
#4457=SPHERICAL_SURFACE('',#72645,0.1) ;
#4458=SPHERICAL_SURFACE('',#72651,0.1) ;
#4459=SPHERICAL_SURFACE('',#72657,0.1) ;
#4460=SPHERICAL_SURFACE('',#72665,0.1) ;
#4461=SPHERICAL_SURFACE('',#72671,0.1) ;
#4462=SPHERICAL_SURFACE('',#72673,0.1) ;
#4463=SPHERICAL_SURFACE('',#72679,0.1) ;
#4464=SPHERICAL_SURFACE('',#72681,0.1) ;
#4465=SPHERICAL_SURFACE('',#72686,0.1) ;
#4466=SPHERICAL_SURFACE('',#72692,0.1) ;
#4467=SPHERICAL_SURFACE('',#72694,0.1) ;
#4468=SPHERICAL_SURFACE('',#72708,0.1) ;
#4469=SPHERICAL_SURFACE('',#72710,0.1) ;
#4470=SPHERICAL_SURFACE('',#72745,0.1) ;
#4471=SPHERICAL_SURFACE('',#72753,0.1) ;
#4472=SPHERICAL_SURFACE('',#72792,0.1) ;
#4473=SPHERICAL_SURFACE('',#72802,0.1) ;
#4474=SPHERICAL_SURFACE('',#72804,0.1) ;
#4475=SPHERICAL_SURFACE('',#72813,0.1) ;
#4476=SPHERICAL_SURFACE('',#72826,0.1) ;
#4477=SPHERICAL_SURFACE('',#72836,0.1) ;
#4478=SPHERICAL_SURFACE('',#72838,0.1) ;
#4479=SPHERICAL_SURFACE('',#72847,0.1) ;
#4480=SPHERICAL_SURFACE('',#72858,0.1) ;
#4481=SPHERICAL_SURFACE('',#72862,0.1) ;
#4482=SPHERICAL_SURFACE('',#72871,0.1) ;
#4483=SPHERICAL_SURFACE('',#72875,0.1) ;
#4484=SPHERICAL_SURFACE('',#72882,0.1) ;
#4485=SPHERICAL_SURFACE('',#72886,0.1) ;
#4486=SPHERICAL_SURFACE('',#72891,0.1) ;
#4487=SPHERICAL_SURFACE('',#72897,0.1) ;
#4488=SPHERICAL_SURFACE('',#73561,0.1) ;
#4489=SPHERICAL_SURFACE('',#73564,0.1) ;
#4490=SPHERICAL_SURFACE('',#73582,0.1) ;
#4491=SPHERICAL_SURFACE('',#73603,0.1) ;
#4492=SPHERICAL_SURFACE('',#73605,0.1) ;
#4493=SPHERICAL_SURFACE('',#73610,0.1) ;
#4494=SPHERICAL_SURFACE('',#73613,0.1) ;
#4495=SPHERICAL_SURFACE('',#73630,0.1) ;
#4496=SPHERICAL_SURFACE('',#73636,0.1) ;
#4497=SPHERICAL_SURFACE('',#73654,0.1) ;
#4498=SPHERICAL_SURFACE('',#73660,0.1) ;
#4499=SPHERICAL_SURFACE('',#73668,0.1) ;
#4500=SPHERICAL_SURFACE('',#73674,0.1) ;
#4501=SPHERICAL_SURFACE('',#73676,0.1) ;
#4502=SPHERICAL_SURFACE('',#73682,0.1) ;
#4503=SPHERICAL_SURFACE('',#73684,0.1) ;
#4504=SPHERICAL_SURFACE('',#73689,0.1) ;
#4505=SPHERICAL_SURFACE('',#73695,0.1) ;
#4506=SPHERICAL_SURFACE('',#73697,0.1) ;
#4507=SPHERICAL_SURFACE('',#73711,0.1) ;
#4508=SPHERICAL_SURFACE('',#73713,0.1) ;
#4509=SPHERICAL_SURFACE('',#73748,0.1) ;
#4510=SPHERICAL_SURFACE('',#73756,0.1) ;
#4511=SPHERICAL_SURFACE('',#73764,0.1) ;
#4512=SPHERICAL_SURFACE('',#73766,0.1) ;
#4513=SPHERICAL_SURFACE('',#73801,0.1) ;
#4514=SPHERICAL_SURFACE('',#73809,0.1) ;
#4515=SPHERICAL_SURFACE('',#73817,0.1) ;
#4516=SPHERICAL_SURFACE('',#73819,0.1) ;
#4517=SPHERICAL_SURFACE('',#73854,0.1) ;
#4518=SPHERICAL_SURFACE('',#73862,0.1) ;
#4519=SPHERICAL_SURFACE('',#73870,0.1) ;
#4520=SPHERICAL_SURFACE('',#73872,0.1) ;
#4521=SPHERICAL_SURFACE('',#73907,0.1) ;
#4522=SPHERICAL_SURFACE('',#73915,0.1) ;
#4523=SPHERICAL_SURFACE('',#73923,0.1) ;
#4524=SPHERICAL_SURFACE('',#73925,0.1) ;
#4525=SPHERICAL_SURFACE('',#73960,0.1) ;
#4526=SPHERICAL_SURFACE('',#73968,0.1) ;
#4527=SPHERICAL_SURFACE('',#73976,0.1) ;
#4528=SPHERICAL_SURFACE('',#73978,0.1) ;
#4529=SPHERICAL_SURFACE('',#74013,0.1) ;
#4530=SPHERICAL_SURFACE('',#74021,0.1) ;
#4531=SPHERICAL_SURFACE('',#74029,0.1) ;
#4532=SPHERICAL_SURFACE('',#74031,0.1) ;
#4533=SPHERICAL_SURFACE('',#74066,0.1) ;
#4534=SPHERICAL_SURFACE('',#74074,0.1) ;
#4535=SPHERICAL_SURFACE('',#74082,0.1) ;
#4536=SPHERICAL_SURFACE('',#74084,0.1) ;
#4537=SPHERICAL_SURFACE('',#74119,0.1) ;
#4538=SPHERICAL_SURFACE('',#74127,0.1) ;
#4539=SPHERICAL_SURFACE('',#74135,0.1) ;
#4540=SPHERICAL_SURFACE('',#74137,0.1) ;
#4541=SPHERICAL_SURFACE('',#74172,0.1) ;
#4542=SPHERICAL_SURFACE('',#74180,0.1) ;
#4543=SPHERICAL_SURFACE('',#74191,0.1) ;
#4544=SPHERICAL_SURFACE('',#74194,0.1) ;
#4545=SPHERICAL_SURFACE('',#74212,0.1) ;
#4546=SPHERICAL_SURFACE('',#74233,0.1) ;
#4547=SPHERICAL_SURFACE('',#74235,0.1) ;
#4548=SPHERICAL_SURFACE('',#74240,0.1) ;
#4549=SPHERICAL_SURFACE('',#74243,0.1) ;
#4550=SPHERICAL_SURFACE('',#74260,0.1) ;
#4551=SPHERICAL_SURFACE('',#74266,0.1) ;
#4552=SPHERICAL_SURFACE('',#74284,0.1) ;
#4553=SPHERICAL_SURFACE('',#74290,0.1) ;
#4554=SPHERICAL_SURFACE('',#74298,0.1) ;
#4555=SPHERICAL_SURFACE('',#74304,0.1) ;
#4556=SPHERICAL_SURFACE('',#74306,0.1) ;
#4557=SPHERICAL_SURFACE('',#74312,0.1) ;
#4558=SPHERICAL_SURFACE('',#74314,0.1) ;
#4559=SPHERICAL_SURFACE('',#74319,0.1) ;
#4560=SPHERICAL_SURFACE('',#74325,0.1) ;
#4561=SPHERICAL_SURFACE('',#74327,0.1) ;
#4562=SPHERICAL_SURFACE('',#74344,0.1) ;
#4563=SPHERICAL_SURFACE('',#74347,0.1) ;
#4564=SPHERICAL_SURFACE('',#74365,0.1) ;
#4565=SPHERICAL_SURFACE('',#74386,0.1) ;
#4566=SPHERICAL_SURFACE('',#74388,0.1) ;
#4567=SPHERICAL_SURFACE('',#74393,0.1) ;
#4568=SPHERICAL_SURFACE('',#74396,0.1) ;
#4569=SPHERICAL_SURFACE('',#74413,0.1) ;
#4570=SPHERICAL_SURFACE('',#74419,0.1) ;
#4571=SPHERICAL_SURFACE('',#74437,0.1) ;
#4572=SPHERICAL_SURFACE('',#74443,0.1) ;
#4573=SPHERICAL_SURFACE('',#74451,0.1) ;
#4574=SPHERICAL_SURFACE('',#74457,0.1) ;
#4575=SPHERICAL_SURFACE('',#74459,0.1) ;
#4576=SPHERICAL_SURFACE('',#74465,0.1) ;
#4577=SPHERICAL_SURFACE('',#74467,0.1) ;
#4578=SPHERICAL_SURFACE('',#74472,0.1) ;
#4579=SPHERICAL_SURFACE('',#74478,0.1) ;
#4580=SPHERICAL_SURFACE('',#74480,0.1) ;
#4581=SPHERICAL_SURFACE('',#74497,0.1) ;
#4582=SPHERICAL_SURFACE('',#74500,0.1) ;
#4583=SPHERICAL_SURFACE('',#74518,0.1) ;
#4584=SPHERICAL_SURFACE('',#74539,0.1) ;
#4585=SPHERICAL_SURFACE('',#74541,0.1) ;
#4586=SPHERICAL_SURFACE('',#74546,0.1) ;
#4587=SPHERICAL_SURFACE('',#74549,0.1) ;
#4588=SPHERICAL_SURFACE('',#74566,0.1) ;
#4589=SPHERICAL_SURFACE('',#74572,0.1) ;
#4590=SPHERICAL_SURFACE('',#74590,0.1) ;
#4591=SPHERICAL_SURFACE('',#74596,0.1) ;
#4592=SPHERICAL_SURFACE('',#74604,0.1) ;
#4593=SPHERICAL_SURFACE('',#74610,0.1) ;
#4594=SPHERICAL_SURFACE('',#74612,0.1) ;
#4595=SPHERICAL_SURFACE('',#74618,0.1) ;
#4596=SPHERICAL_SURFACE('',#74620,0.1) ;
#4597=SPHERICAL_SURFACE('',#74625,0.1) ;
#4598=SPHERICAL_SURFACE('',#74631,0.1) ;
#4599=SPHERICAL_SURFACE('',#74633,0.1) ;
#4600=SPHERICAL_SURFACE('',#74650,0.1) ;
#4601=SPHERICAL_SURFACE('',#74653,0.1) ;
#4602=SPHERICAL_SURFACE('',#74671,0.1) ;
#4603=SPHERICAL_SURFACE('',#74692,0.1) ;
#4604=SPHERICAL_SURFACE('',#74694,0.1) ;
#4605=SPHERICAL_SURFACE('',#74699,0.1) ;
#4606=SPHERICAL_SURFACE('',#74702,0.1) ;
#4607=SPHERICAL_SURFACE('',#74719,0.1) ;
#4608=SPHERICAL_SURFACE('',#74725,0.1) ;
#4609=SPHERICAL_SURFACE('',#74743,0.1) ;
#4610=SPHERICAL_SURFACE('',#74749,0.1) ;
#4611=SPHERICAL_SURFACE('',#74757,0.1) ;
#4612=SPHERICAL_SURFACE('',#74763,0.1) ;
#4613=SPHERICAL_SURFACE('',#74765,0.1) ;
#4614=SPHERICAL_SURFACE('',#74771,0.1) ;
#4615=SPHERICAL_SURFACE('',#74773,0.1) ;
#4616=SPHERICAL_SURFACE('',#74778,0.1) ;
#4617=SPHERICAL_SURFACE('',#74784,0.1) ;
#4618=SPHERICAL_SURFACE('',#74786,0.1) ;
#4619=SPHERICAL_SURFACE('',#74803,0.1) ;
#4620=SPHERICAL_SURFACE('',#74806,0.1) ;
#4621=SPHERICAL_SURFACE('',#74824,0.1) ;
#4622=SPHERICAL_SURFACE('',#74845,0.1) ;
#4623=SPHERICAL_SURFACE('',#74847,0.1) ;
#4624=SPHERICAL_SURFACE('',#74852,0.1) ;
#4625=SPHERICAL_SURFACE('',#74855,0.1) ;
#4626=SPHERICAL_SURFACE('',#74872,0.1) ;
#4627=SPHERICAL_SURFACE('',#74878,0.1) ;
#4628=SPHERICAL_SURFACE('',#74896,0.1) ;
#4629=SPHERICAL_SURFACE('',#74902,0.1) ;
#4630=SPHERICAL_SURFACE('',#74910,0.1) ;
#4631=SPHERICAL_SURFACE('',#74916,0.1) ;
#4632=SPHERICAL_SURFACE('',#74918,0.1) ;
#4633=SPHERICAL_SURFACE('',#74924,0.1) ;
#4634=SPHERICAL_SURFACE('',#74926,0.1) ;
#4635=SPHERICAL_SURFACE('',#74931,0.1) ;
#4636=SPHERICAL_SURFACE('',#74937,0.1) ;
#4637=SPHERICAL_SURFACE('',#74939,0.1) ;
#4638=SPHERICAL_SURFACE('',#74956,0.1) ;
#4639=SPHERICAL_SURFACE('',#74959,0.1) ;
#4640=SPHERICAL_SURFACE('',#74977,0.1) ;
#4641=SPHERICAL_SURFACE('',#74998,0.1) ;
#4642=SPHERICAL_SURFACE('',#75000,0.1) ;
#4643=SPHERICAL_SURFACE('',#75005,0.1) ;
#4644=SPHERICAL_SURFACE('',#75008,0.1) ;
#4645=SPHERICAL_SURFACE('',#75025,0.1) ;
#4646=SPHERICAL_SURFACE('',#75031,0.1) ;
#4647=SPHERICAL_SURFACE('',#75049,0.1) ;
#4648=SPHERICAL_SURFACE('',#75055,0.1) ;
#4649=SPHERICAL_SURFACE('',#75063,0.1) ;
#4650=SPHERICAL_SURFACE('',#75069,0.1) ;
#4651=SPHERICAL_SURFACE('',#75071,0.1) ;
#4652=SPHERICAL_SURFACE('',#75077,0.1) ;
#4653=SPHERICAL_SURFACE('',#75079,0.1) ;
#4654=SPHERICAL_SURFACE('',#75084,0.1) ;
#4655=SPHERICAL_SURFACE('',#75090,0.1) ;
#4656=SPHERICAL_SURFACE('',#75092,0.1) ;
#4657=SPHERICAL_SURFACE('',#75109,0.1) ;
#4658=SPHERICAL_SURFACE('',#75112,0.1) ;
#4659=SPHERICAL_SURFACE('',#75130,0.1) ;
#4660=SPHERICAL_SURFACE('',#75151,0.1) ;
#4661=SPHERICAL_SURFACE('',#75153,0.1) ;
#4662=SPHERICAL_SURFACE('',#75158,0.1) ;
#4663=SPHERICAL_SURFACE('',#75161,0.1) ;
#4664=SPHERICAL_SURFACE('',#75178,0.1) ;
#4665=SPHERICAL_SURFACE('',#75184,0.1) ;
#4666=SPHERICAL_SURFACE('',#75202,0.1) ;
#4667=SPHERICAL_SURFACE('',#75208,0.1) ;
#4668=SPHERICAL_SURFACE('',#75216,0.1) ;
#4669=SPHERICAL_SURFACE('',#75222,0.1) ;
#4670=SPHERICAL_SURFACE('',#75224,0.1) ;
#4671=SPHERICAL_SURFACE('',#75230,0.1) ;
#4672=SPHERICAL_SURFACE('',#75232,0.1) ;
#4673=SPHERICAL_SURFACE('',#75237,0.1) ;
#4674=SPHERICAL_SURFACE('',#75243,0.1) ;
#4675=SPHERICAL_SURFACE('',#75245,0.1) ;
#4676=SPHERICAL_SURFACE('',#75262,0.1) ;
#4677=SPHERICAL_SURFACE('',#75265,0.1) ;
#4678=SPHERICAL_SURFACE('',#75283,0.1) ;
#4679=SPHERICAL_SURFACE('',#75304,0.1) ;
#4680=SPHERICAL_SURFACE('',#75306,0.1) ;
#4681=SPHERICAL_SURFACE('',#75311,0.1) ;
#4682=SPHERICAL_SURFACE('',#75314,0.1) ;
#4683=SPHERICAL_SURFACE('',#75331,0.1) ;
#4684=SPHERICAL_SURFACE('',#75337,0.1) ;
#4685=SPHERICAL_SURFACE('',#75355,0.1) ;
#4686=SPHERICAL_SURFACE('',#75361,0.1) ;
#4687=SPHERICAL_SURFACE('',#75369,0.1) ;
#4688=SPHERICAL_SURFACE('',#75375,0.1) ;
#4689=SPHERICAL_SURFACE('',#75377,0.1) ;
#4690=SPHERICAL_SURFACE('',#75383,0.1) ;
#4691=SPHERICAL_SURFACE('',#75385,0.1) ;
#4692=SPHERICAL_SURFACE('',#75390,0.1) ;
#4693=SPHERICAL_SURFACE('',#75396,0.1) ;
#4694=SPHERICAL_SURFACE('',#75398,0.1) ;
#4695=SPHERICAL_SURFACE('',#75667,0.1) ;
#4696=SPHERICAL_SURFACE('',#75677,0.1) ;
#4697=SPHERICAL_SURFACE('',#75679,0.1) ;
#4698=SPHERICAL_SURFACE('',#75688,0.1) ;
#4699=SPHERICAL_SURFACE('',#75701,0.1) ;
#4700=SPHERICAL_SURFACE('',#75711,0.1) ;
#4701=SPHERICAL_SURFACE('',#75713,0.1) ;
#4702=SPHERICAL_SURFACE('',#75722,0.1) ;
#4703=SPHERICAL_SURFACE('',#75735,0.1) ;
#4704=SPHERICAL_SURFACE('',#75745,0.1) ;
#4705=SPHERICAL_SURFACE('',#75747,0.1) ;
#4706=SPHERICAL_SURFACE('',#75756,0.1) ;
#4707=SPHERICAL_SURFACE('',#75769,0.1) ;
#4708=SPHERICAL_SURFACE('',#75779,0.1) ;
#4709=SPHERICAL_SURFACE('',#75781,0.1) ;
#4710=SPHERICAL_SURFACE('',#75790,0.1) ;
#4711=SPHERICAL_SURFACE('',#75803,0.1) ;
#4712=SPHERICAL_SURFACE('',#75813,0.1) ;
#4713=SPHERICAL_SURFACE('',#75815,0.1) ;
#4714=SPHERICAL_SURFACE('',#75824,0.1) ;
#4715=SPHERICAL_SURFACE('',#75837,0.1) ;
#4716=SPHERICAL_SURFACE('',#75847,0.1) ;
#4717=SPHERICAL_SURFACE('',#75849,0.1) ;
#4718=SPHERICAL_SURFACE('',#75858,0.1) ;
#4719=SPHERICAL_SURFACE('',#75871,0.1) ;
#4720=SPHERICAL_SURFACE('',#75881,0.1) ;
#4721=SPHERICAL_SURFACE('',#75883,0.1) ;
#4722=SPHERICAL_SURFACE('',#75892,0.1) ;
#4723=SPHERICAL_SURFACE('',#75905,0.1) ;
#4724=SPHERICAL_SURFACE('',#75915,0.1) ;
#4725=SPHERICAL_SURFACE('',#75917,0.1) ;
#4726=SPHERICAL_SURFACE('',#75926,0.1) ;
#4727=SPHERICAL_SURFACE('',#75939,0.1) ;
#4728=SPHERICAL_SURFACE('',#75949,0.1) ;
#4729=SPHERICAL_SURFACE('',#75951,0.1) ;
#4730=SPHERICAL_SURFACE('',#75960,0.1) ;
#4731=SPHERICAL_SURFACE('',#75973,0.1) ;
#4732=SPHERICAL_SURFACE('',#75983,0.1) ;
#4733=SPHERICAL_SURFACE('',#75985,0.1) ;
#4734=SPHERICAL_SURFACE('',#75994,0.1) ;
#4735=SPHERICAL_SURFACE('',#76007,0.1) ;
#4736=SPHERICAL_SURFACE('',#76017,0.1) ;
#4737=SPHERICAL_SURFACE('',#76019,0.1) ;
#4738=SPHERICAL_SURFACE('',#76028,0.1) ;
#4739=SPHERICAL_SURFACE('',#76041,0.1) ;
#4740=SPHERICAL_SURFACE('',#76051,0.1) ;
#4741=SPHERICAL_SURFACE('',#76053,0.1) ;
#4742=SPHERICAL_SURFACE('',#76062,0.1) ;
#4743=SPHERICAL_SURFACE('',#76075,0.1) ;
#4744=SPHERICAL_SURFACE('',#76085,0.1) ;
#4745=SPHERICAL_SURFACE('',#76087,0.1) ;
#4746=SPHERICAL_SURFACE('',#76096,0.1) ;
#4747=SPHERICAL_SURFACE('',#76109,0.1) ;
#4748=SPHERICAL_SURFACE('',#76119,0.1) ;
#4749=SPHERICAL_SURFACE('',#76121,0.1) ;
#4750=SPHERICAL_SURFACE('',#76130,0.1) ;
#4751=SPHERICAL_SURFACE('',#76143,0.1) ;
#4752=SPHERICAL_SURFACE('',#76153,0.1) ;
#4753=SPHERICAL_SURFACE('',#76155,0.1) ;
#4754=SPHERICAL_SURFACE('',#76164,0.1) ;
#4755=SPHERICAL_SURFACE('',#76177,0.1) ;
#4756=SPHERICAL_SURFACE('',#76187,0.1) ;
#4757=SPHERICAL_SURFACE('',#76189,0.1) ;
#4758=SPHERICAL_SURFACE('',#76198,0.1) ;
#4759=SPHERICAL_SURFACE('',#76211,0.1) ;
#4760=SPHERICAL_SURFACE('',#76221,0.1) ;
#4761=SPHERICAL_SURFACE('',#76223,0.1) ;
#4762=SPHERICAL_SURFACE('',#76232,0.1) ;
#4763=SPHERICAL_SURFACE('',#76245,0.1) ;
#4764=SPHERICAL_SURFACE('',#76255,0.1) ;
#4765=SPHERICAL_SURFACE('',#76257,0.1) ;
#4766=SPHERICAL_SURFACE('',#76266,0.1) ;
#4767=SPHERICAL_SURFACE('',#76277,0.1) ;
#4768=SPHERICAL_SURFACE('',#76281,0.1) ;
#4769=SPHERICAL_SURFACE('',#76290,0.1) ;
#4770=SPHERICAL_SURFACE('',#76294,0.1) ;
#4771=SPHERICAL_SURFACE('',#76301,0.1) ;
#4772=SPHERICAL_SURFACE('',#76305,0.1) ;
#4773=SPHERICAL_SURFACE('',#76310,0.1) ;
#4774=SPHERICAL_SURFACE('',#76316,0.1) ;
#4775=SPHERICAL_SURFACE('',#76321,0.1) ;
#4776=SPHERICAL_SURFACE('',#76325,0.1) ;
#4777=SPHERICAL_SURFACE('',#76334,0.1) ;
#4778=SPHERICAL_SURFACE('',#76338,0.1) ;
#4779=SPHERICAL_SURFACE('',#76345,0.1) ;
#4780=SPHERICAL_SURFACE('',#76349,0.1) ;
#4781=SPHERICAL_SURFACE('',#76354,0.1) ;
#4782=SPHERICAL_SURFACE('',#76360,0.1) ;
#4783=SPHERICAL_SURFACE('',#76365,0.1) ;
#4784=SPHERICAL_SURFACE('',#76369,0.1) ;
#4785=SPHERICAL_SURFACE('',#76378,0.1) ;
#4786=SPHERICAL_SURFACE('',#76382,0.1) ;
#4787=SPHERICAL_SURFACE('',#76389,0.1) ;
#4788=SPHERICAL_SURFACE('',#76393,0.1) ;
#4789=SPHERICAL_SURFACE('',#76398,0.1) ;
#4790=SPHERICAL_SURFACE('',#76404,0.1) ;
#4791=SPHERICAL_SURFACE('',#76409,0.1) ;
#4792=SPHERICAL_SURFACE('',#76413,0.1) ;
#4793=SPHERICAL_SURFACE('',#76422,0.1) ;
#4794=SPHERICAL_SURFACE('',#76426,0.1) ;
#4795=SPHERICAL_SURFACE('',#76433,0.1) ;
#4796=SPHERICAL_SURFACE('',#76437,0.1) ;
#4797=SPHERICAL_SURFACE('',#76442,0.1) ;
#4798=SPHERICAL_SURFACE('',#76448,0.1) ;
#4799=SPHERICAL_SURFACE('',#76453,0.1) ;
#4800=SPHERICAL_SURFACE('',#76457,0.1) ;
#4801=SPHERICAL_SURFACE('',#76466,0.1) ;
#4802=SPHERICAL_SURFACE('',#76470,0.1) ;
#4803=SPHERICAL_SURFACE('',#76477,0.1) ;
#4804=SPHERICAL_SURFACE('',#76481,0.1) ;
#4805=SPHERICAL_SURFACE('',#76486,0.1) ;
#4806=SPHERICAL_SURFACE('',#76492,0.1) ;
#4807=SPHERICAL_SURFACE('',#76497,0.1) ;
#4808=SPHERICAL_SURFACE('',#76501,0.1) ;
#4809=SPHERICAL_SURFACE('',#76510,0.1) ;
#4810=SPHERICAL_SURFACE('',#76514,0.1) ;
#4811=SPHERICAL_SURFACE('',#76521,0.1) ;
#4812=SPHERICAL_SURFACE('',#76525,0.1) ;
#4813=SPHERICAL_SURFACE('',#76530,0.1) ;
#4814=SPHERICAL_SURFACE('',#76536,0.1) ;
#4815=SPHERICAL_SURFACE('',#76541,0.1) ;
#4816=SPHERICAL_SURFACE('',#76545,0.1) ;
#4817=SPHERICAL_SURFACE('',#76554,0.1) ;
#4818=SPHERICAL_SURFACE('',#76558,0.1) ;
#4819=SPHERICAL_SURFACE('',#76565,0.1) ;
#4820=SPHERICAL_SURFACE('',#76569,0.1) ;
#4821=SPHERICAL_SURFACE('',#76574,0.1) ;
#4822=SPHERICAL_SURFACE('',#76580,0.1) ;
#4823=SPHERICAL_SURFACE('',#76585,0.1) ;
#4824=SPHERICAL_SURFACE('',#76589,0.1) ;
#4825=SPHERICAL_SURFACE('',#76598,0.1) ;
#4826=SPHERICAL_SURFACE('',#76602,0.1) ;
#4827=SPHERICAL_SURFACE('',#76609,0.1) ;
#4828=SPHERICAL_SURFACE('',#76613,0.1) ;
#4829=SPHERICAL_SURFACE('',#76618,0.1) ;
#4830=SPHERICAL_SURFACE('',#76624,0.1) ;
#4831=SPHERICAL_SURFACE('',#76629,0.1) ;
#4832=SPHERICAL_SURFACE('',#76633,0.1) ;
#4833=SPHERICAL_SURFACE('',#76642,0.1) ;
#4834=SPHERICAL_SURFACE('',#76646,0.1) ;
#4835=SPHERICAL_SURFACE('',#76653,0.1) ;
#4836=SPHERICAL_SURFACE('',#76657,0.1) ;
#4837=SPHERICAL_SURFACE('',#76662,0.1) ;
#4838=SPHERICAL_SURFACE('',#76668,0.1) ;
#4973=ELLIPSE('',#71881,0.141421356226833,0.0999999999854714) ;
#4974=ELLIPSE('',#71898,0.141421356205715,0.0999999999561054) ;
#4975=ELLIPSE('',#71915,0.141421356206211,0.0999999999568741) ;
#4976=ELLIPSE('',#71932,0.14142135619891,0.0999999999469108) ;
#4977=ELLIPSE('',#71949,0.14142135620716,0.0999999999583245) ;
#4978=ELLIPSE('',#71966,0.141421356264666,0.100000000037862) ;
#4979=ELLIPSE('',#71983,0.141421356235352,0.0999999999972513) ;
#4980=ELLIPSE('',#72000,0.141421356240128,0.100000000003844) ;
#4981=ELLIPSE('',#72062,0.141421356242718,0.100000000007393) ;
#4982=ELLIPSE('',#72111,0.141421356244824,0.100000000010334) ;
#5031=FACE_BOUND('',#22487,.T.) ;
#5032=FACE_BOUND('',#22488,.T.) ;
#5033=FACE_BOUND('',#22489,.T.) ;
#5034=FACE_BOUND('',#22490,.T.) ;
#5035=FACE_BOUND('',#22491,.T.) ;
#5036=FACE_BOUND('',#22492,.T.) ;
#5037=FACE_BOUND('',#22493,.T.) ;
#5038=FACE_BOUND('',#22494,.T.) ;
#5039=FACE_BOUND('',#22495,.T.) ;
#5040=FACE_BOUND('',#22496,.T.) ;
#5041=FACE_BOUND('',#22533,.T.) ;
#5042=FACE_BOUND('',#22535,.T.) ;
#5043=FACE_BOUND('',#22822,.T.) ;
#5044=FACE_BOUND('',#22851,.T.) ;
#5045=FACE_BOUND('',#22880,.T.) ;
#5046=FACE_BOUND('',#22909,.T.) ;
#5047=FACE_BOUND('',#22938,.T.) ;
#5048=FACE_BOUND('',#22967,.T.) ;
#5049=FACE_BOUND('',#22996,.T.) ;
#5050=FACE_BOUND('',#23025,.T.) ;
#5051=FACE_BOUND('',#23054,.T.) ;
#5052=FACE_BOUND('',#23056,.T.) ;
#5053=FACE_BOUND('',#23058,.T.) ;
#5054=FACE_BOUND('',#23060,.T.) ;
#5055=FACE_BOUND('',#23062,.T.) ;
#5056=FACE_BOUND('',#23064,.T.) ;
#5057=FACE_BOUND('',#23066,.T.) ;
#5058=FACE_BOUND('',#23068,.T.) ;
#5059=FACE_BOUND('',#23070,.T.) ;
#5060=FACE_BOUND('',#23072,.T.) ;
#5483=PLANE('',#72117) ;
#5484=PLANE('',#72122) ;
#5485=PLANE('',#72127) ;
#5486=PLANE('',#72132) ;
#5487=PLANE('',#72137) ;
#5488=PLANE('',#72142) ;
#5489=PLANE('',#72147) ;
#5490=PLANE('',#72152) ;
#5491=PLANE('',#72157) ;
#5492=PLANE('',#72162) ;
#5493=PLANE('',#72164) ;
#5494=PLANE('',#72166) ;
#5495=PLANE('',#72168) ;
#5496=PLANE('',#72170) ;
#5497=PLANE('',#72172) ;
#5498=PLANE('',#72174) ;
#5499=PLANE('',#72176) ;
#5500=PLANE('',#72178) ;
#5501=PLANE('',#72180) ;
#5502=PLANE('',#72182) ;
#5503=PLANE('',#72184) ;
#5504=PLANE('',#72186) ;
#5505=PLANE('',#72188) ;
#5506=PLANE('',#72190) ;
#5507=PLANE('',#72192) ;
#5508=PLANE('',#72194) ;
#5509=PLANE('',#72196) ;
#5510=PLANE('',#72225) ;
#5511=PLANE('',#72230) ;
#5512=PLANE('',#72232) ;
#5513=PLANE('',#72240) ;
#5514=PLANE('',#72264) ;
#5515=PLANE('',#72288) ;
#5516=PLANE('',#72292) ;
#5517=PLANE('',#72296) ;
#5518=PLANE('',#72300) ;
#5519=PLANE('',#72304) ;
#5520=PLANE('',#72308) ;
#5521=PLANE('',#72409) ;
#5522=PLANE('',#72412) ;
#5523=PLANE('',#72415) ;
#5524=PLANE('',#72418) ;
#5525=PLANE('',#72419) ;
#5526=PLANE('',#72420) ;
#5527=PLANE('',#72421) ;
#5528=PLANE('',#72422) ;
#5529=PLANE('',#72426) ;
#5530=PLANE('',#72430) ;
#5531=PLANE('',#72434) ;
#5532=PLANE('',#72437) ;
#5533=PLANE('',#72438) ;
#5534=PLANE('',#72442) ;
#5535=PLANE('',#72446) ;
#5536=PLANE('',#72450) ;
#5537=PLANE('',#72454) ;
#5538=PLANE('',#72458) ;
#5539=PLANE('',#72468) ;
#5540=PLANE('',#72472) ;
#5541=PLANE('',#72476) ;
#5542=PLANE('',#72477) ;
#5543=PLANE('',#72483) ;
#5544=PLANE('',#72758) ;
#5545=PLANE('',#72759) ;
#5546=PLANE('',#72760) ;
#5547=PLANE('',#72761) ;
#5548=PLANE('',#72762) ;
#5549=PLANE('',#72763) ;
#5550=PLANE('',#72766) ;
#5551=PLANE('',#72775) ;
#5552=PLANE('',#72776) ;
#5553=PLANE('',#72777) ;
#5554=PLANE('',#72778) ;
#5555=PLANE('',#72779) ;
#5556=PLANE('',#72780) ;
#5557=PLANE('',#72781) ;
#5558=PLANE('',#72782) ;
#5559=PLANE('',#72783) ;
#5560=PLANE('',#72784) ;
#5561=PLANE('',#72785) ;
#5562=PLANE('',#72898) ;
#5563=PLANE('',#72901) ;
#5564=PLANE('',#72904) ;
#5565=PLANE('',#72907) ;
#5566=PLANE('',#72910) ;
#5567=PLANE('',#72913) ;
#5568=PLANE('',#72916) ;
#5569=PLANE('',#72919) ;
#5570=PLANE('',#72922) ;
#5571=PLANE('',#72925) ;
#5572=PLANE('',#72926) ;
#5573=PLANE('',#72927) ;
#5574=PLANE('',#72928) ;
#5575=PLANE('',#72929) ;
#5576=PLANE('',#72930) ;
#5577=PLANE('',#72931) ;
#5578=PLANE('',#72932) ;
#5579=PLANE('',#72933) ;
#5580=PLANE('',#72934) ;
#5581=PLANE('',#72935) ;
#5582=PLANE('',#72936) ;
#5583=PLANE('',#72937) ;
#5584=PLANE('',#72938) ;
#5585=PLANE('',#72939) ;
#5586=PLANE('',#72940) ;
#5587=PLANE('',#72941) ;
#5588=PLANE('',#72942) ;
#5589=PLANE('',#72943) ;
#5590=PLANE('',#72944) ;
#5591=PLANE('',#72945) ;
#5592=PLANE('',#72946) ;
#5593=PLANE('',#72947) ;
#5594=PLANE('',#72948) ;
#5595=PLANE('',#72949) ;
#5596=PLANE('',#72950) ;
#5597=PLANE('',#72951) ;
#5598=PLANE('',#72952) ;
#5599=PLANE('',#72953) ;
#5600=PLANE('',#72954) ;
#5601=PLANE('',#72955) ;
#5602=PLANE('',#72956) ;
#5603=PLANE('',#72957) ;
#5604=PLANE('',#72958) ;
#5605=PLANE('',#72959) ;
#5606=PLANE('',#72960) ;
#5607=PLANE('',#72961) ;
#5608=PLANE('',#72962) ;
#5609=PLANE('',#72963) ;
#5610=PLANE('',#72964) ;
#5611=PLANE('',#72965) ;
#5612=PLANE('',#72966) ;
#5613=PLANE('',#72967) ;
#5614=PLANE('',#72968) ;
#5615=PLANE('',#72969) ;
#5616=PLANE('',#72973) ;
#5617=PLANE('',#72977) ;
#5618=PLANE('',#72981) ;
#5619=PLANE('',#72984) ;
#5620=PLANE('',#72985) ;
#5621=PLANE('',#72989) ;
#5622=PLANE('',#72993) ;
#5623=PLANE('',#72997) ;
#5624=PLANE('',#73001) ;
#5625=PLANE('',#73005) ;
#5626=PLANE('',#73015) ;
#5627=PLANE('',#73019) ;
#5628=PLANE('',#73023) ;
#5629=PLANE('',#73024) ;
#5630=PLANE('',#73033) ;
#5631=PLANE('',#73037) ;
#5632=PLANE('',#73041) ;
#5633=PLANE('',#73044) ;
#5634=PLANE('',#73045) ;
#5635=PLANE('',#73049) ;
#5636=PLANE('',#73053) ;
#5637=PLANE('',#73057) ;
#5638=PLANE('',#73061) ;
#5639=PLANE('',#73065) ;
#5640=PLANE('',#73075) ;
#5641=PLANE('',#73079) ;
#5642=PLANE('',#73083) ;
#5643=PLANE('',#73084) ;
#5644=PLANE('',#73093) ;
#5645=PLANE('',#73097) ;
#5646=PLANE('',#73101) ;
#5647=PLANE('',#73104) ;
#5648=PLANE('',#73105) ;
#5649=PLANE('',#73109) ;
#5650=PLANE('',#73113) ;
#5651=PLANE('',#73117) ;
#5652=PLANE('',#73121) ;
#5653=PLANE('',#73125) ;
#5654=PLANE('',#73135) ;
#5655=PLANE('',#73139) ;
#5656=PLANE('',#73143) ;
#5657=PLANE('',#73144) ;
#5658=PLANE('',#73153) ;
#5659=PLANE('',#73157) ;
#5660=PLANE('',#73161) ;
#5661=PLANE('',#73164) ;
#5662=PLANE('',#73165) ;
#5663=PLANE('',#73169) ;
#5664=PLANE('',#73173) ;
#5665=PLANE('',#73177) ;
#5666=PLANE('',#73181) ;
#5667=PLANE('',#73185) ;
#5668=PLANE('',#73195) ;
#5669=PLANE('',#73199) ;
#5670=PLANE('',#73203) ;
#5671=PLANE('',#73204) ;
#5672=PLANE('',#73213) ;
#5673=PLANE('',#73217) ;
#5674=PLANE('',#73221) ;
#5675=PLANE('',#73224) ;
#5676=PLANE('',#73225) ;
#5677=PLANE('',#73229) ;
#5678=PLANE('',#73233) ;
#5679=PLANE('',#73237) ;
#5680=PLANE('',#73241) ;
#5681=PLANE('',#73245) ;
#5682=PLANE('',#73255) ;
#5683=PLANE('',#73259) ;
#5684=PLANE('',#73263) ;
#5685=PLANE('',#73264) ;
#5686=PLANE('',#73273) ;
#5687=PLANE('',#73277) ;
#5688=PLANE('',#73281) ;
#5689=PLANE('',#73284) ;
#5690=PLANE('',#73285) ;
#5691=PLANE('',#73289) ;
#5692=PLANE('',#73293) ;
#5693=PLANE('',#73297) ;
#5694=PLANE('',#73301) ;
#5695=PLANE('',#73305) ;
#5696=PLANE('',#73315) ;
#5697=PLANE('',#73319) ;
#5698=PLANE('',#73323) ;
#5699=PLANE('',#73324) ;
#5700=PLANE('',#73333) ;
#5701=PLANE('',#73337) ;
#5702=PLANE('',#73341) ;
#5703=PLANE('',#73344) ;
#5704=PLANE('',#73345) ;
#5705=PLANE('',#73349) ;
#5706=PLANE('',#73353) ;
#5707=PLANE('',#73357) ;
#5708=PLANE('',#73361) ;
#5709=PLANE('',#73365) ;
#5710=PLANE('',#73375) ;
#5711=PLANE('',#73379) ;
#5712=PLANE('',#73383) ;
#5713=PLANE('',#73384) ;
#5714=PLANE('',#73393) ;
#5715=PLANE('',#73397) ;
#5716=PLANE('',#73401) ;
#5717=PLANE('',#73404) ;
#5718=PLANE('',#73405) ;
#5719=PLANE('',#73409) ;
#5720=PLANE('',#73413) ;
#5721=PLANE('',#73417) ;
#5722=PLANE('',#73421) ;
#5723=PLANE('',#73425) ;
#5724=PLANE('',#73435) ;
#5725=PLANE('',#73439) ;
#5726=PLANE('',#73443) ;
#5727=PLANE('',#73444) ;
#5728=PLANE('',#73453) ;
#5729=PLANE('',#73457) ;
#5730=PLANE('',#73461) ;
#5731=PLANE('',#73464) ;
#5732=PLANE('',#73465) ;
#5733=PLANE('',#73469) ;
#5734=PLANE('',#73473) ;
#5735=PLANE('',#73477) ;
#5736=PLANE('',#73481) ;
#5737=PLANE('',#73485) ;
#5738=PLANE('',#73495) ;
#5739=PLANE('',#73499) ;
#5740=PLANE('',#73503) ;
#5741=PLANE('',#73504) ;
#5742=PLANE('',#73510) ;
#5743=PLANE('',#73515) ;
#5744=PLANE('',#73520) ;
#5745=PLANE('',#73525) ;
#5746=PLANE('',#73530) ;
#5747=PLANE('',#73535) ;
#5748=PLANE('',#73540) ;
#5749=PLANE('',#73545) ;
#5750=PLANE('',#73550) ;
#5751=PLANE('',#75409) ;
#5752=PLANE('',#75410) ;
#5753=PLANE('',#75411) ;
#5754=PLANE('',#75412) ;
#5755=PLANE('',#75413) ;
#5756=PLANE('',#75414) ;
#5757=PLANE('',#75417) ;
#5758=PLANE('',#75426) ;
#5759=PLANE('',#75427) ;
#5760=PLANE('',#75428) ;
#5761=PLANE('',#75429) ;
#5762=PLANE('',#75430) ;
#5763=PLANE('',#75431) ;
#5764=PLANE('',#75432) ;
#5765=PLANE('',#75433) ;
#5766=PLANE('',#75434) ;
#5767=PLANE('',#75435) ;
#5768=PLANE('',#75436) ;
#5769=PLANE('',#75437) ;
#5770=PLANE('',#75438) ;
#5771=PLANE('',#75441) ;
#5772=PLANE('',#75450) ;
#5773=PLANE('',#75451) ;
#5774=PLANE('',#75452) ;
#5775=PLANE('',#75453) ;
#5776=PLANE('',#75454) ;
#5777=PLANE('',#75455) ;
#5778=PLANE('',#75456) ;
#5779=PLANE('',#75457) ;
#5780=PLANE('',#75458) ;
#5781=PLANE('',#75459) ;
#5782=PLANE('',#75460) ;
#5783=PLANE('',#75461) ;
#5784=PLANE('',#75462) ;
#5785=PLANE('',#75465) ;
#5786=PLANE('',#75474) ;
#5787=PLANE('',#75475) ;
#5788=PLANE('',#75476) ;
#5789=PLANE('',#75477) ;
#5790=PLANE('',#75478) ;
#5791=PLANE('',#75479) ;
#5792=PLANE('',#75480) ;
#5793=PLANE('',#75481) ;
#5794=PLANE('',#75482) ;
#5795=PLANE('',#75483) ;
#5796=PLANE('',#75484) ;
#5797=PLANE('',#75485) ;
#5798=PLANE('',#75486) ;
#5799=PLANE('',#75489) ;
#5800=PLANE('',#75498) ;
#5801=PLANE('',#75499) ;
#5802=PLANE('',#75500) ;
#5803=PLANE('',#75501) ;
#5804=PLANE('',#75502) ;
#5805=PLANE('',#75503) ;
#5806=PLANE('',#75504) ;
#5807=PLANE('',#75505) ;
#5808=PLANE('',#75506) ;
#5809=PLANE('',#75507) ;
#5810=PLANE('',#75508) ;
#5811=PLANE('',#75509) ;
#5812=PLANE('',#75510) ;
#5813=PLANE('',#75513) ;
#5814=PLANE('',#75522) ;
#5815=PLANE('',#75523) ;
#5816=PLANE('',#75524) ;
#5817=PLANE('',#75525) ;
#5818=PLANE('',#75526) ;
#5819=PLANE('',#75527) ;
#5820=PLANE('',#75528) ;
#5821=PLANE('',#75529) ;
#5822=PLANE('',#75530) ;
#5823=PLANE('',#75531) ;
#5824=PLANE('',#75532) ;
#5825=PLANE('',#75533) ;
#5826=PLANE('',#75534) ;
#5827=PLANE('',#75537) ;
#5828=PLANE('',#75546) ;
#5829=PLANE('',#75547) ;
#5830=PLANE('',#75548) ;
#5831=PLANE('',#75549) ;
#5832=PLANE('',#75550) ;
#5833=PLANE('',#75551) ;
#5834=PLANE('',#75552) ;
#5835=PLANE('',#75553) ;
#5836=PLANE('',#75554) ;
#5837=PLANE('',#75555) ;
#5838=PLANE('',#75556) ;
#5839=PLANE('',#75557) ;
#5840=PLANE('',#75558) ;
#5841=PLANE('',#75561) ;
#5842=PLANE('',#75570) ;
#5843=PLANE('',#75571) ;
#5844=PLANE('',#75572) ;
#5845=PLANE('',#75573) ;
#5846=PLANE('',#75574) ;
#5847=PLANE('',#75575) ;
#5848=PLANE('',#75576) ;
#5849=PLANE('',#75577) ;
#5850=PLANE('',#75578) ;
#5851=PLANE('',#75579) ;
#5852=PLANE('',#75580) ;
#5853=PLANE('',#75581) ;
#5854=PLANE('',#75582) ;
#5855=PLANE('',#75585) ;
#5856=PLANE('',#75594) ;
#5857=PLANE('',#75595) ;
#5858=PLANE('',#75596) ;
#5859=PLANE('',#75597) ;
#5860=PLANE('',#75598) ;
#5861=PLANE('',#75599) ;
#5862=PLANE('',#75600) ;
#5863=PLANE('',#75601) ;
#5864=PLANE('',#75602) ;
#5865=PLANE('',#75603) ;
#5866=PLANE('',#75604) ;
#5867=PLANE('',#75605) ;
#5868=PLANE('',#75606) ;
#5869=PLANE('',#75609) ;
#5870=PLANE('',#75618) ;
#5871=PLANE('',#75619) ;
#5872=PLANE('',#75620) ;
#5873=PLANE('',#75621) ;
#5874=PLANE('',#75622) ;
#5875=PLANE('',#75623) ;
#5876=PLANE('',#75624) ;
#5877=PLANE('',#75625) ;
#5878=PLANE('',#75626) ;
#5879=PLANE('',#75627) ;
#5880=PLANE('',#75628) ;
#5881=PLANE('',#75629) ;
#5882=PLANE('',#75630) ;
#5883=PLANE('',#75631) ;
#5884=PLANE('',#75632) ;
#5885=PLANE('',#75633) ;
#5886=PLANE('',#75634) ;
#5887=PLANE('',#75635) ;
#5888=PLANE('',#75636) ;
#5889=PLANE('',#75637) ;
#5890=PLANE('',#75638) ;
#5891=PLANE('',#75639) ;
#5892=PLANE('',#75640) ;
#5893=PLANE('',#75641) ;
#5894=PLANE('',#75642) ;
#5895=PLANE('',#75643) ;
#5896=PLANE('',#75644) ;
#5897=PLANE('',#75645) ;
#5898=PLANE('',#75646) ;
#5899=PLANE('',#75647) ;
#5900=PLANE('',#75648) ;
#5901=PLANE('',#75649) ;
#5902=PLANE('',#75650) ;
#5903=PLANE('',#75651) ;
#5904=PLANE('',#75652) ;
#5905=PLANE('',#75653) ;
#5906=PLANE('',#75654) ;
#5907=PLANE('',#75655) ;
#5908=PLANE('',#75656) ;
#5909=PLANE('',#75657) ;
#5910=PLANE('',#75658) ;
#5911=PLANE('',#75659) ;
#5912=PLANE('',#75660) ;
#6802=CYLINDRICAL_SURFACE('',#71880,0.1) ;
#6803=CYLINDRICAL_SURFACE('',#71897,0.1) ;
#6804=CYLINDRICAL_SURFACE('',#71914,0.1) ;
#6805=CYLINDRICAL_SURFACE('',#71931,0.1) ;
#6806=CYLINDRICAL_SURFACE('',#71948,0.1) ;
#6807=CYLINDRICAL_SURFACE('',#71965,0.1) ;
#6808=CYLINDRICAL_SURFACE('',#71982,0.1) ;
#6809=CYLINDRICAL_SURFACE('',#71999,0.1) ;
#6810=CYLINDRICAL_SURFACE('',#72061,0.1) ;
#6811=CYLINDRICAL_SURFACE('',#72065,1.) ;
#6812=CYLINDRICAL_SURFACE('',#72066,1.) ;
#6813=CYLINDRICAL_SURFACE('',#72067,1.) ;
#6814=CYLINDRICAL_SURFACE('',#72068,1.) ;
#6815=CYLINDRICAL_SURFACE('',#72069,1.) ;
#6816=CYLINDRICAL_SURFACE('',#72070,0.999999999999999) ;
#6817=CYLINDRICAL_SURFACE('',#72071,0.999999999999999) ;
#6818=CYLINDRICAL_SURFACE('',#72072,1.) ;
#6819=CYLINDRICAL_SURFACE('',#72073,1.) ;
#6820=CYLINDRICAL_SURFACE('',#72074,0.1) ;
#6821=CYLINDRICAL_SURFACE('',#72076,0.100000000000001) ;
#6822=CYLINDRICAL_SURFACE('',#72078,0.100000000000001) ;
#6823=CYLINDRICAL_SURFACE('',#72080,0.0999999999999994) ;
#6824=CYLINDRICAL_SURFACE('',#72082,0.0999999999999994) ;
#6825=CYLINDRICAL_SURFACE('',#72084,0.0999999999999994) ;
#6826=CYLINDRICAL_SURFACE('',#72086,0.0999999999999994) ;
#6827=CYLINDRICAL_SURFACE('',#72088,0.100000000000003) ;
#6828=CYLINDRICAL_SURFACE('',#72090,0.100000000000003) ;
#6829=CYLINDRICAL_SURFACE('',#72110,0.1) ;
#6830=CYLINDRICAL_SURFACE('',#72114,1.) ;
#6831=CYLINDRICAL_SURFACE('',#72115,0.1) ;
#6832=CYLINDRICAL_SURFACE('',#72198,0.1) ;
#6833=CYLINDRICAL_SURFACE('',#72201,0.1) ;
#6834=CYLINDRICAL_SURFACE('',#72204,0.1) ;
#6835=CYLINDRICAL_SURFACE('',#72207,0.1) ;
#6836=CYLINDRICAL_SURFACE('',#72210,0.1) ;
#6837=CYLINDRICAL_SURFACE('',#72213,0.1) ;
#6838=CYLINDRICAL_SURFACE('',#72216,0.1) ;
#6839=CYLINDRICAL_SURFACE('',#72219,0.1) ;
#6840=CYLINDRICAL_SURFACE('',#72222,0.1) ;
#6841=CYLINDRICAL_SURFACE('',#72234,0.1) ;
#6842=CYLINDRICAL_SURFACE('',#72237,0.0999999999999994) ;
#6843=CYLINDRICAL_SURFACE('',#72261,0.1) ;
#6844=CYLINDRICAL_SURFACE('',#72285,0.1) ;
#6845=CYLINDRICAL_SURFACE('',#72289,0.1) ;
#6846=CYLINDRICAL_SURFACE('',#72293,0.1) ;
#6847=CYLINDRICAL_SURFACE('',#72297,0.100000000000001) ;
#6848=CYLINDRICAL_SURFACE('',#72301,0.1) ;
#6849=CYLINDRICAL_SURFACE('',#72305,0.0999999999999994) ;
#6850=CYLINDRICAL_SURFACE('',#72423,0.1) ;
#6851=CYLINDRICAL_SURFACE('',#72427,0.1) ;
#6852=CYLINDRICAL_SURFACE('',#72431,0.0999999999999994) ;
#6853=CYLINDRICAL_SURFACE('',#72435,0.1) ;
#6854=CYLINDRICAL_SURFACE('',#72439,0.1) ;
#6855=CYLINDRICAL_SURFACE('',#72443,0.1) ;
#6856=CYLINDRICAL_SURFACE('',#72447,0.1) ;
#6857=CYLINDRICAL_SURFACE('',#72451,0.1) ;
#6858=CYLINDRICAL_SURFACE('',#72455,0.1) ;
#6859=CYLINDRICAL_SURFACE('',#72459,0.1) ;
#6860=CYLINDRICAL_SURFACE('',#72462,1.65625) ;
#6861=CYLINDRICAL_SURFACE('',#72465,0.1) ;
#6862=CYLINDRICAL_SURFACE('',#72469,0.1) ;
#6863=CYLINDRICAL_SURFACE('',#72473,0.1) ;
#6864=CYLINDRICAL_SURFACE('',#72488,0.1) ;
#6865=CYLINDRICAL_SURFACE('',#72491,0.1) ;
#6866=CYLINDRICAL_SURFACE('',#72502,0.1) ;
#6867=CYLINDRICAL_SURFACE('',#72504,0.1) ;
#6868=CYLINDRICAL_SURFACE('',#72506,0.1) ;
#6869=CYLINDRICAL_SURFACE('',#72508,0.1) ;
#6870=CYLINDRICAL_SURFACE('',#72510,0.1) ;
#6871=CYLINDRICAL_SURFACE('',#72512,0.1) ;
#6872=CYLINDRICAL_SURFACE('',#72523,0.1) ;
#6873=CYLINDRICAL_SURFACE('',#72525,0.0999999999999998) ;
#6874=CYLINDRICAL_SURFACE('',#72527,0.1) ;
#6875=CYLINDRICAL_SURFACE('',#72529,0.1) ;
#6876=CYLINDRICAL_SURFACE('',#72531,0.1) ;
#6877=CYLINDRICAL_SURFACE('',#72541,0.1) ;
#6878=CYLINDRICAL_SURFACE('',#72548,0.1) ;
#6879=CYLINDRICAL_SURFACE('',#72550,0.1) ;
#6880=CYLINDRICAL_SURFACE('',#72552,0.1) ;
#6881=CYLINDRICAL_SURFACE('',#72556,0.1) ;
#6882=CYLINDRICAL_SURFACE('',#72558,0.1) ;
#6883=CYLINDRICAL_SURFACE('',#72560,0.0999999999999998) ;
#6884=CYLINDRICAL_SURFACE('',#72567,0.1) ;
#6885=CYLINDRICAL_SURFACE('',#72574,0.1) ;
#6886=CYLINDRICAL_SURFACE('',#72576,0.1) ;
#6887=CYLINDRICAL_SURFACE('',#72580,0.1) ;
#6888=CYLINDRICAL_SURFACE('',#72583,0.1) ;
#6889=CYLINDRICAL_SURFACE('',#72585,0.1) ;
#6890=CYLINDRICAL_SURFACE('',#72591,0.100000000000003) ;
#6891=CYLINDRICAL_SURFACE('',#72593,0.100000000000003) ;
#6892=CYLINDRICAL_SURFACE('',#72599,0.1) ;
#6893=CYLINDRICAL_SURFACE('',#72601,0.1) ;
#6894=CYLINDRICAL_SURFACE('',#72607,0.1) ;
#6895=CYLINDRICAL_SURFACE('',#72609,0.1) ;
#6896=CYLINDRICAL_SURFACE('',#72615,0.100000000000003) ;
#6897=CYLINDRICAL_SURFACE('',#72617,0.100000000000003) ;
#6898=CYLINDRICAL_SURFACE('',#72623,0.0999999999999998) ;
#6899=CYLINDRICAL_SURFACE('',#72625,0.0999999999999998) ;
#6900=CYLINDRICAL_SURFACE('',#72631,0.1) ;
#6901=CYLINDRICAL_SURFACE('',#72633,0.1) ;
#6902=CYLINDRICAL_SURFACE('',#72639,0.1) ;
#6903=CYLINDRICAL_SURFACE('',#72641,0.1) ;
#6904=CYLINDRICAL_SURFACE('',#72647,0.0999999999999998) ;
#6905=CYLINDRICAL_SURFACE('',#72649,0.0999999999999998) ;
#6906=CYLINDRICAL_SURFACE('',#72652,0.1) ;
#6907=CYLINDRICAL_SURFACE('',#72659,0.1) ;
#6908=CYLINDRICAL_SURFACE('',#72661,0.1) ;
#6909=CYLINDRICAL_SURFACE('',#72667,0.1) ;
#6910=CYLINDRICAL_SURFACE('',#72669,0.1) ;
#6911=CYLINDRICAL_SURFACE('',#72675,0.0999999999999999) ;
#6912=CYLINDRICAL_SURFACE('',#72683,0.1) ;
#6913=CYLINDRICAL_SURFACE('',#72684,0.1) ;
#6914=CYLINDRICAL_SURFACE('',#72688,0.1) ;
#6915=CYLINDRICAL_SURFACE('',#72690,0.1) ;
#6916=CYLINDRICAL_SURFACE('',#72696,0.0999999999999998) ;
#6917=CYLINDRICAL_SURFACE('',#72698,0.1) ;
#6918=CYLINDRICAL_SURFACE('',#72704,0.1) ;
#6919=CYLINDRICAL_SURFACE('',#72705,0.1) ;
#6920=CYLINDRICAL_SURFACE('',#72712,0.0999999999999994) ;
#6921=CYLINDRICAL_SURFACE('',#72714,0.1) ;
#6922=CYLINDRICAL_SURFACE('',#72720,0.1) ;
#6923=CYLINDRICAL_SURFACE('',#72721,0.1) ;
#6924=CYLINDRICAL_SURFACE('',#72725,0.1) ;
#6925=CYLINDRICAL_SURFACE('',#72727,0.0999999999999994) ;
#6926=CYLINDRICAL_SURFACE('',#72733,0.1) ;
#6927=CYLINDRICAL_SURFACE('',#72741,0.0999999999999998) ;
#6928=CYLINDRICAL_SURFACE('',#72743,0.0999999999999994) ;
#6929=CYLINDRICAL_SURFACE('',#72749,0.1) ;
#6930=CYLINDRICAL_SURFACE('',#72751,0.1) ;
#6931=CYLINDRICAL_SURFACE('',#72757,0.1) ;
#6932=CYLINDRICAL_SURFACE('',#72769,1.) ;
#6933=CYLINDRICAL_SURFACE('',#72772,0.2) ;
#6934=CYLINDRICAL_SURFACE('',#72786,0.1) ;
#6935=CYLINDRICAL_SURFACE('',#72789,0.1) ;
#6936=CYLINDRICAL_SURFACE('',#72795,0.1) ;
#6937=CYLINDRICAL_SURFACE('',#72798,0.1) ;
#6938=CYLINDRICAL_SURFACE('',#72800,0.1) ;
#6939=CYLINDRICAL_SURFACE('',#72807,0.1) ;
#6940=CYLINDRICAL_SURFACE('',#72809,0.1) ;
#6941=CYLINDRICAL_SURFACE('',#72811,0.1) ;
#6942=CYLINDRICAL_SURFACE('',#72815,0.1) ;
#6943=CYLINDRICAL_SURFACE('',#72818,0.1) ;
#6944=CYLINDRICAL_SURFACE('',#72820,0.1) ;
#6945=CYLINDRICAL_SURFACE('',#72823,0.1) ;
#6946=CYLINDRICAL_SURFACE('',#72829,0.1) ;
#6947=CYLINDRICAL_SURFACE('',#72832,0.1) ;
#6948=CYLINDRICAL_SURFACE('',#72834,0.1) ;
#6949=CYLINDRICAL_SURFACE('',#72841,0.1) ;
#6950=CYLINDRICAL_SURFACE('',#72843,0.1) ;
#6951=CYLINDRICAL_SURFACE('',#72845,0.1) ;
#6952=CYLINDRICAL_SURFACE('',#72849,0.1) ;
#6953=CYLINDRICAL_SURFACE('',#72852,0.1) ;
#6954=CYLINDRICAL_SURFACE('',#72856,0.1) ;
#6955=CYLINDRICAL_SURFACE('',#72860,0.1) ;
#6956=CYLINDRICAL_SURFACE('',#72864,0.1) ;
#6957=CYLINDRICAL_SURFACE('',#72869,0.1) ;
#6958=CYLINDRICAL_SURFACE('',#72873,0.1) ;
#6959=CYLINDRICAL_SURFACE('',#72877,0.1) ;
#6960=CYLINDRICAL_SURFACE('',#72880,0.1) ;
#6961=CYLINDRICAL_SURFACE('',#72884,0.1) ;
#6962=CYLINDRICAL_SURFACE('',#72888,0.1) ;
#6963=CYLINDRICAL_SURFACE('',#72889,0.1) ;
#6964=CYLINDRICAL_SURFACE('',#72893,0.1) ;
#6965=CYLINDRICAL_SURFACE('',#72895,0.1) ;
#6966=CYLINDRICAL_SURFACE('',#72970,0.100000000000003) ;
#6967=CYLINDRICAL_SURFACE('',#72974,0.100000000000003) ;
#6968=CYLINDRICAL_SURFACE('',#72978,0.0999999999999959) ;
#6969=CYLINDRICAL_SURFACE('',#72982,0.100000000000003) ;
#6970=CYLINDRICAL_SURFACE('',#72986,0.100000000000003) ;
#6971=CYLINDRICAL_SURFACE('',#72990,0.100000000000003) ;
#6972=CYLINDRICAL_SURFACE('',#72994,0.100000000000003) ;
#6973=CYLINDRICAL_SURFACE('',#72998,0.100000000000003) ;
#6974=CYLINDRICAL_SURFACE('',#73002,0.100000000000003) ;
#6975=CYLINDRICAL_SURFACE('',#73006,0.100000000000003) ;
#6976=CYLINDRICAL_SURFACE('',#73009,1.65625) ;
#6977=CYLINDRICAL_SURFACE('',#73012,0.100000000000003) ;
#6978=CYLINDRICAL_SURFACE('',#73016,0.100000000000003) ;
#6979=CYLINDRICAL_SURFACE('',#73020,0.100000000000003) ;
#6980=CYLINDRICAL_SURFACE('',#73030,0.0999999999999994) ;
#6981=CYLINDRICAL_SURFACE('',#73034,0.0999999999999994) ;
#6982=CYLINDRICAL_SURFACE('',#73038,0.0999999999999994) ;
#6983=CYLINDRICAL_SURFACE('',#73042,0.0999999999999994) ;
#6984=CYLINDRICAL_SURFACE('',#73046,0.100000000000003) ;
#6985=CYLINDRICAL_SURFACE('',#73050,0.0999999999999994) ;
#6986=CYLINDRICAL_SURFACE('',#73054,0.0999999999999994) ;
#6987=CYLINDRICAL_SURFACE('',#73058,0.100000000000003) ;
#6988=CYLINDRICAL_SURFACE('',#73062,0.100000000000003) ;
#6989=CYLINDRICAL_SURFACE('',#73066,0.100000000000003) ;
#6990=CYLINDRICAL_SURFACE('',#73069,1.65625) ;
#6991=CYLINDRICAL_SURFACE('',#73072,0.0999999999999994) ;
#6992=CYLINDRICAL_SURFACE('',#73076,0.0999999999999994) ;
#6993=CYLINDRICAL_SURFACE('',#73080,0.0999999999999994) ;
#6994=CYLINDRICAL_SURFACE('',#73090,0.0999999999999994) ;
#6995=CYLINDRICAL_SURFACE('',#73094,0.0999999999999994) ;
#6996=CYLINDRICAL_SURFACE('',#73098,0.0999999999999994) ;
#6997=CYLINDRICAL_SURFACE('',#73102,0.0999999999999994) ;
#6998=CYLINDRICAL_SURFACE('',#73106,0.0999999999999994) ;
#6999=CYLINDRICAL_SURFACE('',#73110,0.0999999999999994) ;
#7000=CYLINDRICAL_SURFACE('',#73114,0.0999999999999994) ;
#7001=CYLINDRICAL_SURFACE('',#73118,0.0999999999999994) ;
#7002=CYLINDRICAL_SURFACE('',#73122,0.0999999999999994) ;
#7003=CYLINDRICAL_SURFACE('',#73126,0.0999999999999994) ;
#7004=CYLINDRICAL_SURFACE('',#73129,1.65625) ;
#7005=CYLINDRICAL_SURFACE('',#73132,0.0999999999999994) ;
#7006=CYLINDRICAL_SURFACE('',#73136,0.0999999999999994) ;
#7007=CYLINDRICAL_SURFACE('',#73140,0.0999999999999994) ;
#7008=CYLINDRICAL_SURFACE('',#73150,0.0999999999999994) ;
#7009=CYLINDRICAL_SURFACE('',#73154,0.0999999999999994) ;
#7010=CYLINDRICAL_SURFACE('',#73158,0.0999999999999994) ;
#7011=CYLINDRICAL_SURFACE('',#73162,0.0999999999999994) ;
#7012=CYLINDRICAL_SURFACE('',#73166,0.0999999999999994) ;
#7013=CYLINDRICAL_SURFACE('',#73170,0.0999999999999994) ;
#7014=CYLINDRICAL_SURFACE('',#73174,0.0999999999999994) ;
#7015=CYLINDRICAL_SURFACE('',#73178,0.0999999999999994) ;
#7016=CYLINDRICAL_SURFACE('',#73182,0.0999999999999994) ;
#7017=CYLINDRICAL_SURFACE('',#73186,0.0999999999999994) ;
#7018=CYLINDRICAL_SURFACE('',#73189,1.65625) ;
#7019=CYLINDRICAL_SURFACE('',#73192,0.0999999999999994) ;
#7020=CYLINDRICAL_SURFACE('',#73196,0.0999999999999994) ;
#7021=CYLINDRICAL_SURFACE('',#73200,0.0999999999999994) ;
#7022=CYLINDRICAL_SURFACE('',#73210,0.0999999999999994) ;
#7023=CYLINDRICAL_SURFACE('',#73214,0.0999999999999994) ;
#7024=CYLINDRICAL_SURFACE('',#73218,0.0999999999999994) ;
#7025=CYLINDRICAL_SURFACE('',#73222,0.0999999999999994) ;
#7026=CYLINDRICAL_SURFACE('',#73226,0.0999999999999994) ;
#7027=CYLINDRICAL_SURFACE('',#73230,0.0999999999999994) ;
#7028=CYLINDRICAL_SURFACE('',#73234,0.0999999999999994) ;
#7029=CYLINDRICAL_SURFACE('',#73238,0.0999999999999994) ;
#7030=CYLINDRICAL_SURFACE('',#73242,0.0999999999999994) ;
#7031=CYLINDRICAL_SURFACE('',#73246,0.0999999999999994) ;
#7032=CYLINDRICAL_SURFACE('',#73249,1.65625) ;
#7033=CYLINDRICAL_SURFACE('',#73252,0.0999999999999994) ;
#7034=CYLINDRICAL_SURFACE('',#73256,0.0999999999999994) ;
#7035=CYLINDRICAL_SURFACE('',#73260,0.0999999999999994) ;
#7036=CYLINDRICAL_SURFACE('',#73270,0.0999999999999994) ;
#7037=CYLINDRICAL_SURFACE('',#73274,0.0999999999999994) ;
#7038=CYLINDRICAL_SURFACE('',#73278,0.0999999999999994) ;
#7039=CYLINDRICAL_SURFACE('',#73282,0.100000000000001) ;
#7040=CYLINDRICAL_SURFACE('',#73286,0.0999999999999994) ;
#7041=CYLINDRICAL_SURFACE('',#73290,0.0999999999999994) ;
#7042=CYLINDRICAL_SURFACE('',#73294,0.0999999999999994) ;
#7043=CYLINDRICAL_SURFACE('',#73298,0.0999999999999994) ;
#7044=CYLINDRICAL_SURFACE('',#73302,0.0999999999999994) ;
#7045=CYLINDRICAL_SURFACE('',#73306,0.0999999999999994) ;
#7046=CYLINDRICAL_SURFACE('',#73309,1.65625) ;
#7047=CYLINDRICAL_SURFACE('',#73312,0.0999999999999994) ;
#7048=CYLINDRICAL_SURFACE('',#73316,0.0999999999999994) ;
#7049=CYLINDRICAL_SURFACE('',#73320,0.0999999999999994) ;
#7050=CYLINDRICAL_SURFACE('',#73330,0.0999999999999994) ;
#7051=CYLINDRICAL_SURFACE('',#73334,0.0999999999999994) ;
#7052=CYLINDRICAL_SURFACE('',#73338,0.0999999999999994) ;
#7053=CYLINDRICAL_SURFACE('',#73342,0.100000000000001) ;
#7054=CYLINDRICAL_SURFACE('',#73346,0.100000000000001) ;
#7055=CYLINDRICAL_SURFACE('',#73350,0.0999999999999994) ;
#7056=CYLINDRICAL_SURFACE('',#73354,0.0999999999999994) ;
#7057=CYLINDRICAL_SURFACE('',#73358,0.0999999999999994) ;
#7058=CYLINDRICAL_SURFACE('',#73362,0.0999999999999994) ;
#7059=CYLINDRICAL_SURFACE('',#73366,0.0999999999999994) ;
#7060=CYLINDRICAL_SURFACE('',#73369,1.65625) ;
#7061=CYLINDRICAL_SURFACE('',#73372,0.0999999999999994) ;
#7062=CYLINDRICAL_SURFACE('',#73376,0.0999999999999994) ;
#7063=CYLINDRICAL_SURFACE('',#73380,0.0999999999999994) ;
#7064=CYLINDRICAL_SURFACE('',#73390,0.1) ;
#7065=CYLINDRICAL_SURFACE('',#73394,0.1) ;
#7066=CYLINDRICAL_SURFACE('',#73398,0.0999999999999994) ;
#7067=CYLINDRICAL_SURFACE('',#73402,0.1) ;
#7068=CYLINDRICAL_SURFACE('',#73406,0.100000000000001) ;
#7069=CYLINDRICAL_SURFACE('',#73410,0.0999999999999994) ;
#7070=CYLINDRICAL_SURFACE('',#73414,0.0999999999999994) ;
#7071=CYLINDRICAL_SURFACE('',#73418,0.0999999999999994) ;
#7072=CYLINDRICAL_SURFACE('',#73422,0.0999999999999994) ;
#7073=CYLINDRICAL_SURFACE('',#73426,0.0999999999999994) ;
#7074=CYLINDRICAL_SURFACE('',#73429,1.65625) ;
#7075=CYLINDRICAL_SURFACE('',#73432,0.1) ;
#7076=CYLINDRICAL_SURFACE('',#73436,0.1) ;
#7077=CYLINDRICAL_SURFACE('',#73440,0.1) ;
#7078=CYLINDRICAL_SURFACE('',#73450,0.0999999999999998) ;
#7079=CYLINDRICAL_SURFACE('',#73454,0.0999999999999998) ;
#7080=CYLINDRICAL_SURFACE('',#73458,0.0999999999999994) ;
#7081=CYLINDRICAL_SURFACE('',#73462,0.100000000000001) ;
#7082=CYLINDRICAL_SURFACE('',#73466,0.1) ;
#7083=CYLINDRICAL_SURFACE('',#73470,0.1) ;
#7084=CYLINDRICAL_SURFACE('',#73474,0.1) ;
#7085=CYLINDRICAL_SURFACE('',#73478,0.1) ;
#7086=CYLINDRICAL_SURFACE('',#73482,0.1) ;
#7087=CYLINDRICAL_SURFACE('',#73486,0.1) ;
#7088=CYLINDRICAL_SURFACE('',#73489,1.65625) ;
#7089=CYLINDRICAL_SURFACE('',#73492,0.0999999999999998) ;
#7090=CYLINDRICAL_SURFACE('',#73496,0.0999999999999998) ;
#7091=CYLINDRICAL_SURFACE('',#73500,0.1) ;
#7092=CYLINDRICAL_SURFACE('',#73555,0.1) ;
#7093=CYLINDRICAL_SURFACE('',#73558,0.1) ;
#7094=CYLINDRICAL_SURFACE('',#73569,0.1) ;
#7095=CYLINDRICAL_SURFACE('',#73571,0.1) ;
#7096=CYLINDRICAL_SURFACE('',#73573,0.1) ;
#7097=CYLINDRICAL_SURFACE('',#73575,0.1) ;
#7098=CYLINDRICAL_SURFACE('',#73577,0.1) ;
#7099=CYLINDRICAL_SURFACE('',#73579,0.1) ;
#7100=CYLINDRICAL_SURFACE('',#73590,0.1) ;
#7101=CYLINDRICAL_SURFACE('',#73592,0.0999999999999998) ;
#7102=CYLINDRICAL_SURFACE('',#73594,0.1) ;
#7103=CYLINDRICAL_SURFACE('',#73596,0.1) ;
#7104=CYLINDRICAL_SURFACE('',#73598,0.1) ;
#7105=CYLINDRICAL_SURFACE('',#73608,0.1) ;
#7106=CYLINDRICAL_SURFACE('',#73615,0.1) ;
#7107=CYLINDRICAL_SURFACE('',#73617,0.1) ;
#7108=CYLINDRICAL_SURFACE('',#73619,0.0999999999999998) ;
#7109=CYLINDRICAL_SURFACE('',#73623,0.1) ;
#7110=CYLINDRICAL_SURFACE('',#73625,0.1) ;
#7111=CYLINDRICAL_SURFACE('',#73627,0.0999999999999998) ;
#7112=CYLINDRICAL_SURFACE('',#73634,0.1) ;
#7113=CYLINDRICAL_SURFACE('',#73641,0.1) ;
#7114=CYLINDRICAL_SURFACE('',#73643,0.1) ;
#7115=CYLINDRICAL_SURFACE('',#73647,0.1) ;
#7116=CYLINDRICAL_SURFACE('',#73650,0.1) ;
#7117=CYLINDRICAL_SURFACE('',#73652,0.1) ;
#7118=CYLINDRICAL_SURFACE('',#73655,0.1) ;
#7119=CYLINDRICAL_SURFACE('',#73662,0.1) ;
#7120=CYLINDRICAL_SURFACE('',#73664,0.1) ;
#7121=CYLINDRICAL_SURFACE('',#73670,0.1) ;
#7122=CYLINDRICAL_SURFACE('',#73672,0.1) ;
#7123=CYLINDRICAL_SURFACE('',#73678,0.1) ;
#7124=CYLINDRICAL_SURFACE('',#73686,0.1) ;
#7125=CYLINDRICAL_SURFACE('',#73687,0.1) ;
#7126=CYLINDRICAL_SURFACE('',#73691,0.1) ;
#7127=CYLINDRICAL_SURFACE('',#73693,0.0999999999999998) ;
#7128=CYLINDRICAL_SURFACE('',#73699,0.0999999999999998) ;
#7129=CYLINDRICAL_SURFACE('',#73701,0.1) ;
#7130=CYLINDRICAL_SURFACE('',#73707,0.0999999999999998) ;
#7131=CYLINDRICAL_SURFACE('',#73708,0.100000000000003) ;
#7132=CYLINDRICAL_SURFACE('',#73715,0.0999999999999994) ;
#7133=CYLINDRICAL_SURFACE('',#73717,0.1) ;
#7134=CYLINDRICAL_SURFACE('',#73723,0.0999999999999989) ;
#7135=CYLINDRICAL_SURFACE('',#73724,0.100000000000003) ;
#7136=CYLINDRICAL_SURFACE('',#73728,0.1) ;
#7137=CYLINDRICAL_SURFACE('',#73730,0.0999999999999994) ;
#7138=CYLINDRICAL_SURFACE('',#73736,0.0999999999999989) ;
#7139=CYLINDRICAL_SURFACE('',#73744,0.0999999999999998) ;
#7140=CYLINDRICAL_SURFACE('',#73746,0.0999999999999994) ;
#7141=CYLINDRICAL_SURFACE('',#73752,0.100000000000003) ;
#7142=CYLINDRICAL_SURFACE('',#73754,0.100000000000003) ;
#7143=CYLINDRICAL_SURFACE('',#73760,0.1) ;
#7144=CYLINDRICAL_SURFACE('',#73761,0.0999999999999994) ;
#7145=CYLINDRICAL_SURFACE('',#73768,0.0999999999999994) ;
#7146=CYLINDRICAL_SURFACE('',#73770,0.1) ;
#7147=CYLINDRICAL_SURFACE('',#73776,0.0999999999999989) ;
#7148=CYLINDRICAL_SURFACE('',#73777,0.100000000000003) ;
#7149=CYLINDRICAL_SURFACE('',#73781,0.1) ;
#7150=CYLINDRICAL_SURFACE('',#73783,0.0999999999999994) ;
#7151=CYLINDRICAL_SURFACE('',#73789,0.0999999999999989) ;
#7152=CYLINDRICAL_SURFACE('',#73797,0.0999999999999998) ;
#7153=CYLINDRICAL_SURFACE('',#73799,0.0999999999999994) ;
#7154=CYLINDRICAL_SURFACE('',#73805,0.0999999999999994) ;
#7155=CYLINDRICAL_SURFACE('',#73807,0.0999999999999994) ;
#7156=CYLINDRICAL_SURFACE('',#73813,0.1) ;
#7157=CYLINDRICAL_SURFACE('',#73814,0.0999999999999994) ;
#7158=CYLINDRICAL_SURFACE('',#73821,0.0999999999999994) ;
#7159=CYLINDRICAL_SURFACE('',#73823,0.1) ;
#7160=CYLINDRICAL_SURFACE('',#73829,0.0999999999999989) ;
#7161=CYLINDRICAL_SURFACE('',#73830,0.0999999999999994) ;
#7162=CYLINDRICAL_SURFACE('',#73834,0.1) ;
#7163=CYLINDRICAL_SURFACE('',#73836,0.0999999999999994) ;
#7164=CYLINDRICAL_SURFACE('',#73842,0.0999999999999989) ;
#7165=CYLINDRICAL_SURFACE('',#73850,0.0999999999999998) ;
#7166=CYLINDRICAL_SURFACE('',#73852,0.0999999999999994) ;
#7167=CYLINDRICAL_SURFACE('',#73858,0.0999999999999994) ;
#7168=CYLINDRICAL_SURFACE('',#73860,0.0999999999999994) ;
#7169=CYLINDRICAL_SURFACE('',#73866,0.1) ;
#7170=CYLINDRICAL_SURFACE('',#73867,0.0999999999999994) ;
#7171=CYLINDRICAL_SURFACE('',#73874,0.0999999999999994) ;
#7172=CYLINDRICAL_SURFACE('',#73876,0.1) ;
#7173=CYLINDRICAL_SURFACE('',#73882,0.0999999999999989) ;
#7174=CYLINDRICAL_SURFACE('',#73883,0.0999999999999994) ;
#7175=CYLINDRICAL_SURFACE('',#73887,0.1) ;
#7176=CYLINDRICAL_SURFACE('',#73889,0.0999999999999994) ;
#7177=CYLINDRICAL_SURFACE('',#73895,0.0999999999999989) ;
#7178=CYLINDRICAL_SURFACE('',#73903,0.0999999999999998) ;
#7179=CYLINDRICAL_SURFACE('',#73905,0.0999999999999994) ;
#7180=CYLINDRICAL_SURFACE('',#73911,0.0999999999999994) ;
#7181=CYLINDRICAL_SURFACE('',#73913,0.0999999999999994) ;
#7182=CYLINDRICAL_SURFACE('',#73919,0.1) ;
#7183=CYLINDRICAL_SURFACE('',#73920,0.0999999999999994) ;
#7184=CYLINDRICAL_SURFACE('',#73927,0.0999999999999994) ;
#7185=CYLINDRICAL_SURFACE('',#73929,0.1) ;
#7186=CYLINDRICAL_SURFACE('',#73935,0.0999999999999989) ;
#7187=CYLINDRICAL_SURFACE('',#73936,0.0999999999999994) ;
#7188=CYLINDRICAL_SURFACE('',#73940,0.1) ;
#7189=CYLINDRICAL_SURFACE('',#73942,0.0999999999999994) ;
#7190=CYLINDRICAL_SURFACE('',#73948,0.0999999999999989) ;
#7191=CYLINDRICAL_SURFACE('',#73956,0.0999999999999998) ;
#7192=CYLINDRICAL_SURFACE('',#73958,0.0999999999999994) ;
#7193=CYLINDRICAL_SURFACE('',#73964,0.0999999999999994) ;
#7194=CYLINDRICAL_SURFACE('',#73966,0.0999999999999994) ;
#7195=CYLINDRICAL_SURFACE('',#73972,0.1) ;
#7196=CYLINDRICAL_SURFACE('',#73973,0.0999999999999994) ;
#7197=CYLINDRICAL_SURFACE('',#73980,0.0999999999999994) ;
#7198=CYLINDRICAL_SURFACE('',#73982,0.1) ;
#7199=CYLINDRICAL_SURFACE('',#73988,0.0999999999999989) ;
#7200=CYLINDRICAL_SURFACE('',#73989,0.0999999999999994) ;
#7201=CYLINDRICAL_SURFACE('',#73993,0.1) ;
#7202=CYLINDRICAL_SURFACE('',#73995,0.0999999999999994) ;
#7203=CYLINDRICAL_SURFACE('',#74001,0.1) ;
#7204=CYLINDRICAL_SURFACE('',#74009,0.0999999999999998) ;
#7205=CYLINDRICAL_SURFACE('',#74011,0.0999999999999994) ;
#7206=CYLINDRICAL_SURFACE('',#74017,0.0999999999999994) ;
#7207=CYLINDRICAL_SURFACE('',#74019,0.0999999999999994) ;
#7208=CYLINDRICAL_SURFACE('',#74025,0.1) ;
#7209=CYLINDRICAL_SURFACE('',#74026,0.0999999999999994) ;
#7210=CYLINDRICAL_SURFACE('',#74033,0.0999999999999994) ;
#7211=CYLINDRICAL_SURFACE('',#74035,0.1) ;
#7212=CYLINDRICAL_SURFACE('',#74041,0.1) ;
#7213=CYLINDRICAL_SURFACE('',#74042,0.0999999999999994) ;
#7214=CYLINDRICAL_SURFACE('',#74046,0.1) ;
#7215=CYLINDRICAL_SURFACE('',#74048,0.0999999999999994) ;
#7216=CYLINDRICAL_SURFACE('',#74054,0.1) ;
#7217=CYLINDRICAL_SURFACE('',#74062,0.0999999999999998) ;
#7218=CYLINDRICAL_SURFACE('',#74064,0.0999999999999994) ;
#7219=CYLINDRICAL_SURFACE('',#74070,0.0999999999999994) ;
#7220=CYLINDRICAL_SURFACE('',#74072,0.0999999999999994) ;
#7221=CYLINDRICAL_SURFACE('',#74078,0.1) ;
#7222=CYLINDRICAL_SURFACE('',#74079,0.0999999999999994) ;
#7223=CYLINDRICAL_SURFACE('',#74086,0.0999999999999994) ;
#7224=CYLINDRICAL_SURFACE('',#74088,0.1) ;
#7225=CYLINDRICAL_SURFACE('',#74094,0.1) ;
#7226=CYLINDRICAL_SURFACE('',#74095,0.0999999999999994) ;
#7227=CYLINDRICAL_SURFACE('',#74099,0.1) ;
#7228=CYLINDRICAL_SURFACE('',#74101,0.0999999999999994) ;
#7229=CYLINDRICAL_SURFACE('',#74107,0.1) ;
#7230=CYLINDRICAL_SURFACE('',#74115,0.0999999999999998) ;
#7231=CYLINDRICAL_SURFACE('',#74117,0.0999999999999994) ;
#7232=CYLINDRICAL_SURFACE('',#74123,0.1) ;
#7233=CYLINDRICAL_SURFACE('',#74125,0.1) ;
#7234=CYLINDRICAL_SURFACE('',#74131,0.1) ;
#7235=CYLINDRICAL_SURFACE('',#74132,0.1) ;
#7236=CYLINDRICAL_SURFACE('',#74139,0.0999999999999994) ;
#7237=CYLINDRICAL_SURFACE('',#74141,0.1) ;
#7238=CYLINDRICAL_SURFACE('',#74147,0.1) ;
#7239=CYLINDRICAL_SURFACE('',#74148,0.1) ;
#7240=CYLINDRICAL_SURFACE('',#74152,0.1) ;
#7241=CYLINDRICAL_SURFACE('',#74154,0.0999999999999994) ;
#7242=CYLINDRICAL_SURFACE('',#74160,0.1) ;
#7243=CYLINDRICAL_SURFACE('',#74168,0.0999999999999998) ;
#7244=CYLINDRICAL_SURFACE('',#74170,0.0999999999999994) ;
#7245=CYLINDRICAL_SURFACE('',#74176,0.0999999999999998) ;
#7246=CYLINDRICAL_SURFACE('',#74178,0.0999999999999998) ;
#7247=CYLINDRICAL_SURFACE('',#74184,0.1) ;
#7248=CYLINDRICAL_SURFACE('',#74185,0.1) ;
#7249=CYLINDRICAL_SURFACE('',#74188,0.1) ;
#7250=CYLINDRICAL_SURFACE('',#74199,0.1) ;
#7251=CYLINDRICAL_SURFACE('',#74201,0.1) ;
#7252=CYLINDRICAL_SURFACE('',#74203,0.1) ;
#7253=CYLINDRICAL_SURFACE('',#74205,0.1) ;
#7254=CYLINDRICAL_SURFACE('',#74207,0.1) ;
#7255=CYLINDRICAL_SURFACE('',#74209,0.1) ;
#7256=CYLINDRICAL_SURFACE('',#74220,0.1) ;
#7257=CYLINDRICAL_SURFACE('',#74222,0.0999999999999998) ;
#7258=CYLINDRICAL_SURFACE('',#74224,0.1) ;
#7259=CYLINDRICAL_SURFACE('',#74226,0.1) ;
#7260=CYLINDRICAL_SURFACE('',#74228,0.1) ;
#7261=CYLINDRICAL_SURFACE('',#74238,0.1) ;
#7262=CYLINDRICAL_SURFACE('',#74245,0.1) ;
#7263=CYLINDRICAL_SURFACE('',#74247,0.1) ;
#7264=CYLINDRICAL_SURFACE('',#74249,0.1) ;
#7265=CYLINDRICAL_SURFACE('',#74253,0.1) ;
#7266=CYLINDRICAL_SURFACE('',#74255,0.1) ;
#7267=CYLINDRICAL_SURFACE('',#74257,0.0999999999999998) ;
#7268=CYLINDRICAL_SURFACE('',#74264,0.1) ;
#7269=CYLINDRICAL_SURFACE('',#74271,0.1) ;
#7270=CYLINDRICAL_SURFACE('',#74273,0.1) ;
#7271=CYLINDRICAL_SURFACE('',#74277,0.1) ;
#7272=CYLINDRICAL_SURFACE('',#74280,0.1) ;
#7273=CYLINDRICAL_SURFACE('',#74282,0.0999999999999994) ;
#7274=CYLINDRICAL_SURFACE('',#74285,0.1) ;
#7275=CYLINDRICAL_SURFACE('',#74292,0.0999999999999994) ;
#7276=CYLINDRICAL_SURFACE('',#74294,0.0999999999999994) ;
#7277=CYLINDRICAL_SURFACE('',#74300,0.1) ;
#7278=CYLINDRICAL_SURFACE('',#74302,0.1) ;
#7279=CYLINDRICAL_SURFACE('',#74308,0.1) ;
#7280=CYLINDRICAL_SURFACE('',#74316,0.1) ;
#7281=CYLINDRICAL_SURFACE('',#74317,0.1) ;
#7282=CYLINDRICAL_SURFACE('',#74321,0.1) ;
#7283=CYLINDRICAL_SURFACE('',#74323,0.1) ;
#7284=CYLINDRICAL_SURFACE('',#74329,0.0999999999999998) ;
#7285=CYLINDRICAL_SURFACE('',#74331,0.1) ;
#7286=CYLINDRICAL_SURFACE('',#74337,0.1) ;
#7287=CYLINDRICAL_SURFACE('',#74338,0.1) ;
#7288=CYLINDRICAL_SURFACE('',#74341,0.1) ;
#7289=CYLINDRICAL_SURFACE('',#74352,0.1) ;
#7290=CYLINDRICAL_SURFACE('',#74354,0.1) ;
#7291=CYLINDRICAL_SURFACE('',#74356,0.1) ;
#7292=CYLINDRICAL_SURFACE('',#74358,0.1) ;
#7293=CYLINDRICAL_SURFACE('',#74360,0.1) ;
#7294=CYLINDRICAL_SURFACE('',#74362,0.1) ;
#7295=CYLINDRICAL_SURFACE('',#74373,0.1) ;
#7296=CYLINDRICAL_SURFACE('',#74375,0.0999999999999998) ;
#7297=CYLINDRICAL_SURFACE('',#74377,0.1) ;
#7298=CYLINDRICAL_SURFACE('',#74379,0.1) ;
#7299=CYLINDRICAL_SURFACE('',#74381,0.1) ;
#7300=CYLINDRICAL_SURFACE('',#74391,0.1) ;
#7301=CYLINDRICAL_SURFACE('',#74398,0.1) ;
#7302=CYLINDRICAL_SURFACE('',#74400,0.1) ;
#7303=CYLINDRICAL_SURFACE('',#74402,0.0999999999999994) ;
#7304=CYLINDRICAL_SURFACE('',#74406,0.1) ;
#7305=CYLINDRICAL_SURFACE('',#74408,0.1) ;
#7306=CYLINDRICAL_SURFACE('',#74410,0.0999999999999998) ;
#7307=CYLINDRICAL_SURFACE('',#74417,0.1) ;
#7308=CYLINDRICAL_SURFACE('',#74424,0.1) ;
#7309=CYLINDRICAL_SURFACE('',#74426,0.1) ;
#7310=CYLINDRICAL_SURFACE('',#74430,0.1) ;
#7311=CYLINDRICAL_SURFACE('',#74433,0.1) ;
#7312=CYLINDRICAL_SURFACE('',#74435,0.0999999999999994) ;
#7313=CYLINDRICAL_SURFACE('',#74438,0.1) ;
#7314=CYLINDRICAL_SURFACE('',#74445,0.0999999999999994) ;
#7315=CYLINDRICAL_SURFACE('',#74447,0.0999999999999994) ;
#7316=CYLINDRICAL_SURFACE('',#74453,0.1) ;
#7317=CYLINDRICAL_SURFACE('',#74455,0.1) ;
#7318=CYLINDRICAL_SURFACE('',#74461,0.1) ;
#7319=CYLINDRICAL_SURFACE('',#74469,0.1) ;
#7320=CYLINDRICAL_SURFACE('',#74470,0.1) ;
#7321=CYLINDRICAL_SURFACE('',#74474,0.1) ;
#7322=CYLINDRICAL_SURFACE('',#74476,0.0999999999999994) ;
#7323=CYLINDRICAL_SURFACE('',#74482,0.0999999999999998) ;
#7324=CYLINDRICAL_SURFACE('',#74484,0.1) ;
#7325=CYLINDRICAL_SURFACE('',#74490,0.0999999999999994) ;
#7326=CYLINDRICAL_SURFACE('',#74491,0.1) ;
#7327=CYLINDRICAL_SURFACE('',#74494,0.1) ;
#7328=CYLINDRICAL_SURFACE('',#74505,0.1) ;
#7329=CYLINDRICAL_SURFACE('',#74507,0.1) ;
#7330=CYLINDRICAL_SURFACE('',#74509,0.1) ;
#7331=CYLINDRICAL_SURFACE('',#74511,0.1) ;
#7332=CYLINDRICAL_SURFACE('',#74513,0.1) ;
#7333=CYLINDRICAL_SURFACE('',#74515,0.1) ;
#7334=CYLINDRICAL_SURFACE('',#74526,0.1) ;
#7335=CYLINDRICAL_SURFACE('',#74528,0.0999999999999998) ;
#7336=CYLINDRICAL_SURFACE('',#74530,0.1) ;
#7337=CYLINDRICAL_SURFACE('',#74532,0.1) ;
#7338=CYLINDRICAL_SURFACE('',#74534,0.1) ;
#7339=CYLINDRICAL_SURFACE('',#74544,0.1) ;
#7340=CYLINDRICAL_SURFACE('',#74551,0.1) ;
#7341=CYLINDRICAL_SURFACE('',#74553,0.1) ;
#7342=CYLINDRICAL_SURFACE('',#74555,0.0999999999999994) ;
#7343=CYLINDRICAL_SURFACE('',#74559,0.1) ;
#7344=CYLINDRICAL_SURFACE('',#74561,0.1) ;
#7345=CYLINDRICAL_SURFACE('',#74563,0.0999999999999998) ;
#7346=CYLINDRICAL_SURFACE('',#74570,0.1) ;
#7347=CYLINDRICAL_SURFACE('',#74577,0.1) ;
#7348=CYLINDRICAL_SURFACE('',#74579,0.1) ;
#7349=CYLINDRICAL_SURFACE('',#74583,0.1) ;
#7350=CYLINDRICAL_SURFACE('',#74586,0.1) ;
#7351=CYLINDRICAL_SURFACE('',#74588,0.0999999999999994) ;
#7352=CYLINDRICAL_SURFACE('',#74591,0.1) ;
#7353=CYLINDRICAL_SURFACE('',#74598,0.0999999999999994) ;
#7354=CYLINDRICAL_SURFACE('',#74600,0.0999999999999994) ;
#7355=CYLINDRICAL_SURFACE('',#74606,0.1) ;
#7356=CYLINDRICAL_SURFACE('',#74608,0.1) ;
#7357=CYLINDRICAL_SURFACE('',#74614,0.1) ;
#7358=CYLINDRICAL_SURFACE('',#74622,0.1) ;
#7359=CYLINDRICAL_SURFACE('',#74623,0.1) ;
#7360=CYLINDRICAL_SURFACE('',#74627,0.1) ;
#7361=CYLINDRICAL_SURFACE('',#74629,0.0999999999999994) ;
#7362=CYLINDRICAL_SURFACE('',#74635,0.0999999999999998) ;
#7363=CYLINDRICAL_SURFACE('',#74637,0.1) ;
#7364=CYLINDRICAL_SURFACE('',#74643,0.0999999999999994) ;
#7365=CYLINDRICAL_SURFACE('',#74644,0.1) ;
#7366=CYLINDRICAL_SURFACE('',#74647,0.1) ;
#7367=CYLINDRICAL_SURFACE('',#74658,0.1) ;
#7368=CYLINDRICAL_SURFACE('',#74660,0.1) ;
#7369=CYLINDRICAL_SURFACE('',#74662,0.1) ;
#7370=CYLINDRICAL_SURFACE('',#74664,0.1) ;
#7371=CYLINDRICAL_SURFACE('',#74666,0.1) ;
#7372=CYLINDRICAL_SURFACE('',#74668,0.1) ;
#7373=CYLINDRICAL_SURFACE('',#74679,0.1) ;
#7374=CYLINDRICAL_SURFACE('',#74681,0.0999999999999998) ;
#7375=CYLINDRICAL_SURFACE('',#74683,0.1) ;
#7376=CYLINDRICAL_SURFACE('',#74685,0.1) ;
#7377=CYLINDRICAL_SURFACE('',#74687,0.1) ;
#7378=CYLINDRICAL_SURFACE('',#74697,0.1) ;
#7379=CYLINDRICAL_SURFACE('',#74704,0.1) ;
#7380=CYLINDRICAL_SURFACE('',#74706,0.1) ;
#7381=CYLINDRICAL_SURFACE('',#74708,0.0999999999999994) ;
#7382=CYLINDRICAL_SURFACE('',#74712,0.1) ;
#7383=CYLINDRICAL_SURFACE('',#74714,0.1) ;
#7384=CYLINDRICAL_SURFACE('',#74716,0.0999999999999998) ;
#7385=CYLINDRICAL_SURFACE('',#74723,0.1) ;
#7386=CYLINDRICAL_SURFACE('',#74730,0.1) ;
#7387=CYLINDRICAL_SURFACE('',#74732,0.1) ;
#7388=CYLINDRICAL_SURFACE('',#74736,0.1) ;
#7389=CYLINDRICAL_SURFACE('',#74739,0.1) ;
#7390=CYLINDRICAL_SURFACE('',#74741,0.0999999999999994) ;
#7391=CYLINDRICAL_SURFACE('',#74744,0.1) ;
#7392=CYLINDRICAL_SURFACE('',#74751,0.0999999999999994) ;
#7393=CYLINDRICAL_SURFACE('',#74753,0.0999999999999994) ;
#7394=CYLINDRICAL_SURFACE('',#74759,0.1) ;
#7395=CYLINDRICAL_SURFACE('',#74761,0.1) ;
#7396=CYLINDRICAL_SURFACE('',#74767,0.0999999999999988) ;
#7397=CYLINDRICAL_SURFACE('',#74775,0.1) ;
#7398=CYLINDRICAL_SURFACE('',#74776,0.1) ;
#7399=CYLINDRICAL_SURFACE('',#74780,0.0999999999999989) ;
#7400=CYLINDRICAL_SURFACE('',#74782,0.0999999999999994) ;
#7401=CYLINDRICAL_SURFACE('',#74788,0.0999999999999998) ;
#7402=CYLINDRICAL_SURFACE('',#74790,0.1) ;
#7403=CYLINDRICAL_SURFACE('',#74796,0.0999999999999994) ;
#7404=CYLINDRICAL_SURFACE('',#74797,0.1) ;
#7405=CYLINDRICAL_SURFACE('',#74800,0.1) ;
#7406=CYLINDRICAL_SURFACE('',#74811,0.1) ;
#7407=CYLINDRICAL_SURFACE('',#74813,0.1) ;
#7408=CYLINDRICAL_SURFACE('',#74815,0.1) ;
#7409=CYLINDRICAL_SURFACE('',#74817,0.1) ;
#7410=CYLINDRICAL_SURFACE('',#74819,0.1) ;
#7411=CYLINDRICAL_SURFACE('',#74821,0.1) ;
#7412=CYLINDRICAL_SURFACE('',#74832,0.1) ;
#7413=CYLINDRICAL_SURFACE('',#74834,0.0999999999999998) ;
#7414=CYLINDRICAL_SURFACE('',#74836,0.1) ;
#7415=CYLINDRICAL_SURFACE('',#74838,0.1) ;
#7416=CYLINDRICAL_SURFACE('',#74840,0.1) ;
#7417=CYLINDRICAL_SURFACE('',#74850,0.1) ;
#7418=CYLINDRICAL_SURFACE('',#74857,0.1) ;
#7419=CYLINDRICAL_SURFACE('',#74859,0.1) ;
#7420=CYLINDRICAL_SURFACE('',#74861,0.0999999999999994) ;
#7421=CYLINDRICAL_SURFACE('',#74865,0.1) ;
#7422=CYLINDRICAL_SURFACE('',#74867,0.1) ;
#7423=CYLINDRICAL_SURFACE('',#74869,0.0999999999999998) ;
#7424=CYLINDRICAL_SURFACE('',#74876,0.1) ;
#7425=CYLINDRICAL_SURFACE('',#74883,0.1) ;
#7426=CYLINDRICAL_SURFACE('',#74885,0.1) ;
#7427=CYLINDRICAL_SURFACE('',#74889,0.1) ;
#7428=CYLINDRICAL_SURFACE('',#74892,0.1) ;
#7429=CYLINDRICAL_SURFACE('',#74894,0.0999999999999994) ;
#7430=CYLINDRICAL_SURFACE('',#74897,0.1) ;
#7431=CYLINDRICAL_SURFACE('',#74904,0.0999999999999994) ;
#7432=CYLINDRICAL_SURFACE('',#74906,0.0999999999999994) ;
#7433=CYLINDRICAL_SURFACE('',#74912,0.1) ;
#7434=CYLINDRICAL_SURFACE('',#74914,0.1) ;
#7435=CYLINDRICAL_SURFACE('',#74920,0.0999999999999988) ;
#7436=CYLINDRICAL_SURFACE('',#74928,0.1) ;
#7437=CYLINDRICAL_SURFACE('',#74929,0.1) ;
#7438=CYLINDRICAL_SURFACE('',#74933,0.0999999999999989) ;
#7439=CYLINDRICAL_SURFACE('',#74935,0.0999999999999994) ;
#7440=CYLINDRICAL_SURFACE('',#74941,0.0999999999999998) ;
#7441=CYLINDRICAL_SURFACE('',#74943,0.1) ;
#7442=CYLINDRICAL_SURFACE('',#74949,0.0999999999999994) ;
#7443=CYLINDRICAL_SURFACE('',#74950,0.1) ;
#7444=CYLINDRICAL_SURFACE('',#74953,0.1) ;
#7445=CYLINDRICAL_SURFACE('',#74964,0.1) ;
#7446=CYLINDRICAL_SURFACE('',#74966,0.1) ;
#7447=CYLINDRICAL_SURFACE('',#74968,0.1) ;
#7448=CYLINDRICAL_SURFACE('',#74970,0.1) ;
#7449=CYLINDRICAL_SURFACE('',#74972,0.1) ;
#7450=CYLINDRICAL_SURFACE('',#74974,0.1) ;
#7451=CYLINDRICAL_SURFACE('',#74985,0.1) ;
#7452=CYLINDRICAL_SURFACE('',#74987,0.0999999999999998) ;
#7453=CYLINDRICAL_SURFACE('',#74989,0.1) ;
#7454=CYLINDRICAL_SURFACE('',#74991,0.1) ;
#7455=CYLINDRICAL_SURFACE('',#74993,0.1) ;
#7456=CYLINDRICAL_SURFACE('',#75003,0.1) ;
#7457=CYLINDRICAL_SURFACE('',#75010,0.1) ;
#7458=CYLINDRICAL_SURFACE('',#75012,0.1) ;
#7459=CYLINDRICAL_SURFACE('',#75014,0.0999999999999994) ;
#7460=CYLINDRICAL_SURFACE('',#75018,0.1) ;
#7461=CYLINDRICAL_SURFACE('',#75020,0.1) ;
#7462=CYLINDRICAL_SURFACE('',#75022,0.0999999999999998) ;
#7463=CYLINDRICAL_SURFACE('',#75029,0.1) ;
#7464=CYLINDRICAL_SURFACE('',#75036,0.1) ;
#7465=CYLINDRICAL_SURFACE('',#75038,0.1) ;
#7466=CYLINDRICAL_SURFACE('',#75042,0.1) ;
#7467=CYLINDRICAL_SURFACE('',#75045,0.1) ;
#7468=CYLINDRICAL_SURFACE('',#75047,0.0999999999999994) ;
#7469=CYLINDRICAL_SURFACE('',#75050,0.1) ;
#7470=CYLINDRICAL_SURFACE('',#75057,0.0999999999999994) ;
#7471=CYLINDRICAL_SURFACE('',#75059,0.0999999999999994) ;
#7472=CYLINDRICAL_SURFACE('',#75065,0.1) ;
#7473=CYLINDRICAL_SURFACE('',#75067,0.1) ;
#7474=CYLINDRICAL_SURFACE('',#75073,0.0999999999999988) ;
#7475=CYLINDRICAL_SURFACE('',#75081,0.1) ;
#7476=CYLINDRICAL_SURFACE('',#75082,0.1) ;
#7477=CYLINDRICAL_SURFACE('',#75086,0.0999999999999989) ;
#7478=CYLINDRICAL_SURFACE('',#75088,0.0999999999999994) ;
#7479=CYLINDRICAL_SURFACE('',#75094,0.0999999999999998) ;
#7480=CYLINDRICAL_SURFACE('',#75096,0.1) ;
#7481=CYLINDRICAL_SURFACE('',#75102,0.0999999999999994) ;
#7482=CYLINDRICAL_SURFACE('',#75103,0.1) ;
#7483=CYLINDRICAL_SURFACE('',#75106,0.1) ;
#7484=CYLINDRICAL_SURFACE('',#75117,0.1) ;
#7485=CYLINDRICAL_SURFACE('',#75119,0.1) ;
#7486=CYLINDRICAL_SURFACE('',#75121,0.1) ;
#7487=CYLINDRICAL_SURFACE('',#75123,0.1) ;
#7488=CYLINDRICAL_SURFACE('',#75125,0.1) ;
#7489=CYLINDRICAL_SURFACE('',#75127,0.1) ;
#7490=CYLINDRICAL_SURFACE('',#75138,0.1) ;
#7491=CYLINDRICAL_SURFACE('',#75140,0.0999999999999998) ;
#7492=CYLINDRICAL_SURFACE('',#75142,0.1) ;
#7493=CYLINDRICAL_SURFACE('',#75144,0.1) ;
#7494=CYLINDRICAL_SURFACE('',#75146,0.1) ;
#7495=CYLINDRICAL_SURFACE('',#75156,0.1) ;
#7496=CYLINDRICAL_SURFACE('',#75163,0.1) ;
#7497=CYLINDRICAL_SURFACE('',#75165,0.1) ;
#7498=CYLINDRICAL_SURFACE('',#75167,0.0999999999999994) ;
#7499=CYLINDRICAL_SURFACE('',#75171,0.1) ;
#7500=CYLINDRICAL_SURFACE('',#75173,0.1) ;
#7501=CYLINDRICAL_SURFACE('',#75175,0.0999999999999998) ;
#7502=CYLINDRICAL_SURFACE('',#75182,0.1) ;
#7503=CYLINDRICAL_SURFACE('',#75189,0.1) ;
#7504=CYLINDRICAL_SURFACE('',#75191,0.1) ;
#7505=CYLINDRICAL_SURFACE('',#75195,0.1) ;
#7506=CYLINDRICAL_SURFACE('',#75198,0.1) ;
#7507=CYLINDRICAL_SURFACE('',#75200,0.100000000000003) ;
#7508=CYLINDRICAL_SURFACE('',#75203,0.1) ;
#7509=CYLINDRICAL_SURFACE('',#75210,0.0999999999999994) ;
#7510=CYLINDRICAL_SURFACE('',#75212,0.100000000000003) ;
#7511=CYLINDRICAL_SURFACE('',#75218,0.1) ;
#7512=CYLINDRICAL_SURFACE('',#75220,0.1) ;
#7513=CYLINDRICAL_SURFACE('',#75226,0.0999999999999988) ;
#7514=CYLINDRICAL_SURFACE('',#75234,0.1) ;
#7515=CYLINDRICAL_SURFACE('',#75235,0.1) ;
#7516=CYLINDRICAL_SURFACE('',#75239,0.0999999999999989) ;
#7517=CYLINDRICAL_SURFACE('',#75241,0.0999999999999994) ;
#7518=CYLINDRICAL_SURFACE('',#75247,0.0999999999999998) ;
#7519=CYLINDRICAL_SURFACE('',#75249,0.1) ;
#7520=CYLINDRICAL_SURFACE('',#75255,0.0999999999999994) ;
#7521=CYLINDRICAL_SURFACE('',#75256,0.1) ;
#7522=CYLINDRICAL_SURFACE('',#75259,0.1) ;
#7523=CYLINDRICAL_SURFACE('',#75270,0.1) ;
#7524=CYLINDRICAL_SURFACE('',#75272,0.1) ;
#7525=CYLINDRICAL_SURFACE('',#75274,0.1) ;
#7526=CYLINDRICAL_SURFACE('',#75276,0.1) ;
#7527=CYLINDRICAL_SURFACE('',#75278,0.1) ;
#7528=CYLINDRICAL_SURFACE('',#75280,0.1) ;
#7529=CYLINDRICAL_SURFACE('',#75291,0.1) ;
#7530=CYLINDRICAL_SURFACE('',#75293,0.0999999999999998) ;
#7531=CYLINDRICAL_SURFACE('',#75295,0.1) ;
#7532=CYLINDRICAL_SURFACE('',#75297,0.1) ;
#7533=CYLINDRICAL_SURFACE('',#75299,0.1) ;
#7534=CYLINDRICAL_SURFACE('',#75309,0.1) ;
#7535=CYLINDRICAL_SURFACE('',#75316,0.1) ;
#7536=CYLINDRICAL_SURFACE('',#75318,0.1) ;
#7537=CYLINDRICAL_SURFACE('',#75320,0.100000000000003) ;
#7538=CYLINDRICAL_SURFACE('',#75324,0.1) ;
#7539=CYLINDRICAL_SURFACE('',#75326,0.1) ;
#7540=CYLINDRICAL_SURFACE('',#75328,0.0999999999999998) ;
#7541=CYLINDRICAL_SURFACE('',#75335,0.1) ;
#7542=CYLINDRICAL_SURFACE('',#75342,0.1) ;
#7543=CYLINDRICAL_SURFACE('',#75344,0.1) ;
#7544=CYLINDRICAL_SURFACE('',#75348,0.1) ;
#7545=CYLINDRICAL_SURFACE('',#75351,0.1) ;
#7546=CYLINDRICAL_SURFACE('',#75353,0.100000000000003) ;
#7547=CYLINDRICAL_SURFACE('',#75356,0.1) ;
#7548=CYLINDRICAL_SURFACE('',#75363,0.100000000000003) ;
#7549=CYLINDRICAL_SURFACE('',#75365,0.100000000000003) ;
#7550=CYLINDRICAL_SURFACE('',#75371,0.1) ;
#7551=CYLINDRICAL_SURFACE('',#75373,0.1) ;
#7552=CYLINDRICAL_SURFACE('',#75379,0.0999999999999988) ;
#7553=CYLINDRICAL_SURFACE('',#75387,0.1) ;
#7554=CYLINDRICAL_SURFACE('',#75388,0.1) ;
#7555=CYLINDRICAL_SURFACE('',#75392,0.0999999999999989) ;
#7556=CYLINDRICAL_SURFACE('',#75394,0.100000000000003) ;
#7557=CYLINDRICAL_SURFACE('',#75400,0.0999999999999998) ;
#7558=CYLINDRICAL_SURFACE('',#75402,0.1) ;
#7559=CYLINDRICAL_SURFACE('',#75408,0.100000000000003) ;
#7560=CYLINDRICAL_SURFACE('',#75420,1.) ;
#7561=CYLINDRICAL_SURFACE('',#75423,0.2) ;
#7562=CYLINDRICAL_SURFACE('',#75444,1.) ;
#7563=CYLINDRICAL_SURFACE('',#75447,0.2) ;
#7564=CYLINDRICAL_SURFACE('',#75468,1.) ;
#7565=CYLINDRICAL_SURFACE('',#75471,0.2) ;
#7566=CYLINDRICAL_SURFACE('',#75492,1.) ;
#7567=CYLINDRICAL_SURFACE('',#75495,0.2) ;
#7568=CYLINDRICAL_SURFACE('',#75516,1.) ;
#7569=CYLINDRICAL_SURFACE('',#75519,0.2) ;
#7570=CYLINDRICAL_SURFACE('',#75540,1.) ;
#7571=CYLINDRICAL_SURFACE('',#75543,0.2) ;
#7572=CYLINDRICAL_SURFACE('',#75564,1.) ;
#7573=CYLINDRICAL_SURFACE('',#75567,0.2) ;
#7574=CYLINDRICAL_SURFACE('',#75588,1.) ;
#7575=CYLINDRICAL_SURFACE('',#75591,0.2) ;
#7576=CYLINDRICAL_SURFACE('',#75612,1.) ;
#7577=CYLINDRICAL_SURFACE('',#75615,0.2) ;
#7578=CYLINDRICAL_SURFACE('',#75661,0.0999999999999999) ;
#7579=CYLINDRICAL_SURFACE('',#75664,0.1) ;
#7580=CYLINDRICAL_SURFACE('',#75670,0.0999999999999999) ;
#7581=CYLINDRICAL_SURFACE('',#75673,0.1) ;
#7582=CYLINDRICAL_SURFACE('',#75675,0.0999999999999998) ;
#7583=CYLINDRICAL_SURFACE('',#75682,0.0999999999999998) ;
#7584=CYLINDRICAL_SURFACE('',#75684,0.1) ;
#7585=CYLINDRICAL_SURFACE('',#75686,0.1) ;
#7586=CYLINDRICAL_SURFACE('',#75690,0.1) ;
#7587=CYLINDRICAL_SURFACE('',#75693,0.0999999999999999) ;
#7588=CYLINDRICAL_SURFACE('',#75695,0.1) ;
#7589=CYLINDRICAL_SURFACE('',#75698,0.1) ;
#7590=CYLINDRICAL_SURFACE('',#75704,0.1) ;
#7591=CYLINDRICAL_SURFACE('',#75707,0.1) ;
#7592=CYLINDRICAL_SURFACE('',#75709,0.0999999999999998) ;
#7593=CYLINDRICAL_SURFACE('',#75716,0.0999999999999998) ;
#7594=CYLINDRICAL_SURFACE('',#75718,0.1) ;
#7595=CYLINDRICAL_SURFACE('',#75720,0.1) ;
#7596=CYLINDRICAL_SURFACE('',#75724,0.1) ;
#7597=CYLINDRICAL_SURFACE('',#75727,0.1) ;
#7598=CYLINDRICAL_SURFACE('',#75729,0.1) ;
#7599=CYLINDRICAL_SURFACE('',#75732,0.1) ;
#7600=CYLINDRICAL_SURFACE('',#75738,0.1) ;
#7601=CYLINDRICAL_SURFACE('',#75741,0.1) ;
#7602=CYLINDRICAL_SURFACE('',#75743,0.1) ;
#7603=CYLINDRICAL_SURFACE('',#75750,0.1) ;
#7604=CYLINDRICAL_SURFACE('',#75752,0.1) ;
#7605=CYLINDRICAL_SURFACE('',#75754,0.1) ;
#7606=CYLINDRICAL_SURFACE('',#75758,0.1) ;
#7607=CYLINDRICAL_SURFACE('',#75761,0.1) ;
#7608=CYLINDRICAL_SURFACE('',#75763,0.1) ;
#7609=CYLINDRICAL_SURFACE('',#75766,0.1) ;
#7610=CYLINDRICAL_SURFACE('',#75772,0.1) ;
#7611=CYLINDRICAL_SURFACE('',#75775,0.1) ;
#7612=CYLINDRICAL_SURFACE('',#75777,0.1) ;
#7613=CYLINDRICAL_SURFACE('',#75784,0.1) ;
#7614=CYLINDRICAL_SURFACE('',#75786,0.1) ;
#7615=CYLINDRICAL_SURFACE('',#75788,0.1) ;
#7616=CYLINDRICAL_SURFACE('',#75792,0.1) ;
#7617=CYLINDRICAL_SURFACE('',#75795,0.1) ;
#7618=CYLINDRICAL_SURFACE('',#75797,0.1) ;
#7619=CYLINDRICAL_SURFACE('',#75800,0.1) ;
#7620=CYLINDRICAL_SURFACE('',#75806,0.1) ;
#7621=CYLINDRICAL_SURFACE('',#75809,0.1) ;
#7622=CYLINDRICAL_SURFACE('',#75811,0.0999999999999994) ;
#7623=CYLINDRICAL_SURFACE('',#75818,0.0999999999999994) ;
#7624=CYLINDRICAL_SURFACE('',#75820,0.1) ;
#7625=CYLINDRICAL_SURFACE('',#75822,0.1) ;
#7626=CYLINDRICAL_SURFACE('',#75826,0.1) ;
#7627=CYLINDRICAL_SURFACE('',#75829,0.1) ;
#7628=CYLINDRICAL_SURFACE('',#75831,0.1) ;
#7629=CYLINDRICAL_SURFACE('',#75834,0.1) ;
#7630=CYLINDRICAL_SURFACE('',#75840,0.1) ;
#7631=CYLINDRICAL_SURFACE('',#75843,0.1) ;
#7632=CYLINDRICAL_SURFACE('',#75845,0.0999999999999994) ;
#7633=CYLINDRICAL_SURFACE('',#75852,0.0999999999999994) ;
#7634=CYLINDRICAL_SURFACE('',#75854,0.1) ;
#7635=CYLINDRICAL_SURFACE('',#75856,0.1) ;
#7636=CYLINDRICAL_SURFACE('',#75860,0.1) ;
#7637=CYLINDRICAL_SURFACE('',#75863,0.1) ;
#7638=CYLINDRICAL_SURFACE('',#75865,0.1) ;
#7639=CYLINDRICAL_SURFACE('',#75868,0.1) ;
#7640=CYLINDRICAL_SURFACE('',#75874,0.1) ;
#7641=CYLINDRICAL_SURFACE('',#75877,0.1) ;
#7642=CYLINDRICAL_SURFACE('',#75879,0.0999999999999994) ;
#7643=CYLINDRICAL_SURFACE('',#75886,0.0999999999999994) ;
#7644=CYLINDRICAL_SURFACE('',#75888,0.1) ;
#7645=CYLINDRICAL_SURFACE('',#75890,0.1) ;
#7646=CYLINDRICAL_SURFACE('',#75894,0.1) ;
#7647=CYLINDRICAL_SURFACE('',#75897,0.1) ;
#7648=CYLINDRICAL_SURFACE('',#75899,0.1) ;
#7649=CYLINDRICAL_SURFACE('',#75902,0.1) ;
#7650=CYLINDRICAL_SURFACE('',#75908,0.1) ;
#7651=CYLINDRICAL_SURFACE('',#75911,0.1) ;
#7652=CYLINDRICAL_SURFACE('',#75913,0.0999999999999994) ;
#7653=CYLINDRICAL_SURFACE('',#75920,0.0999999999999994) ;
#7654=CYLINDRICAL_SURFACE('',#75922,0.1) ;
#7655=CYLINDRICAL_SURFACE('',#75924,0.1) ;
#7656=CYLINDRICAL_SURFACE('',#75928,0.1) ;
#7657=CYLINDRICAL_SURFACE('',#75931,0.1) ;
#7658=CYLINDRICAL_SURFACE('',#75933,0.099999999999999) ;
#7659=CYLINDRICAL_SURFACE('',#75936,0.1) ;
#7660=CYLINDRICAL_SURFACE('',#75942,0.099999999999999) ;
#7661=CYLINDRICAL_SURFACE('',#75945,0.1) ;
#7662=CYLINDRICAL_SURFACE('',#75947,0.0999999999999994) ;
#7663=CYLINDRICAL_SURFACE('',#75954,0.0999999999999994) ;
#7664=CYLINDRICAL_SURFACE('',#75956,0.1) ;
#7665=CYLINDRICAL_SURFACE('',#75958,0.099999999999999) ;
#7666=CYLINDRICAL_SURFACE('',#75962,0.1) ;
#7667=CYLINDRICAL_SURFACE('',#75965,0.099999999999999) ;
#7668=CYLINDRICAL_SURFACE('',#75967,0.0999999999999989) ;
#7669=CYLINDRICAL_SURFACE('',#75970,0.1) ;
#7670=CYLINDRICAL_SURFACE('',#75976,0.0999999999999989) ;
#7671=CYLINDRICAL_SURFACE('',#75979,0.1) ;
#7672=CYLINDRICAL_SURFACE('',#75981,0.0999999999999994) ;
#7673=CYLINDRICAL_SURFACE('',#75988,0.0999999999999994) ;
#7674=CYLINDRICAL_SURFACE('',#75990,0.1) ;
#7675=CYLINDRICAL_SURFACE('',#75992,0.0999999999999989) ;
#7676=CYLINDRICAL_SURFACE('',#75996,0.1) ;
#7677=CYLINDRICAL_SURFACE('',#75999,0.0999999999999989) ;
#7678=CYLINDRICAL_SURFACE('',#76001,0.099999999999999) ;
#7679=CYLINDRICAL_SURFACE('',#76004,0.1) ;
#7680=CYLINDRICAL_SURFACE('',#76010,0.099999999999999) ;
#7681=CYLINDRICAL_SURFACE('',#76013,0.1) ;
#7682=CYLINDRICAL_SURFACE('',#76015,0.0999999999999994) ;
#7683=CYLINDRICAL_SURFACE('',#76022,0.0999999999999994) ;
#7684=CYLINDRICAL_SURFACE('',#76024,0.1) ;
#7685=CYLINDRICAL_SURFACE('',#76026,0.099999999999999) ;
#7686=CYLINDRICAL_SURFACE('',#76030,0.1) ;
#7687=CYLINDRICAL_SURFACE('',#76033,0.099999999999999) ;
#7688=CYLINDRICAL_SURFACE('',#76035,0.0999999999999989) ;
#7689=CYLINDRICAL_SURFACE('',#76038,0.1) ;
#7690=CYLINDRICAL_SURFACE('',#76044,0.0999999999999989) ;
#7691=CYLINDRICAL_SURFACE('',#76047,0.1) ;
#7692=CYLINDRICAL_SURFACE('',#76049,0.0999999999999994) ;
#7693=CYLINDRICAL_SURFACE('',#76056,0.0999999999999994) ;
#7694=CYLINDRICAL_SURFACE('',#76058,0.1) ;
#7695=CYLINDRICAL_SURFACE('',#76060,0.0999999999999989) ;
#7696=CYLINDRICAL_SURFACE('',#76064,0.1) ;
#7697=CYLINDRICAL_SURFACE('',#76067,0.0999999999999989) ;
#7698=CYLINDRICAL_SURFACE('',#76069,0.099999999999999) ;
#7699=CYLINDRICAL_SURFACE('',#76072,0.1) ;
#7700=CYLINDRICAL_SURFACE('',#76078,0.099999999999999) ;
#7701=CYLINDRICAL_SURFACE('',#76081,0.1) ;
#7702=CYLINDRICAL_SURFACE('',#76083,0.0999999999999994) ;
#7703=CYLINDRICAL_SURFACE('',#76090,0.0999999999999994) ;
#7704=CYLINDRICAL_SURFACE('',#76092,0.1) ;
#7705=CYLINDRICAL_SURFACE('',#76094,0.099999999999999) ;
#7706=CYLINDRICAL_SURFACE('',#76098,0.1) ;
#7707=CYLINDRICAL_SURFACE('',#76101,0.099999999999999) ;
#7708=CYLINDRICAL_SURFACE('',#76103,0.0999999999999989) ;
#7709=CYLINDRICAL_SURFACE('',#76106,0.1) ;
#7710=CYLINDRICAL_SURFACE('',#76112,0.0999999999999989) ;
#7711=CYLINDRICAL_SURFACE('',#76115,0.1) ;
#7712=CYLINDRICAL_SURFACE('',#76117,0.0999999999999994) ;
#7713=CYLINDRICAL_SURFACE('',#76124,0.0999999999999994) ;
#7714=CYLINDRICAL_SURFACE('',#76126,0.1) ;
#7715=CYLINDRICAL_SURFACE('',#76128,0.0999999999999989) ;
#7716=CYLINDRICAL_SURFACE('',#76132,0.1) ;
#7717=CYLINDRICAL_SURFACE('',#76135,0.0999999999999989) ;
#7718=CYLINDRICAL_SURFACE('',#76137,0.099999999999999) ;
#7719=CYLINDRICAL_SURFACE('',#76140,0.1) ;
#7720=CYLINDRICAL_SURFACE('',#76146,0.099999999999999) ;
#7721=CYLINDRICAL_SURFACE('',#76149,0.1) ;
#7722=CYLINDRICAL_SURFACE('',#76151,0.0999999999999994) ;
#7723=CYLINDRICAL_SURFACE('',#76158,0.0999999999999994) ;
#7724=CYLINDRICAL_SURFACE('',#76160,0.1) ;
#7725=CYLINDRICAL_SURFACE('',#76162,0.099999999999999) ;
#7726=CYLINDRICAL_SURFACE('',#76166,0.1) ;
#7727=CYLINDRICAL_SURFACE('',#76169,0.099999999999999) ;
#7728=CYLINDRICAL_SURFACE('',#76171,0.0999999999999989) ;
#7729=CYLINDRICAL_SURFACE('',#76174,0.1) ;
#7730=CYLINDRICAL_SURFACE('',#76180,0.0999999999999989) ;
#7731=CYLINDRICAL_SURFACE('',#76183,0.1) ;
#7732=CYLINDRICAL_SURFACE('',#76185,0.0999999999999994) ;
#7733=CYLINDRICAL_SURFACE('',#76192,0.0999999999999994) ;
#7734=CYLINDRICAL_SURFACE('',#76194,0.1) ;
#7735=CYLINDRICAL_SURFACE('',#76196,0.0999999999999989) ;
#7736=CYLINDRICAL_SURFACE('',#76200,0.1) ;
#7737=CYLINDRICAL_SURFACE('',#76203,0.0999999999999989) ;
#7738=CYLINDRICAL_SURFACE('',#76205,0.099999999999999) ;
#7739=CYLINDRICAL_SURFACE('',#76208,0.1) ;
#7740=CYLINDRICAL_SURFACE('',#76214,0.099999999999999) ;
#7741=CYLINDRICAL_SURFACE('',#76217,0.1) ;
#7742=CYLINDRICAL_SURFACE('',#76219,0.100000000000003) ;
#7743=CYLINDRICAL_SURFACE('',#76226,0.100000000000003) ;
#7744=CYLINDRICAL_SURFACE('',#76228,0.1) ;
#7745=CYLINDRICAL_SURFACE('',#76230,0.099999999999999) ;
#7746=CYLINDRICAL_SURFACE('',#76234,0.1) ;
#7747=CYLINDRICAL_SURFACE('',#76237,0.099999999999999) ;
#7748=CYLINDRICAL_SURFACE('',#76239,0.0999999999999989) ;
#7749=CYLINDRICAL_SURFACE('',#76242,0.1) ;
#7750=CYLINDRICAL_SURFACE('',#76248,0.0999999999999989) ;
#7751=CYLINDRICAL_SURFACE('',#76251,0.1) ;
#7752=CYLINDRICAL_SURFACE('',#76253,0.100000000000003) ;
#7753=CYLINDRICAL_SURFACE('',#76260,0.100000000000003) ;
#7754=CYLINDRICAL_SURFACE('',#76262,0.1) ;
#7755=CYLINDRICAL_SURFACE('',#76264,0.0999999999999989) ;
#7756=CYLINDRICAL_SURFACE('',#76268,0.1) ;
#7757=CYLINDRICAL_SURFACE('',#76271,0.0999999999999989) ;
#7758=CYLINDRICAL_SURFACE('',#76275,0.1) ;
#7759=CYLINDRICAL_SURFACE('',#76279,0.1) ;
#7760=CYLINDRICAL_SURFACE('',#76283,0.1) ;
#7761=CYLINDRICAL_SURFACE('',#76288,0.1) ;
#7762=CYLINDRICAL_SURFACE('',#76292,0.1) ;
#7763=CYLINDRICAL_SURFACE('',#76296,0.1) ;
#7764=CYLINDRICAL_SURFACE('',#76299,0.1) ;
#7765=CYLINDRICAL_SURFACE('',#76303,0.1) ;
#7766=CYLINDRICAL_SURFACE('',#76307,0.1) ;
#7767=CYLINDRICAL_SURFACE('',#76308,0.1) ;
#7768=CYLINDRICAL_SURFACE('',#76312,0.1) ;
#7769=CYLINDRICAL_SURFACE('',#76314,0.1) ;
#7770=CYLINDRICAL_SURFACE('',#76319,0.1) ;
#7771=CYLINDRICAL_SURFACE('',#76323,0.1) ;
#7772=CYLINDRICAL_SURFACE('',#76327,0.1) ;
#7773=CYLINDRICAL_SURFACE('',#76332,0.1) ;
#7774=CYLINDRICAL_SURFACE('',#76336,0.1) ;
#7775=CYLINDRICAL_SURFACE('',#76340,0.1) ;
#7776=CYLINDRICAL_SURFACE('',#76343,0.1) ;
#7777=CYLINDRICAL_SURFACE('',#76347,0.1) ;
#7778=CYLINDRICAL_SURFACE('',#76351,0.1) ;
#7779=CYLINDRICAL_SURFACE('',#76352,0.1) ;
#7780=CYLINDRICAL_SURFACE('',#76356,0.1) ;
#7781=CYLINDRICAL_SURFACE('',#76358,0.1) ;
#7782=CYLINDRICAL_SURFACE('',#76363,0.1) ;
#7783=CYLINDRICAL_SURFACE('',#76367,0.1) ;
#7784=CYLINDRICAL_SURFACE('',#76371,0.1) ;
#7785=CYLINDRICAL_SURFACE('',#76376,0.1) ;
#7786=CYLINDRICAL_SURFACE('',#76380,0.1) ;
#7787=CYLINDRICAL_SURFACE('',#76384,0.1) ;
#7788=CYLINDRICAL_SURFACE('',#76387,0.1) ;
#7789=CYLINDRICAL_SURFACE('',#76391,0.1) ;
#7790=CYLINDRICAL_SURFACE('',#76395,0.1) ;
#7791=CYLINDRICAL_SURFACE('',#76396,0.1) ;
#7792=CYLINDRICAL_SURFACE('',#76400,0.1) ;
#7793=CYLINDRICAL_SURFACE('',#76402,0.1) ;
#7794=CYLINDRICAL_SURFACE('',#76407,0.1) ;
#7795=CYLINDRICAL_SURFACE('',#76411,0.1) ;
#7796=CYLINDRICAL_SURFACE('',#76415,0.1) ;
#7797=CYLINDRICAL_SURFACE('',#76420,0.1) ;
#7798=CYLINDRICAL_SURFACE('',#76424,0.1) ;
#7799=CYLINDRICAL_SURFACE('',#76428,0.1) ;
#7800=CYLINDRICAL_SURFACE('',#76431,0.1) ;
#7801=CYLINDRICAL_SURFACE('',#76435,0.1) ;
#7802=CYLINDRICAL_SURFACE('',#76439,0.1) ;
#7803=CYLINDRICAL_SURFACE('',#76440,0.1) ;
#7804=CYLINDRICAL_SURFACE('',#76444,0.1) ;
#7805=CYLINDRICAL_SURFACE('',#76446,0.1) ;
#7806=CYLINDRICAL_SURFACE('',#76451,0.1) ;
#7807=CYLINDRICAL_SURFACE('',#76455,0.1) ;
#7808=CYLINDRICAL_SURFACE('',#76459,0.1) ;
#7809=CYLINDRICAL_SURFACE('',#76464,0.1) ;
#7810=CYLINDRICAL_SURFACE('',#76468,0.1) ;
#7811=CYLINDRICAL_SURFACE('',#76472,0.1) ;
#7812=CYLINDRICAL_SURFACE('',#76475,0.1) ;
#7813=CYLINDRICAL_SURFACE('',#76479,0.1) ;
#7814=CYLINDRICAL_SURFACE('',#76483,0.1) ;
#7815=CYLINDRICAL_SURFACE('',#76484,0.1) ;
#7816=CYLINDRICAL_SURFACE('',#76488,0.1) ;
#7817=CYLINDRICAL_SURFACE('',#76490,0.1) ;
#7818=CYLINDRICAL_SURFACE('',#76495,0.1) ;
#7819=CYLINDRICAL_SURFACE('',#76499,0.1) ;
#7820=CYLINDRICAL_SURFACE('',#76503,0.1) ;
#7821=CYLINDRICAL_SURFACE('',#76508,0.1) ;
#7822=CYLINDRICAL_SURFACE('',#76512,0.1) ;
#7823=CYLINDRICAL_SURFACE('',#76516,0.1) ;
#7824=CYLINDRICAL_SURFACE('',#76519,0.1) ;
#7825=CYLINDRICAL_SURFACE('',#76523,0.1) ;
#7826=CYLINDRICAL_SURFACE('',#76527,0.1) ;
#7827=CYLINDRICAL_SURFACE('',#76528,0.1) ;
#7828=CYLINDRICAL_SURFACE('',#76532,0.1) ;
#7829=CYLINDRICAL_SURFACE('',#76534,0.1) ;
#7830=CYLINDRICAL_SURFACE('',#76539,0.1) ;
#7831=CYLINDRICAL_SURFACE('',#76543,0.1) ;
#7832=CYLINDRICAL_SURFACE('',#76547,0.1) ;
#7833=CYLINDRICAL_SURFACE('',#76552,0.1) ;
#7834=CYLINDRICAL_SURFACE('',#76556,0.1) ;
#7835=CYLINDRICAL_SURFACE('',#76560,0.1) ;
#7836=CYLINDRICAL_SURFACE('',#76563,0.1) ;
#7837=CYLINDRICAL_SURFACE('',#76567,0.1) ;
#7838=CYLINDRICAL_SURFACE('',#76571,0.1) ;
#7839=CYLINDRICAL_SURFACE('',#76572,0.1) ;
#7840=CYLINDRICAL_SURFACE('',#76576,0.1) ;
#7841=CYLINDRICAL_SURFACE('',#76578,0.1) ;
#7842=CYLINDRICAL_SURFACE('',#76583,0.1) ;
#7843=CYLINDRICAL_SURFACE('',#76587,0.1) ;
#7844=CYLINDRICAL_SURFACE('',#76591,0.1) ;
#7845=CYLINDRICAL_SURFACE('',#76596,0.1) ;
#7846=CYLINDRICAL_SURFACE('',#76600,0.1) ;
#7847=CYLINDRICAL_SURFACE('',#76604,0.1) ;
#7848=CYLINDRICAL_SURFACE('',#76607,0.1) ;
#7849=CYLINDRICAL_SURFACE('',#76611,0.1) ;
#7850=CYLINDRICAL_SURFACE('',#76615,0.1) ;
#7851=CYLINDRICAL_SURFACE('',#76616,0.1) ;
#7852=CYLINDRICAL_SURFACE('',#76620,0.1) ;
#7853=CYLINDRICAL_SURFACE('',#76622,0.1) ;
#7854=CYLINDRICAL_SURFACE('',#76627,0.1) ;
#7855=CYLINDRICAL_SURFACE('',#76631,0.1) ;
#7856=CYLINDRICAL_SURFACE('',#76635,0.1) ;
#7857=CYLINDRICAL_SURFACE('',#76640,0.1) ;
#7858=CYLINDRICAL_SURFACE('',#76644,0.1) ;
#7859=CYLINDRICAL_SURFACE('',#76648,0.1) ;
#7860=CYLINDRICAL_SURFACE('',#76651,0.1) ;
#7861=CYLINDRICAL_SURFACE('',#76655,0.1) ;
#7862=CYLINDRICAL_SURFACE('',#76659,0.1) ;
#7863=CYLINDRICAL_SURFACE('',#76660,0.1) ;
#7864=CYLINDRICAL_SURFACE('',#76664,0.1) ;
#7865=CYLINDRICAL_SURFACE('',#76666,0.1) ;
#9806=LINE('',#113887,#13922) ;
#9807=LINE('',#113891,#13923) ;
#9808=LINE('',#113893,#13924) ;
#9809=LINE('',#113930,#13925) ;
#9810=LINE('',#113934,#13926) ;
#9811=LINE('',#113936,#13927) ;
#9812=LINE('',#113973,#13928) ;
#9813=LINE('',#113977,#13929) ;
#9814=LINE('',#113979,#13930) ;
#9815=LINE('',#114016,#13931) ;
#9816=LINE('',#114020,#13932) ;
#9817=LINE('',#114022,#13933) ;
#9818=LINE('',#114059,#13934) ;
#9819=LINE('',#114063,#13935) ;
#9820=LINE('',#114065,#13936) ;
#9821=LINE('',#114102,#13937) ;
#9822=LINE('',#114106,#13938) ;
#9823=LINE('',#114108,#13939) ;
#9824=LINE('',#114145,#13940) ;
#9825=LINE('',#114149,#13941) ;
#9826=LINE('',#114151,#13942) ;
#9827=LINE('',#114188,#13943) ;
#9828=LINE('',#114192,#13944) ;
#9829=LINE('',#114194,#13945) ;
#9830=LINE('',#114312,#13946) ;
#9831=LINE('',#114316,#13947) ;
#9832=LINE('',#114318,#13948) ;
#9833=LINE('',#114328,#13949) ;
#9834=LINE('',#114330,#13950) ;
#9835=LINE('',#114332,#13951) ;
#9836=LINE('',#114334,#13952) ;
#9837=LINE('',#114336,#13953) ;
#9838=LINE('',#114338,#13954) ;
#9839=LINE('',#114340,#13955) ;
#9840=LINE('',#114342,#13956) ;
#9841=LINE('',#114344,#13957) ;
#9842=LINE('',#114349,#13958) ;
#9843=LINE('',#114350,#13959) ;
#9844=LINE('',#114355,#13960) ;
#9845=LINE('',#114356,#13961) ;
#9846=LINE('',#114361,#13962) ;
#9847=LINE('',#114362,#13963) ;
#9848=LINE('',#114367,#13964) ;
#9849=LINE('',#114368,#13965) ;
#9850=LINE('',#114373,#13966) ;
#9851=LINE('',#114374,#13967) ;
#9852=LINE('',#114379,#13968) ;
#9853=LINE('',#114380,#13969) ;
#9854=LINE('',#114385,#13970) ;
#9855=LINE('',#114386,#13971) ;
#9856=LINE('',#114391,#13972) ;
#9857=LINE('',#114392,#13973) ;
#9858=LINE('',#114397,#13974) ;
#9859=LINE('',#114398,#13975) ;
#9860=LINE('',#114436,#13976) ;
#9861=LINE('',#114440,#13977) ;
#9862=LINE('',#114442,#13978) ;
#9863=LINE('',#114452,#13979) ;
#9864=LINE('',#114457,#13980) ;
#9865=LINE('',#114458,#13981) ;
#9866=LINE('',#114462,#13982) ;
#9867=LINE('',#114466,#13983) ;
#9868=LINE('',#114471,#13984) ;
#9869=LINE('',#114473,#13985) ;
#9870=LINE('',#114475,#13986) ;
#9871=LINE('',#114477,#13987) ;
#9872=LINE('',#114479,#13988) ;
#9873=LINE('',#114484,#13989) ;
#9874=LINE('',#114488,#13990) ;
#9875=LINE('',#114493,#13991) ;
#9876=LINE('',#114495,#13992) ;
#9877=LINE('',#114497,#13993) ;
#9878=LINE('',#114499,#13994) ;
#9879=LINE('',#114501,#13995) ;
#9880=LINE('',#114506,#13996) ;
#9881=LINE('',#114510,#13997) ;
#9882=LINE('',#114515,#13998) ;
#9883=LINE('',#114517,#13999) ;
#9884=LINE('',#114519,#14000) ;
#9885=LINE('',#114521,#14001) ;
#9886=LINE('',#114523,#14002) ;
#9887=LINE('',#114528,#14003) ;
#9888=LINE('',#114532,#14004) ;
#9889=LINE('',#114537,#14005) ;
#9890=LINE('',#114539,#14006) ;
#9891=LINE('',#114541,#14007) ;
#9892=LINE('',#114543,#14008) ;
#9893=LINE('',#114545,#14009) ;
#9894=LINE('',#114550,#14010) ;
#9895=LINE('',#114554,#14011) ;
#9896=LINE('',#114559,#14012) ;
#9897=LINE('',#114561,#14013) ;
#9898=LINE('',#114563,#14014) ;
#9899=LINE('',#114565,#14015) ;
#9900=LINE('',#114567,#14016) ;
#9901=LINE('',#114572,#14017) ;
#9902=LINE('',#114576,#14018) ;
#9903=LINE('',#114581,#14019) ;
#9904=LINE('',#114583,#14020) ;
#9905=LINE('',#114585,#14021) ;
#9906=LINE('',#114587,#14022) ;
#9907=LINE('',#114589,#14023) ;
#9908=LINE('',#114594,#14024) ;
#9909=LINE('',#114598,#14025) ;
#9910=LINE('',#114603,#14026) ;
#9911=LINE('',#114605,#14027) ;
#9912=LINE('',#114607,#14028) ;
#9913=LINE('',#114609,#14029) ;
#9914=LINE('',#114611,#14030) ;
#9915=LINE('',#114616,#14031) ;
#9916=LINE('',#114620,#14032) ;
#9917=LINE('',#114625,#14033) ;
#9918=LINE('',#114627,#14034) ;
#9919=LINE('',#114629,#14035) ;
#9920=LINE('',#114631,#14036) ;
#9921=LINE('',#114633,#14037) ;
#9922=LINE('',#114638,#14038) ;
#9923=LINE('',#114642,#14039) ;
#9924=LINE('',#114647,#14040) ;
#9925=LINE('',#114649,#14041) ;
#9926=LINE('',#114651,#14042) ;
#9927=LINE('',#114653,#14043) ;
#9928=LINE('',#114655,#14044) ;
#9929=LINE('',#114662,#14045) ;
#9930=LINE('',#114664,#14046) ;
#9931=LINE('',#114666,#14047) ;
#9932=LINE('',#114667,#14048) ;
#9933=LINE('',#114673,#14049) ;
#9934=LINE('',#114675,#14050) ;
#9935=LINE('',#114677,#14051) ;
#9936=LINE('',#114678,#14052) ;
#9937=LINE('',#114684,#14053) ;
#9938=LINE('',#114686,#14054) ;
#9939=LINE('',#114688,#14055) ;
#9940=LINE('',#114689,#14056) ;
#9941=LINE('',#114695,#14057) ;
#9942=LINE('',#114697,#14058) ;
#9943=LINE('',#114699,#14059) ;
#9944=LINE('',#114700,#14060) ;
#9945=LINE('',#114706,#14061) ;
#9946=LINE('',#114708,#14062) ;
#9947=LINE('',#114710,#14063) ;
#9948=LINE('',#114711,#14064) ;
#9949=LINE('',#114717,#14065) ;
#9950=LINE('',#114719,#14066) ;
#9951=LINE('',#114721,#14067) ;
#9952=LINE('',#114722,#14068) ;
#9953=LINE('',#114728,#14069) ;
#9954=LINE('',#114730,#14070) ;
#9955=LINE('',#114732,#14071) ;
#9956=LINE('',#114733,#14072) ;
#9957=LINE('',#114739,#14073) ;
#9958=LINE('',#114741,#14074) ;
#9959=LINE('',#114743,#14075) ;
#9960=LINE('',#114744,#14076) ;
#9961=LINE('',#114750,#14077) ;
#9962=LINE('',#114752,#14078) ;
#9963=LINE('',#114754,#14079) ;
#9964=LINE('',#114755,#14080) ;
#9965=LINE('',#114761,#14081) ;
#9966=LINE('',#114763,#14082) ;
#9967=LINE('',#114765,#14083) ;
#9968=LINE('',#114766,#14084) ;
#9969=LINE('',#114772,#14085) ;
#9970=LINE('',#114774,#14086) ;
#9971=LINE('',#114776,#14087) ;
#9972=LINE('',#114777,#14088) ;
#9973=LINE('',#114783,#14089) ;
#9974=LINE('',#114785,#14090) ;
#9975=LINE('',#114787,#14091) ;
#9976=LINE('',#114788,#14092) ;
#9977=LINE('',#114794,#14093) ;
#9978=LINE('',#114796,#14094) ;
#9979=LINE('',#114798,#14095) ;
#9980=LINE('',#114799,#14096) ;
#9981=LINE('',#114805,#14097) ;
#9982=LINE('',#114807,#14098) ;
#9983=LINE('',#114809,#14099) ;
#9984=LINE('',#114810,#14100) ;
#9985=LINE('',#114816,#14101) ;
#9986=LINE('',#114818,#14102) ;
#9987=LINE('',#114820,#14103) ;
#9988=LINE('',#114821,#14104) ;
#9989=LINE('',#114827,#14105) ;
#9990=LINE('',#114829,#14106) ;
#9991=LINE('',#114831,#14107) ;
#9992=LINE('',#114832,#14108) ;
#9993=LINE('',#114838,#14109) ;
#9994=LINE('',#114840,#14110) ;
#9995=LINE('',#114842,#14111) ;
#9996=LINE('',#114843,#14112) ;
#9997=LINE('',#114849,#14113) ;
#9998=LINE('',#114851,#14114) ;
#9999=LINE('',#114853,#14115) ;
#10000=LINE('',#114854,#14116) ;
#10001=LINE('',#114858,#14117) ;
#10002=LINE('',#114862,#14118) ;
#10003=LINE('',#114867,#14119) ;
#10004=LINE('',#114871,#14120) ;
#10005=LINE('',#114876,#14121) ;
#10006=LINE('',#114880,#14122) ;
#10007=LINE('',#114885,#14123) ;
#10008=LINE('',#114889,#14124) ;
#10009=LINE('',#114894,#14125) ;
#10010=LINE('',#114898,#14126) ;
#10011=LINE('',#114903,#14127) ;
#10012=LINE('',#114907,#14128) ;
#10013=LINE('',#114912,#14129) ;
#10014=LINE('',#114916,#14130) ;
#10015=LINE('',#114921,#14131) ;
#10016=LINE('',#114925,#14132) ;
#10017=LINE('',#114930,#14133) ;
#10018=LINE('',#114934,#14134) ;
#10019=LINE('',#114939,#14135) ;
#10020=LINE('',#114943,#14136) ;
#10021=LINE('',#114948,#14137) ;
#10022=LINE('',#114950,#14138) ;
#10023=LINE('',#114952,#14139) ;
#10024=LINE('',#114954,#14140) ;
#10025=LINE('',#114956,#14141) ;
#10026=LINE('',#114963,#14142) ;
#10027=LINE('',#114965,#14143) ;
#10028=LINE('',#114967,#14144) ;
#10029=LINE('',#114968,#14145) ;
#10030=LINE('',#114974,#14146) ;
#10031=LINE('',#114976,#14147) ;
#10032=LINE('',#114978,#14148) ;
#10033=LINE('',#114979,#14149) ;
#10034=LINE('',#114983,#14150) ;
#10035=LINE('',#114987,#14151) ;
#10036=LINE('',#114992,#14152) ;
#10037=LINE('',#114996,#14153) ;
#10038=LINE('',#115003,#14154) ;
#10039=LINE('',#115005,#14155) ;
#10040=LINE('',#115006,#14156) ;
#10041=LINE('',#115007,#14157) ;
#10042=LINE('',#115009,#14158) ;
#10043=LINE('',#115013,#14159) ;
#10044=LINE('',#115016,#14160) ;
#10045=LINE('',#115018,#14161) ;
#10046=LINE('',#115022,#14162) ;
#10047=LINE('',#115025,#14163) ;
#10048=LINE('',#115027,#14164) ;
#10049=LINE('',#115031,#14165) ;
#10050=LINE('',#115034,#14166) ;
#10051=LINE('',#115036,#14167) ;
#10052=LINE('',#115040,#14168) ;
#10053=LINE('',#115043,#14169) ;
#10054=LINE('',#115045,#14170) ;
#10055=LINE('',#115049,#14171) ;
#10056=LINE('',#115052,#14172) ;
#10057=LINE('',#115054,#14173) ;
#10058=LINE('',#115058,#14174) ;
#10059=LINE('',#115061,#14175) ;
#10060=LINE('',#115063,#14176) ;
#10061=LINE('',#115067,#14177) ;
#10062=LINE('',#115070,#14178) ;
#10063=LINE('',#115072,#14179) ;
#10064=LINE('',#115076,#14180) ;
#10065=LINE('',#115079,#14181) ;
#10066=LINE('',#115081,#14182) ;
#10067=LINE('',#115085,#14183) ;
#10068=LINE('',#115088,#14184) ;
#10069=LINE('',#115090,#14185) ;
#10070=LINE('',#115093,#14186) ;
#10071=LINE('',#115098,#14187) ;
#10072=LINE('',#115104,#14188) ;
#10073=LINE('',#115106,#14189) ;
#10074=LINE('',#115110,#14190) ;
#10075=LINE('',#115113,#14191) ;
#10076=LINE('',#115115,#14192) ;
#10077=LINE('',#115119,#14193) ;
#10078=LINE('',#115122,#14194) ;
#10079=LINE('',#115124,#14195) ;
#10080=LINE('',#115128,#14196) ;
#10081=LINE('',#115131,#14197) ;
#10082=LINE('',#115133,#14198) ;
#10083=LINE('',#115137,#14199) ;
#10084=LINE('',#115140,#14200) ;
#10085=LINE('',#115142,#14201) ;
#10086=LINE('',#115146,#14202) ;
#10087=LINE('',#115149,#14203) ;
#10088=LINE('',#115151,#14204) ;
#10089=LINE('',#115155,#14205) ;
#10090=LINE('',#115158,#14206) ;
#10091=LINE('',#115160,#14207) ;
#10092=LINE('',#115164,#14208) ;
#10093=LINE('',#115167,#14209) ;
#10094=LINE('',#115169,#14210) ;
#10095=LINE('',#115173,#14211) ;
#10096=LINE('',#115176,#14212) ;
#10097=LINE('',#115178,#14213) ;
#10098=LINE('',#115182,#14214) ;
#10099=LINE('',#115185,#14215) ;
#10100=LINE('',#115187,#14216) ;
#10101=LINE('',#115189,#14217) ;
#10102=LINE('',#115190,#14218) ;
#10103=LINE('',#115192,#14219) ;
#10104=LINE('',#115195,#14220) ;
#10105=LINE('',#115199,#14221) ;
#10106=LINE('',#115205,#14222) ;
#10107=LINE('',#115206,#14223) ;
#10108=LINE('',#115207,#14224) ;
#10109=LINE('',#115211,#14225) ;
#10110=LINE('',#115217,#14226) ;
#10111=LINE('',#115218,#14227) ;
#10112=LINE('',#115219,#14228) ;
#10113=LINE('',#115223,#14229) ;
#10114=LINE('',#115229,#14230) ;
#10115=LINE('',#115230,#14231) ;
#10116=LINE('',#115231,#14232) ;
#10117=LINE('',#115235,#14233) ;
#10118=LINE('',#115241,#14234) ;
#10119=LINE('',#115242,#14235) ;
#10120=LINE('',#115243,#14236) ;
#10121=LINE('',#115247,#14237) ;
#10122=LINE('',#115253,#14238) ;
#10123=LINE('',#115254,#14239) ;
#10124=LINE('',#115255,#14240) ;
#10125=LINE('',#115259,#14241) ;
#10126=LINE('',#115263,#14242) ;
#10127=LINE('',#115264,#14243) ;
#10128=LINE('',#115269,#14244) ;
#10129=LINE('',#115271,#14245) ;
#10130=LINE('',#115273,#14246) ;
#10131=LINE('',#115277,#14247) ;
#10132=LINE('',#115280,#14248) ;
#10133=LINE('',#115282,#14249) ;
#10134=LINE('',#115286,#14250) ;
#10135=LINE('',#115288,#14251) ;
#10136=LINE('',#115290,#14252) ;
#10137=LINE('',#115294,#14253) ;
#10138=LINE('',#115298,#14254) ;
#10139=LINE('',#115306,#14255) ;
#10140=LINE('',#115309,#14256) ;
#10141=LINE('',#115314,#14257) ;
#10142=LINE('',#115316,#14258) ;
#10143=LINE('',#115318,#14259) ;
#10144=LINE('',#115322,#14260) ;
#10145=LINE('',#115325,#14261) ;
#10146=LINE('',#115327,#14262) ;
#10147=LINE('',#115331,#14263) ;
#10148=LINE('',#115333,#14264) ;
#10149=LINE('',#115335,#14265) ;
#10150=LINE('',#115339,#14266) ;
#10151=LINE('',#115343,#14267) ;
#10152=LINE('',#115351,#14268) ;
#10153=LINE('',#115354,#14269) ;
#10154=LINE('',#115359,#14270) ;
#10155=LINE('',#115361,#14271) ;
#10156=LINE('',#115363,#14272) ;
#10157=LINE('',#115367,#14273) ;
#10158=LINE('',#115370,#14274) ;
#10159=LINE('',#115372,#14275) ;
#10160=LINE('',#115376,#14276) ;
#10161=LINE('',#115378,#14277) ;
#10162=LINE('',#115380,#14278) ;
#10163=LINE('',#115384,#14279) ;
#10164=LINE('',#115388,#14280) ;
#10165=LINE('',#115396,#14281) ;
#10166=LINE('',#115399,#14282) ;
#10167=LINE('',#115404,#14283) ;
#10168=LINE('',#115406,#14284) ;
#10169=LINE('',#115408,#14285) ;
#10170=LINE('',#115412,#14286) ;
#10171=LINE('',#115415,#14287) ;
#10172=LINE('',#115417,#14288) ;
#10173=LINE('',#115421,#14289) ;
#10174=LINE('',#115423,#14290) ;
#10175=LINE('',#115425,#14291) ;
#10176=LINE('',#115429,#14292) ;
#10177=LINE('',#115433,#14293) ;
#10178=LINE('',#115441,#14294) ;
#10179=LINE('',#115444,#14295) ;
#10180=LINE('',#115449,#14296) ;
#10181=LINE('',#115451,#14297) ;
#10182=LINE('',#115453,#14298) ;
#10183=LINE('',#115457,#14299) ;
#10184=LINE('',#115460,#14300) ;
#10185=LINE('',#115462,#14301) ;
#10186=LINE('',#115466,#14302) ;
#10187=LINE('',#115468,#14303) ;
#10188=LINE('',#115470,#14304) ;
#10189=LINE('',#115474,#14305) ;
#10190=LINE('',#115478,#14306) ;
#10191=LINE('',#115486,#14307) ;
#10192=LINE('',#115489,#14308) ;
#10193=LINE('',#115494,#14309) ;
#10194=LINE('',#115496,#14310) ;
#10195=LINE('',#115498,#14311) ;
#10196=LINE('',#115502,#14312) ;
#10197=LINE('',#115505,#14313) ;
#10198=LINE('',#115507,#14314) ;
#10199=LINE('',#115511,#14315) ;
#10200=LINE('',#115513,#14316) ;
#10201=LINE('',#115515,#14317) ;
#10202=LINE('',#115519,#14318) ;
#10203=LINE('',#115523,#14319) ;
#10204=LINE('',#115531,#14320) ;
#10205=LINE('',#115534,#14321) ;
#10206=LINE('',#115539,#14322) ;
#10207=LINE('',#115541,#14323) ;
#10208=LINE('',#115543,#14324) ;
#10209=LINE('',#115547,#14325) ;
#10210=LINE('',#115550,#14326) ;
#10211=LINE('',#115552,#14327) ;
#10212=LINE('',#115556,#14328) ;
#10213=LINE('',#115558,#14329) ;
#10214=LINE('',#115560,#14330) ;
#10215=LINE('',#115564,#14331) ;
#10216=LINE('',#115568,#14332) ;
#10217=LINE('',#115576,#14333) ;
#10218=LINE('',#115579,#14334) ;
#10219=LINE('',#115584,#14335) ;
#10220=LINE('',#115586,#14336) ;
#10221=LINE('',#115588,#14337) ;
#10222=LINE('',#115592,#14338) ;
#10223=LINE('',#115595,#14339) ;
#10224=LINE('',#115597,#14340) ;
#10225=LINE('',#115601,#14341) ;
#10226=LINE('',#115603,#14342) ;
#10227=LINE('',#115605,#14343) ;
#10228=LINE('',#115609,#14344) ;
#10229=LINE('',#115613,#14345) ;
#10230=LINE('',#115621,#14346) ;
#10231=LINE('',#115624,#14347) ;
#10232=LINE('',#115629,#14348) ;
#10233=LINE('',#115631,#14349) ;
#10234=LINE('',#115633,#14350) ;
#10235=LINE('',#115637,#14351) ;
#10236=LINE('',#115640,#14352) ;
#10237=LINE('',#115642,#14353) ;
#10238=LINE('',#115646,#14354) ;
#10239=LINE('',#115648,#14355) ;
#10240=LINE('',#115650,#14356) ;
#10241=LINE('',#115654,#14357) ;
#10242=LINE('',#115658,#14358) ;
#10243=LINE('',#115666,#14359) ;
#10244=LINE('',#115669,#14360) ;
#10245=LINE('',#115674,#14361) ;
#10246=LINE('',#115676,#14362) ;
#10247=LINE('',#115678,#14363) ;
#10248=LINE('',#115682,#14364) ;
#10249=LINE('',#115685,#14365) ;
#10250=LINE('',#115687,#14366) ;
#10251=LINE('',#115691,#14367) ;
#10252=LINE('',#115693,#14368) ;
#10253=LINE('',#115695,#14369) ;
#10254=LINE('',#115699,#14370) ;
#10255=LINE('',#115703,#14371) ;
#10256=LINE('',#115711,#14372) ;
#10257=LINE('',#115714,#14373) ;
#10258=LINE('',#115718,#14374) ;
#10259=LINE('',#115720,#14375) ;
#10260=LINE('',#115722,#14376) ;
#10261=LINE('',#115724,#14377) ;
#10262=LINE('',#115728,#14378) ;
#10263=LINE('',#115730,#14379) ;
#10264=LINE('',#115732,#14380) ;
#10265=LINE('',#115735,#14381) ;
#10266=LINE('',#115739,#14382) ;
#10267=LINE('',#115741,#14383) ;
#10268=LINE('',#115743,#14384) ;
#10269=LINE('',#115745,#14385) ;
#10270=LINE('',#115749,#14386) ;
#10271=LINE('',#115751,#14387) ;
#10272=LINE('',#115753,#14388) ;
#10273=LINE('',#115756,#14389) ;
#10274=LINE('',#115760,#14390) ;
#10275=LINE('',#115762,#14391) ;
#10276=LINE('',#115764,#14392) ;
#10277=LINE('',#115766,#14393) ;
#10278=LINE('',#115768,#14394) ;
#10279=LINE('',#115770,#14395) ;
#10280=LINE('',#115774,#14396) ;
#10281=LINE('',#115777,#14397) ;
#10282=LINE('',#115781,#14398) ;
#10283=LINE('',#115783,#14399) ;
#10284=LINE('',#115785,#14400) ;
#10285=LINE('',#115786,#14401) ;
#10286=LINE('',#115789,#14402) ;
#10287=LINE('',#115791,#14403) ;
#10288=LINE('',#115792,#14404) ;
#10289=LINE('',#115796,#14405) ;
#10290=LINE('',#115798,#14406) ;
#10291=LINE('',#115800,#14407) ;
#10292=LINE('',#115801,#14408) ;
#10293=LINE('',#115805,#14409) ;
#10294=LINE('',#115807,#14410) ;
#10295=LINE('',#115809,#14411) ;
#10296=LINE('',#115810,#14412) ;
#10297=LINE('',#115814,#14413) ;
#10298=LINE('',#115816,#14414) ;
#10299=LINE('',#115818,#14415) ;
#10300=LINE('',#115819,#14416) ;
#10301=LINE('',#115823,#14417) ;
#10302=LINE('',#115827,#14418) ;
#10303=LINE('',#115831,#14419) ;
#10304=LINE('',#115833,#14420) ;
#10305=LINE('',#115834,#14421) ;
#10306=LINE('',#115839,#14422) ;
#10307=LINE('',#115843,#14423) ;
#10308=LINE('',#115845,#14424) ;
#10309=LINE('',#115846,#14425) ;
#10310=LINE('',#115851,#14426) ;
#10311=LINE('',#115854,#14427) ;
#10312=LINE('',#115856,#14428) ;
#10313=LINE('',#115857,#14429) ;
#10314=LINE('',#115860,#14430) ;
#10315=LINE('',#115863,#14431) ;
#10316=LINE('',#115864,#14432) ;
#10317=LINE('',#115867,#14433) ;
#10318=LINE('',#115869,#14434) ;
#10319=LINE('',#115870,#14435) ;
#10320=LINE('',#115875,#14436) ;
#10321=LINE('',#115879,#14437) ;
#10322=LINE('',#115881,#14438) ;
#10323=LINE('',#115882,#14439) ;
#10324=LINE('',#115887,#14440) ;
#10325=LINE('',#115891,#14441) ;
#10326=LINE('',#115893,#14442) ;
#10327=LINE('',#115894,#14443) ;
#10328=LINE('',#115899,#14444) ;
#10329=LINE('',#115903,#14445) ;
#10330=LINE('',#115905,#14446) ;
#10331=LINE('',#115906,#14447) ;
#10332=LINE('',#115911,#14448) ;
#10333=LINE('',#115915,#14449) ;
#10334=LINE('',#115917,#14450) ;
#10335=LINE('',#115918,#14451) ;
#10336=LINE('',#115923,#14452) ;
#10337=LINE('',#115927,#14453) ;
#10338=LINE('',#115929,#14454) ;
#10339=LINE('',#115930,#14455) ;
#10340=LINE('',#115935,#14456) ;
#10341=LINE('',#115941,#14457) ;
#10342=LINE('',#115947,#14458) ;
#10343=LINE('',#115951,#14459) ;
#10344=LINE('',#115953,#14460) ;
#10345=LINE('',#115954,#14461) ;
#10346=LINE('',#115959,#14462) ;
#10347=LINE('',#115963,#14463) ;
#10348=LINE('',#115965,#14464) ;
#10349=LINE('',#115966,#14465) ;
#10350=LINE('',#115971,#14466) ;
#10351=LINE('',#115974,#14467) ;
#10352=LINE('',#115975,#14468) ;
#10353=LINE('',#115981,#14469) ;
#10354=LINE('',#115985,#14470) ;
#10355=LINE('',#115987,#14471) ;
#10356=LINE('',#115989,#14472) ;
#10357=LINE('',#115993,#14473) ;
#10358=LINE('',#115995,#14474) ;
#10359=LINE('',#115997,#14475) ;
#10360=LINE('',#116001,#14476) ;
#10361=LINE('',#116005,#14477) ;
#10362=LINE('',#116007,#14478) ;
#10363=LINE('',#116008,#14479) ;
#10364=LINE('',#116010,#14480) ;
#10365=LINE('',#116011,#14481) ;
#10366=LINE('',#116015,#14482) ;
#10367=LINE('',#116019,#14483) ;
#10368=LINE('',#116023,#14484) ;
#10369=LINE('',#116027,#14485) ;
#10370=LINE('',#116055,#14486) ;
#10371=LINE('',#116112,#14487) ;
#10372=LINE('',#116137,#14488) ;
#10373=LINE('',#116169,#14489) ;
#10374=LINE('',#116195,#14490) ;
#10375=LINE('',#116376,#14491) ;
#10376=LINE('',#116378,#14492) ;
#10377=LINE('',#116380,#14493) ;
#10378=LINE('',#116381,#14494) ;
#10379=LINE('',#116385,#14495) ;
#10380=LINE('',#116387,#14496) ;
#10381=LINE('',#116389,#14497) ;
#10382=LINE('',#116390,#14498) ;
#10383=LINE('',#116394,#14499) ;
#10384=LINE('',#116396,#14500) ;
#10385=LINE('',#116398,#14501) ;
#10386=LINE('',#116399,#14502) ;
#10387=LINE('',#116403,#14503) ;
#10388=LINE('',#116405,#14504) ;
#10389=LINE('',#116407,#14505) ;
#10390=LINE('',#116408,#14506) ;
#10391=LINE('',#116412,#14507) ;
#10392=LINE('',#116414,#14508) ;
#10393=LINE('',#116416,#14509) ;
#10394=LINE('',#116417,#14510) ;
#10395=LINE('',#116421,#14511) ;
#10396=LINE('',#116426,#14512) ;
#10397=LINE('',#116427,#14513) ;
#10398=LINE('',#116431,#14514) ;
#10399=LINE('',#116436,#14515) ;
#10400=LINE('',#116437,#14516) ;
#10401=LINE('',#116447,#14517) ;
#10402=LINE('',#116449,#14518) ;
#10403=LINE('',#116451,#14519) ;
#10404=LINE('',#116452,#14520) ;
#10405=LINE('',#116456,#14521) ;
#10406=LINE('',#116457,#14522) ;
#10407=LINE('',#116458,#14523) ;
#10408=LINE('',#116461,#14524) ;
#10409=LINE('',#116463,#14525) ;
#10410=LINE('',#116464,#14526) ;
#10411=LINE('',#116468,#14527) ;
#10412=LINE('',#116470,#14528) ;
#10413=LINE('',#116472,#14529) ;
#10414=LINE('',#116473,#14530) ;
#10415=LINE('',#116477,#14531) ;
#10416=LINE('',#116479,#14532) ;
#10417=LINE('',#116481,#14533) ;
#10418=LINE('',#116482,#14534) ;
#10419=LINE('',#116486,#14535) ;
#10420=LINE('',#116487,#14536) ;
#10421=LINE('',#116488,#14537) ;
#10422=LINE('',#116491,#14538) ;
#10423=LINE('',#116493,#14539) ;
#10424=LINE('',#116494,#14540) ;
#10425=LINE('',#116498,#14541) ;
#10426=LINE('',#116500,#14542) ;
#10427=LINE('',#116502,#14543) ;
#10428=LINE('',#116503,#14544) ;
#10429=LINE('',#116507,#14545) ;
#10430=LINE('',#116509,#14546) ;
#10431=LINE('',#116511,#14547) ;
#10432=LINE('',#116512,#14548) ;
#10433=LINE('',#116516,#14549) ;
#10434=LINE('',#116518,#14550) ;
#10435=LINE('',#116520,#14551) ;
#10436=LINE('',#116521,#14552) ;
#10437=LINE('',#116525,#14553) ;
#10438=LINE('',#116527,#14554) ;
#10439=LINE('',#116529,#14555) ;
#10440=LINE('',#116530,#14556) ;
#10441=LINE('',#116646,#14557) ;
#10442=LINE('',#116648,#14558) ;
#10443=LINE('',#116650,#14559) ;
#10444=LINE('',#116652,#14560) ;
#10445=LINE('',#116654,#14561) ;
#10446=LINE('',#116656,#14562) ;
#10447=LINE('',#116660,#14563) ;
#10448=LINE('',#116663,#14564) ;
#10449=LINE('',#116667,#14565) ;
#10450=LINE('',#116669,#14566) ;
#10451=LINE('',#116671,#14567) ;
#10452=LINE('',#116673,#14568) ;
#10453=LINE('',#116675,#14569) ;
#10454=LINE('',#116677,#14570) ;
#10455=LINE('',#116681,#14571) ;
#10456=LINE('',#116684,#14572) ;
#10457=LINE('',#116688,#14573) ;
#10458=LINE('',#116690,#14574) ;
#10459=LINE('',#116692,#14575) ;
#10460=LINE('',#116694,#14576) ;
#10461=LINE('',#116696,#14577) ;
#10462=LINE('',#116698,#14578) ;
#10463=LINE('',#116702,#14579) ;
#10464=LINE('',#116705,#14580) ;
#10465=LINE('',#116709,#14581) ;
#10466=LINE('',#116711,#14582) ;
#10467=LINE('',#116713,#14583) ;
#10468=LINE('',#116715,#14584) ;
#10469=LINE('',#116717,#14585) ;
#10470=LINE('',#116719,#14586) ;
#10471=LINE('',#116723,#14587) ;
#10472=LINE('',#116726,#14588) ;
#10473=LINE('',#116730,#14589) ;
#10474=LINE('',#116732,#14590) ;
#10475=LINE('',#116734,#14591) ;
#10476=LINE('',#116736,#14592) ;
#10477=LINE('',#116738,#14593) ;
#10478=LINE('',#116740,#14594) ;
#10479=LINE('',#116744,#14595) ;
#10480=LINE('',#116747,#14596) ;
#10481=LINE('',#116751,#14597) ;
#10482=LINE('',#116753,#14598) ;
#10483=LINE('',#116755,#14599) ;
#10484=LINE('',#116757,#14600) ;
#10485=LINE('',#116759,#14601) ;
#10486=LINE('',#116761,#14602) ;
#10487=LINE('',#116765,#14603) ;
#10488=LINE('',#116768,#14604) ;
#10489=LINE('',#116772,#14605) ;
#10490=LINE('',#116774,#14606) ;
#10491=LINE('',#116776,#14607) ;
#10492=LINE('',#116778,#14608) ;
#10493=LINE('',#116780,#14609) ;
#10494=LINE('',#116782,#14610) ;
#10495=LINE('',#116786,#14611) ;
#10496=LINE('',#116789,#14612) ;
#10497=LINE('',#116793,#14613) ;
#10498=LINE('',#116795,#14614) ;
#10499=LINE('',#116797,#14615) ;
#10500=LINE('',#116799,#14616) ;
#10501=LINE('',#116801,#14617) ;
#10502=LINE('',#116803,#14618) ;
#10503=LINE('',#116807,#14619) ;
#10504=LINE('',#116810,#14620) ;
#10505=LINE('',#116814,#14621) ;
#10506=LINE('',#116816,#14622) ;
#10507=LINE('',#116818,#14623) ;
#10508=LINE('',#116820,#14624) ;
#10509=LINE('',#116822,#14625) ;
#10510=LINE('',#116824,#14626) ;
#10511=LINE('',#116828,#14627) ;
#10512=LINE('',#116831,#14628) ;
#10513=LINE('',#116835,#14629) ;
#10514=LINE('',#116837,#14630) ;
#10515=LINE('',#116839,#14631) ;
#10516=LINE('',#116840,#14632) ;
#10517=LINE('',#116843,#14633) ;
#10518=LINE('',#116845,#14634) ;
#10519=LINE('',#116846,#14635) ;
#10520=LINE('',#116850,#14636) ;
#10521=LINE('',#116852,#14637) ;
#10522=LINE('',#116854,#14638) ;
#10523=LINE('',#116855,#14639) ;
#10524=LINE('',#116859,#14640) ;
#10525=LINE('',#116861,#14641) ;
#10526=LINE('',#116863,#14642) ;
#10527=LINE('',#116864,#14643) ;
#10528=LINE('',#116868,#14644) ;
#10529=LINE('',#116870,#14645) ;
#10530=LINE('',#116872,#14646) ;
#10531=LINE('',#116873,#14647) ;
#10532=LINE('',#116877,#14648) ;
#10533=LINE('',#116879,#14649) ;
#10534=LINE('',#116881,#14650) ;
#10535=LINE('',#116882,#14651) ;
#10536=LINE('',#116885,#14652) ;
#10537=LINE('',#116887,#14653) ;
#10538=LINE('',#116888,#14654) ;
#10539=LINE('',#116892,#14655) ;
#10540=LINE('',#116894,#14656) ;
#10541=LINE('',#116896,#14657) ;
#10542=LINE('',#116897,#14658) ;
#10543=LINE('',#116901,#14659) ;
#10544=LINE('',#116903,#14660) ;
#10545=LINE('',#116905,#14661) ;
#10546=LINE('',#116906,#14662) ;
#10547=LINE('',#116910,#14663) ;
#10548=LINE('',#116912,#14664) ;
#10549=LINE('',#116914,#14665) ;
#10550=LINE('',#116915,#14666) ;
#10551=LINE('',#116919,#14667) ;
#10552=LINE('',#116921,#14668) ;
#10553=LINE('',#116923,#14669) ;
#10554=LINE('',#116924,#14670) ;
#10555=LINE('',#116927,#14671) ;
#10556=LINE('',#116929,#14672) ;
#10557=LINE('',#116930,#14673) ;
#10558=LINE('',#116934,#14674) ;
#10559=LINE('',#116936,#14675) ;
#10560=LINE('',#116938,#14676) ;
#10561=LINE('',#116939,#14677) ;
#10562=LINE('',#116943,#14678) ;
#10563=LINE('',#116945,#14679) ;
#10564=LINE('',#116947,#14680) ;
#10565=LINE('',#116948,#14681) ;
#10566=LINE('',#116952,#14682) ;
#10567=LINE('',#116954,#14683) ;
#10568=LINE('',#116956,#14684) ;
#10569=LINE('',#116957,#14685) ;
#10570=LINE('',#116961,#14686) ;
#10571=LINE('',#116963,#14687) ;
#10572=LINE('',#116965,#14688) ;
#10573=LINE('',#116966,#14689) ;
#10574=LINE('',#116969,#14690) ;
#10575=LINE('',#116971,#14691) ;
#10576=LINE('',#116972,#14692) ;
#10577=LINE('',#116976,#14693) ;
#10578=LINE('',#116978,#14694) ;
#10579=LINE('',#116980,#14695) ;
#10580=LINE('',#116981,#14696) ;
#10581=LINE('',#116985,#14697) ;
#10582=LINE('',#116987,#14698) ;
#10583=LINE('',#116989,#14699) ;
#10584=LINE('',#116990,#14700) ;
#10585=LINE('',#116994,#14701) ;
#10586=LINE('',#116996,#14702) ;
#10587=LINE('',#116998,#14703) ;
#10588=LINE('',#116999,#14704) ;
#10589=LINE('',#117003,#14705) ;
#10590=LINE('',#117005,#14706) ;
#10591=LINE('',#117007,#14707) ;
#10592=LINE('',#117008,#14708) ;
#10593=LINE('',#117011,#14709) ;
#10594=LINE('',#117013,#14710) ;
#10595=LINE('',#117014,#14711) ;
#10596=LINE('',#117018,#14712) ;
#10597=LINE('',#117020,#14713) ;
#10598=LINE('',#117022,#14714) ;
#10599=LINE('',#117023,#14715) ;
#10600=LINE('',#117027,#14716) ;
#10601=LINE('',#117029,#14717) ;
#10602=LINE('',#117031,#14718) ;
#10603=LINE('',#117032,#14719) ;
#10604=LINE('',#117036,#14720) ;
#10605=LINE('',#117038,#14721) ;
#10606=LINE('',#117040,#14722) ;
#10607=LINE('',#117041,#14723) ;
#10608=LINE('',#117045,#14724) ;
#10609=LINE('',#117047,#14725) ;
#10610=LINE('',#117049,#14726) ;
#10611=LINE('',#117050,#14727) ;
#10612=LINE('',#117053,#14728) ;
#10613=LINE('',#117055,#14729) ;
#10614=LINE('',#117056,#14730) ;
#10615=LINE('',#117060,#14731) ;
#10616=LINE('',#117062,#14732) ;
#10617=LINE('',#117064,#14733) ;
#10618=LINE('',#117065,#14734) ;
#10619=LINE('',#117069,#14735) ;
#10620=LINE('',#117071,#14736) ;
#10621=LINE('',#117073,#14737) ;
#10622=LINE('',#117074,#14738) ;
#10623=LINE('',#117078,#14739) ;
#10624=LINE('',#117080,#14740) ;
#10625=LINE('',#117082,#14741) ;
#10626=LINE('',#117083,#14742) ;
#10627=LINE('',#117087,#14743) ;
#10628=LINE('',#117089,#14744) ;
#10629=LINE('',#117091,#14745) ;
#10630=LINE('',#117092,#14746) ;
#10631=LINE('',#117095,#14747) ;
#10632=LINE('',#117097,#14748) ;
#10633=LINE('',#117098,#14749) ;
#10634=LINE('',#117102,#14750) ;
#10635=LINE('',#117104,#14751) ;
#10636=LINE('',#117106,#14752) ;
#10637=LINE('',#117107,#14753) ;
#10638=LINE('',#117111,#14754) ;
#10639=LINE('',#117113,#14755) ;
#10640=LINE('',#117115,#14756) ;
#10641=LINE('',#117116,#14757) ;
#10642=LINE('',#117120,#14758) ;
#10643=LINE('',#117122,#14759) ;
#10644=LINE('',#117124,#14760) ;
#10645=LINE('',#117125,#14761) ;
#10646=LINE('',#117129,#14762) ;
#10647=LINE('',#117131,#14763) ;
#10648=LINE('',#117133,#14764) ;
#10649=LINE('',#117134,#14765) ;
#10650=LINE('',#117137,#14766) ;
#10651=LINE('',#117139,#14767) ;
#10652=LINE('',#117140,#14768) ;
#10653=LINE('',#117144,#14769) ;
#10654=LINE('',#117146,#14770) ;
#10655=LINE('',#117148,#14771) ;
#10656=LINE('',#117149,#14772) ;
#10657=LINE('',#117153,#14773) ;
#10658=LINE('',#117155,#14774) ;
#10659=LINE('',#117157,#14775) ;
#10660=LINE('',#117158,#14776) ;
#10661=LINE('',#117162,#14777) ;
#10662=LINE('',#117164,#14778) ;
#10663=LINE('',#117166,#14779) ;
#10664=LINE('',#117167,#14780) ;
#10665=LINE('',#117171,#14781) ;
#10666=LINE('',#117173,#14782) ;
#10667=LINE('',#117175,#14783) ;
#10668=LINE('',#117176,#14784) ;
#10669=LINE('',#117179,#14785) ;
#10670=LINE('',#117181,#14786) ;
#10671=LINE('',#117182,#14787) ;
#10672=LINE('',#117186,#14788) ;
#10673=LINE('',#117188,#14789) ;
#10674=LINE('',#117190,#14790) ;
#10675=LINE('',#117191,#14791) ;
#10676=LINE('',#117195,#14792) ;
#10677=LINE('',#117197,#14793) ;
#10678=LINE('',#117199,#14794) ;
#10679=LINE('',#117200,#14795) ;
#10680=LINE('',#117204,#14796) ;
#10681=LINE('',#117206,#14797) ;
#10682=LINE('',#117208,#14798) ;
#10683=LINE('',#117209,#14799) ;
#10684=LINE('',#117213,#14800) ;
#10685=LINE('',#117217,#14801) ;
#10686=LINE('',#117221,#14802) ;
#10687=LINE('',#117223,#14803) ;
#10688=LINE('',#117224,#14804) ;
#10689=LINE('',#117229,#14805) ;
#10690=LINE('',#117233,#14806) ;
#10691=LINE('',#117235,#14807) ;
#10692=LINE('',#117236,#14808) ;
#10693=LINE('',#117241,#14809) ;
#10694=LINE('',#117244,#14810) ;
#10695=LINE('',#117246,#14811) ;
#10696=LINE('',#117247,#14812) ;
#10697=LINE('',#117250,#14813) ;
#10698=LINE('',#117253,#14814) ;
#10699=LINE('',#117254,#14815) ;
#10700=LINE('',#117257,#14816) ;
#10701=LINE('',#117259,#14817) ;
#10702=LINE('',#117260,#14818) ;
#10703=LINE('',#117265,#14819) ;
#10704=LINE('',#117269,#14820) ;
#10705=LINE('',#117271,#14821) ;
#10706=LINE('',#117272,#14822) ;
#10707=LINE('',#117277,#14823) ;
#10708=LINE('',#117281,#14824) ;
#10709=LINE('',#117283,#14825) ;
#10710=LINE('',#117284,#14826) ;
#10711=LINE('',#117289,#14827) ;
#10712=LINE('',#117293,#14828) ;
#10713=LINE('',#117295,#14829) ;
#10714=LINE('',#117296,#14830) ;
#10715=LINE('',#117301,#14831) ;
#10716=LINE('',#117305,#14832) ;
#10717=LINE('',#117307,#14833) ;
#10718=LINE('',#117308,#14834) ;
#10719=LINE('',#117313,#14835) ;
#10720=LINE('',#117317,#14836) ;
#10721=LINE('',#117319,#14837) ;
#10722=LINE('',#117320,#14838) ;
#10723=LINE('',#117325,#14839) ;
#10724=LINE('',#117331,#14840) ;
#10725=LINE('',#117337,#14841) ;
#10726=LINE('',#117341,#14842) ;
#10727=LINE('',#117343,#14843) ;
#10728=LINE('',#117344,#14844) ;
#10729=LINE('',#117349,#14845) ;
#10730=LINE('',#117353,#14846) ;
#10731=LINE('',#117355,#14847) ;
#10732=LINE('',#117356,#14848) ;
#10733=LINE('',#117361,#14849) ;
#10734=LINE('',#117364,#14850) ;
#10735=LINE('',#117365,#14851) ;
#10736=LINE('',#117371,#14852) ;
#10737=LINE('',#117375,#14853) ;
#10738=LINE('',#117377,#14854) ;
#10739=LINE('',#117379,#14855) ;
#10740=LINE('',#117383,#14856) ;
#10741=LINE('',#117385,#14857) ;
#10742=LINE('',#117387,#14858) ;
#10743=LINE('',#117391,#14859) ;
#10744=LINE('',#117395,#14860) ;
#10745=LINE('',#117397,#14861) ;
#10746=LINE('',#117398,#14862) ;
#10747=LINE('',#117400,#14863) ;
#10748=LINE('',#117401,#14864) ;
#10749=LINE('',#117405,#14865) ;
#10750=LINE('',#117409,#14866) ;
#10751=LINE('',#117413,#14867) ;
#10752=LINE('',#117415,#14868) ;
#10753=LINE('',#117416,#14869) ;
#10754=LINE('',#117421,#14870) ;
#10755=LINE('',#117425,#14871) ;
#10756=LINE('',#117427,#14872) ;
#10757=LINE('',#117428,#14873) ;
#10758=LINE('',#117433,#14874) ;
#10759=LINE('',#117436,#14875) ;
#10760=LINE('',#117438,#14876) ;
#10761=LINE('',#117439,#14877) ;
#10762=LINE('',#117442,#14878) ;
#10763=LINE('',#117445,#14879) ;
#10764=LINE('',#117446,#14880) ;
#10765=LINE('',#117449,#14881) ;
#10766=LINE('',#117451,#14882) ;
#10767=LINE('',#117452,#14883) ;
#10768=LINE('',#117457,#14884) ;
#10769=LINE('',#117461,#14885) ;
#10770=LINE('',#117463,#14886) ;
#10771=LINE('',#117464,#14887) ;
#10772=LINE('',#117469,#14888) ;
#10773=LINE('',#117473,#14889) ;
#10774=LINE('',#117475,#14890) ;
#10775=LINE('',#117476,#14891) ;
#10776=LINE('',#117481,#14892) ;
#10777=LINE('',#117485,#14893) ;
#10778=LINE('',#117487,#14894) ;
#10779=LINE('',#117488,#14895) ;
#10780=LINE('',#117493,#14896) ;
#10781=LINE('',#117497,#14897) ;
#10782=LINE('',#117499,#14898) ;
#10783=LINE('',#117500,#14899) ;
#10784=LINE('',#117505,#14900) ;
#10785=LINE('',#117509,#14901) ;
#10786=LINE('',#117511,#14902) ;
#10787=LINE('',#117512,#14903) ;
#10788=LINE('',#117517,#14904) ;
#10789=LINE('',#117523,#14905) ;
#10790=LINE('',#117529,#14906) ;
#10791=LINE('',#117533,#14907) ;
#10792=LINE('',#117535,#14908) ;
#10793=LINE('',#117536,#14909) ;
#10794=LINE('',#117541,#14910) ;
#10795=LINE('',#117545,#14911) ;
#10796=LINE('',#117547,#14912) ;
#10797=LINE('',#117548,#14913) ;
#10798=LINE('',#117553,#14914) ;
#10799=LINE('',#117556,#14915) ;
#10800=LINE('',#117557,#14916) ;
#10801=LINE('',#117563,#14917) ;
#10802=LINE('',#117567,#14918) ;
#10803=LINE('',#117569,#14919) ;
#10804=LINE('',#117571,#14920) ;
#10805=LINE('',#117575,#14921) ;
#10806=LINE('',#117577,#14922) ;
#10807=LINE('',#117579,#14923) ;
#10808=LINE('',#117583,#14924) ;
#10809=LINE('',#117587,#14925) ;
#10810=LINE('',#117589,#14926) ;
#10811=LINE('',#117590,#14927) ;
#10812=LINE('',#117592,#14928) ;
#10813=LINE('',#117593,#14929) ;
#10814=LINE('',#117597,#14930) ;
#10815=LINE('',#117601,#14931) ;
#10816=LINE('',#117605,#14932) ;
#10817=LINE('',#117607,#14933) ;
#10818=LINE('',#117608,#14934) ;
#10819=LINE('',#117613,#14935) ;
#10820=LINE('',#117617,#14936) ;
#10821=LINE('',#117619,#14937) ;
#10822=LINE('',#117620,#14938) ;
#10823=LINE('',#117625,#14939) ;
#10824=LINE('',#117628,#14940) ;
#10825=LINE('',#117630,#14941) ;
#10826=LINE('',#117631,#14942) ;
#10827=LINE('',#117634,#14943) ;
#10828=LINE('',#117637,#14944) ;
#10829=LINE('',#117638,#14945) ;
#10830=LINE('',#117641,#14946) ;
#10831=LINE('',#117643,#14947) ;
#10832=LINE('',#117644,#14948) ;
#10833=LINE('',#117649,#14949) ;
#10834=LINE('',#117653,#14950) ;
#10835=LINE('',#117655,#14951) ;
#10836=LINE('',#117656,#14952) ;
#10837=LINE('',#117661,#14953) ;
#10838=LINE('',#117665,#14954) ;
#10839=LINE('',#117667,#14955) ;
#10840=LINE('',#117668,#14956) ;
#10841=LINE('',#117673,#14957) ;
#10842=LINE('',#117677,#14958) ;
#10843=LINE('',#117679,#14959) ;
#10844=LINE('',#117680,#14960) ;
#10845=LINE('',#117685,#14961) ;
#10846=LINE('',#117689,#14962) ;
#10847=LINE('',#117691,#14963) ;
#10848=LINE('',#117692,#14964) ;
#10849=LINE('',#117697,#14965) ;
#10850=LINE('',#117701,#14966) ;
#10851=LINE('',#117703,#14967) ;
#10852=LINE('',#117704,#14968) ;
#10853=LINE('',#117709,#14969) ;
#10854=LINE('',#117715,#14970) ;
#10855=LINE('',#117721,#14971) ;
#10856=LINE('',#117725,#14972) ;
#10857=LINE('',#117727,#14973) ;
#10858=LINE('',#117728,#14974) ;
#10859=LINE('',#117733,#14975) ;
#10860=LINE('',#117737,#14976) ;
#10861=LINE('',#117739,#14977) ;
#10862=LINE('',#117740,#14978) ;
#10863=LINE('',#117745,#14979) ;
#10864=LINE('',#117748,#14980) ;
#10865=LINE('',#117749,#14981) ;
#10866=LINE('',#117755,#14982) ;
#10867=LINE('',#117759,#14983) ;
#10868=LINE('',#117761,#14984) ;
#10869=LINE('',#117763,#14985) ;
#10870=LINE('',#117767,#14986) ;
#10871=LINE('',#117769,#14987) ;
#10872=LINE('',#117771,#14988) ;
#10873=LINE('',#117775,#14989) ;
#10874=LINE('',#117779,#14990) ;
#10875=LINE('',#117781,#14991) ;
#10876=LINE('',#117782,#14992) ;
#10877=LINE('',#117784,#14993) ;
#10878=LINE('',#117785,#14994) ;
#10879=LINE('',#117789,#14995) ;
#10880=LINE('',#117793,#14996) ;
#10881=LINE('',#117797,#14997) ;
#10882=LINE('',#117799,#14998) ;
#10883=LINE('',#117800,#14999) ;
#10884=LINE('',#117805,#15000) ;
#10885=LINE('',#117809,#15001) ;
#10886=LINE('',#117811,#15002) ;
#10887=LINE('',#117812,#15003) ;
#10888=LINE('',#117817,#15004) ;
#10889=LINE('',#117820,#15005) ;
#10890=LINE('',#117822,#15006) ;
#10891=LINE('',#117823,#15007) ;
#10892=LINE('',#117826,#15008) ;
#10893=LINE('',#117829,#15009) ;
#10894=LINE('',#117830,#15010) ;
#10895=LINE('',#117833,#15011) ;
#10896=LINE('',#117835,#15012) ;
#10897=LINE('',#117836,#15013) ;
#10898=LINE('',#117841,#15014) ;
#10899=LINE('',#117845,#15015) ;
#10900=LINE('',#117847,#15016) ;
#10901=LINE('',#117848,#15017) ;
#10902=LINE('',#117853,#15018) ;
#10903=LINE('',#117857,#15019) ;
#10904=LINE('',#117859,#15020) ;
#10905=LINE('',#117860,#15021) ;
#10906=LINE('',#117865,#15022) ;
#10907=LINE('',#117869,#15023) ;
#10908=LINE('',#117871,#15024) ;
#10909=LINE('',#117872,#15025) ;
#10910=LINE('',#117877,#15026) ;
#10911=LINE('',#117881,#15027) ;
#10912=LINE('',#117883,#15028) ;
#10913=LINE('',#117884,#15029) ;
#10914=LINE('',#117889,#15030) ;
#10915=LINE('',#117893,#15031) ;
#10916=LINE('',#117895,#15032) ;
#10917=LINE('',#117896,#15033) ;
#10918=LINE('',#117901,#15034) ;
#10919=LINE('',#117907,#15035) ;
#10920=LINE('',#117913,#15036) ;
#10921=LINE('',#117917,#15037) ;
#10922=LINE('',#117919,#15038) ;
#10923=LINE('',#117920,#15039) ;
#10924=LINE('',#117925,#15040) ;
#10925=LINE('',#117929,#15041) ;
#10926=LINE('',#117931,#15042) ;
#10927=LINE('',#117932,#15043) ;
#10928=LINE('',#117937,#15044) ;
#10929=LINE('',#117940,#15045) ;
#10930=LINE('',#117941,#15046) ;
#10931=LINE('',#117947,#15047) ;
#10932=LINE('',#117951,#15048) ;
#10933=LINE('',#117953,#15049) ;
#10934=LINE('',#117955,#15050) ;
#10935=LINE('',#117959,#15051) ;
#10936=LINE('',#117961,#15052) ;
#10937=LINE('',#117963,#15053) ;
#10938=LINE('',#117967,#15054) ;
#10939=LINE('',#117971,#15055) ;
#10940=LINE('',#117973,#15056) ;
#10941=LINE('',#117974,#15057) ;
#10942=LINE('',#117976,#15058) ;
#10943=LINE('',#117977,#15059) ;
#10944=LINE('',#117981,#15060) ;
#10945=LINE('',#117985,#15061) ;
#10946=LINE('',#117989,#15062) ;
#10947=LINE('',#117991,#15063) ;
#10948=LINE('',#117992,#15064) ;
#10949=LINE('',#117997,#15065) ;
#10950=LINE('',#118001,#15066) ;
#10951=LINE('',#118003,#15067) ;
#10952=LINE('',#118004,#15068) ;
#10953=LINE('',#118009,#15069) ;
#10954=LINE('',#118012,#15070) ;
#10955=LINE('',#118014,#15071) ;
#10956=LINE('',#118015,#15072) ;
#10957=LINE('',#118018,#15073) ;
#10958=LINE('',#118021,#15074) ;
#10959=LINE('',#118022,#15075) ;
#10960=LINE('',#118025,#15076) ;
#10961=LINE('',#118027,#15077) ;
#10962=LINE('',#118028,#15078) ;
#10963=LINE('',#118033,#15079) ;
#10964=LINE('',#118037,#15080) ;
#10965=LINE('',#118039,#15081) ;
#10966=LINE('',#118040,#15082) ;
#10967=LINE('',#118045,#15083) ;
#10968=LINE('',#118049,#15084) ;
#10969=LINE('',#118051,#15085) ;
#10970=LINE('',#118052,#15086) ;
#10971=LINE('',#118057,#15087) ;
#10972=LINE('',#118061,#15088) ;
#10973=LINE('',#118063,#15089) ;
#10974=LINE('',#118064,#15090) ;
#10975=LINE('',#118069,#15091) ;
#10976=LINE('',#118073,#15092) ;
#10977=LINE('',#118075,#15093) ;
#10978=LINE('',#118076,#15094) ;
#10979=LINE('',#118081,#15095) ;
#10980=LINE('',#118085,#15096) ;
#10981=LINE('',#118087,#15097) ;
#10982=LINE('',#118088,#15098) ;
#10983=LINE('',#118093,#15099) ;
#10984=LINE('',#118099,#15100) ;
#10985=LINE('',#118105,#15101) ;
#10986=LINE('',#118109,#15102) ;
#10987=LINE('',#118111,#15103) ;
#10988=LINE('',#118112,#15104) ;
#10989=LINE('',#118117,#15105) ;
#10990=LINE('',#118121,#15106) ;
#10991=LINE('',#118123,#15107) ;
#10992=LINE('',#118124,#15108) ;
#10993=LINE('',#118129,#15109) ;
#10994=LINE('',#118132,#15110) ;
#10995=LINE('',#118133,#15111) ;
#10996=LINE('',#118139,#15112) ;
#10997=LINE('',#118143,#15113) ;
#10998=LINE('',#118145,#15114) ;
#10999=LINE('',#118147,#15115) ;
#11000=LINE('',#118151,#15116) ;
#11001=LINE('',#118153,#15117) ;
#11002=LINE('',#118155,#15118) ;
#11003=LINE('',#118159,#15119) ;
#11004=LINE('',#118163,#15120) ;
#11005=LINE('',#118165,#15121) ;
#11006=LINE('',#118166,#15122) ;
#11007=LINE('',#118168,#15123) ;
#11008=LINE('',#118169,#15124) ;
#11009=LINE('',#118173,#15125) ;
#11010=LINE('',#118177,#15126) ;
#11011=LINE('',#118181,#15127) ;
#11012=LINE('',#118183,#15128) ;
#11013=LINE('',#118184,#15129) ;
#11014=LINE('',#118189,#15130) ;
#11015=LINE('',#118193,#15131) ;
#11016=LINE('',#118195,#15132) ;
#11017=LINE('',#118196,#15133) ;
#11018=LINE('',#118201,#15134) ;
#11019=LINE('',#118204,#15135) ;
#11020=LINE('',#118206,#15136) ;
#11021=LINE('',#118207,#15137) ;
#11022=LINE('',#118210,#15138) ;
#11023=LINE('',#118213,#15139) ;
#11024=LINE('',#118214,#15140) ;
#11025=LINE('',#118217,#15141) ;
#11026=LINE('',#118219,#15142) ;
#11027=LINE('',#118220,#15143) ;
#11028=LINE('',#118225,#15144) ;
#11029=LINE('',#118229,#15145) ;
#11030=LINE('',#118231,#15146) ;
#11031=LINE('',#118232,#15147) ;
#11032=LINE('',#118237,#15148) ;
#11033=LINE('',#118241,#15149) ;
#11034=LINE('',#118243,#15150) ;
#11035=LINE('',#118244,#15151) ;
#11036=LINE('',#118249,#15152) ;
#11037=LINE('',#118253,#15153) ;
#11038=LINE('',#118255,#15154) ;
#11039=LINE('',#118256,#15155) ;
#11040=LINE('',#118261,#15156) ;
#11041=LINE('',#118265,#15157) ;
#11042=LINE('',#118267,#15158) ;
#11043=LINE('',#118268,#15159) ;
#11044=LINE('',#118273,#15160) ;
#11045=LINE('',#118277,#15161) ;
#11046=LINE('',#118279,#15162) ;
#11047=LINE('',#118280,#15163) ;
#11048=LINE('',#118285,#15164) ;
#11049=LINE('',#118291,#15165) ;
#11050=LINE('',#118297,#15166) ;
#11051=LINE('',#118301,#15167) ;
#11052=LINE('',#118303,#15168) ;
#11053=LINE('',#118304,#15169) ;
#11054=LINE('',#118309,#15170) ;
#11055=LINE('',#118313,#15171) ;
#11056=LINE('',#118315,#15172) ;
#11057=LINE('',#118316,#15173) ;
#11058=LINE('',#118321,#15174) ;
#11059=LINE('',#118324,#15175) ;
#11060=LINE('',#118325,#15176) ;
#11061=LINE('',#118331,#15177) ;
#11062=LINE('',#118335,#15178) ;
#11063=LINE('',#118337,#15179) ;
#11064=LINE('',#118339,#15180) ;
#11065=LINE('',#118343,#15181) ;
#11066=LINE('',#118345,#15182) ;
#11067=LINE('',#118347,#15183) ;
#11068=LINE('',#118351,#15184) ;
#11069=LINE('',#118355,#15185) ;
#11070=LINE('',#118357,#15186) ;
#11071=LINE('',#118358,#15187) ;
#11072=LINE('',#118360,#15188) ;
#11073=LINE('',#118361,#15189) ;
#11074=LINE('',#118365,#15190) ;
#11075=LINE('',#118369,#15191) ;
#11076=LINE('',#118373,#15192) ;
#11077=LINE('',#118375,#15193) ;
#11078=LINE('',#118376,#15194) ;
#11079=LINE('',#118381,#15195) ;
#11080=LINE('',#118385,#15196) ;
#11081=LINE('',#118387,#15197) ;
#11082=LINE('',#118388,#15198) ;
#11083=LINE('',#118393,#15199) ;
#11084=LINE('',#118396,#15200) ;
#11085=LINE('',#118398,#15201) ;
#11086=LINE('',#118399,#15202) ;
#11087=LINE('',#118402,#15203) ;
#11088=LINE('',#118405,#15204) ;
#11089=LINE('',#118406,#15205) ;
#11090=LINE('',#118409,#15206) ;
#11091=LINE('',#118411,#15207) ;
#11092=LINE('',#118412,#15208) ;
#11093=LINE('',#118417,#15209) ;
#11094=LINE('',#118421,#15210) ;
#11095=LINE('',#118423,#15211) ;
#11096=LINE('',#118424,#15212) ;
#11097=LINE('',#118429,#15213) ;
#11098=LINE('',#118433,#15214) ;
#11099=LINE('',#118435,#15215) ;
#11100=LINE('',#118436,#15216) ;
#11101=LINE('',#118441,#15217) ;
#11102=LINE('',#118445,#15218) ;
#11103=LINE('',#118447,#15219) ;
#11104=LINE('',#118448,#15220) ;
#11105=LINE('',#118453,#15221) ;
#11106=LINE('',#118457,#15222) ;
#11107=LINE('',#118459,#15223) ;
#11108=LINE('',#118460,#15224) ;
#11109=LINE('',#118465,#15225) ;
#11110=LINE('',#118469,#15226) ;
#11111=LINE('',#118471,#15227) ;
#11112=LINE('',#118472,#15228) ;
#11113=LINE('',#118477,#15229) ;
#11114=LINE('',#118483,#15230) ;
#11115=LINE('',#118489,#15231) ;
#11116=LINE('',#118493,#15232) ;
#11117=LINE('',#118495,#15233) ;
#11118=LINE('',#118496,#15234) ;
#11119=LINE('',#118501,#15235) ;
#11120=LINE('',#118505,#15236) ;
#11121=LINE('',#118507,#15237) ;
#11122=LINE('',#118508,#15238) ;
#11123=LINE('',#118513,#15239) ;
#11124=LINE('',#118516,#15240) ;
#11125=LINE('',#118517,#15241) ;
#11126=LINE('',#118523,#15242) ;
#11127=LINE('',#118527,#15243) ;
#11128=LINE('',#118529,#15244) ;
#11129=LINE('',#118531,#15245) ;
#11130=LINE('',#118535,#15246) ;
#11131=LINE('',#118537,#15247) ;
#11132=LINE('',#118539,#15248) ;
#11133=LINE('',#118543,#15249) ;
#11134=LINE('',#118547,#15250) ;
#11135=LINE('',#118549,#15251) ;
#11136=LINE('',#118550,#15252) ;
#11137=LINE('',#118552,#15253) ;
#11138=LINE('',#118553,#15254) ;
#11139=LINE('',#118557,#15255) ;
#11140=LINE('',#118561,#15256) ;
#11141=LINE('',#118565,#15257) ;
#11142=LINE('',#118567,#15258) ;
#11143=LINE('',#118568,#15259) ;
#11144=LINE('',#118573,#15260) ;
#11145=LINE('',#118577,#15261) ;
#11146=LINE('',#118579,#15262) ;
#11147=LINE('',#118580,#15263) ;
#11148=LINE('',#118585,#15264) ;
#11149=LINE('',#118588,#15265) ;
#11150=LINE('',#118590,#15266) ;
#11151=LINE('',#118591,#15267) ;
#11152=LINE('',#118594,#15268) ;
#11153=LINE('',#118597,#15269) ;
#11154=LINE('',#118598,#15270) ;
#11155=LINE('',#118601,#15271) ;
#11156=LINE('',#118603,#15272) ;
#11157=LINE('',#118604,#15273) ;
#11158=LINE('',#118609,#15274) ;
#11159=LINE('',#118613,#15275) ;
#11160=LINE('',#118615,#15276) ;
#11161=LINE('',#118616,#15277) ;
#11162=LINE('',#118621,#15278) ;
#11163=LINE('',#118625,#15279) ;
#11164=LINE('',#118627,#15280) ;
#11165=LINE('',#118628,#15281) ;
#11166=LINE('',#118633,#15282) ;
#11167=LINE('',#118637,#15283) ;
#11168=LINE('',#118639,#15284) ;
#11169=LINE('',#118640,#15285) ;
#11170=LINE('',#118645,#15286) ;
#11171=LINE('',#118649,#15287) ;
#11172=LINE('',#118651,#15288) ;
#11173=LINE('',#118652,#15289) ;
#11174=LINE('',#118657,#15290) ;
#11175=LINE('',#118661,#15291) ;
#11176=LINE('',#118663,#15292) ;
#11177=LINE('',#118664,#15293) ;
#11178=LINE('',#118669,#15294) ;
#11179=LINE('',#118675,#15295) ;
#11180=LINE('',#118681,#15296) ;
#11181=LINE('',#118685,#15297) ;
#11182=LINE('',#118687,#15298) ;
#11183=LINE('',#118688,#15299) ;
#11184=LINE('',#118693,#15300) ;
#11185=LINE('',#118697,#15301) ;
#11186=LINE('',#118699,#15302) ;
#11187=LINE('',#118700,#15303) ;
#11188=LINE('',#118705,#15304) ;
#11189=LINE('',#118708,#15305) ;
#11190=LINE('',#118709,#15306) ;
#11191=LINE('',#118715,#15307) ;
#11192=LINE('',#118719,#15308) ;
#11193=LINE('',#118721,#15309) ;
#11194=LINE('',#118723,#15310) ;
#11195=LINE('',#118727,#15311) ;
#11196=LINE('',#118729,#15312) ;
#11197=LINE('',#118731,#15313) ;
#11198=LINE('',#118735,#15314) ;
#11199=LINE('',#118739,#15315) ;
#11200=LINE('',#118741,#15316) ;
#11201=LINE('',#118742,#15317) ;
#11202=LINE('',#118744,#15318) ;
#11203=LINE('',#118745,#15319) ;
#11204=LINE('',#118749,#15320) ;
#11205=LINE('',#118753,#15321) ;
#11206=LINE('',#118757,#15322) ;
#11207=LINE('',#118759,#15323) ;
#11208=LINE('',#118760,#15324) ;
#11209=LINE('',#118765,#15325) ;
#11210=LINE('',#118769,#15326) ;
#11211=LINE('',#118771,#15327) ;
#11212=LINE('',#118772,#15328) ;
#11213=LINE('',#118777,#15329) ;
#11214=LINE('',#118780,#15330) ;
#11215=LINE('',#118782,#15331) ;
#11216=LINE('',#118783,#15332) ;
#11217=LINE('',#118786,#15333) ;
#11218=LINE('',#118789,#15334) ;
#11219=LINE('',#118790,#15335) ;
#11220=LINE('',#118793,#15336) ;
#11221=LINE('',#118795,#15337) ;
#11222=LINE('',#118796,#15338) ;
#11223=LINE('',#118801,#15339) ;
#11224=LINE('',#118805,#15340) ;
#11225=LINE('',#118807,#15341) ;
#11226=LINE('',#118808,#15342) ;
#11227=LINE('',#118813,#15343) ;
#11228=LINE('',#118817,#15344) ;
#11229=LINE('',#118819,#15345) ;
#11230=LINE('',#118820,#15346) ;
#11231=LINE('',#118825,#15347) ;
#11232=LINE('',#118829,#15348) ;
#11233=LINE('',#118831,#15349) ;
#11234=LINE('',#118832,#15350) ;
#11235=LINE('',#118837,#15351) ;
#11236=LINE('',#118841,#15352) ;
#11237=LINE('',#118843,#15353) ;
#11238=LINE('',#118844,#15354) ;
#11239=LINE('',#118849,#15355) ;
#11240=LINE('',#118853,#15356) ;
#11241=LINE('',#118855,#15357) ;
#11242=LINE('',#118856,#15358) ;
#11243=LINE('',#118861,#15359) ;
#11244=LINE('',#118867,#15360) ;
#11245=LINE('',#118873,#15361) ;
#11246=LINE('',#118877,#15362) ;
#11247=LINE('',#118879,#15363) ;
#11248=LINE('',#118880,#15364) ;
#11249=LINE('',#118885,#15365) ;
#11250=LINE('',#118889,#15366) ;
#11251=LINE('',#118891,#15367) ;
#11252=LINE('',#118892,#15368) ;
#11253=LINE('',#118897,#15369) ;
#11254=LINE('',#118900,#15370) ;
#11255=LINE('',#118901,#15371) ;
#11256=LINE('',#118907,#15372) ;
#11257=LINE('',#118911,#15373) ;
#11258=LINE('',#118913,#15374) ;
#11259=LINE('',#118915,#15375) ;
#11260=LINE('',#118919,#15376) ;
#11261=LINE('',#118921,#15377) ;
#11262=LINE('',#118923,#15378) ;
#11263=LINE('',#118927,#15379) ;
#11264=LINE('',#118931,#15380) ;
#11265=LINE('',#118933,#15381) ;
#11266=LINE('',#118934,#15382) ;
#11267=LINE('',#118936,#15383) ;
#11268=LINE('',#118937,#15384) ;
#11269=LINE('',#118941,#15385) ;
#11270=LINE('',#118945,#15386) ;
#11271=LINE('',#118949,#15387) ;
#11272=LINE('',#118953,#15388) ;
#11273=LINE('',#118958,#15389) ;
#11274=LINE('',#118962,#15390) ;
#11275=LINE('',#118966,#15391) ;
#11276=LINE('',#118970,#15392) ;
#11277=LINE('',#118975,#15393) ;
#11278=LINE('',#118979,#15394) ;
#11279=LINE('',#118983,#15395) ;
#11280=LINE('',#118987,#15396) ;
#11281=LINE('',#118992,#15397) ;
#11282=LINE('',#118996,#15398) ;
#11283=LINE('',#119000,#15399) ;
#11284=LINE('',#119004,#15400) ;
#11285=LINE('',#119009,#15401) ;
#11286=LINE('',#119013,#15402) ;
#11287=LINE('',#119017,#15403) ;
#11288=LINE('',#119021,#15404) ;
#11289=LINE('',#119026,#15405) ;
#11290=LINE('',#119030,#15406) ;
#11291=LINE('',#119034,#15407) ;
#11292=LINE('',#119038,#15408) ;
#11293=LINE('',#119043,#15409) ;
#11294=LINE('',#119047,#15410) ;
#11295=LINE('',#119051,#15411) ;
#11296=LINE('',#119055,#15412) ;
#11297=LINE('',#119060,#15413) ;
#11298=LINE('',#119064,#15414) ;
#11299=LINE('',#119068,#15415) ;
#11300=LINE('',#119072,#15416) ;
#11301=LINE('',#119077,#15417) ;
#11302=LINE('',#119081,#15418) ;
#11303=LINE('',#119085,#15419) ;
#11304=LINE('',#119089,#15420) ;
#11305=LINE('',#119117,#15421) ;
#11306=LINE('',#119174,#15422) ;
#11307=LINE('',#119199,#15423) ;
#11308=LINE('',#119231,#15424) ;
#11309=LINE('',#119257,#15425) ;
#11310=LINE('',#119821,#15426) ;
#11311=LINE('',#119878,#15427) ;
#11312=LINE('',#119903,#15428) ;
#11313=LINE('',#119935,#15429) ;
#11314=LINE('',#119961,#15430) ;
#11315=LINE('',#120048,#15431) ;
#11316=LINE('',#120105,#15432) ;
#11317=LINE('',#120130,#15433) ;
#11318=LINE('',#120162,#15434) ;
#11319=LINE('',#120188,#15435) ;
#11320=LINE('',#120275,#15436) ;
#11321=LINE('',#120332,#15437) ;
#11322=LINE('',#120357,#15438) ;
#11323=LINE('',#120389,#15439) ;
#11324=LINE('',#120415,#15440) ;
#11325=LINE('',#120502,#15441) ;
#11326=LINE('',#120559,#15442) ;
#11327=LINE('',#120584,#15443) ;
#11328=LINE('',#120616,#15444) ;
#11329=LINE('',#120642,#15445) ;
#11330=LINE('',#120729,#15446) ;
#11331=LINE('',#120786,#15447) ;
#11332=LINE('',#120811,#15448) ;
#11333=LINE('',#120843,#15449) ;
#11334=LINE('',#120869,#15450) ;
#11335=LINE('',#120956,#15451) ;
#11336=LINE('',#121013,#15452) ;
#11337=LINE('',#121038,#15453) ;
#11338=LINE('',#121070,#15454) ;
#11339=LINE('',#121096,#15455) ;
#11340=LINE('',#121183,#15456) ;
#11341=LINE('',#121240,#15457) ;
#11342=LINE('',#121265,#15458) ;
#11343=LINE('',#121297,#15459) ;
#11344=LINE('',#121323,#15460) ;
#11345=LINE('',#121410,#15461) ;
#11346=LINE('',#121467,#15462) ;
#11347=LINE('',#121492,#15463) ;
#11348=LINE('',#121524,#15464) ;
#11349=LINE('',#121550,#15465) ;
#11350=LINE('',#121614,#15466) ;
#11351=LINE('',#121616,#15467) ;
#11352=LINE('',#121618,#15468) ;
#11353=LINE('',#121619,#15469) ;
#11354=LINE('',#121623,#15470) ;
#11355=LINE('',#121625,#15471) ;
#11356=LINE('',#121627,#15472) ;
#11357=LINE('',#121628,#15473) ;
#11358=LINE('',#121632,#15474) ;
#11359=LINE('',#121634,#15475) ;
#11360=LINE('',#121636,#15476) ;
#11361=LINE('',#121637,#15477) ;
#11362=LINE('',#121641,#15478) ;
#11363=LINE('',#121643,#15479) ;
#11364=LINE('',#121645,#15480) ;
#11365=LINE('',#121646,#15481) ;
#11366=LINE('',#121650,#15482) ;
#11367=LINE('',#121652,#15483) ;
#11368=LINE('',#121654,#15484) ;
#11369=LINE('',#121655,#15485) ;
#11370=LINE('',#121659,#15486) ;
#11371=LINE('',#121664,#15487) ;
#11372=LINE('',#121665,#15488) ;
#11373=LINE('',#121669,#15489) ;
#11374=LINE('',#121674,#15490) ;
#11375=LINE('',#121675,#15491) ;
#11376=LINE('',#121685,#15492) ;
#11377=LINE('',#121687,#15493) ;
#11378=LINE('',#121689,#15494) ;
#11379=LINE('',#121690,#15495) ;
#11380=LINE('',#121694,#15496) ;
#11381=LINE('',#121695,#15497) ;
#11382=LINE('',#121696,#15498) ;
#11383=LINE('',#121699,#15499) ;
#11384=LINE('',#121701,#15500) ;
#11385=LINE('',#121702,#15501) ;
#11386=LINE('',#121706,#15502) ;
#11387=LINE('',#121708,#15503) ;
#11388=LINE('',#121710,#15504) ;
#11389=LINE('',#121711,#15505) ;
#11390=LINE('',#121715,#15506) ;
#11391=LINE('',#121717,#15507) ;
#11392=LINE('',#121719,#15508) ;
#11393=LINE('',#121720,#15509) ;
#11394=LINE('',#121724,#15510) ;
#11395=LINE('',#121725,#15511) ;
#11396=LINE('',#121726,#15512) ;
#11397=LINE('',#121729,#15513) ;
#11398=LINE('',#121731,#15514) ;
#11399=LINE('',#121732,#15515) ;
#11400=LINE('',#121736,#15516) ;
#11401=LINE('',#121738,#15517) ;
#11402=LINE('',#121740,#15518) ;
#11403=LINE('',#121741,#15519) ;
#11404=LINE('',#121745,#15520) ;
#11405=LINE('',#121747,#15521) ;
#11406=LINE('',#121749,#15522) ;
#11407=LINE('',#121750,#15523) ;
#11408=LINE('',#121754,#15524) ;
#11409=LINE('',#121756,#15525) ;
#11410=LINE('',#121758,#15526) ;
#11411=LINE('',#121759,#15527) ;
#11412=LINE('',#121763,#15528) ;
#11413=LINE('',#121765,#15529) ;
#11414=LINE('',#121767,#15530) ;
#11415=LINE('',#121768,#15531) ;
#11416=LINE('',#121772,#15532) ;
#11417=LINE('',#121774,#15533) ;
#11418=LINE('',#121776,#15534) ;
#11419=LINE('',#121777,#15535) ;
#11420=LINE('',#121781,#15536) ;
#11421=LINE('',#121786,#15537) ;
#11422=LINE('',#121787,#15538) ;
#11423=LINE('',#121791,#15539) ;
#11424=LINE('',#121796,#15540) ;
#11425=LINE('',#121797,#15541) ;
#11426=LINE('',#121807,#15542) ;
#11427=LINE('',#121809,#15543) ;
#11428=LINE('',#121811,#15544) ;
#11429=LINE('',#121812,#15545) ;
#11430=LINE('',#121816,#15546) ;
#11431=LINE('',#121817,#15547) ;
#11432=LINE('',#121818,#15548) ;
#11433=LINE('',#121821,#15549) ;
#11434=LINE('',#121823,#15550) ;
#11435=LINE('',#121824,#15551) ;
#11436=LINE('',#121828,#15552) ;
#11437=LINE('',#121830,#15553) ;
#11438=LINE('',#121832,#15554) ;
#11439=LINE('',#121833,#15555) ;
#11440=LINE('',#121837,#15556) ;
#11441=LINE('',#121839,#15557) ;
#11442=LINE('',#121841,#15558) ;
#11443=LINE('',#121842,#15559) ;
#11444=LINE('',#121846,#15560) ;
#11445=LINE('',#121847,#15561) ;
#11446=LINE('',#121848,#15562) ;
#11447=LINE('',#121851,#15563) ;
#11448=LINE('',#121853,#15564) ;
#11449=LINE('',#121854,#15565) ;
#11450=LINE('',#121858,#15566) ;
#11451=LINE('',#121860,#15567) ;
#11452=LINE('',#121862,#15568) ;
#11453=LINE('',#121863,#15569) ;
#11454=LINE('',#121867,#15570) ;
#11455=LINE('',#121869,#15571) ;
#11456=LINE('',#121871,#15572) ;
#11457=LINE('',#121872,#15573) ;
#11458=LINE('',#121876,#15574) ;
#11459=LINE('',#121878,#15575) ;
#11460=LINE('',#121880,#15576) ;
#11461=LINE('',#121881,#15577) ;
#11462=LINE('',#121885,#15578) ;
#11463=LINE('',#121887,#15579) ;
#11464=LINE('',#121889,#15580) ;
#11465=LINE('',#121890,#15581) ;
#11466=LINE('',#121894,#15582) ;
#11467=LINE('',#121896,#15583) ;
#11468=LINE('',#121898,#15584) ;
#11469=LINE('',#121899,#15585) ;
#11470=LINE('',#121903,#15586) ;
#11471=LINE('',#121908,#15587) ;
#11472=LINE('',#121909,#15588) ;
#11473=LINE('',#121913,#15589) ;
#11474=LINE('',#121918,#15590) ;
#11475=LINE('',#121919,#15591) ;
#11476=LINE('',#121929,#15592) ;
#11477=LINE('',#121931,#15593) ;
#11478=LINE('',#121933,#15594) ;
#11479=LINE('',#121934,#15595) ;
#11480=LINE('',#121938,#15596) ;
#11481=LINE('',#121939,#15597) ;
#11482=LINE('',#121940,#15598) ;
#11483=LINE('',#121943,#15599) ;
#11484=LINE('',#121945,#15600) ;
#11485=LINE('',#121946,#15601) ;
#11486=LINE('',#121950,#15602) ;
#11487=LINE('',#121952,#15603) ;
#11488=LINE('',#121954,#15604) ;
#11489=LINE('',#121955,#15605) ;
#11490=LINE('',#121959,#15606) ;
#11491=LINE('',#121961,#15607) ;
#11492=LINE('',#121963,#15608) ;
#11493=LINE('',#121964,#15609) ;
#11494=LINE('',#121968,#15610) ;
#11495=LINE('',#121969,#15611) ;
#11496=LINE('',#121970,#15612) ;
#11497=LINE('',#121973,#15613) ;
#11498=LINE('',#121975,#15614) ;
#11499=LINE('',#121976,#15615) ;
#11500=LINE('',#121980,#15616) ;
#11501=LINE('',#121982,#15617) ;
#11502=LINE('',#121984,#15618) ;
#11503=LINE('',#121985,#15619) ;
#11504=LINE('',#121989,#15620) ;
#11505=LINE('',#121991,#15621) ;
#11506=LINE('',#121993,#15622) ;
#11507=LINE('',#121994,#15623) ;
#11508=LINE('',#121998,#15624) ;
#11509=LINE('',#122000,#15625) ;
#11510=LINE('',#122002,#15626) ;
#11511=LINE('',#122003,#15627) ;
#11512=LINE('',#122007,#15628) ;
#11513=LINE('',#122009,#15629) ;
#11514=LINE('',#122011,#15630) ;
#11515=LINE('',#122012,#15631) ;
#11516=LINE('',#122016,#15632) ;
#11517=LINE('',#122018,#15633) ;
#11518=LINE('',#122020,#15634) ;
#11519=LINE('',#122021,#15635) ;
#11520=LINE('',#122025,#15636) ;
#11521=LINE('',#122030,#15637) ;
#11522=LINE('',#122031,#15638) ;
#11523=LINE('',#122035,#15639) ;
#11524=LINE('',#122040,#15640) ;
#11525=LINE('',#122041,#15641) ;
#11526=LINE('',#122051,#15642) ;
#11527=LINE('',#122053,#15643) ;
#11528=LINE('',#122055,#15644) ;
#11529=LINE('',#122056,#15645) ;
#11530=LINE('',#122060,#15646) ;
#11531=LINE('',#122061,#15647) ;
#11532=LINE('',#122062,#15648) ;
#11533=LINE('',#122065,#15649) ;
#11534=LINE('',#122067,#15650) ;
#11535=LINE('',#122068,#15651) ;
#11536=LINE('',#122072,#15652) ;
#11537=LINE('',#122074,#15653) ;
#11538=LINE('',#122076,#15654) ;
#11539=LINE('',#122077,#15655) ;
#11540=LINE('',#122081,#15656) ;
#11541=LINE('',#122083,#15657) ;
#11542=LINE('',#122085,#15658) ;
#11543=LINE('',#122086,#15659) ;
#11544=LINE('',#122090,#15660) ;
#11545=LINE('',#122091,#15661) ;
#11546=LINE('',#122092,#15662) ;
#11547=LINE('',#122095,#15663) ;
#11548=LINE('',#122097,#15664) ;
#11549=LINE('',#122098,#15665) ;
#11550=LINE('',#122102,#15666) ;
#11551=LINE('',#122104,#15667) ;
#11552=LINE('',#122106,#15668) ;
#11553=LINE('',#122107,#15669) ;
#11554=LINE('',#122111,#15670) ;
#11555=LINE('',#122113,#15671) ;
#11556=LINE('',#122115,#15672) ;
#11557=LINE('',#122116,#15673) ;
#11558=LINE('',#122120,#15674) ;
#11559=LINE('',#122122,#15675) ;
#11560=LINE('',#122124,#15676) ;
#11561=LINE('',#122125,#15677) ;
#11562=LINE('',#122129,#15678) ;
#11563=LINE('',#122131,#15679) ;
#11564=LINE('',#122133,#15680) ;
#11565=LINE('',#122134,#15681) ;
#11566=LINE('',#122138,#15682) ;
#11567=LINE('',#122140,#15683) ;
#11568=LINE('',#122142,#15684) ;
#11569=LINE('',#122143,#15685) ;
#11570=LINE('',#122147,#15686) ;
#11571=LINE('',#122152,#15687) ;
#11572=LINE('',#122153,#15688) ;
#11573=LINE('',#122157,#15689) ;
#11574=LINE('',#122162,#15690) ;
#11575=LINE('',#122163,#15691) ;
#11576=LINE('',#122173,#15692) ;
#11577=LINE('',#122175,#15693) ;
#11578=LINE('',#122177,#15694) ;
#11579=LINE('',#122178,#15695) ;
#11580=LINE('',#122182,#15696) ;
#11581=LINE('',#122183,#15697) ;
#11582=LINE('',#122184,#15698) ;
#11583=LINE('',#122187,#15699) ;
#11584=LINE('',#122189,#15700) ;
#11585=LINE('',#122190,#15701) ;
#11586=LINE('',#122194,#15702) ;
#11587=LINE('',#122196,#15703) ;
#11588=LINE('',#122198,#15704) ;
#11589=LINE('',#122199,#15705) ;
#11590=LINE('',#122203,#15706) ;
#11591=LINE('',#122205,#15707) ;
#11592=LINE('',#122207,#15708) ;
#11593=LINE('',#122208,#15709) ;
#11594=LINE('',#122212,#15710) ;
#11595=LINE('',#122213,#15711) ;
#11596=LINE('',#122214,#15712) ;
#11597=LINE('',#122217,#15713) ;
#11598=LINE('',#122219,#15714) ;
#11599=LINE('',#122220,#15715) ;
#11600=LINE('',#122224,#15716) ;
#11601=LINE('',#122226,#15717) ;
#11602=LINE('',#122228,#15718) ;
#11603=LINE('',#122229,#15719) ;
#11604=LINE('',#122233,#15720) ;
#11605=LINE('',#122235,#15721) ;
#11606=LINE('',#122237,#15722) ;
#11607=LINE('',#122238,#15723) ;
#11608=LINE('',#122242,#15724) ;
#11609=LINE('',#122244,#15725) ;
#11610=LINE('',#122246,#15726) ;
#11611=LINE('',#122247,#15727) ;
#11612=LINE('',#122251,#15728) ;
#11613=LINE('',#122253,#15729) ;
#11614=LINE('',#122255,#15730) ;
#11615=LINE('',#122256,#15731) ;
#11616=LINE('',#122260,#15732) ;
#11617=LINE('',#122262,#15733) ;
#11618=LINE('',#122264,#15734) ;
#11619=LINE('',#122265,#15735) ;
#11620=LINE('',#122269,#15736) ;
#11621=LINE('',#122274,#15737) ;
#11622=LINE('',#122275,#15738) ;
#11623=LINE('',#122279,#15739) ;
#11624=LINE('',#122284,#15740) ;
#11625=LINE('',#122285,#15741) ;
#11626=LINE('',#122295,#15742) ;
#11627=LINE('',#122297,#15743) ;
#11628=LINE('',#122299,#15744) ;
#11629=LINE('',#122300,#15745) ;
#11630=LINE('',#122304,#15746) ;
#11631=LINE('',#122305,#15747) ;
#11632=LINE('',#122306,#15748) ;
#11633=LINE('',#122309,#15749) ;
#11634=LINE('',#122311,#15750) ;
#11635=LINE('',#122312,#15751) ;
#11636=LINE('',#122316,#15752) ;
#11637=LINE('',#122318,#15753) ;
#11638=LINE('',#122320,#15754) ;
#11639=LINE('',#122321,#15755) ;
#11640=LINE('',#122325,#15756) ;
#11641=LINE('',#122327,#15757) ;
#11642=LINE('',#122329,#15758) ;
#11643=LINE('',#122330,#15759) ;
#11644=LINE('',#122334,#15760) ;
#11645=LINE('',#122335,#15761) ;
#11646=LINE('',#122336,#15762) ;
#11647=LINE('',#122339,#15763) ;
#11648=LINE('',#122341,#15764) ;
#11649=LINE('',#122342,#15765) ;
#11650=LINE('',#122346,#15766) ;
#11651=LINE('',#122348,#15767) ;
#11652=LINE('',#122350,#15768) ;
#11653=LINE('',#122351,#15769) ;
#11654=LINE('',#122355,#15770) ;
#11655=LINE('',#122357,#15771) ;
#11656=LINE('',#122359,#15772) ;
#11657=LINE('',#122360,#15773) ;
#11658=LINE('',#122364,#15774) ;
#11659=LINE('',#122366,#15775) ;
#11660=LINE('',#122368,#15776) ;
#11661=LINE('',#122369,#15777) ;
#11662=LINE('',#122373,#15778) ;
#11663=LINE('',#122375,#15779) ;
#11664=LINE('',#122377,#15780) ;
#11665=LINE('',#122378,#15781) ;
#11666=LINE('',#122382,#15782) ;
#11667=LINE('',#122384,#15783) ;
#11668=LINE('',#122386,#15784) ;
#11669=LINE('',#122387,#15785) ;
#11670=LINE('',#122391,#15786) ;
#11671=LINE('',#122396,#15787) ;
#11672=LINE('',#122397,#15788) ;
#11673=LINE('',#122401,#15789) ;
#11674=LINE('',#122406,#15790) ;
#11675=LINE('',#122407,#15791) ;
#11676=LINE('',#122417,#15792) ;
#11677=LINE('',#122419,#15793) ;
#11678=LINE('',#122421,#15794) ;
#11679=LINE('',#122422,#15795) ;
#11680=LINE('',#122426,#15796) ;
#11681=LINE('',#122427,#15797) ;
#11682=LINE('',#122428,#15798) ;
#11683=LINE('',#122431,#15799) ;
#11684=LINE('',#122433,#15800) ;
#11685=LINE('',#122434,#15801) ;
#11686=LINE('',#122438,#15802) ;
#11687=LINE('',#122440,#15803) ;
#11688=LINE('',#122442,#15804) ;
#11689=LINE('',#122443,#15805) ;
#11690=LINE('',#122447,#15806) ;
#11691=LINE('',#122449,#15807) ;
#11692=LINE('',#122451,#15808) ;
#11693=LINE('',#122452,#15809) ;
#11694=LINE('',#122456,#15810) ;
#11695=LINE('',#122457,#15811) ;
#11696=LINE('',#122458,#15812) ;
#11697=LINE('',#122461,#15813) ;
#11698=LINE('',#122463,#15814) ;
#11699=LINE('',#122464,#15815) ;
#11700=LINE('',#122468,#15816) ;
#11701=LINE('',#122470,#15817) ;
#11702=LINE('',#122472,#15818) ;
#11703=LINE('',#122473,#15819) ;
#11704=LINE('',#122477,#15820) ;
#11705=LINE('',#122479,#15821) ;
#11706=LINE('',#122481,#15822) ;
#11707=LINE('',#122482,#15823) ;
#11708=LINE('',#122486,#15824) ;
#11709=LINE('',#122488,#15825) ;
#11710=LINE('',#122490,#15826) ;
#11711=LINE('',#122491,#15827) ;
#11712=LINE('',#122495,#15828) ;
#11713=LINE('',#122497,#15829) ;
#11714=LINE('',#122499,#15830) ;
#11715=LINE('',#122500,#15831) ;
#11716=LINE('',#122504,#15832) ;
#11717=LINE('',#122506,#15833) ;
#11718=LINE('',#122508,#15834) ;
#11719=LINE('',#122509,#15835) ;
#11720=LINE('',#122513,#15836) ;
#11721=LINE('',#122518,#15837) ;
#11722=LINE('',#122519,#15838) ;
#11723=LINE('',#122523,#15839) ;
#11724=LINE('',#122528,#15840) ;
#11725=LINE('',#122529,#15841) ;
#11726=LINE('',#122539,#15842) ;
#11727=LINE('',#122541,#15843) ;
#11728=LINE('',#122543,#15844) ;
#11729=LINE('',#122544,#15845) ;
#11730=LINE('',#122548,#15846) ;
#11731=LINE('',#122549,#15847) ;
#11732=LINE('',#122550,#15848) ;
#11733=LINE('',#122553,#15849) ;
#11734=LINE('',#122555,#15850) ;
#11735=LINE('',#122556,#15851) ;
#11736=LINE('',#122560,#15852) ;
#11737=LINE('',#122562,#15853) ;
#11738=LINE('',#122564,#15854) ;
#11739=LINE('',#122565,#15855) ;
#11740=LINE('',#122569,#15856) ;
#11741=LINE('',#122571,#15857) ;
#11742=LINE('',#122573,#15858) ;
#11743=LINE('',#122574,#15859) ;
#11744=LINE('',#122578,#15860) ;
#11745=LINE('',#122579,#15861) ;
#11746=LINE('',#122580,#15862) ;
#11747=LINE('',#122583,#15863) ;
#11748=LINE('',#122585,#15864) ;
#11749=LINE('',#122586,#15865) ;
#11750=LINE('',#122590,#15866) ;
#11751=LINE('',#122592,#15867) ;
#11752=LINE('',#122594,#15868) ;
#11753=LINE('',#122595,#15869) ;
#11754=LINE('',#122599,#15870) ;
#11755=LINE('',#122601,#15871) ;
#11756=LINE('',#122603,#15872) ;
#11757=LINE('',#122604,#15873) ;
#11758=LINE('',#122608,#15874) ;
#11759=LINE('',#122610,#15875) ;
#11760=LINE('',#122612,#15876) ;
#11761=LINE('',#122613,#15877) ;
#11762=LINE('',#122617,#15878) ;
#11763=LINE('',#122619,#15879) ;
#11764=LINE('',#122621,#15880) ;
#11765=LINE('',#122622,#15881) ;
#11766=LINE('',#122626,#15882) ;
#11767=LINE('',#122628,#15883) ;
#11768=LINE('',#122630,#15884) ;
#11769=LINE('',#122631,#15885) ;
#11770=LINE('',#122635,#15886) ;
#11771=LINE('',#122640,#15887) ;
#11772=LINE('',#122641,#15888) ;
#11773=LINE('',#122645,#15889) ;
#11774=LINE('',#122650,#15890) ;
#11775=LINE('',#122651,#15891) ;
#11776=LINE('',#122661,#15892) ;
#11777=LINE('',#122663,#15893) ;
#11778=LINE('',#122665,#15894) ;
#11779=LINE('',#122666,#15895) ;
#11780=LINE('',#122670,#15896) ;
#11781=LINE('',#122671,#15897) ;
#11782=LINE('',#122672,#15898) ;
#11783=LINE('',#122675,#15899) ;
#11784=LINE('',#122677,#15900) ;
#11785=LINE('',#122678,#15901) ;
#11786=LINE('',#122682,#15902) ;
#11787=LINE('',#122684,#15903) ;
#11788=LINE('',#122686,#15904) ;
#11789=LINE('',#122687,#15905) ;
#11790=LINE('',#122691,#15906) ;
#11791=LINE('',#122693,#15907) ;
#11792=LINE('',#122695,#15908) ;
#11793=LINE('',#122696,#15909) ;
#11794=LINE('',#122700,#15910) ;
#11795=LINE('',#122701,#15911) ;
#11796=LINE('',#122702,#15912) ;
#11797=LINE('',#122705,#15913) ;
#11798=LINE('',#122707,#15914) ;
#11799=LINE('',#122708,#15915) ;
#11800=LINE('',#122712,#15916) ;
#11801=LINE('',#122714,#15917) ;
#11802=LINE('',#122716,#15918) ;
#11803=LINE('',#122717,#15919) ;
#11804=LINE('',#122721,#15920) ;
#11805=LINE('',#122723,#15921) ;
#11806=LINE('',#122725,#15922) ;
#11807=LINE('',#122726,#15923) ;
#11808=LINE('',#122730,#15924) ;
#11809=LINE('',#122732,#15925) ;
#11810=LINE('',#122734,#15926) ;
#11811=LINE('',#122735,#15927) ;
#11812=LINE('',#122739,#15928) ;
#11813=LINE('',#122741,#15929) ;
#11814=LINE('',#122743,#15930) ;
#11815=LINE('',#122744,#15931) ;
#11816=LINE('',#122748,#15932) ;
#11817=LINE('',#122750,#15933) ;
#11818=LINE('',#122752,#15934) ;
#11819=LINE('',#122753,#15935) ;
#11820=LINE('',#122757,#15936) ;
#11821=LINE('',#122759,#15937) ;
#11822=LINE('',#122761,#15938) ;
#11823=LINE('',#122762,#15939) ;
#11824=LINE('',#122766,#15940) ;
#11825=LINE('',#122768,#15941) ;
#11826=LINE('',#122770,#15942) ;
#11827=LINE('',#122771,#15943) ;
#11828=LINE('',#122775,#15944) ;
#11829=LINE('',#122777,#15945) ;
#11830=LINE('',#122779,#15946) ;
#11831=LINE('',#122780,#15947) ;
#11832=LINE('',#122784,#15948) ;
#11833=LINE('',#122786,#15949) ;
#11834=LINE('',#122788,#15950) ;
#11835=LINE('',#122789,#15951) ;
#11836=LINE('',#122793,#15952) ;
#11837=LINE('',#122795,#15953) ;
#11838=LINE('',#122797,#15954) ;
#11839=LINE('',#122798,#15955) ;
#11840=LINE('',#122802,#15956) ;
#11841=LINE('',#122804,#15957) ;
#11842=LINE('',#122806,#15958) ;
#11843=LINE('',#122807,#15959) ;
#11844=LINE('',#122811,#15960) ;
#11845=LINE('',#122813,#15961) ;
#11846=LINE('',#122815,#15962) ;
#11847=LINE('',#122816,#15963) ;
#11848=LINE('',#122820,#15964) ;
#11849=LINE('',#122822,#15965) ;
#11850=LINE('',#122824,#15966) ;
#11851=LINE('',#122825,#15967) ;
#11852=LINE('',#122829,#15968) ;
#11853=LINE('',#122831,#15969) ;
#11854=LINE('',#122833,#15970) ;
#11855=LINE('',#122834,#15971) ;
#11856=LINE('',#122838,#15972) ;
#11857=LINE('',#122840,#15973) ;
#11858=LINE('',#122842,#15974) ;
#11859=LINE('',#122843,#15975) ;
#11860=LINE('',#122847,#15976) ;
#11861=LINE('',#122849,#15977) ;
#11862=LINE('',#122851,#15978) ;
#11863=LINE('',#122852,#15979) ;
#11864=LINE('',#122856,#15980) ;
#11865=LINE('',#122858,#15981) ;
#11866=LINE('',#122860,#15982) ;
#11867=LINE('',#122861,#15983) ;
#11868=LINE('',#122865,#15984) ;
#11869=LINE('',#122867,#15985) ;
#11870=LINE('',#122869,#15986) ;
#11871=LINE('',#122870,#15987) ;
#11872=LINE('',#122874,#15988) ;
#11873=LINE('',#122876,#15989) ;
#11874=LINE('',#122878,#15990) ;
#11875=LINE('',#122879,#15991) ;
#11876=LINE('',#122883,#15992) ;
#11877=LINE('',#122885,#15993) ;
#11878=LINE('',#122887,#15994) ;
#11879=LINE('',#122888,#15995) ;
#11880=LINE('',#122892,#15996) ;
#11881=LINE('',#122894,#15997) ;
#11882=LINE('',#122896,#15998) ;
#11883=LINE('',#122897,#15999) ;
#11884=LINE('',#122901,#16000) ;
#11885=LINE('',#122903,#16001) ;
#11886=LINE('',#122905,#16002) ;
#11887=LINE('',#122906,#16003) ;
#11888=LINE('',#122910,#16004) ;
#11889=LINE('',#122912,#16005) ;
#11890=LINE('',#122914,#16006) ;
#11891=LINE('',#122915,#16007) ;
#11892=LINE('',#122919,#16008) ;
#11893=LINE('',#122921,#16009) ;
#11894=LINE('',#122923,#16010) ;
#11895=LINE('',#122924,#16011) ;
#11896=LINE('',#122928,#16012) ;
#11897=LINE('',#122930,#16013) ;
#11898=LINE('',#122932,#16014) ;
#11899=LINE('',#122933,#16015) ;
#11900=LINE('',#122937,#16016) ;
#11901=LINE('',#122939,#16017) ;
#11902=LINE('',#122941,#16018) ;
#11903=LINE('',#122942,#16019) ;
#11904=LINE('',#122946,#16020) ;
#11905=LINE('',#122948,#16021) ;
#11906=LINE('',#122950,#16022) ;
#11907=LINE('',#122951,#16023) ;
#11908=LINE('',#122955,#16024) ;
#11909=LINE('',#122957,#16025) ;
#11910=LINE('',#122959,#16026) ;
#11911=LINE('',#122960,#16027) ;
#11912=LINE('',#122964,#16028) ;
#11913=LINE('',#122966,#16029) ;
#11914=LINE('',#122968,#16030) ;
#11915=LINE('',#122969,#16031) ;
#11916=LINE('',#122973,#16032) ;
#11917=LINE('',#122975,#16033) ;
#11918=LINE('',#122977,#16034) ;
#11919=LINE('',#122978,#16035) ;
#11920=LINE('',#122982,#16036) ;
#11921=LINE('',#122984,#16037) ;
#11922=LINE('',#122986,#16038) ;
#11923=LINE('',#122987,#16039) ;
#11924=LINE('',#122991,#16040) ;
#11925=LINE('',#122993,#16041) ;
#11926=LINE('',#122995,#16042) ;
#11927=LINE('',#122996,#16043) ;
#11928=LINE('',#123000,#16044) ;
#11929=LINE('',#123002,#16045) ;
#11930=LINE('',#123004,#16046) ;
#11931=LINE('',#123005,#16047) ;
#11932=LINE('',#123009,#16048) ;
#11933=LINE('',#123011,#16049) ;
#11934=LINE('',#123013,#16050) ;
#11935=LINE('',#123014,#16051) ;
#11936=LINE('',#123018,#16052) ;
#11937=LINE('',#123020,#16053) ;
#11938=LINE('',#123022,#16054) ;
#11939=LINE('',#123023,#16055) ;
#11940=LINE('',#123027,#16056) ;
#11941=LINE('',#123029,#16057) ;
#11942=LINE('',#123031,#16058) ;
#11943=LINE('',#123032,#16059) ;
#13922=VECTOR('',#87002,1000.) ;
#13923=VECTOR('',#87005,1000.) ;
#13924=VECTOR('',#87006,1000.) ;
#13925=VECTOR('',#87039,1000.) ;
#13926=VECTOR('',#87042,1000.) ;
#13927=VECTOR('',#87043,1000.) ;
#13928=VECTOR('',#87076,1000.) ;
#13929=VECTOR('',#87079,1000.) ;
#13930=VECTOR('',#87080,1000.) ;
#13931=VECTOR('',#87113,1000.) ;
#13932=VECTOR('',#87116,1000.) ;
#13933=VECTOR('',#87117,1000.) ;
#13934=VECTOR('',#87150,1000.) ;
#13935=VECTOR('',#87153,1000.) ;
#13936=VECTOR('',#87154,1000.) ;
#13937=VECTOR('',#87187,1000.) ;
#13938=VECTOR('',#87190,1000.) ;
#13939=VECTOR('',#87191,1000.) ;
#13940=VECTOR('',#87224,1000.) ;
#13941=VECTOR('',#87227,1000.) ;
#13942=VECTOR('',#87228,1000.) ;
#13943=VECTOR('',#87261,1000.) ;
#13944=VECTOR('',#87264,1000.) ;
#13945=VECTOR('',#87265,1000.) ;
#13946=VECTOR('',#87388,1000.) ;
#13947=VECTOR('',#87391,1000.) ;
#13948=VECTOR('',#87392,1000.) ;
#13949=VECTOR('',#87395,1.) ;
#13950=VECTOR('',#87398,1.) ;
#13951=VECTOR('',#87401,1.) ;
#13952=VECTOR('',#87404,1.) ;
#13953=VECTOR('',#87407,1.) ;
#13954=VECTOR('',#87410,0.999999999999999) ;
#13955=VECTOR('',#87413,0.999999999999999) ;
#13956=VECTOR('',#87416,1.) ;
#13957=VECTOR('',#87419,1.) ;
#13958=VECTOR('',#87424,1000.) ;
#13959=VECTOR('',#87425,1000.) ;
#13960=VECTOR('',#87430,1000.) ;
#13961=VECTOR('',#87431,1000.) ;
#13962=VECTOR('',#87436,1000.) ;
#13963=VECTOR('',#87437,1000.) ;
#13964=VECTOR('',#87442,1000.) ;
#13965=VECTOR('',#87443,1000.) ;
#13966=VECTOR('',#87448,1000.) ;
#13967=VECTOR('',#87449,1000.) ;
#13968=VECTOR('',#87454,1000.) ;
#13969=VECTOR('',#87455,1000.) ;
#13970=VECTOR('',#87460,1000.) ;
#13971=VECTOR('',#87461,1000.) ;
#13972=VECTOR('',#87466,1000.) ;
#13973=VECTOR('',#87467,1000.) ;
#13974=VECTOR('',#87472,1000.) ;
#13975=VECTOR('',#87473,1000.) ;
#13976=VECTOR('',#87516,1000.) ;
#13977=VECTOR('',#87519,1000.) ;
#13978=VECTOR('',#87520,1000.) ;
#13979=VECTOR('',#87523,1.) ;
#13980=VECTOR('',#87528,1000.) ;
#13981=VECTOR('',#87529,1000.) ;
#13982=VECTOR('',#87532,1000.) ;
#13983=VECTOR('',#87535,1000.) ;
#13984=VECTOR('',#87540,1000.) ;
#13985=VECTOR('',#87541,1000.) ;
#13986=VECTOR('',#87542,1000.) ;
#13987=VECTOR('',#87543,1000.) ;
#13988=VECTOR('',#87544,1000.) ;
#13989=VECTOR('',#87549,1000.) ;
#13990=VECTOR('',#87552,1000.) ;
#13991=VECTOR('',#87557,1000.) ;
#13992=VECTOR('',#87558,1000.) ;
#13993=VECTOR('',#87559,1000.) ;
#13994=VECTOR('',#87560,1000.) ;
#13995=VECTOR('',#87561,1000.) ;
#13996=VECTOR('',#87566,1000.) ;
#13997=VECTOR('',#87569,1000.) ;
#13998=VECTOR('',#87574,1000.) ;
#13999=VECTOR('',#87575,1000.) ;
#14000=VECTOR('',#87576,1000.) ;
#14001=VECTOR('',#87577,1000.) ;
#14002=VECTOR('',#87578,1000.) ;
#14003=VECTOR('',#87583,1000.) ;
#14004=VECTOR('',#87586,1000.) ;
#14005=VECTOR('',#87591,1000.) ;
#14006=VECTOR('',#87592,1000.) ;
#14007=VECTOR('',#87593,1000.) ;
#14008=VECTOR('',#87594,1000.) ;
#14009=VECTOR('',#87595,1000.) ;
#14010=VECTOR('',#87600,1000.) ;
#14011=VECTOR('',#87603,1000.) ;
#14012=VECTOR('',#87608,1000.) ;
#14013=VECTOR('',#87609,1000.) ;
#14014=VECTOR('',#87610,1000.) ;
#14015=VECTOR('',#87611,1000.) ;
#14016=VECTOR('',#87612,1000.) ;
#14017=VECTOR('',#87617,1000.) ;
#14018=VECTOR('',#87620,1000.) ;
#14019=VECTOR('',#87625,1000.) ;
#14020=VECTOR('',#87626,1000.) ;
#14021=VECTOR('',#87627,1000.) ;
#14022=VECTOR('',#87628,1000.) ;
#14023=VECTOR('',#87629,1000.) ;
#14024=VECTOR('',#87634,1000.) ;
#14025=VECTOR('',#87637,1000.) ;
#14026=VECTOR('',#87642,1000.) ;
#14027=VECTOR('',#87643,1000.) ;
#14028=VECTOR('',#87644,1000.) ;
#14029=VECTOR('',#87645,1000.) ;
#14030=VECTOR('',#87646,1000.) ;
#14031=VECTOR('',#87651,1000.) ;
#14032=VECTOR('',#87654,1000.) ;
#14033=VECTOR('',#87659,1000.) ;
#14034=VECTOR('',#87660,1000.) ;
#14035=VECTOR('',#87661,1000.) ;
#14036=VECTOR('',#87662,1000.) ;
#14037=VECTOR('',#87663,1000.) ;
#14038=VECTOR('',#87668,1000.) ;
#14039=VECTOR('',#87671,1000.) ;
#14040=VECTOR('',#87676,1000.) ;
#14041=VECTOR('',#87677,1000.) ;
#14042=VECTOR('',#87678,1000.) ;
#14043=VECTOR('',#87679,1000.) ;
#14044=VECTOR('',#87680,1000.) ;
#14045=VECTOR('',#87687,1000.) ;
#14046=VECTOR('',#87688,1000.) ;
#14047=VECTOR('',#87689,1000.) ;
#14048=VECTOR('',#87690,1000.) ;
#14049=VECTOR('',#87695,1000.) ;
#14050=VECTOR('',#87696,1000.) ;
#14051=VECTOR('',#87697,1000.) ;
#14052=VECTOR('',#87698,1000.) ;
#14053=VECTOR('',#87703,1000.) ;
#14054=VECTOR('',#87704,1000.) ;
#14055=VECTOR('',#87705,1000.) ;
#14056=VECTOR('',#87706,1000.) ;
#14057=VECTOR('',#87711,1000.) ;
#14058=VECTOR('',#87712,1000.) ;
#14059=VECTOR('',#87713,1000.) ;
#14060=VECTOR('',#87714,1000.) ;
#14061=VECTOR('',#87719,1000.) ;
#14062=VECTOR('',#87720,1000.) ;
#14063=VECTOR('',#87721,1000.) ;
#14064=VECTOR('',#87722,1000.) ;
#14065=VECTOR('',#87727,1000.) ;
#14066=VECTOR('',#87728,1000.) ;
#14067=VECTOR('',#87729,1000.) ;
#14068=VECTOR('',#87730,1000.) ;
#14069=VECTOR('',#87735,1000.) ;
#14070=VECTOR('',#87736,1000.) ;
#14071=VECTOR('',#87737,1000.) ;
#14072=VECTOR('',#87738,1000.) ;
#14073=VECTOR('',#87743,1000.) ;
#14074=VECTOR('',#87744,1000.) ;
#14075=VECTOR('',#87745,1000.) ;
#14076=VECTOR('',#87746,1000.) ;
#14077=VECTOR('',#87751,1000.) ;
#14078=VECTOR('',#87752,1000.) ;
#14079=VECTOR('',#87753,1000.) ;
#14080=VECTOR('',#87754,1000.) ;
#14081=VECTOR('',#87759,1000.) ;
#14082=VECTOR('',#87760,1000.) ;
#14083=VECTOR('',#87761,1000.) ;
#14084=VECTOR('',#87762,1000.) ;
#14085=VECTOR('',#87767,1000.) ;
#14086=VECTOR('',#87768,1000.) ;
#14087=VECTOR('',#87769,1000.) ;
#14088=VECTOR('',#87770,1000.) ;
#14089=VECTOR('',#87775,1000.) ;
#14090=VECTOR('',#87776,1000.) ;
#14091=VECTOR('',#87777,1000.) ;
#14092=VECTOR('',#87778,1000.) ;
#14093=VECTOR('',#87783,1000.) ;
#14094=VECTOR('',#87784,1000.) ;
#14095=VECTOR('',#87785,1000.) ;
#14096=VECTOR('',#87786,1000.) ;
#14097=VECTOR('',#87791,1000.) ;
#14098=VECTOR('',#87792,1000.) ;
#14099=VECTOR('',#87793,1000.) ;
#14100=VECTOR('',#87794,1000.) ;
#14101=VECTOR('',#87799,1000.) ;
#14102=VECTOR('',#87800,1000.) ;
#14103=VECTOR('',#87801,1000.) ;
#14104=VECTOR('',#87802,1000.) ;
#14105=VECTOR('',#87807,1000.) ;
#14106=VECTOR('',#87808,1000.) ;
#14107=VECTOR('',#87809,1000.) ;
#14108=VECTOR('',#87810,1000.) ;
#14109=VECTOR('',#87815,1000.) ;
#14110=VECTOR('',#87816,1000.) ;
#14111=VECTOR('',#87817,1000.) ;
#14112=VECTOR('',#87818,1000.) ;
#14113=VECTOR('',#87823,1000.) ;
#14114=VECTOR('',#87824,1000.) ;
#14115=VECTOR('',#87825,1000.) ;
#14116=VECTOR('',#87826,1000.) ;
#14117=VECTOR('',#87829,1000.) ;
#14118=VECTOR('',#87832,1000.) ;
#14119=VECTOR('',#87837,1000.) ;
#14120=VECTOR('',#87840,1000.) ;
#14121=VECTOR('',#87845,1000.) ;
#14122=VECTOR('',#87848,1000.) ;
#14123=VECTOR('',#87853,1000.) ;
#14124=VECTOR('',#87856,1000.) ;
#14125=VECTOR('',#87861,1000.) ;
#14126=VECTOR('',#87864,1000.) ;
#14127=VECTOR('',#87869,1000.) ;
#14128=VECTOR('',#87872,1000.) ;
#14129=VECTOR('',#87877,1000.) ;
#14130=VECTOR('',#87880,1000.) ;
#14131=VECTOR('',#87885,1000.) ;
#14132=VECTOR('',#87888,1000.) ;
#14133=VECTOR('',#87893,1000.) ;
#14134=VECTOR('',#87896,1000.) ;
#14135=VECTOR('',#87901,1000.) ;
#14136=VECTOR('',#87904,1000.) ;
#14137=VECTOR('',#87909,1000.) ;
#14138=VECTOR('',#87910,1000.) ;
#14139=VECTOR('',#87911,1000.) ;
#14140=VECTOR('',#87912,1000.) ;
#14141=VECTOR('',#87913,1000.) ;
#14142=VECTOR('',#87920,1000.) ;
#14143=VECTOR('',#87921,1000.) ;
#14144=VECTOR('',#87922,1000.) ;
#14145=VECTOR('',#87923,1000.) ;
#14146=VECTOR('',#87928,1000.) ;
#14147=VECTOR('',#87929,1000.) ;
#14148=VECTOR('',#87930,1000.) ;
#14149=VECTOR('',#87931,1000.) ;
#14150=VECTOR('',#87934,1000.) ;
#14151=VECTOR('',#87937,1000.) ;
#14152=VECTOR('',#87942,1000.) ;
#14153=VECTOR('',#87945,1000.) ;
#14154=VECTOR('',#87952,1000.) ;
#14155=VECTOR('',#87953,1000.) ;
#14156=VECTOR('',#87954,1000.) ;
#14157=VECTOR('',#87955,1000.) ;
#14158=VECTOR('',#87956,1000.) ;
#14159=VECTOR('',#87959,1000.) ;
#14160=VECTOR('',#87962,1000.) ;
#14161=VECTOR('',#87963,1000.) ;
#14162=VECTOR('',#87966,1000.) ;
#14163=VECTOR('',#87969,1000.) ;
#14164=VECTOR('',#87970,1000.) ;
#14165=VECTOR('',#87973,1000.) ;
#14166=VECTOR('',#87976,1000.) ;
#14167=VECTOR('',#87977,1000.) ;
#14168=VECTOR('',#87980,1000.) ;
#14169=VECTOR('',#87983,1000.) ;
#14170=VECTOR('',#87984,1000.) ;
#14171=VECTOR('',#87987,1000.) ;
#14172=VECTOR('',#87990,1000.) ;
#14173=VECTOR('',#87991,1000.) ;
#14174=VECTOR('',#87994,1000.) ;
#14175=VECTOR('',#87997,1000.) ;
#14176=VECTOR('',#87998,1000.) ;
#14177=VECTOR('',#88001,1000.) ;
#14178=VECTOR('',#88004,1000.) ;
#14179=VECTOR('',#88005,1000.) ;
#14180=VECTOR('',#88008,1000.) ;
#14181=VECTOR('',#88011,1000.) ;
#14182=VECTOR('',#88012,1000.) ;
#14183=VECTOR('',#88015,1000.) ;
#14184=VECTOR('',#88018,1000.) ;
#14185=VECTOR('',#88019,1000.) ;
#14186=VECTOR('',#88022,1000.) ;
#14187=VECTOR('',#88027,1000.) ;
#14188=VECTOR('',#88034,1000.) ;
#14189=VECTOR('',#88035,1000.) ;
#14190=VECTOR('',#88038,1000.) ;
#14191=VECTOR('',#88041,1000.) ;
#14192=VECTOR('',#88042,1000.) ;
#14193=VECTOR('',#88045,1000.) ;
#14194=VECTOR('',#88048,1000.) ;
#14195=VECTOR('',#88049,1000.) ;
#14196=VECTOR('',#88052,1000.) ;
#14197=VECTOR('',#88055,1000.) ;
#14198=VECTOR('',#88056,1000.) ;
#14199=VECTOR('',#88059,1000.) ;
#14200=VECTOR('',#88062,1000.) ;
#14201=VECTOR('',#88063,1000.) ;
#14202=VECTOR('',#88066,1000.) ;
#14203=VECTOR('',#88069,1000.) ;
#14204=VECTOR('',#88070,1000.) ;
#14205=VECTOR('',#88073,1000.) ;
#14206=VECTOR('',#88076,1000.) ;
#14207=VECTOR('',#88077,1000.) ;
#14208=VECTOR('',#88080,1000.) ;
#14209=VECTOR('',#88083,1000.) ;
#14210=VECTOR('',#88084,1000.) ;
#14211=VECTOR('',#88087,1000.) ;
#14212=VECTOR('',#88090,1000.) ;
#14213=VECTOR('',#88091,1000.) ;
#14214=VECTOR('',#88094,1000.) ;
#14215=VECTOR('',#88097,1000.) ;
#14216=VECTOR('',#88098,1000.) ;
#14217=VECTOR('',#88099,1000.) ;
#14218=VECTOR('',#88100,1000.) ;
#14219=VECTOR('',#88101,1000.) ;
#14220=VECTOR('',#88104,1000.) ;
#14221=VECTOR('',#88107,1000.) ;
#14222=VECTOR('',#88114,1000.) ;
#14223=VECTOR('',#88115,1000.) ;
#14224=VECTOR('',#88116,1000.) ;
#14225=VECTOR('',#88119,1000.) ;
#14226=VECTOR('',#88126,1000.) ;
#14227=VECTOR('',#88127,1000.) ;
#14228=VECTOR('',#88128,1000.) ;
#14229=VECTOR('',#88131,1000.) ;
#14230=VECTOR('',#88138,1000.) ;
#14231=VECTOR('',#88139,1000.) ;
#14232=VECTOR('',#88140,1000.) ;
#14233=VECTOR('',#88143,1000.) ;
#14234=VECTOR('',#88150,1000.) ;
#14235=VECTOR('',#88151,1000.) ;
#14236=VECTOR('',#88152,1000.) ;
#14237=VECTOR('',#88155,1000.) ;
#14238=VECTOR('',#88162,1000.) ;
#14239=VECTOR('',#88163,1000.) ;
#14240=VECTOR('',#88164,1000.) ;
#14241=VECTOR('',#88167,1000.) ;
#14242=VECTOR('',#88174,1000.) ;
#14243=VECTOR('',#88175,1000.) ;
#14244=VECTOR('',#88178,1000.) ;
#14245=VECTOR('',#88179,1000.) ;
#14246=VECTOR('',#88180,1000.) ;
#14247=VECTOR('',#88183,1000.) ;
#14248=VECTOR('',#88186,1000.) ;
#14249=VECTOR('',#88187,1000.) ;
#14250=VECTOR('',#88190,1000.) ;
#14251=VECTOR('',#88191,1000.) ;
#14252=VECTOR('',#88192,1000.) ;
#14253=VECTOR('',#88195,1000.) ;
#14254=VECTOR('',#88198,1000.) ;
#14255=VECTOR('',#88205,1000.) ;
#14256=VECTOR('',#88208,1000.) ;
#14257=VECTOR('',#88211,1000.) ;
#14258=VECTOR('',#88212,1000.) ;
#14259=VECTOR('',#88213,1000.) ;
#14260=VECTOR('',#88216,1000.) ;
#14261=VECTOR('',#88219,1000.) ;
#14262=VECTOR('',#88220,1000.) ;
#14263=VECTOR('',#88223,1000.) ;
#14264=VECTOR('',#88224,1000.) ;
#14265=VECTOR('',#88225,1000.) ;
#14266=VECTOR('',#88228,1000.) ;
#14267=VECTOR('',#88231,1000.) ;
#14268=VECTOR('',#88238,1000.) ;
#14269=VECTOR('',#88241,1000.) ;
#14270=VECTOR('',#88244,1000.) ;
#14271=VECTOR('',#88245,1000.) ;
#14272=VECTOR('',#88246,1000.) ;
#14273=VECTOR('',#88249,1000.) ;
#14274=VECTOR('',#88252,1000.) ;
#14275=VECTOR('',#88253,1000.) ;
#14276=VECTOR('',#88256,1000.) ;
#14277=VECTOR('',#88257,1000.) ;
#14278=VECTOR('',#88258,1000.) ;
#14279=VECTOR('',#88261,1000.) ;
#14280=VECTOR('',#88264,1000.) ;
#14281=VECTOR('',#88271,1000.) ;
#14282=VECTOR('',#88274,1000.) ;
#14283=VECTOR('',#88277,1000.) ;
#14284=VECTOR('',#88278,1000.) ;
#14285=VECTOR('',#88279,1000.) ;
#14286=VECTOR('',#88282,1000.) ;
#14287=VECTOR('',#88285,1000.) ;
#14288=VECTOR('',#88286,1000.) ;
#14289=VECTOR('',#88289,1000.) ;
#14290=VECTOR('',#88290,1000.) ;
#14291=VECTOR('',#88291,1000.) ;
#14292=VECTOR('',#88294,1000.) ;
#14293=VECTOR('',#88297,1000.) ;
#14294=VECTOR('',#88304,1000.) ;
#14295=VECTOR('',#88307,1000.) ;
#14296=VECTOR('',#88310,1000.) ;
#14297=VECTOR('',#88311,1000.) ;
#14298=VECTOR('',#88312,1000.) ;
#14299=VECTOR('',#88315,1000.) ;
#14300=VECTOR('',#88318,1000.) ;
#14301=VECTOR('',#88319,1000.) ;
#14302=VECTOR('',#88322,1000.) ;
#14303=VECTOR('',#88323,1000.) ;
#14304=VECTOR('',#88324,1000.) ;
#14305=VECTOR('',#88327,1000.) ;
#14306=VECTOR('',#88330,1000.) ;
#14307=VECTOR('',#88337,1000.) ;
#14308=VECTOR('',#88340,1000.) ;
#14309=VECTOR('',#88343,1000.) ;
#14310=VECTOR('',#88344,1000.) ;
#14311=VECTOR('',#88345,1000.) ;
#14312=VECTOR('',#88348,1000.) ;
#14313=VECTOR('',#88351,1000.) ;
#14314=VECTOR('',#88352,1000.) ;
#14315=VECTOR('',#88355,1000.) ;
#14316=VECTOR('',#88356,1000.) ;
#14317=VECTOR('',#88357,1000.) ;
#14318=VECTOR('',#88360,1000.) ;
#14319=VECTOR('',#88363,1000.) ;
#14320=VECTOR('',#88370,1000.) ;
#14321=VECTOR('',#88373,1000.) ;
#14322=VECTOR('',#88376,1000.) ;
#14323=VECTOR('',#88377,1000.) ;
#14324=VECTOR('',#88378,1000.) ;
#14325=VECTOR('',#88381,1000.) ;
#14326=VECTOR('',#88384,1000.) ;
#14327=VECTOR('',#88385,1000.) ;
#14328=VECTOR('',#88388,1000.) ;
#14329=VECTOR('',#88389,1000.) ;
#14330=VECTOR('',#88390,1000.) ;
#14331=VECTOR('',#88393,1000.) ;
#14332=VECTOR('',#88396,1000.) ;
#14333=VECTOR('',#88403,1000.) ;
#14334=VECTOR('',#88406,1000.) ;
#14335=VECTOR('',#88409,1000.) ;
#14336=VECTOR('',#88410,1000.) ;
#14337=VECTOR('',#88411,1000.) ;
#14338=VECTOR('',#88414,1000.) ;
#14339=VECTOR('',#88417,1000.) ;
#14340=VECTOR('',#88418,1000.) ;
#14341=VECTOR('',#88421,1000.) ;
#14342=VECTOR('',#88422,1000.) ;
#14343=VECTOR('',#88423,1000.) ;
#14344=VECTOR('',#88426,1000.) ;
#14345=VECTOR('',#88429,1000.) ;
#14346=VECTOR('',#88436,1000.) ;
#14347=VECTOR('',#88439,1000.) ;
#14348=VECTOR('',#88442,1000.) ;
#14349=VECTOR('',#88443,1000.) ;
#14350=VECTOR('',#88444,1000.) ;
#14351=VECTOR('',#88447,1000.) ;
#14352=VECTOR('',#88450,1000.) ;
#14353=VECTOR('',#88451,1000.) ;
#14354=VECTOR('',#88454,1000.) ;
#14355=VECTOR('',#88455,1000.) ;
#14356=VECTOR('',#88456,1000.) ;
#14357=VECTOR('',#88459,1000.) ;
#14358=VECTOR('',#88462,1000.) ;
#14359=VECTOR('',#88469,1000.) ;
#14360=VECTOR('',#88472,1000.) ;
#14361=VECTOR('',#88475,1000.) ;
#14362=VECTOR('',#88476,1000.) ;
#14363=VECTOR('',#88477,1000.) ;
#14364=VECTOR('',#88480,1000.) ;
#14365=VECTOR('',#88483,1000.) ;
#14366=VECTOR('',#88484,1000.) ;
#14367=VECTOR('',#88487,1000.) ;
#14368=VECTOR('',#88488,1000.) ;
#14369=VECTOR('',#88489,1000.) ;
#14370=VECTOR('',#88492,1000.) ;
#14371=VECTOR('',#88495,1000.) ;
#14372=VECTOR('',#88502,1000.) ;
#14373=VECTOR('',#88505,1000.) ;
#14374=VECTOR('',#88508,1000.) ;
#14375=VECTOR('',#88509,1000.) ;
#14376=VECTOR('',#88510,1000.) ;
#14377=VECTOR('',#88511,1000.) ;
#14378=VECTOR('',#88514,1000.) ;
#14379=VECTOR('',#88515,1000.) ;
#14380=VECTOR('',#88516,1000.) ;
#14381=VECTOR('',#88519,1000.) ;
#14382=VECTOR('',#88522,1000.) ;
#14383=VECTOR('',#88523,1000.) ;
#14384=VECTOR('',#88524,1000.) ;
#14385=VECTOR('',#88525,1000.) ;
#14386=VECTOR('',#88528,1000.) ;
#14387=VECTOR('',#88529,1000.) ;
#14388=VECTOR('',#88530,1000.) ;
#14389=VECTOR('',#88533,1000.) ;
#14390=VECTOR('',#88536,1000.) ;
#14391=VECTOR('',#88537,1000.) ;
#14392=VECTOR('',#88538,1000.) ;
#14393=VECTOR('',#88539,1000.) ;
#14394=VECTOR('',#88540,1000.) ;
#14395=VECTOR('',#88541,1000.) ;
#14396=VECTOR('',#88544,1000.) ;
#14397=VECTOR('',#88547,1000.) ;
#14398=VECTOR('',#88550,1000.) ;
#14399=VECTOR('',#88551,1000.) ;
#14400=VECTOR('',#88552,1000.) ;
#14401=VECTOR('',#88553,1000.) ;
#14402=VECTOR('',#88556,1000.) ;
#14403=VECTOR('',#88557,1000.) ;
#14404=VECTOR('',#88558,1000.) ;
#14405=VECTOR('',#88561,1000.) ;
#14406=VECTOR('',#88562,1000.) ;
#14407=VECTOR('',#88563,1000.) ;
#14408=VECTOR('',#88564,1000.) ;
#14409=VECTOR('',#88567,1000.) ;
#14410=VECTOR('',#88568,1000.) ;
#14411=VECTOR('',#88569,1000.) ;
#14412=VECTOR('',#88570,1000.) ;
#14413=VECTOR('',#88573,1000.) ;
#14414=VECTOR('',#88574,1000.) ;
#14415=VECTOR('',#88575,1000.) ;
#14416=VECTOR('',#88576,1000.) ;
#14417=VECTOR('',#88579,1000.) ;
#14418=VECTOR('',#88582,1000.) ;
#14419=VECTOR('',#88587,1000.) ;
#14420=VECTOR('',#88588,1000.) ;
#14421=VECTOR('',#88589,1000.) ;
#14422=VECTOR('',#88594,1000.) ;
#14423=VECTOR('',#88599,1000.) ;
#14424=VECTOR('',#88600,1000.) ;
#14425=VECTOR('',#88601,1000.) ;
#14426=VECTOR('',#88606,1000.) ;
#14427=VECTOR('',#88611,1000.) ;
#14428=VECTOR('',#88612,1000.) ;
#14429=VECTOR('',#88613,1000.) ;
#14430=VECTOR('',#88616,1000.) ;
#14431=VECTOR('',#88621,1000.) ;
#14432=VECTOR('',#88622,1000.) ;
#14433=VECTOR('',#88625,1000.) ;
#14434=VECTOR('',#88626,1000.) ;
#14435=VECTOR('',#88627,1000.) ;
#14436=VECTOR('',#88632,1000.) ;
#14437=VECTOR('',#88637,1000.) ;
#14438=VECTOR('',#88638,1000.) ;
#14439=VECTOR('',#88639,1000.) ;
#14440=VECTOR('',#88644,1000.) ;
#14441=VECTOR('',#88649,1000.) ;
#14442=VECTOR('',#88650,1000.) ;
#14443=VECTOR('',#88651,1000.) ;
#14444=VECTOR('',#88656,1000.) ;
#14445=VECTOR('',#88661,1000.) ;
#14446=VECTOR('',#88662,1000.) ;
#14447=VECTOR('',#88663,1000.) ;
#14448=VECTOR('',#88668,1000.) ;
#14449=VECTOR('',#88673,1000.) ;
#14450=VECTOR('',#88674,1000.) ;
#14451=VECTOR('',#88675,1000.) ;
#14452=VECTOR('',#88680,1000.) ;
#14453=VECTOR('',#88685,1000.) ;
#14454=VECTOR('',#88686,1000.) ;
#14455=VECTOR('',#88687,1000.) ;
#14456=VECTOR('',#88692,1000.) ;
#14457=VECTOR('',#88699,1000.) ;
#14458=VECTOR('',#88706,1000.) ;
#14459=VECTOR('',#88711,1000.) ;
#14460=VECTOR('',#88712,1000.) ;
#14461=VECTOR('',#88713,1000.) ;
#14462=VECTOR('',#88718,1000.) ;
#14463=VECTOR('',#88723,1000.) ;
#14464=VECTOR('',#88724,1000.) ;
#14465=VECTOR('',#88725,1000.) ;
#14466=VECTOR('',#88730,1000.) ;
#14467=VECTOR('',#88735,1000.) ;
#14468=VECTOR('',#88736,1000.) ;
#14469=VECTOR('',#88741,1000.) ;
#14470=VECTOR('',#88744,1000.) ;
#14471=VECTOR('',#88745,1000.) ;
#14472=VECTOR('',#88746,1000.) ;
#14473=VECTOR('',#88749,1000.) ;
#14474=VECTOR('',#88750,1000.) ;
#14475=VECTOR('',#88751,1000.) ;
#14476=VECTOR('',#88754,1000.) ;
#14477=VECTOR('',#88757,1000.) ;
#14478=VECTOR('',#88758,1000.) ;
#14479=VECTOR('',#88759,1000.) ;
#14480=VECTOR('',#88760,1000.) ;
#14481=VECTOR('',#88761,1000.) ;
#14482=VECTOR('',#88764,1000.) ;
#14483=VECTOR('',#88767,1000.) ;
#14484=VECTOR('',#88770,1000.) ;
#14485=VECTOR('',#88773,1000.) ;
#14486=VECTOR('',#88808,1000.) ;
#14487=VECTOR('',#88811,1000.) ;
#14488=VECTOR('',#88858,1000.) ;
#14489=VECTOR('',#88917,1000.) ;
#14490=VECTOR('',#88966,1000.) ;
#14491=VECTOR('',#89323,1000.) ;
#14492=VECTOR('',#89324,1000.) ;
#14493=VECTOR('',#89325,1000.) ;
#14494=VECTOR('',#89326,1000.) ;
#14495=VECTOR('',#89329,1000.) ;
#14496=VECTOR('',#89330,1000.) ;
#14497=VECTOR('',#89331,1000.) ;
#14498=VECTOR('',#89332,1000.) ;
#14499=VECTOR('',#89335,1000.) ;
#14500=VECTOR('',#89336,1000.) ;
#14501=VECTOR('',#89337,1000.) ;
#14502=VECTOR('',#89338,1000.) ;
#14503=VECTOR('',#89341,1000.) ;
#14504=VECTOR('',#89342,1000.) ;
#14505=VECTOR('',#89343,1000.) ;
#14506=VECTOR('',#89344,1000.) ;
#14507=VECTOR('',#89347,1000.) ;
#14508=VECTOR('',#89348,1000.) ;
#14509=VECTOR('',#89349,1000.) ;
#14510=VECTOR('',#89350,1000.) ;
#14511=VECTOR('',#89353,1000.) ;
#14512=VECTOR('',#89358,1000.) ;
#14513=VECTOR('',#89359,1000.) ;
#14514=VECTOR('',#89362,1000.) ;
#14515=VECTOR('',#89367,1000.) ;
#14516=VECTOR('',#89368,1000.) ;
#14517=VECTOR('',#89383,1000.) ;
#14518=VECTOR('',#89384,1000.) ;
#14519=VECTOR('',#89385,1000.) ;
#14520=VECTOR('',#89386,1000.) ;
#14521=VECTOR('',#89389,1000.) ;
#14522=VECTOR('',#89390,1000.) ;
#14523=VECTOR('',#89391,1000.) ;
#14524=VECTOR('',#89394,1000.) ;
#14525=VECTOR('',#89395,1000.) ;
#14526=VECTOR('',#89396,1000.) ;
#14527=VECTOR('',#89399,1000.) ;
#14528=VECTOR('',#89400,1000.) ;
#14529=VECTOR('',#89401,1000.) ;
#14530=VECTOR('',#89402,1000.) ;
#14531=VECTOR('',#89405,1000.) ;
#14532=VECTOR('',#89406,1000.) ;
#14533=VECTOR('',#89407,1000.) ;
#14534=VECTOR('',#89408,1000.) ;
#14535=VECTOR('',#89411,1000.) ;
#14536=VECTOR('',#89412,1000.) ;
#14537=VECTOR('',#89413,1000.) ;
#14538=VECTOR('',#89416,1000.) ;
#14539=VECTOR('',#89417,1000.) ;
#14540=VECTOR('',#89418,1000.) ;
#14541=VECTOR('',#89421,1000.) ;
#14542=VECTOR('',#89422,1000.) ;
#14543=VECTOR('',#89423,1000.) ;
#14544=VECTOR('',#89424,1000.) ;
#14545=VECTOR('',#89427,1000.) ;
#14546=VECTOR('',#89428,1000.) ;
#14547=VECTOR('',#89429,1000.) ;
#14548=VECTOR('',#89430,1000.) ;
#14549=VECTOR('',#89433,1000.) ;
#14550=VECTOR('',#89434,1000.) ;
#14551=VECTOR('',#89435,1000.) ;
#14552=VECTOR('',#89436,1000.) ;
#14553=VECTOR('',#89439,1000.) ;
#14554=VECTOR('',#89440,1000.) ;
#14555=VECTOR('',#89441,1000.) ;
#14556=VECTOR('',#89442,1000.) ;
#14557=VECTOR('',#89669,1000.) ;
#14558=VECTOR('',#89670,1000.) ;
#14559=VECTOR('',#89671,1000.) ;
#14560=VECTOR('',#89672,1000.) ;
#14561=VECTOR('',#89673,1000.) ;
#14562=VECTOR('',#89674,1000.) ;
#14563=VECTOR('',#89677,1000.) ;
#14564=VECTOR('',#89680,1000.) ;
#14565=VECTOR('',#89683,1000.) ;
#14566=VECTOR('',#89684,1000.) ;
#14567=VECTOR('',#89685,1000.) ;
#14568=VECTOR('',#89686,1000.) ;
#14569=VECTOR('',#89687,1000.) ;
#14570=VECTOR('',#89688,1000.) ;
#14571=VECTOR('',#89691,1000.) ;
#14572=VECTOR('',#89694,1000.) ;
#14573=VECTOR('',#89697,1000.) ;
#14574=VECTOR('',#89698,1000.) ;
#14575=VECTOR('',#89699,1000.) ;
#14576=VECTOR('',#89700,1000.) ;
#14577=VECTOR('',#89701,1000.) ;
#14578=VECTOR('',#89702,1000.) ;
#14579=VECTOR('',#89705,1000.) ;
#14580=VECTOR('',#89708,1000.) ;
#14581=VECTOR('',#89711,1000.) ;
#14582=VECTOR('',#89712,1000.) ;
#14583=VECTOR('',#89713,1000.) ;
#14584=VECTOR('',#89714,1000.) ;
#14585=VECTOR('',#89715,1000.) ;
#14586=VECTOR('',#89716,1000.) ;
#14587=VECTOR('',#89719,1000.) ;
#14588=VECTOR('',#89722,1000.) ;
#14589=VECTOR('',#89725,1000.) ;
#14590=VECTOR('',#89726,1000.) ;
#14591=VECTOR('',#89727,1000.) ;
#14592=VECTOR('',#89728,1000.) ;
#14593=VECTOR('',#89729,1000.) ;
#14594=VECTOR('',#89730,1000.) ;
#14595=VECTOR('',#89733,1000.) ;
#14596=VECTOR('',#89736,1000.) ;
#14597=VECTOR('',#89739,1000.) ;
#14598=VECTOR('',#89740,1000.) ;
#14599=VECTOR('',#89741,1000.) ;
#14600=VECTOR('',#89742,1000.) ;
#14601=VECTOR('',#89743,1000.) ;
#14602=VECTOR('',#89744,1000.) ;
#14603=VECTOR('',#89747,1000.) ;
#14604=VECTOR('',#89750,1000.) ;
#14605=VECTOR('',#89753,1000.) ;
#14606=VECTOR('',#89754,1000.) ;
#14607=VECTOR('',#89755,1000.) ;
#14608=VECTOR('',#89756,1000.) ;
#14609=VECTOR('',#89757,1000.) ;
#14610=VECTOR('',#89758,1000.) ;
#14611=VECTOR('',#89761,1000.) ;
#14612=VECTOR('',#89764,1000.) ;
#14613=VECTOR('',#89767,1000.) ;
#14614=VECTOR('',#89768,1000.) ;
#14615=VECTOR('',#89769,1000.) ;
#14616=VECTOR('',#89770,1000.) ;
#14617=VECTOR('',#89771,1000.) ;
#14618=VECTOR('',#89772,1000.) ;
#14619=VECTOR('',#89775,1000.) ;
#14620=VECTOR('',#89778,1000.) ;
#14621=VECTOR('',#89781,1000.) ;
#14622=VECTOR('',#89782,1000.) ;
#14623=VECTOR('',#89783,1000.) ;
#14624=VECTOR('',#89784,1000.) ;
#14625=VECTOR('',#89785,1000.) ;
#14626=VECTOR('',#89786,1000.) ;
#14627=VECTOR('',#89789,1000.) ;
#14628=VECTOR('',#89792,1000.) ;
#14629=VECTOR('',#89795,1000.) ;
#14630=VECTOR('',#89796,1000.) ;
#14631=VECTOR('',#89797,1000.) ;
#14632=VECTOR('',#89798,1000.) ;
#14633=VECTOR('',#89801,1000.) ;
#14634=VECTOR('',#89802,1000.) ;
#14635=VECTOR('',#89803,1000.) ;
#14636=VECTOR('',#89806,1000.) ;
#14637=VECTOR('',#89807,1000.) ;
#14638=VECTOR('',#89808,1000.) ;
#14639=VECTOR('',#89809,1000.) ;
#14640=VECTOR('',#89812,1000.) ;
#14641=VECTOR('',#89813,1000.) ;
#14642=VECTOR('',#89814,1000.) ;
#14643=VECTOR('',#89815,1000.) ;
#14644=VECTOR('',#89818,1000.) ;
#14645=VECTOR('',#89819,1000.) ;
#14646=VECTOR('',#89820,1000.) ;
#14647=VECTOR('',#89821,1000.) ;
#14648=VECTOR('',#89824,1000.) ;
#14649=VECTOR('',#89825,1000.) ;
#14650=VECTOR('',#89826,1000.) ;
#14651=VECTOR('',#89827,1000.) ;
#14652=VECTOR('',#89830,1000.) ;
#14653=VECTOR('',#89831,1000.) ;
#14654=VECTOR('',#89832,1000.) ;
#14655=VECTOR('',#89835,1000.) ;
#14656=VECTOR('',#89836,1000.) ;
#14657=VECTOR('',#89837,1000.) ;
#14658=VECTOR('',#89838,1000.) ;
#14659=VECTOR('',#89841,1000.) ;
#14660=VECTOR('',#89842,1000.) ;
#14661=VECTOR('',#89843,1000.) ;
#14662=VECTOR('',#89844,1000.) ;
#14663=VECTOR('',#89847,1000.) ;
#14664=VECTOR('',#89848,1000.) ;
#14665=VECTOR('',#89849,1000.) ;
#14666=VECTOR('',#89850,1000.) ;
#14667=VECTOR('',#89853,1000.) ;
#14668=VECTOR('',#89854,1000.) ;
#14669=VECTOR('',#89855,1000.) ;
#14670=VECTOR('',#89856,1000.) ;
#14671=VECTOR('',#89859,1000.) ;
#14672=VECTOR('',#89860,1000.) ;
#14673=VECTOR('',#89861,1000.) ;
#14674=VECTOR('',#89864,1000.) ;
#14675=VECTOR('',#89865,1000.) ;
#14676=VECTOR('',#89866,1000.) ;
#14677=VECTOR('',#89867,1000.) ;
#14678=VECTOR('',#89870,1000.) ;
#14679=VECTOR('',#89871,1000.) ;
#14680=VECTOR('',#89872,1000.) ;
#14681=VECTOR('',#89873,1000.) ;
#14682=VECTOR('',#89876,1000.) ;
#14683=VECTOR('',#89877,1000.) ;
#14684=VECTOR('',#89878,1000.) ;
#14685=VECTOR('',#89879,1000.) ;
#14686=VECTOR('',#89882,1000.) ;
#14687=VECTOR('',#89883,1000.) ;
#14688=VECTOR('',#89884,1000.) ;
#14689=VECTOR('',#89885,1000.) ;
#14690=VECTOR('',#89888,1000.) ;
#14691=VECTOR('',#89889,1000.) ;
#14692=VECTOR('',#89890,1000.) ;
#14693=VECTOR('',#89893,1000.) ;
#14694=VECTOR('',#89894,1000.) ;
#14695=VECTOR('',#89895,1000.) ;
#14696=VECTOR('',#89896,1000.) ;
#14697=VECTOR('',#89899,1000.) ;
#14698=VECTOR('',#89900,1000.) ;
#14699=VECTOR('',#89901,1000.) ;
#14700=VECTOR('',#89902,1000.) ;
#14701=VECTOR('',#89905,1000.) ;
#14702=VECTOR('',#89906,1000.) ;
#14703=VECTOR('',#89907,1000.) ;
#14704=VECTOR('',#89908,1000.) ;
#14705=VECTOR('',#89911,1000.) ;
#14706=VECTOR('',#89912,1000.) ;
#14707=VECTOR('',#89913,1000.) ;
#14708=VECTOR('',#89914,1000.) ;
#14709=VECTOR('',#89917,1000.) ;
#14710=VECTOR('',#89918,1000.) ;
#14711=VECTOR('',#89919,1000.) ;
#14712=VECTOR('',#89922,1000.) ;
#14713=VECTOR('',#89923,1000.) ;
#14714=VECTOR('',#89924,1000.) ;
#14715=VECTOR('',#89925,1000.) ;
#14716=VECTOR('',#89928,1000.) ;
#14717=VECTOR('',#89929,1000.) ;
#14718=VECTOR('',#89930,1000.) ;
#14719=VECTOR('',#89931,1000.) ;
#14720=VECTOR('',#89934,1000.) ;
#14721=VECTOR('',#89935,1000.) ;
#14722=VECTOR('',#89936,1000.) ;
#14723=VECTOR('',#89937,1000.) ;
#14724=VECTOR('',#89940,1000.) ;
#14725=VECTOR('',#89941,1000.) ;
#14726=VECTOR('',#89942,1000.) ;
#14727=VECTOR('',#89943,1000.) ;
#14728=VECTOR('',#89946,1000.) ;
#14729=VECTOR('',#89947,1000.) ;
#14730=VECTOR('',#89948,1000.) ;
#14731=VECTOR('',#89951,1000.) ;
#14732=VECTOR('',#89952,1000.) ;
#14733=VECTOR('',#89953,1000.) ;
#14734=VECTOR('',#89954,1000.) ;
#14735=VECTOR('',#89957,1000.) ;
#14736=VECTOR('',#89958,1000.) ;
#14737=VECTOR('',#89959,1000.) ;
#14738=VECTOR('',#89960,1000.) ;
#14739=VECTOR('',#89963,1000.) ;
#14740=VECTOR('',#89964,1000.) ;
#14741=VECTOR('',#89965,1000.) ;
#14742=VECTOR('',#89966,1000.) ;
#14743=VECTOR('',#89969,1000.) ;
#14744=VECTOR('',#89970,1000.) ;
#14745=VECTOR('',#89971,1000.) ;
#14746=VECTOR('',#89972,1000.) ;
#14747=VECTOR('',#89975,1000.) ;
#14748=VECTOR('',#89976,1000.) ;
#14749=VECTOR('',#89977,1000.) ;
#14750=VECTOR('',#89980,1000.) ;
#14751=VECTOR('',#89981,1000.) ;
#14752=VECTOR('',#89982,1000.) ;
#14753=VECTOR('',#89983,1000.) ;
#14754=VECTOR('',#89986,1000.) ;
#14755=VECTOR('',#89987,1000.) ;
#14756=VECTOR('',#89988,1000.) ;
#14757=VECTOR('',#89989,1000.) ;
#14758=VECTOR('',#89992,1000.) ;
#14759=VECTOR('',#89993,1000.) ;
#14760=VECTOR('',#89994,1000.) ;
#14761=VECTOR('',#89995,1000.) ;
#14762=VECTOR('',#89998,1000.) ;
#14763=VECTOR('',#89999,1000.) ;
#14764=VECTOR('',#90000,1000.) ;
#14765=VECTOR('',#90001,1000.) ;
#14766=VECTOR('',#90004,1000.) ;
#14767=VECTOR('',#90005,1000.) ;
#14768=VECTOR('',#90006,1000.) ;
#14769=VECTOR('',#90009,1000.) ;
#14770=VECTOR('',#90010,1000.) ;
#14771=VECTOR('',#90011,1000.) ;
#14772=VECTOR('',#90012,1000.) ;
#14773=VECTOR('',#90015,1000.) ;
#14774=VECTOR('',#90016,1000.) ;
#14775=VECTOR('',#90017,1000.) ;
#14776=VECTOR('',#90018,1000.) ;
#14777=VECTOR('',#90021,1000.) ;
#14778=VECTOR('',#90022,1000.) ;
#14779=VECTOR('',#90023,1000.) ;
#14780=VECTOR('',#90024,1000.) ;
#14781=VECTOR('',#90027,1000.) ;
#14782=VECTOR('',#90028,1000.) ;
#14783=VECTOR('',#90029,1000.) ;
#14784=VECTOR('',#90030,1000.) ;
#14785=VECTOR('',#90033,1000.) ;
#14786=VECTOR('',#90034,1000.) ;
#14787=VECTOR('',#90035,1000.) ;
#14788=VECTOR('',#90038,1000.) ;
#14789=VECTOR('',#90039,1000.) ;
#14790=VECTOR('',#90040,1000.) ;
#14791=VECTOR('',#90041,1000.) ;
#14792=VECTOR('',#90044,1000.) ;
#14793=VECTOR('',#90045,1000.) ;
#14794=VECTOR('',#90046,1000.) ;
#14795=VECTOR('',#90047,1000.) ;
#14796=VECTOR('',#90050,1000.) ;
#14797=VECTOR('',#90051,1000.) ;
#14798=VECTOR('',#90052,1000.) ;
#14799=VECTOR('',#90053,1000.) ;
#14800=VECTOR('',#90056,1000.) ;
#14801=VECTOR('',#90059,1000.) ;
#14802=VECTOR('',#90064,1000.) ;
#14803=VECTOR('',#90065,1000.) ;
#14804=VECTOR('',#90066,1000.) ;
#14805=VECTOR('',#90071,1000.) ;
#14806=VECTOR('',#90076,1000.) ;
#14807=VECTOR('',#90077,1000.) ;
#14808=VECTOR('',#90078,1000.) ;
#14809=VECTOR('',#90083,1000.) ;
#14810=VECTOR('',#90088,1000.) ;
#14811=VECTOR('',#90089,1000.) ;
#14812=VECTOR('',#90090,1000.) ;
#14813=VECTOR('',#90093,1000.) ;
#14814=VECTOR('',#90098,1000.) ;
#14815=VECTOR('',#90099,1000.) ;
#14816=VECTOR('',#90102,1000.) ;
#14817=VECTOR('',#90103,1000.) ;
#14818=VECTOR('',#90104,1000.) ;
#14819=VECTOR('',#90109,1000.) ;
#14820=VECTOR('',#90114,1000.) ;
#14821=VECTOR('',#90115,1000.) ;
#14822=VECTOR('',#90116,1000.) ;
#14823=VECTOR('',#90121,1000.) ;
#14824=VECTOR('',#90126,1000.) ;
#14825=VECTOR('',#90127,1000.) ;
#14826=VECTOR('',#90128,1000.) ;
#14827=VECTOR('',#90133,1000.) ;
#14828=VECTOR('',#90138,1000.) ;
#14829=VECTOR('',#90139,1000.) ;
#14830=VECTOR('',#90140,1000.) ;
#14831=VECTOR('',#90145,1000.) ;
#14832=VECTOR('',#90150,1000.) ;
#14833=VECTOR('',#90151,1000.) ;
#14834=VECTOR('',#90152,1000.) ;
#14835=VECTOR('',#90157,1000.) ;
#14836=VECTOR('',#90162,1000.) ;
#14837=VECTOR('',#90163,1000.) ;
#14838=VECTOR('',#90164,1000.) ;
#14839=VECTOR('',#90169,1000.) ;
#14840=VECTOR('',#90176,1000.) ;
#14841=VECTOR('',#90183,1000.) ;
#14842=VECTOR('',#90188,1000.) ;
#14843=VECTOR('',#90189,1000.) ;
#14844=VECTOR('',#90190,1000.) ;
#14845=VECTOR('',#90195,1000.) ;
#14846=VECTOR('',#90200,1000.) ;
#14847=VECTOR('',#90201,1000.) ;
#14848=VECTOR('',#90202,1000.) ;
#14849=VECTOR('',#90207,1000.) ;
#14850=VECTOR('',#90212,1000.) ;
#14851=VECTOR('',#90213,1000.) ;
#14852=VECTOR('',#90218,1000.) ;
#14853=VECTOR('',#90221,1000.) ;
#14854=VECTOR('',#90222,1000.) ;
#14855=VECTOR('',#90223,1000.) ;
#14856=VECTOR('',#90226,1000.) ;
#14857=VECTOR('',#90227,1000.) ;
#14858=VECTOR('',#90228,1000.) ;
#14859=VECTOR('',#90231,1000.) ;
#14860=VECTOR('',#90234,1000.) ;
#14861=VECTOR('',#90235,1000.) ;
#14862=VECTOR('',#90236,1000.) ;
#14863=VECTOR('',#90237,1000.) ;
#14864=VECTOR('',#90238,1000.) ;
#14865=VECTOR('',#90241,1000.) ;
#14866=VECTOR('',#90244,1000.) ;
#14867=VECTOR('',#90249,1000.) ;
#14868=VECTOR('',#90250,1000.) ;
#14869=VECTOR('',#90251,1000.) ;
#14870=VECTOR('',#90256,1000.) ;
#14871=VECTOR('',#90261,1000.) ;
#14872=VECTOR('',#90262,1000.) ;
#14873=VECTOR('',#90263,1000.) ;
#14874=VECTOR('',#90268,1000.) ;
#14875=VECTOR('',#90273,1000.) ;
#14876=VECTOR('',#90274,1000.) ;
#14877=VECTOR('',#90275,1000.) ;
#14878=VECTOR('',#90278,1000.) ;
#14879=VECTOR('',#90283,1000.) ;
#14880=VECTOR('',#90284,1000.) ;
#14881=VECTOR('',#90287,1000.) ;
#14882=VECTOR('',#90288,1000.) ;
#14883=VECTOR('',#90289,1000.) ;
#14884=VECTOR('',#90294,1000.) ;
#14885=VECTOR('',#90299,1000.) ;
#14886=VECTOR('',#90300,1000.) ;
#14887=VECTOR('',#90301,1000.) ;
#14888=VECTOR('',#90306,1000.) ;
#14889=VECTOR('',#90311,1000.) ;
#14890=VECTOR('',#90312,1000.) ;
#14891=VECTOR('',#90313,1000.) ;
#14892=VECTOR('',#90318,1000.) ;
#14893=VECTOR('',#90323,1000.) ;
#14894=VECTOR('',#90324,1000.) ;
#14895=VECTOR('',#90325,1000.) ;
#14896=VECTOR('',#90330,1000.) ;
#14897=VECTOR('',#90335,1000.) ;
#14898=VECTOR('',#90336,1000.) ;
#14899=VECTOR('',#90337,1000.) ;
#14900=VECTOR('',#90342,1000.) ;
#14901=VECTOR('',#90347,1000.) ;
#14902=VECTOR('',#90348,1000.) ;
#14903=VECTOR('',#90349,1000.) ;
#14904=VECTOR('',#90354,1000.) ;
#14905=VECTOR('',#90361,1000.) ;
#14906=VECTOR('',#90368,1000.) ;
#14907=VECTOR('',#90373,1000.) ;
#14908=VECTOR('',#90374,1000.) ;
#14909=VECTOR('',#90375,1000.) ;
#14910=VECTOR('',#90380,1000.) ;
#14911=VECTOR('',#90385,1000.) ;
#14912=VECTOR('',#90386,1000.) ;
#14913=VECTOR('',#90387,1000.) ;
#14914=VECTOR('',#90392,1000.) ;
#14915=VECTOR('',#90397,1000.) ;
#14916=VECTOR('',#90398,1000.) ;
#14917=VECTOR('',#90403,1000.) ;
#14918=VECTOR('',#90406,1000.) ;
#14919=VECTOR('',#90407,1000.) ;
#14920=VECTOR('',#90408,1000.) ;
#14921=VECTOR('',#90411,1000.) ;
#14922=VECTOR('',#90412,1000.) ;
#14923=VECTOR('',#90413,1000.) ;
#14924=VECTOR('',#90416,1000.) ;
#14925=VECTOR('',#90419,1000.) ;
#14926=VECTOR('',#90420,1000.) ;
#14927=VECTOR('',#90421,1000.) ;
#14928=VECTOR('',#90422,1000.) ;
#14929=VECTOR('',#90423,1000.) ;
#14930=VECTOR('',#90426,1000.) ;
#14931=VECTOR('',#90429,1000.) ;
#14932=VECTOR('',#90434,1000.) ;
#14933=VECTOR('',#90435,1000.) ;
#14934=VECTOR('',#90436,1000.) ;
#14935=VECTOR('',#90441,1000.) ;
#14936=VECTOR('',#90446,1000.) ;
#14937=VECTOR('',#90447,1000.) ;
#14938=VECTOR('',#90448,1000.) ;
#14939=VECTOR('',#90453,1000.) ;
#14940=VECTOR('',#90458,1000.) ;
#14941=VECTOR('',#90459,1000.) ;
#14942=VECTOR('',#90460,1000.) ;
#14943=VECTOR('',#90463,1000.) ;
#14944=VECTOR('',#90468,1000.) ;
#14945=VECTOR('',#90469,1000.) ;
#14946=VECTOR('',#90472,1000.) ;
#14947=VECTOR('',#90473,1000.) ;
#14948=VECTOR('',#90474,1000.) ;
#14949=VECTOR('',#90479,1000.) ;
#14950=VECTOR('',#90484,1000.) ;
#14951=VECTOR('',#90485,1000.) ;
#14952=VECTOR('',#90486,1000.) ;
#14953=VECTOR('',#90491,1000.) ;
#14954=VECTOR('',#90496,1000.) ;
#14955=VECTOR('',#90497,1000.) ;
#14956=VECTOR('',#90498,1000.) ;
#14957=VECTOR('',#90503,1000.) ;
#14958=VECTOR('',#90508,1000.) ;
#14959=VECTOR('',#90509,1000.) ;
#14960=VECTOR('',#90510,1000.) ;
#14961=VECTOR('',#90515,1000.) ;
#14962=VECTOR('',#90520,1000.) ;
#14963=VECTOR('',#90521,1000.) ;
#14964=VECTOR('',#90522,1000.) ;
#14965=VECTOR('',#90527,1000.) ;
#14966=VECTOR('',#90532,1000.) ;
#14967=VECTOR('',#90533,1000.) ;
#14968=VECTOR('',#90534,1000.) ;
#14969=VECTOR('',#90539,1000.) ;
#14970=VECTOR('',#90546,1000.) ;
#14971=VECTOR('',#90553,1000.) ;
#14972=VECTOR('',#90558,1000.) ;
#14973=VECTOR('',#90559,1000.) ;
#14974=VECTOR('',#90560,1000.) ;
#14975=VECTOR('',#90565,1000.) ;
#14976=VECTOR('',#90570,1000.) ;
#14977=VECTOR('',#90571,1000.) ;
#14978=VECTOR('',#90572,1000.) ;
#14979=VECTOR('',#90577,1000.) ;
#14980=VECTOR('',#90582,1000.) ;
#14981=VECTOR('',#90583,1000.) ;
#14982=VECTOR('',#90588,1000.) ;
#14983=VECTOR('',#90591,1000.) ;
#14984=VECTOR('',#90592,1000.) ;
#14985=VECTOR('',#90593,1000.) ;
#14986=VECTOR('',#90596,1000.) ;
#14987=VECTOR('',#90597,1000.) ;
#14988=VECTOR('',#90598,1000.) ;
#14989=VECTOR('',#90601,1000.) ;
#14990=VECTOR('',#90604,1000.) ;
#14991=VECTOR('',#90605,1000.) ;
#14992=VECTOR('',#90606,1000.) ;
#14993=VECTOR('',#90607,1000.) ;
#14994=VECTOR('',#90608,1000.) ;
#14995=VECTOR('',#90611,1000.) ;
#14996=VECTOR('',#90614,1000.) ;
#14997=VECTOR('',#90619,1000.) ;
#14998=VECTOR('',#90620,1000.) ;
#14999=VECTOR('',#90621,1000.) ;
#15000=VECTOR('',#90626,1000.) ;
#15001=VECTOR('',#90631,1000.) ;
#15002=VECTOR('',#90632,1000.) ;
#15003=VECTOR('',#90633,1000.) ;
#15004=VECTOR('',#90638,1000.) ;
#15005=VECTOR('',#90643,1000.) ;
#15006=VECTOR('',#90644,1000.) ;
#15007=VECTOR('',#90645,1000.) ;
#15008=VECTOR('',#90648,1000.) ;
#15009=VECTOR('',#90653,1000.) ;
#15010=VECTOR('',#90654,1000.) ;
#15011=VECTOR('',#90657,1000.) ;
#15012=VECTOR('',#90658,1000.) ;
#15013=VECTOR('',#90659,1000.) ;
#15014=VECTOR('',#90664,1000.) ;
#15015=VECTOR('',#90669,1000.) ;
#15016=VECTOR('',#90670,1000.) ;
#15017=VECTOR('',#90671,1000.) ;
#15018=VECTOR('',#90676,1000.) ;
#15019=VECTOR('',#90681,1000.) ;
#15020=VECTOR('',#90682,1000.) ;
#15021=VECTOR('',#90683,1000.) ;
#15022=VECTOR('',#90688,1000.) ;
#15023=VECTOR('',#90693,1000.) ;
#15024=VECTOR('',#90694,1000.) ;
#15025=VECTOR('',#90695,1000.) ;
#15026=VECTOR('',#90700,1000.) ;
#15027=VECTOR('',#90705,1000.) ;
#15028=VECTOR('',#90706,1000.) ;
#15029=VECTOR('',#90707,1000.) ;
#15030=VECTOR('',#90712,1000.) ;
#15031=VECTOR('',#90717,1000.) ;
#15032=VECTOR('',#90718,1000.) ;
#15033=VECTOR('',#90719,1000.) ;
#15034=VECTOR('',#90724,1000.) ;
#15035=VECTOR('',#90731,1000.) ;
#15036=VECTOR('',#90738,1000.) ;
#15037=VECTOR('',#90743,1000.) ;
#15038=VECTOR('',#90744,1000.) ;
#15039=VECTOR('',#90745,1000.) ;
#15040=VECTOR('',#90750,1000.) ;
#15041=VECTOR('',#90755,1000.) ;
#15042=VECTOR('',#90756,1000.) ;
#15043=VECTOR('',#90757,1000.) ;
#15044=VECTOR('',#90762,1000.) ;
#15045=VECTOR('',#90767,1000.) ;
#15046=VECTOR('',#90768,1000.) ;
#15047=VECTOR('',#90773,1000.) ;
#15048=VECTOR('',#90776,1000.) ;
#15049=VECTOR('',#90777,1000.) ;
#15050=VECTOR('',#90778,1000.) ;
#15051=VECTOR('',#90781,1000.) ;
#15052=VECTOR('',#90782,1000.) ;
#15053=VECTOR('',#90783,1000.) ;
#15054=VECTOR('',#90786,1000.) ;
#15055=VECTOR('',#90789,1000.) ;
#15056=VECTOR('',#90790,1000.) ;
#15057=VECTOR('',#90791,1000.) ;
#15058=VECTOR('',#90792,1000.) ;
#15059=VECTOR('',#90793,1000.) ;
#15060=VECTOR('',#90796,1000.) ;
#15061=VECTOR('',#90799,1000.) ;
#15062=VECTOR('',#90804,1000.) ;
#15063=VECTOR('',#90805,1000.) ;
#15064=VECTOR('',#90806,1000.) ;
#15065=VECTOR('',#90811,1000.) ;
#15066=VECTOR('',#90816,1000.) ;
#15067=VECTOR('',#90817,1000.) ;
#15068=VECTOR('',#90818,1000.) ;
#15069=VECTOR('',#90823,1000.) ;
#15070=VECTOR('',#90828,1000.) ;
#15071=VECTOR('',#90829,1000.) ;
#15072=VECTOR('',#90830,1000.) ;
#15073=VECTOR('',#90833,1000.) ;
#15074=VECTOR('',#90838,1000.) ;
#15075=VECTOR('',#90839,1000.) ;
#15076=VECTOR('',#90842,1000.) ;
#15077=VECTOR('',#90843,1000.) ;
#15078=VECTOR('',#90844,1000.) ;
#15079=VECTOR('',#90849,1000.) ;
#15080=VECTOR('',#90854,1000.) ;
#15081=VECTOR('',#90855,1000.) ;
#15082=VECTOR('',#90856,1000.) ;
#15083=VECTOR('',#90861,1000.) ;
#15084=VECTOR('',#90866,1000.) ;
#15085=VECTOR('',#90867,1000.) ;
#15086=VECTOR('',#90868,1000.) ;
#15087=VECTOR('',#90873,1000.) ;
#15088=VECTOR('',#90878,1000.) ;
#15089=VECTOR('',#90879,1000.) ;
#15090=VECTOR('',#90880,1000.) ;
#15091=VECTOR('',#90885,1000.) ;
#15092=VECTOR('',#90890,1000.) ;
#15093=VECTOR('',#90891,1000.) ;
#15094=VECTOR('',#90892,1000.) ;
#15095=VECTOR('',#90897,1000.) ;
#15096=VECTOR('',#90902,1000.) ;
#15097=VECTOR('',#90903,1000.) ;
#15098=VECTOR('',#90904,1000.) ;
#15099=VECTOR('',#90909,1000.) ;
#15100=VECTOR('',#90916,1000.) ;
#15101=VECTOR('',#90923,1000.) ;
#15102=VECTOR('',#90928,1000.) ;
#15103=VECTOR('',#90929,1000.) ;
#15104=VECTOR('',#90930,1000.) ;
#15105=VECTOR('',#90935,1000.) ;
#15106=VECTOR('',#90940,1000.) ;
#15107=VECTOR('',#90941,1000.) ;
#15108=VECTOR('',#90942,1000.) ;
#15109=VECTOR('',#90947,1000.) ;
#15110=VECTOR('',#90952,1000.) ;
#15111=VECTOR('',#90953,1000.) ;
#15112=VECTOR('',#90958,1000.) ;
#15113=VECTOR('',#90961,1000.) ;
#15114=VECTOR('',#90962,1000.) ;
#15115=VECTOR('',#90963,1000.) ;
#15116=VECTOR('',#90966,1000.) ;
#15117=VECTOR('',#90967,1000.) ;
#15118=VECTOR('',#90968,1000.) ;
#15119=VECTOR('',#90971,1000.) ;
#15120=VECTOR('',#90974,1000.) ;
#15121=VECTOR('',#90975,1000.) ;
#15122=VECTOR('',#90976,1000.) ;
#15123=VECTOR('',#90977,1000.) ;
#15124=VECTOR('',#90978,1000.) ;
#15125=VECTOR('',#90981,1000.) ;
#15126=VECTOR('',#90984,1000.) ;
#15127=VECTOR('',#90989,1000.) ;
#15128=VECTOR('',#90990,1000.) ;
#15129=VECTOR('',#90991,1000.) ;
#15130=VECTOR('',#90996,1000.) ;
#15131=VECTOR('',#91001,1000.) ;
#15132=VECTOR('',#91002,1000.) ;
#15133=VECTOR('',#91003,1000.) ;
#15134=VECTOR('',#91008,1000.) ;
#15135=VECTOR('',#91013,1000.) ;
#15136=VECTOR('',#91014,1000.) ;
#15137=VECTOR('',#91015,1000.) ;
#15138=VECTOR('',#91018,1000.) ;
#15139=VECTOR('',#91023,1000.) ;
#15140=VECTOR('',#91024,1000.) ;
#15141=VECTOR('',#91027,1000.) ;
#15142=VECTOR('',#91028,1000.) ;
#15143=VECTOR('',#91029,1000.) ;
#15144=VECTOR('',#91034,1000.) ;
#15145=VECTOR('',#91039,1000.) ;
#15146=VECTOR('',#91040,1000.) ;
#15147=VECTOR('',#91041,1000.) ;
#15148=VECTOR('',#91046,1000.) ;
#15149=VECTOR('',#91051,1000.) ;
#15150=VECTOR('',#91052,1000.) ;
#15151=VECTOR('',#91053,1000.) ;
#15152=VECTOR('',#91058,1000.) ;
#15153=VECTOR('',#91063,1000.) ;
#15154=VECTOR('',#91064,1000.) ;
#15155=VECTOR('',#91065,1000.) ;
#15156=VECTOR('',#91070,1000.) ;
#15157=VECTOR('',#91075,1000.) ;
#15158=VECTOR('',#91076,1000.) ;
#15159=VECTOR('',#91077,1000.) ;
#15160=VECTOR('',#91082,1000.) ;
#15161=VECTOR('',#91087,1000.) ;
#15162=VECTOR('',#91088,1000.) ;
#15163=VECTOR('',#91089,1000.) ;
#15164=VECTOR('',#91094,1000.) ;
#15165=VECTOR('',#91101,1000.) ;
#15166=VECTOR('',#91108,1000.) ;
#15167=VECTOR('',#91113,1000.) ;
#15168=VECTOR('',#91114,1000.) ;
#15169=VECTOR('',#91115,1000.) ;
#15170=VECTOR('',#91120,1000.) ;
#15171=VECTOR('',#91125,1000.) ;
#15172=VECTOR('',#91126,1000.) ;
#15173=VECTOR('',#91127,1000.) ;
#15174=VECTOR('',#91132,1000.) ;
#15175=VECTOR('',#91137,1000.) ;
#15176=VECTOR('',#91138,1000.) ;
#15177=VECTOR('',#91143,1000.) ;
#15178=VECTOR('',#91146,1000.) ;
#15179=VECTOR('',#91147,1000.) ;
#15180=VECTOR('',#91148,1000.) ;
#15181=VECTOR('',#91151,1000.) ;
#15182=VECTOR('',#91152,1000.) ;
#15183=VECTOR('',#91153,1000.) ;
#15184=VECTOR('',#91156,1000.) ;
#15185=VECTOR('',#91159,1000.) ;
#15186=VECTOR('',#91160,1000.) ;
#15187=VECTOR('',#91161,1000.) ;
#15188=VECTOR('',#91162,1000.) ;
#15189=VECTOR('',#91163,1000.) ;
#15190=VECTOR('',#91166,1000.) ;
#15191=VECTOR('',#91169,1000.) ;
#15192=VECTOR('',#91174,1000.) ;
#15193=VECTOR('',#91175,1000.) ;
#15194=VECTOR('',#91176,1000.) ;
#15195=VECTOR('',#91181,1000.) ;
#15196=VECTOR('',#91186,1000.) ;
#15197=VECTOR('',#91187,1000.) ;
#15198=VECTOR('',#91188,1000.) ;
#15199=VECTOR('',#91193,1000.) ;
#15200=VECTOR('',#91198,1000.) ;
#15201=VECTOR('',#91199,1000.) ;
#15202=VECTOR('',#91200,1000.) ;
#15203=VECTOR('',#91203,1000.) ;
#15204=VECTOR('',#91208,1000.) ;
#15205=VECTOR('',#91209,1000.) ;
#15206=VECTOR('',#91212,1000.) ;
#15207=VECTOR('',#91213,1000.) ;
#15208=VECTOR('',#91214,1000.) ;
#15209=VECTOR('',#91219,1000.) ;
#15210=VECTOR('',#91224,1000.) ;
#15211=VECTOR('',#91225,1000.) ;
#15212=VECTOR('',#91226,1000.) ;
#15213=VECTOR('',#91231,1000.) ;
#15214=VECTOR('',#91236,1000.) ;
#15215=VECTOR('',#91237,1000.) ;
#15216=VECTOR('',#91238,1000.) ;
#15217=VECTOR('',#91243,1000.) ;
#15218=VECTOR('',#91248,1000.) ;
#15219=VECTOR('',#91249,1000.) ;
#15220=VECTOR('',#91250,1000.) ;
#15221=VECTOR('',#91255,1000.) ;
#15222=VECTOR('',#91260,1000.) ;
#15223=VECTOR('',#91261,1000.) ;
#15224=VECTOR('',#91262,1000.) ;
#15225=VECTOR('',#91267,1000.) ;
#15226=VECTOR('',#91272,1000.) ;
#15227=VECTOR('',#91273,1000.) ;
#15228=VECTOR('',#91274,1000.) ;
#15229=VECTOR('',#91279,1000.) ;
#15230=VECTOR('',#91286,1000.) ;
#15231=VECTOR('',#91293,1000.) ;
#15232=VECTOR('',#91298,1000.) ;
#15233=VECTOR('',#91299,1000.) ;
#15234=VECTOR('',#91300,1000.) ;
#15235=VECTOR('',#91305,1000.) ;
#15236=VECTOR('',#91310,1000.) ;
#15237=VECTOR('',#91311,1000.) ;
#15238=VECTOR('',#91312,1000.) ;
#15239=VECTOR('',#91317,1000.) ;
#15240=VECTOR('',#91322,1000.) ;
#15241=VECTOR('',#91323,1000.) ;
#15242=VECTOR('',#91328,1000.) ;
#15243=VECTOR('',#91331,1000.) ;
#15244=VECTOR('',#91332,1000.) ;
#15245=VECTOR('',#91333,1000.) ;
#15246=VECTOR('',#91336,1000.) ;
#15247=VECTOR('',#91337,1000.) ;
#15248=VECTOR('',#91338,1000.) ;
#15249=VECTOR('',#91341,1000.) ;
#15250=VECTOR('',#91344,1000.) ;
#15251=VECTOR('',#91345,1000.) ;
#15252=VECTOR('',#91346,1000.) ;
#15253=VECTOR('',#91347,1000.) ;
#15254=VECTOR('',#91348,1000.) ;
#15255=VECTOR('',#91351,1000.) ;
#15256=VECTOR('',#91354,1000.) ;
#15257=VECTOR('',#91359,1000.) ;
#15258=VECTOR('',#91360,1000.) ;
#15259=VECTOR('',#91361,1000.) ;
#15260=VECTOR('',#91366,1000.) ;
#15261=VECTOR('',#91371,1000.) ;
#15262=VECTOR('',#91372,1000.) ;
#15263=VECTOR('',#91373,1000.) ;
#15264=VECTOR('',#91378,1000.) ;
#15265=VECTOR('',#91383,1000.) ;
#15266=VECTOR('',#91384,1000.) ;
#15267=VECTOR('',#91385,1000.) ;
#15268=VECTOR('',#91388,1000.) ;
#15269=VECTOR('',#91393,1000.) ;
#15270=VECTOR('',#91394,1000.) ;
#15271=VECTOR('',#91397,1000.) ;
#15272=VECTOR('',#91398,1000.) ;
#15273=VECTOR('',#91399,1000.) ;
#15274=VECTOR('',#91404,1000.) ;
#15275=VECTOR('',#91409,1000.) ;
#15276=VECTOR('',#91410,1000.) ;
#15277=VECTOR('',#91411,1000.) ;
#15278=VECTOR('',#91416,1000.) ;
#15279=VECTOR('',#91421,1000.) ;
#15280=VECTOR('',#91422,1000.) ;
#15281=VECTOR('',#91423,1000.) ;
#15282=VECTOR('',#91428,1000.) ;
#15283=VECTOR('',#91433,1000.) ;
#15284=VECTOR('',#91434,1000.) ;
#15285=VECTOR('',#91435,1000.) ;
#15286=VECTOR('',#91440,1000.) ;
#15287=VECTOR('',#91445,1000.) ;
#15288=VECTOR('',#91446,1000.) ;
#15289=VECTOR('',#91447,1000.) ;
#15290=VECTOR('',#91452,1000.) ;
#15291=VECTOR('',#91457,1000.) ;
#15292=VECTOR('',#91458,1000.) ;
#15293=VECTOR('',#91459,1000.) ;
#15294=VECTOR('',#91464,1000.) ;
#15295=VECTOR('',#91471,1000.) ;
#15296=VECTOR('',#91478,1000.) ;
#15297=VECTOR('',#91483,1000.) ;
#15298=VECTOR('',#91484,1000.) ;
#15299=VECTOR('',#91485,1000.) ;
#15300=VECTOR('',#91490,1000.) ;
#15301=VECTOR('',#91495,1000.) ;
#15302=VECTOR('',#91496,1000.) ;
#15303=VECTOR('',#91497,1000.) ;
#15304=VECTOR('',#91502,1000.) ;
#15305=VECTOR('',#91507,1000.) ;
#15306=VECTOR('',#91508,1000.) ;
#15307=VECTOR('',#91513,1000.) ;
#15308=VECTOR('',#91516,1000.) ;
#15309=VECTOR('',#91517,1000.) ;
#15310=VECTOR('',#91518,1000.) ;
#15311=VECTOR('',#91521,1000.) ;
#15312=VECTOR('',#91522,1000.) ;
#15313=VECTOR('',#91523,1000.) ;
#15314=VECTOR('',#91526,1000.) ;
#15315=VECTOR('',#91529,1000.) ;
#15316=VECTOR('',#91530,1000.) ;
#15317=VECTOR('',#91531,1000.) ;
#15318=VECTOR('',#91532,1000.) ;
#15319=VECTOR('',#91533,1000.) ;
#15320=VECTOR('',#91536,1000.) ;
#15321=VECTOR('',#91539,1000.) ;
#15322=VECTOR('',#91544,1000.) ;
#15323=VECTOR('',#91545,1000.) ;
#15324=VECTOR('',#91546,1000.) ;
#15325=VECTOR('',#91551,1000.) ;
#15326=VECTOR('',#91556,1000.) ;
#15327=VECTOR('',#91557,1000.) ;
#15328=VECTOR('',#91558,1000.) ;
#15329=VECTOR('',#91563,1000.) ;
#15330=VECTOR('',#91568,1000.) ;
#15331=VECTOR('',#91569,1000.) ;
#15332=VECTOR('',#91570,1000.) ;
#15333=VECTOR('',#91573,1000.) ;
#15334=VECTOR('',#91578,1000.) ;
#15335=VECTOR('',#91579,1000.) ;
#15336=VECTOR('',#91582,1000.) ;
#15337=VECTOR('',#91583,1000.) ;
#15338=VECTOR('',#91584,1000.) ;
#15339=VECTOR('',#91589,1000.) ;
#15340=VECTOR('',#91594,1000.) ;
#15341=VECTOR('',#91595,1000.) ;
#15342=VECTOR('',#91596,1000.) ;
#15343=VECTOR('',#91601,1000.) ;
#15344=VECTOR('',#91606,1000.) ;
#15345=VECTOR('',#91607,1000.) ;
#15346=VECTOR('',#91608,1000.) ;
#15347=VECTOR('',#91613,1000.) ;
#15348=VECTOR('',#91618,1000.) ;
#15349=VECTOR('',#91619,1000.) ;
#15350=VECTOR('',#91620,1000.) ;
#15351=VECTOR('',#91625,1000.) ;
#15352=VECTOR('',#91630,1000.) ;
#15353=VECTOR('',#91631,1000.) ;
#15354=VECTOR('',#91632,1000.) ;
#15355=VECTOR('',#91637,1000.) ;
#15356=VECTOR('',#91642,1000.) ;
#15357=VECTOR('',#91643,1000.) ;
#15358=VECTOR('',#91644,1000.) ;
#15359=VECTOR('',#91649,1000.) ;
#15360=VECTOR('',#91656,1000.) ;
#15361=VECTOR('',#91663,1000.) ;
#15362=VECTOR('',#91668,1000.) ;
#15363=VECTOR('',#91669,1000.) ;
#15364=VECTOR('',#91670,1000.) ;
#15365=VECTOR('',#91675,1000.) ;
#15366=VECTOR('',#91680,1000.) ;
#15367=VECTOR('',#91681,1000.) ;
#15368=VECTOR('',#91682,1000.) ;
#15369=VECTOR('',#91687,1000.) ;
#15370=VECTOR('',#91692,1000.) ;
#15371=VECTOR('',#91693,1000.) ;
#15372=VECTOR('',#91698,1000.) ;
#15373=VECTOR('',#91701,1000.) ;
#15374=VECTOR('',#91702,1000.) ;
#15375=VECTOR('',#91703,1000.) ;
#15376=VECTOR('',#91706,1000.) ;
#15377=VECTOR('',#91707,1000.) ;
#15378=VECTOR('',#91708,1000.) ;
#15379=VECTOR('',#91711,1000.) ;
#15380=VECTOR('',#91714,1000.) ;
#15381=VECTOR('',#91715,1000.) ;
#15382=VECTOR('',#91716,1000.) ;
#15383=VECTOR('',#91717,1000.) ;
#15384=VECTOR('',#91718,1000.) ;
#15385=VECTOR('',#91721,1000.) ;
#15386=VECTOR('',#91724,1000.) ;
#15387=VECTOR('',#91727,1000.) ;
#15388=VECTOR('',#91730,1000.) ;
#15389=VECTOR('',#91735,1000.) ;
#15390=VECTOR('',#91738,1000.) ;
#15391=VECTOR('',#91741,1000.) ;
#15392=VECTOR('',#91744,1000.) ;
#15393=VECTOR('',#91749,1000.) ;
#15394=VECTOR('',#91752,1000.) ;
#15395=VECTOR('',#91755,1000.) ;
#15396=VECTOR('',#91758,1000.) ;
#15397=VECTOR('',#91763,1000.) ;
#15398=VECTOR('',#91766,1000.) ;
#15399=VECTOR('',#91769,1000.) ;
#15400=VECTOR('',#91772,1000.) ;
#15401=VECTOR('',#91777,1000.) ;
#15402=VECTOR('',#91780,1000.) ;
#15403=VECTOR('',#91783,1000.) ;
#15404=VECTOR('',#91786,1000.) ;
#15405=VECTOR('',#91791,1000.) ;
#15406=VECTOR('',#91794,1000.) ;
#15407=VECTOR('',#91797,1000.) ;
#15408=VECTOR('',#91800,1000.) ;
#15409=VECTOR('',#91805,1000.) ;
#15410=VECTOR('',#91808,1000.) ;
#15411=VECTOR('',#91811,1000.) ;
#15412=VECTOR('',#91814,1000.) ;
#15413=VECTOR('',#91819,1000.) ;
#15414=VECTOR('',#91822,1000.) ;
#15415=VECTOR('',#91825,1000.) ;
#15416=VECTOR('',#91828,1000.) ;
#15417=VECTOR('',#91833,1000.) ;
#15418=VECTOR('',#91836,1000.) ;
#15419=VECTOR('',#91839,1000.) ;
#15420=VECTOR('',#91842,1000.) ;
#15421=VECTOR('',#91877,1000.) ;
#15422=VECTOR('',#91880,1000.) ;
#15423=VECTOR('',#91927,1000.) ;
#15424=VECTOR('',#91986,1000.) ;
#15425=VECTOR('',#92035,1000.) ;
#15426=VECTOR('',#93142,1000.) ;
#15427=VECTOR('',#93145,1000.) ;
#15428=VECTOR('',#93192,1000.) ;
#15429=VECTOR('',#93251,1000.) ;
#15430=VECTOR('',#93300,1000.) ;
#15431=VECTOR('',#93453,1000.) ;
#15432=VECTOR('',#93456,1000.) ;
#15433=VECTOR('',#93503,1000.) ;
#15434=VECTOR('',#93562,1000.) ;
#15435=VECTOR('',#93611,1000.) ;
#15436=VECTOR('',#93764,1000.) ;
#15437=VECTOR('',#93767,1000.) ;
#15438=VECTOR('',#93814,1000.) ;
#15439=VECTOR('',#93873,1000.) ;
#15440=VECTOR('',#93922,1000.) ;
#15441=VECTOR('',#94075,1000.) ;
#15442=VECTOR('',#94078,1000.) ;
#15443=VECTOR('',#94125,1000.) ;
#15444=VECTOR('',#94184,1000.) ;
#15445=VECTOR('',#94233,1000.) ;
#15446=VECTOR('',#94386,1000.) ;
#15447=VECTOR('',#94389,1000.) ;
#15448=VECTOR('',#94436,1000.) ;
#15449=VECTOR('',#94495,1000.) ;
#15450=VECTOR('',#94544,1000.) ;
#15451=VECTOR('',#94697,1000.) ;
#15452=VECTOR('',#94700,1000.) ;
#15453=VECTOR('',#94747,1000.) ;
#15454=VECTOR('',#94806,1000.) ;
#15455=VECTOR('',#94855,1000.) ;
#15456=VECTOR('',#95008,1000.) ;
#15457=VECTOR('',#95011,1000.) ;
#15458=VECTOR('',#95058,1000.) ;
#15459=VECTOR('',#95117,1000.) ;
#15460=VECTOR('',#95166,1000.) ;
#15461=VECTOR('',#95319,1000.) ;
#15462=VECTOR('',#95322,1000.) ;
#15463=VECTOR('',#95369,1000.) ;
#15464=VECTOR('',#95428,1000.) ;
#15465=VECTOR('',#95477,1000.) ;
#15466=VECTOR('',#95600,1000.) ;
#15467=VECTOR('',#95601,1000.) ;
#15468=VECTOR('',#95602,1000.) ;
#15469=VECTOR('',#95603,1000.) ;
#15470=VECTOR('',#95606,1000.) ;
#15471=VECTOR('',#95607,1000.) ;
#15472=VECTOR('',#95608,1000.) ;
#15473=VECTOR('',#95609,1000.) ;
#15474=VECTOR('',#95612,1000.) ;
#15475=VECTOR('',#95613,1000.) ;
#15476=VECTOR('',#95614,1000.) ;
#15477=VECTOR('',#95615,1000.) ;
#15478=VECTOR('',#95618,1000.) ;
#15479=VECTOR('',#95619,1000.) ;
#15480=VECTOR('',#95620,1000.) ;
#15481=VECTOR('',#95621,1000.) ;
#15482=VECTOR('',#95624,1000.) ;
#15483=VECTOR('',#95625,1000.) ;
#15484=VECTOR('',#95626,1000.) ;
#15485=VECTOR('',#95627,1000.) ;
#15486=VECTOR('',#95630,1000.) ;
#15487=VECTOR('',#95635,1000.) ;
#15488=VECTOR('',#95636,1000.) ;
#15489=VECTOR('',#95639,1000.) ;
#15490=VECTOR('',#95644,1000.) ;
#15491=VECTOR('',#95645,1000.) ;
#15492=VECTOR('',#95660,1000.) ;
#15493=VECTOR('',#95661,1000.) ;
#15494=VECTOR('',#95662,1000.) ;
#15495=VECTOR('',#95663,1000.) ;
#15496=VECTOR('',#95666,1000.) ;
#15497=VECTOR('',#95667,1000.) ;
#15498=VECTOR('',#95668,1000.) ;
#15499=VECTOR('',#95671,1000.) ;
#15500=VECTOR('',#95672,1000.) ;
#15501=VECTOR('',#95673,1000.) ;
#15502=VECTOR('',#95676,1000.) ;
#15503=VECTOR('',#95677,1000.) ;
#15504=VECTOR('',#95678,1000.) ;
#15505=VECTOR('',#95679,1000.) ;
#15506=VECTOR('',#95682,1000.) ;
#15507=VECTOR('',#95683,1000.) ;
#15508=VECTOR('',#95684,1000.) ;
#15509=VECTOR('',#95685,1000.) ;
#15510=VECTOR('',#95688,1000.) ;
#15511=VECTOR('',#95689,1000.) ;
#15512=VECTOR('',#95690,1000.) ;
#15513=VECTOR('',#95693,1000.) ;
#15514=VECTOR('',#95694,1000.) ;
#15515=VECTOR('',#95695,1000.) ;
#15516=VECTOR('',#95698,1000.) ;
#15517=VECTOR('',#95699,1000.) ;
#15518=VECTOR('',#95700,1000.) ;
#15519=VECTOR('',#95701,1000.) ;
#15520=VECTOR('',#95704,1000.) ;
#15521=VECTOR('',#95705,1000.) ;
#15522=VECTOR('',#95706,1000.) ;
#15523=VECTOR('',#95707,1000.) ;
#15524=VECTOR('',#95710,1000.) ;
#15525=VECTOR('',#95711,1000.) ;
#15526=VECTOR('',#95712,1000.) ;
#15527=VECTOR('',#95713,1000.) ;
#15528=VECTOR('',#95716,1000.) ;
#15529=VECTOR('',#95717,1000.) ;
#15530=VECTOR('',#95718,1000.) ;
#15531=VECTOR('',#95719,1000.) ;
#15532=VECTOR('',#95722,1000.) ;
#15533=VECTOR('',#95723,1000.) ;
#15534=VECTOR('',#95724,1000.) ;
#15535=VECTOR('',#95725,1000.) ;
#15536=VECTOR('',#95728,1000.) ;
#15537=VECTOR('',#95733,1000.) ;
#15538=VECTOR('',#95734,1000.) ;
#15539=VECTOR('',#95737,1000.) ;
#15540=VECTOR('',#95742,1000.) ;
#15541=VECTOR('',#95743,1000.) ;
#15542=VECTOR('',#95758,1000.) ;
#15543=VECTOR('',#95759,1000.) ;
#15544=VECTOR('',#95760,1000.) ;
#15545=VECTOR('',#95761,1000.) ;
#15546=VECTOR('',#95764,1000.) ;
#15547=VECTOR('',#95765,1000.) ;
#15548=VECTOR('',#95766,1000.) ;
#15549=VECTOR('',#95769,1000.) ;
#15550=VECTOR('',#95770,1000.) ;
#15551=VECTOR('',#95771,1000.) ;
#15552=VECTOR('',#95774,1000.) ;
#15553=VECTOR('',#95775,1000.) ;
#15554=VECTOR('',#95776,1000.) ;
#15555=VECTOR('',#95777,1000.) ;
#15556=VECTOR('',#95780,1000.) ;
#15557=VECTOR('',#95781,1000.) ;
#15558=VECTOR('',#95782,1000.) ;
#15559=VECTOR('',#95783,1000.) ;
#15560=VECTOR('',#95786,1000.) ;
#15561=VECTOR('',#95787,1000.) ;
#15562=VECTOR('',#95788,1000.) ;
#15563=VECTOR('',#95791,1000.) ;
#15564=VECTOR('',#95792,1000.) ;
#15565=VECTOR('',#95793,1000.) ;
#15566=VECTOR('',#95796,1000.) ;
#15567=VECTOR('',#95797,1000.) ;
#15568=VECTOR('',#95798,1000.) ;
#15569=VECTOR('',#95799,1000.) ;
#15570=VECTOR('',#95802,1000.) ;
#15571=VECTOR('',#95803,1000.) ;
#15572=VECTOR('',#95804,1000.) ;
#15573=VECTOR('',#95805,1000.) ;
#15574=VECTOR('',#95808,1000.) ;
#15575=VECTOR('',#95809,1000.) ;
#15576=VECTOR('',#95810,1000.) ;
#15577=VECTOR('',#95811,1000.) ;
#15578=VECTOR('',#95814,1000.) ;
#15579=VECTOR('',#95815,1000.) ;
#15580=VECTOR('',#95816,1000.) ;
#15581=VECTOR('',#95817,1000.) ;
#15582=VECTOR('',#95820,1000.) ;
#15583=VECTOR('',#95821,1000.) ;
#15584=VECTOR('',#95822,1000.) ;
#15585=VECTOR('',#95823,1000.) ;
#15586=VECTOR('',#95826,1000.) ;
#15587=VECTOR('',#95831,1000.) ;
#15588=VECTOR('',#95832,1000.) ;
#15589=VECTOR('',#95835,1000.) ;
#15590=VECTOR('',#95840,1000.) ;
#15591=VECTOR('',#95841,1000.) ;
#15592=VECTOR('',#95856,1000.) ;
#15593=VECTOR('',#95857,1000.) ;
#15594=VECTOR('',#95858,1000.) ;
#15595=VECTOR('',#95859,1000.) ;
#15596=VECTOR('',#95862,1000.) ;
#15597=VECTOR('',#95863,1000.) ;
#15598=VECTOR('',#95864,1000.) ;
#15599=VECTOR('',#95867,1000.) ;
#15600=VECTOR('',#95868,1000.) ;
#15601=VECTOR('',#95869,1000.) ;
#15602=VECTOR('',#95872,1000.) ;
#15603=VECTOR('',#95873,1000.) ;
#15604=VECTOR('',#95874,1000.) ;
#15605=VECTOR('',#95875,1000.) ;
#15606=VECTOR('',#95878,1000.) ;
#15607=VECTOR('',#95879,1000.) ;
#15608=VECTOR('',#95880,1000.) ;
#15609=VECTOR('',#95881,1000.) ;
#15610=VECTOR('',#95884,1000.) ;
#15611=VECTOR('',#95885,1000.) ;
#15612=VECTOR('',#95886,1000.) ;
#15613=VECTOR('',#95889,1000.) ;
#15614=VECTOR('',#95890,1000.) ;
#15615=VECTOR('',#95891,1000.) ;
#15616=VECTOR('',#95894,1000.) ;
#15617=VECTOR('',#95895,1000.) ;
#15618=VECTOR('',#95896,1000.) ;
#15619=VECTOR('',#95897,1000.) ;
#15620=VECTOR('',#95900,1000.) ;
#15621=VECTOR('',#95901,1000.) ;
#15622=VECTOR('',#95902,1000.) ;
#15623=VECTOR('',#95903,1000.) ;
#15624=VECTOR('',#95906,1000.) ;
#15625=VECTOR('',#95907,1000.) ;
#15626=VECTOR('',#95908,1000.) ;
#15627=VECTOR('',#95909,1000.) ;
#15628=VECTOR('',#95912,1000.) ;
#15629=VECTOR('',#95913,1000.) ;
#15630=VECTOR('',#95914,1000.) ;
#15631=VECTOR('',#95915,1000.) ;
#15632=VECTOR('',#95918,1000.) ;
#15633=VECTOR('',#95919,1000.) ;
#15634=VECTOR('',#95920,1000.) ;
#15635=VECTOR('',#95921,1000.) ;
#15636=VECTOR('',#95924,1000.) ;
#15637=VECTOR('',#95929,1000.) ;
#15638=VECTOR('',#95930,1000.) ;
#15639=VECTOR('',#95933,1000.) ;
#15640=VECTOR('',#95938,1000.) ;
#15641=VECTOR('',#95939,1000.) ;
#15642=VECTOR('',#95954,1000.) ;
#15643=VECTOR('',#95955,1000.) ;
#15644=VECTOR('',#95956,1000.) ;
#15645=VECTOR('',#95957,1000.) ;
#15646=VECTOR('',#95960,1000.) ;
#15647=VECTOR('',#95961,1000.) ;
#15648=VECTOR('',#95962,1000.) ;
#15649=VECTOR('',#95965,1000.) ;
#15650=VECTOR('',#95966,1000.) ;
#15651=VECTOR('',#95967,1000.) ;
#15652=VECTOR('',#95970,1000.) ;
#15653=VECTOR('',#95971,1000.) ;
#15654=VECTOR('',#95972,1000.) ;
#15655=VECTOR('',#95973,1000.) ;
#15656=VECTOR('',#95976,1000.) ;
#15657=VECTOR('',#95977,1000.) ;
#15658=VECTOR('',#95978,1000.) ;
#15659=VECTOR('',#95979,1000.) ;
#15660=VECTOR('',#95982,1000.) ;
#15661=VECTOR('',#95983,1000.) ;
#15662=VECTOR('',#95984,1000.) ;
#15663=VECTOR('',#95987,1000.) ;
#15664=VECTOR('',#95988,1000.) ;
#15665=VECTOR('',#95989,1000.) ;
#15666=VECTOR('',#95992,1000.) ;
#15667=VECTOR('',#95993,1000.) ;
#15668=VECTOR('',#95994,1000.) ;
#15669=VECTOR('',#95995,1000.) ;
#15670=VECTOR('',#95998,1000.) ;
#15671=VECTOR('',#95999,1000.) ;
#15672=VECTOR('',#96000,1000.) ;
#15673=VECTOR('',#96001,1000.) ;
#15674=VECTOR('',#96004,1000.) ;
#15675=VECTOR('',#96005,1000.) ;
#15676=VECTOR('',#96006,1000.) ;
#15677=VECTOR('',#96007,1000.) ;
#15678=VECTOR('',#96010,1000.) ;
#15679=VECTOR('',#96011,1000.) ;
#15680=VECTOR('',#96012,1000.) ;
#15681=VECTOR('',#96013,1000.) ;
#15682=VECTOR('',#96016,1000.) ;
#15683=VECTOR('',#96017,1000.) ;
#15684=VECTOR('',#96018,1000.) ;
#15685=VECTOR('',#96019,1000.) ;
#15686=VECTOR('',#96022,1000.) ;
#15687=VECTOR('',#96027,1000.) ;
#15688=VECTOR('',#96028,1000.) ;
#15689=VECTOR('',#96031,1000.) ;
#15690=VECTOR('',#96036,1000.) ;
#15691=VECTOR('',#96037,1000.) ;
#15692=VECTOR('',#96052,1000.) ;
#15693=VECTOR('',#96053,1000.) ;
#15694=VECTOR('',#96054,1000.) ;
#15695=VECTOR('',#96055,1000.) ;
#15696=VECTOR('',#96058,1000.) ;
#15697=VECTOR('',#96059,1000.) ;
#15698=VECTOR('',#96060,1000.) ;
#15699=VECTOR('',#96063,1000.) ;
#15700=VECTOR('',#96064,1000.) ;
#15701=VECTOR('',#96065,1000.) ;
#15702=VECTOR('',#96068,1000.) ;
#15703=VECTOR('',#96069,1000.) ;
#15704=VECTOR('',#96070,1000.) ;
#15705=VECTOR('',#96071,1000.) ;
#15706=VECTOR('',#96074,1000.) ;
#15707=VECTOR('',#96075,1000.) ;
#15708=VECTOR('',#96076,1000.) ;
#15709=VECTOR('',#96077,1000.) ;
#15710=VECTOR('',#96080,1000.) ;
#15711=VECTOR('',#96081,1000.) ;
#15712=VECTOR('',#96082,1000.) ;
#15713=VECTOR('',#96085,1000.) ;
#15714=VECTOR('',#96086,1000.) ;
#15715=VECTOR('',#96087,1000.) ;
#15716=VECTOR('',#96090,1000.) ;
#15717=VECTOR('',#96091,1000.) ;
#15718=VECTOR('',#96092,1000.) ;
#15719=VECTOR('',#96093,1000.) ;
#15720=VECTOR('',#96096,1000.) ;
#15721=VECTOR('',#96097,1000.) ;
#15722=VECTOR('',#96098,1000.) ;
#15723=VECTOR('',#96099,1000.) ;
#15724=VECTOR('',#96102,1000.) ;
#15725=VECTOR('',#96103,1000.) ;
#15726=VECTOR('',#96104,1000.) ;
#15727=VECTOR('',#96105,1000.) ;
#15728=VECTOR('',#96108,1000.) ;
#15729=VECTOR('',#96109,1000.) ;
#15730=VECTOR('',#96110,1000.) ;
#15731=VECTOR('',#96111,1000.) ;
#15732=VECTOR('',#96114,1000.) ;
#15733=VECTOR('',#96115,1000.) ;
#15734=VECTOR('',#96116,1000.) ;
#15735=VECTOR('',#96117,1000.) ;
#15736=VECTOR('',#96120,1000.) ;
#15737=VECTOR('',#96125,1000.) ;
#15738=VECTOR('',#96126,1000.) ;
#15739=VECTOR('',#96129,1000.) ;
#15740=VECTOR('',#96134,1000.) ;
#15741=VECTOR('',#96135,1000.) ;
#15742=VECTOR('',#96150,1000.) ;
#15743=VECTOR('',#96151,1000.) ;
#15744=VECTOR('',#96152,1000.) ;
#15745=VECTOR('',#96153,1000.) ;
#15746=VECTOR('',#96156,1000.) ;
#15747=VECTOR('',#96157,1000.) ;
#15748=VECTOR('',#96158,1000.) ;
#15749=VECTOR('',#96161,1000.) ;
#15750=VECTOR('',#96162,1000.) ;
#15751=VECTOR('',#96163,1000.) ;
#15752=VECTOR('',#96166,1000.) ;
#15753=VECTOR('',#96167,1000.) ;
#15754=VECTOR('',#96168,1000.) ;
#15755=VECTOR('',#96169,1000.) ;
#15756=VECTOR('',#96172,1000.) ;
#15757=VECTOR('',#96173,1000.) ;
#15758=VECTOR('',#96174,1000.) ;
#15759=VECTOR('',#96175,1000.) ;
#15760=VECTOR('',#96178,1000.) ;
#15761=VECTOR('',#96179,1000.) ;
#15762=VECTOR('',#96180,1000.) ;
#15763=VECTOR('',#96183,1000.) ;
#15764=VECTOR('',#96184,1000.) ;
#15765=VECTOR('',#96185,1000.) ;
#15766=VECTOR('',#96188,1000.) ;
#15767=VECTOR('',#96189,1000.) ;
#15768=VECTOR('',#96190,1000.) ;
#15769=VECTOR('',#96191,1000.) ;
#15770=VECTOR('',#96194,1000.) ;
#15771=VECTOR('',#96195,1000.) ;
#15772=VECTOR('',#96196,1000.) ;
#15773=VECTOR('',#96197,1000.) ;
#15774=VECTOR('',#96200,1000.) ;
#15775=VECTOR('',#96201,1000.) ;
#15776=VECTOR('',#96202,1000.) ;
#15777=VECTOR('',#96203,1000.) ;
#15778=VECTOR('',#96206,1000.) ;
#15779=VECTOR('',#96207,1000.) ;
#15780=VECTOR('',#96208,1000.) ;
#15781=VECTOR('',#96209,1000.) ;
#15782=VECTOR('',#96212,1000.) ;
#15783=VECTOR('',#96213,1000.) ;
#15784=VECTOR('',#96214,1000.) ;
#15785=VECTOR('',#96215,1000.) ;
#15786=VECTOR('',#96218,1000.) ;
#15787=VECTOR('',#96223,1000.) ;
#15788=VECTOR('',#96224,1000.) ;
#15789=VECTOR('',#96227,1000.) ;
#15790=VECTOR('',#96232,1000.) ;
#15791=VECTOR('',#96233,1000.) ;
#15792=VECTOR('',#96248,1000.) ;
#15793=VECTOR('',#96249,1000.) ;
#15794=VECTOR('',#96250,1000.) ;
#15795=VECTOR('',#96251,1000.) ;
#15796=VECTOR('',#96254,1000.) ;
#15797=VECTOR('',#96255,1000.) ;
#15798=VECTOR('',#96256,1000.) ;
#15799=VECTOR('',#96259,1000.) ;
#15800=VECTOR('',#96260,1000.) ;
#15801=VECTOR('',#96261,1000.) ;
#15802=VECTOR('',#96264,1000.) ;
#15803=VECTOR('',#96265,1000.) ;
#15804=VECTOR('',#96266,1000.) ;
#15805=VECTOR('',#96267,1000.) ;
#15806=VECTOR('',#96270,1000.) ;
#15807=VECTOR('',#96271,1000.) ;
#15808=VECTOR('',#96272,1000.) ;
#15809=VECTOR('',#96273,1000.) ;
#15810=VECTOR('',#96276,1000.) ;
#15811=VECTOR('',#96277,1000.) ;
#15812=VECTOR('',#96278,1000.) ;
#15813=VECTOR('',#96281,1000.) ;
#15814=VECTOR('',#96282,1000.) ;
#15815=VECTOR('',#96283,1000.) ;
#15816=VECTOR('',#96286,1000.) ;
#15817=VECTOR('',#96287,1000.) ;
#15818=VECTOR('',#96288,1000.) ;
#15819=VECTOR('',#96289,1000.) ;
#15820=VECTOR('',#96292,1000.) ;
#15821=VECTOR('',#96293,1000.) ;
#15822=VECTOR('',#96294,1000.) ;
#15823=VECTOR('',#96295,1000.) ;
#15824=VECTOR('',#96298,1000.) ;
#15825=VECTOR('',#96299,1000.) ;
#15826=VECTOR('',#96300,1000.) ;
#15827=VECTOR('',#96301,1000.) ;
#15828=VECTOR('',#96304,1000.) ;
#15829=VECTOR('',#96305,1000.) ;
#15830=VECTOR('',#96306,1000.) ;
#15831=VECTOR('',#96307,1000.) ;
#15832=VECTOR('',#96310,1000.) ;
#15833=VECTOR('',#96311,1000.) ;
#15834=VECTOR('',#96312,1000.) ;
#15835=VECTOR('',#96313,1000.) ;
#15836=VECTOR('',#96316,1000.) ;
#15837=VECTOR('',#96321,1000.) ;
#15838=VECTOR('',#96322,1000.) ;
#15839=VECTOR('',#96325,1000.) ;
#15840=VECTOR('',#96330,1000.) ;
#15841=VECTOR('',#96331,1000.) ;
#15842=VECTOR('',#96346,1000.) ;
#15843=VECTOR('',#96347,1000.) ;
#15844=VECTOR('',#96348,1000.) ;
#15845=VECTOR('',#96349,1000.) ;
#15846=VECTOR('',#96352,1000.) ;
#15847=VECTOR('',#96353,1000.) ;
#15848=VECTOR('',#96354,1000.) ;
#15849=VECTOR('',#96357,1000.) ;
#15850=VECTOR('',#96358,1000.) ;
#15851=VECTOR('',#96359,1000.) ;
#15852=VECTOR('',#96362,1000.) ;
#15853=VECTOR('',#96363,1000.) ;
#15854=VECTOR('',#96364,1000.) ;
#15855=VECTOR('',#96365,1000.) ;
#15856=VECTOR('',#96368,1000.) ;
#15857=VECTOR('',#96369,1000.) ;
#15858=VECTOR('',#96370,1000.) ;
#15859=VECTOR('',#96371,1000.) ;
#15860=VECTOR('',#96374,1000.) ;
#15861=VECTOR('',#96375,1000.) ;
#15862=VECTOR('',#96376,1000.) ;
#15863=VECTOR('',#96379,1000.) ;
#15864=VECTOR('',#96380,1000.) ;
#15865=VECTOR('',#96381,1000.) ;
#15866=VECTOR('',#96384,1000.) ;
#15867=VECTOR('',#96385,1000.) ;
#15868=VECTOR('',#96386,1000.) ;
#15869=VECTOR('',#96387,1000.) ;
#15870=VECTOR('',#96390,1000.) ;
#15871=VECTOR('',#96391,1000.) ;
#15872=VECTOR('',#96392,1000.) ;
#15873=VECTOR('',#96393,1000.) ;
#15874=VECTOR('',#96396,1000.) ;
#15875=VECTOR('',#96397,1000.) ;
#15876=VECTOR('',#96398,1000.) ;
#15877=VECTOR('',#96399,1000.) ;
#15878=VECTOR('',#96402,1000.) ;
#15879=VECTOR('',#96403,1000.) ;
#15880=VECTOR('',#96404,1000.) ;
#15881=VECTOR('',#96405,1000.) ;
#15882=VECTOR('',#96408,1000.) ;
#15883=VECTOR('',#96409,1000.) ;
#15884=VECTOR('',#96410,1000.) ;
#15885=VECTOR('',#96411,1000.) ;
#15886=VECTOR('',#96414,1000.) ;
#15887=VECTOR('',#96419,1000.) ;
#15888=VECTOR('',#96420,1000.) ;
#15889=VECTOR('',#96423,1000.) ;
#15890=VECTOR('',#96428,1000.) ;
#15891=VECTOR('',#96429,1000.) ;
#15892=VECTOR('',#96444,1000.) ;
#15893=VECTOR('',#96445,1000.) ;
#15894=VECTOR('',#96446,1000.) ;
#15895=VECTOR('',#96447,1000.) ;
#15896=VECTOR('',#96450,1000.) ;
#15897=VECTOR('',#96451,1000.) ;
#15898=VECTOR('',#96452,1000.) ;
#15899=VECTOR('',#96455,1000.) ;
#15900=VECTOR('',#96456,1000.) ;
#15901=VECTOR('',#96457,1000.) ;
#15902=VECTOR('',#96460,1000.) ;
#15903=VECTOR('',#96461,1000.) ;
#15904=VECTOR('',#96462,1000.) ;
#15905=VECTOR('',#96463,1000.) ;
#15906=VECTOR('',#96466,1000.) ;
#15907=VECTOR('',#96467,1000.) ;
#15908=VECTOR('',#96468,1000.) ;
#15909=VECTOR('',#96469,1000.) ;
#15910=VECTOR('',#96472,1000.) ;
#15911=VECTOR('',#96473,1000.) ;
#15912=VECTOR('',#96474,1000.) ;
#15913=VECTOR('',#96477,1000.) ;
#15914=VECTOR('',#96478,1000.) ;
#15915=VECTOR('',#96479,1000.) ;
#15916=VECTOR('',#96482,1000.) ;
#15917=VECTOR('',#96483,1000.) ;
#15918=VECTOR('',#96484,1000.) ;
#15919=VECTOR('',#96485,1000.) ;
#15920=VECTOR('',#96488,1000.) ;
#15921=VECTOR('',#96489,1000.) ;
#15922=VECTOR('',#96490,1000.) ;
#15923=VECTOR('',#96491,1000.) ;
#15924=VECTOR('',#96494,1000.) ;
#15925=VECTOR('',#96495,1000.) ;
#15926=VECTOR('',#96496,1000.) ;
#15927=VECTOR('',#96497,1000.) ;
#15928=VECTOR('',#96500,1000.) ;
#15929=VECTOR('',#96501,1000.) ;
#15930=VECTOR('',#96502,1000.) ;
#15931=VECTOR('',#96503,1000.) ;
#15932=VECTOR('',#96506,1000.) ;
#15933=VECTOR('',#96507,1000.) ;
#15934=VECTOR('',#96508,1000.) ;
#15935=VECTOR('',#96509,1000.) ;
#15936=VECTOR('',#96512,1000.) ;
#15937=VECTOR('',#96513,1000.) ;
#15938=VECTOR('',#96514,1000.) ;
#15939=VECTOR('',#96515,1000.) ;
#15940=VECTOR('',#96518,1000.) ;
#15941=VECTOR('',#96519,1000.) ;
#15942=VECTOR('',#96520,1000.) ;
#15943=VECTOR('',#96521,1000.) ;
#15944=VECTOR('',#96524,1000.) ;
#15945=VECTOR('',#96525,1000.) ;
#15946=VECTOR('',#96526,1000.) ;
#15947=VECTOR('',#96527,1000.) ;
#15948=VECTOR('',#96530,1000.) ;
#15949=VECTOR('',#96531,1000.) ;
#15950=VECTOR('',#96532,1000.) ;
#15951=VECTOR('',#96533,1000.) ;
#15952=VECTOR('',#96536,1000.) ;
#15953=VECTOR('',#96537,1000.) ;
#15954=VECTOR('',#96538,1000.) ;
#15955=VECTOR('',#96539,1000.) ;
#15956=VECTOR('',#96542,1000.) ;
#15957=VECTOR('',#96543,1000.) ;
#15958=VECTOR('',#96544,1000.) ;
#15959=VECTOR('',#96545,1000.) ;
#15960=VECTOR('',#96548,1000.) ;
#15961=VECTOR('',#96549,1000.) ;
#15962=VECTOR('',#96550,1000.) ;
#15963=VECTOR('',#96551,1000.) ;
#15964=VECTOR('',#96554,1000.) ;
#15965=VECTOR('',#96555,1000.) ;
#15966=VECTOR('',#96556,1000.) ;
#15967=VECTOR('',#96557,1000.) ;
#15968=VECTOR('',#96560,1000.) ;
#15969=VECTOR('',#96561,1000.) ;
#15970=VECTOR('',#96562,1000.) ;
#15971=VECTOR('',#96563,1000.) ;
#15972=VECTOR('',#96566,1000.) ;
#15973=VECTOR('',#96567,1000.) ;
#15974=VECTOR('',#96568,1000.) ;
#15975=VECTOR('',#96569,1000.) ;
#15976=VECTOR('',#96572,1000.) ;
#15977=VECTOR('',#96573,1000.) ;
#15978=VECTOR('',#96574,1000.) ;
#15979=VECTOR('',#96575,1000.) ;
#15980=VECTOR('',#96578,1000.) ;
#15981=VECTOR('',#96579,1000.) ;
#15982=VECTOR('',#96580,1000.) ;
#15983=VECTOR('',#96581,1000.) ;
#15984=VECTOR('',#96584,1000.) ;
#15985=VECTOR('',#96585,1000.) ;
#15986=VECTOR('',#96586,1000.) ;
#15987=VECTOR('',#96587,1000.) ;
#15988=VECTOR('',#96590,1000.) ;
#15989=VECTOR('',#96591,1000.) ;
#15990=VECTOR('',#96592,1000.) ;
#15991=VECTOR('',#96593,1000.) ;
#15992=VECTOR('',#96596,1000.) ;
#15993=VECTOR('',#96597,1000.) ;
#15994=VECTOR('',#96598,1000.) ;
#15995=VECTOR('',#96599,1000.) ;
#15996=VECTOR('',#96602,1000.) ;
#15997=VECTOR('',#96603,1000.) ;
#15998=VECTOR('',#96604,1000.) ;
#15999=VECTOR('',#96605,1000.) ;
#16000=VECTOR('',#96608,1000.) ;
#16001=VECTOR('',#96609,1000.) ;
#16002=VECTOR('',#96610,1000.) ;
#16003=VECTOR('',#96611,1000.) ;
#16004=VECTOR('',#96614,1000.) ;
#16005=VECTOR('',#96615,1000.) ;
#16006=VECTOR('',#96616,1000.) ;
#16007=VECTOR('',#96617,1000.) ;
#16008=VECTOR('',#96620,1000.) ;
#16009=VECTOR('',#96621,1000.) ;
#16010=VECTOR('',#96622,1000.) ;
#16011=VECTOR('',#96623,1000.) ;
#16012=VECTOR('',#96626,1000.) ;
#16013=VECTOR('',#96627,1000.) ;
#16014=VECTOR('',#96628,1000.) ;
#16015=VECTOR('',#96629,1000.) ;
#16016=VECTOR('',#96632,1000.) ;
#16017=VECTOR('',#96633,1000.) ;
#16018=VECTOR('',#96634,1000.) ;
#16019=VECTOR('',#96635,1000.) ;
#16020=VECTOR('',#96638,1000.) ;
#16021=VECTOR('',#96639,1000.) ;
#16022=VECTOR('',#96640,1000.) ;
#16023=VECTOR('',#96641,1000.) ;
#16024=VECTOR('',#96644,1000.) ;
#16025=VECTOR('',#96645,1000.) ;
#16026=VECTOR('',#96646,1000.) ;
#16027=VECTOR('',#96647,1000.) ;
#16028=VECTOR('',#96650,1000.) ;
#16029=VECTOR('',#96651,1000.) ;
#16030=VECTOR('',#96652,1000.) ;
#16031=VECTOR('',#96653,1000.) ;
#16032=VECTOR('',#96656,1000.) ;
#16033=VECTOR('',#96657,1000.) ;
#16034=VECTOR('',#96658,1000.) ;
#16035=VECTOR('',#96659,1000.) ;
#16036=VECTOR('',#96662,1000.) ;
#16037=VECTOR('',#96663,1000.) ;
#16038=VECTOR('',#96664,1000.) ;
#16039=VECTOR('',#96665,1000.) ;
#16040=VECTOR('',#96668,1000.) ;
#16041=VECTOR('',#96669,1000.) ;
#16042=VECTOR('',#96670,1000.) ;
#16043=VECTOR('',#96671,1000.) ;
#16044=VECTOR('',#96674,1000.) ;
#16045=VECTOR('',#96675,1000.) ;
#16046=VECTOR('',#96676,1000.) ;
#16047=VECTOR('',#96677,1000.) ;
#16048=VECTOR('',#96680,1000.) ;
#16049=VECTOR('',#96681,1000.) ;
#16050=VECTOR('',#96682,1000.) ;
#16051=VECTOR('',#96683,1000.) ;
#16052=VECTOR('',#96686,1000.) ;
#16053=VECTOR('',#96687,1000.) ;
#16054=VECTOR('',#96688,1000.) ;
#16055=VECTOR('',#96689,1000.) ;
#16056=VECTOR('',#96692,1000.) ;
#16057=VECTOR('',#96693,1000.) ;
#16058=VECTOR('',#96694,1000.) ;
#16059=VECTOR('',#96695,1000.) ;
#18077=FACE_OUTER_BOUND('',#22361,.T.) ;
#18078=FACE_OUTER_BOUND('',#22362,.T.) ;
#18079=FACE_OUTER_BOUND('',#22363,.T.) ;
#18080=FACE_OUTER_BOUND('',#22364,.T.) ;
#18081=FACE_OUTER_BOUND('',#22365,.T.) ;
#18082=FACE_OUTER_BOUND('',#22366,.T.) ;
#18083=FACE_OUTER_BOUND('',#22367,.T.) ;
#18084=FACE_OUTER_BOUND('',#22368,.T.) ;
#18085=FACE_OUTER_BOUND('',#22369,.T.) ;
#18086=FACE_OUTER_BOUND('',#22370,.T.) ;
#18087=FACE_OUTER_BOUND('',#22371,.T.) ;
#18088=FACE_OUTER_BOUND('',#22372,.T.) ;
#18089=FACE_OUTER_BOUND('',#22373,.T.) ;
#18090=FACE_OUTER_BOUND('',#22374,.T.) ;
#18091=FACE_OUTER_BOUND('',#22375,.T.) ;
#18092=FACE_OUTER_BOUND('',#22376,.T.) ;
#18093=FACE_OUTER_BOUND('',#22377,.T.) ;
#18094=FACE_OUTER_BOUND('',#22378,.T.) ;
#18095=FACE_OUTER_BOUND('',#22379,.T.) ;
#18096=FACE_OUTER_BOUND('',#22380,.T.) ;
#18097=FACE_OUTER_BOUND('',#22381,.T.) ;
#18098=FACE_OUTER_BOUND('',#22382,.T.) ;
#18099=FACE_OUTER_BOUND('',#22383,.T.) ;
#18100=FACE_OUTER_BOUND('',#22384,.T.) ;
#18101=FACE_OUTER_BOUND('',#22385,.T.) ;
#18102=FACE_OUTER_BOUND('',#22386,.T.) ;
#18103=FACE_OUTER_BOUND('',#22387,.T.) ;
#18104=FACE_OUTER_BOUND('',#22388,.T.) ;
#18105=FACE_OUTER_BOUND('',#22389,.T.) ;
#18106=FACE_OUTER_BOUND('',#22390,.T.) ;
#18107=FACE_OUTER_BOUND('',#22391,.T.) ;
#18108=FACE_OUTER_BOUND('',#22392,.T.) ;
#18109=FACE_OUTER_BOUND('',#22393,.T.) ;
#18110=FACE_OUTER_BOUND('',#22394,.T.) ;
#18111=FACE_OUTER_BOUND('',#22395,.T.) ;
#18112=FACE_OUTER_BOUND('',#22396,.T.) ;
#18113=FACE_OUTER_BOUND('',#22397,.T.) ;
#18114=FACE_OUTER_BOUND('',#22398,.T.) ;
#18115=FACE_OUTER_BOUND('',#22399,.T.) ;
#18116=FACE_OUTER_BOUND('',#22400,.T.) ;
#18117=FACE_OUTER_BOUND('',#22401,.T.) ;
#18118=FACE_OUTER_BOUND('',#22402,.T.) ;
#18119=FACE_OUTER_BOUND('',#22403,.T.) ;
#18120=FACE_OUTER_BOUND('',#22404,.T.) ;
#18121=FACE_OUTER_BOUND('',#22405,.T.) ;
#18122=FACE_OUTER_BOUND('',#22406,.T.) ;
#18123=FACE_OUTER_BOUND('',#22407,.T.) ;
#18124=FACE_OUTER_BOUND('',#22408,.T.) ;
#18125=FACE_OUTER_BOUND('',#22409,.T.) ;
#18126=FACE_OUTER_BOUND('',#22410,.T.) ;
#18127=FACE_OUTER_BOUND('',#22411,.T.) ;
#18128=FACE_OUTER_BOUND('',#22412,.T.) ;
#18129=FACE_OUTER_BOUND('',#22413,.T.) ;
#18130=FACE_OUTER_BOUND('',#22414,.T.) ;
#18131=FACE_OUTER_BOUND('',#22415,.T.) ;
#18132=FACE_OUTER_BOUND('',#22416,.T.) ;
#18133=FACE_OUTER_BOUND('',#22417,.T.) ;
#18134=FACE_OUTER_BOUND('',#22418,.T.) ;
#18135=FACE_OUTER_BOUND('',#22419,.T.) ;
#18136=FACE_OUTER_BOUND('',#22420,.T.) ;
#18137=FACE_OUTER_BOUND('',#22421,.T.) ;
#18138=FACE_OUTER_BOUND('',#22422,.T.) ;
#18139=FACE_OUTER_BOUND('',#22423,.T.) ;
#18140=FACE_OUTER_BOUND('',#22424,.T.) ;
#18141=FACE_OUTER_BOUND('',#22425,.T.) ;
#18142=FACE_OUTER_BOUND('',#22426,.T.) ;
#18143=FACE_OUTER_BOUND('',#22427,.T.) ;
#18144=FACE_OUTER_BOUND('',#22428,.T.) ;
#18145=FACE_OUTER_BOUND('',#22429,.T.) ;
#18146=FACE_OUTER_BOUND('',#22430,.T.) ;
#18147=FACE_OUTER_BOUND('',#22431,.T.) ;
#18148=FACE_OUTER_BOUND('',#22432,.T.) ;
#18149=FACE_OUTER_BOUND('',#22433,.T.) ;
#18150=FACE_OUTER_BOUND('',#22434,.T.) ;
#18151=FACE_OUTER_BOUND('',#22435,.T.) ;
#18152=FACE_OUTER_BOUND('',#22436,.T.) ;
#18153=FACE_OUTER_BOUND('',#22437,.T.) ;
#18154=FACE_OUTER_BOUND('',#22438,.T.) ;
#18155=FACE_OUTER_BOUND('',#22439,.T.) ;
#18156=FACE_OUTER_BOUND('',#22440,.T.) ;
#18157=FACE_OUTER_BOUND('',#22441,.T.) ;
#18158=FACE_OUTER_BOUND('',#22442,.T.) ;
#18159=FACE_OUTER_BOUND('',#22443,.T.) ;
#18160=FACE_OUTER_BOUND('',#22444,.T.) ;
#18161=FACE_OUTER_BOUND('',#22445,.T.) ;
#18162=FACE_OUTER_BOUND('',#22446,.T.) ;
#18163=FACE_OUTER_BOUND('',#22447,.T.) ;
#18164=FACE_OUTER_BOUND('',#22448,.T.) ;
#18165=FACE_OUTER_BOUND('',#22449,.T.) ;
#18166=FACE_OUTER_BOUND('',#22450,.T.) ;
#18167=FACE_OUTER_BOUND('',#22451,.T.) ;
#18168=FACE_OUTER_BOUND('',#22452,.T.) ;
#18169=FACE_OUTER_BOUND('',#22453,.T.) ;
#18170=FACE_OUTER_BOUND('',#22454,.T.) ;
#18171=FACE_OUTER_BOUND('',#22455,.T.) ;
#18172=FACE_OUTER_BOUND('',#22456,.T.) ;
#18173=FACE_OUTER_BOUND('',#22457,.T.) ;
#18174=FACE_OUTER_BOUND('',#22458,.T.) ;
#18175=FACE_OUTER_BOUND('',#22459,.T.) ;
#18176=FACE_OUTER_BOUND('',#22460,.T.) ;
#18177=FACE_OUTER_BOUND('',#22461,.T.) ;
#18178=FACE_OUTER_BOUND('',#22462,.T.) ;
#18179=FACE_OUTER_BOUND('',#22463,.T.) ;
#18180=FACE_OUTER_BOUND('',#22464,.T.) ;
#18181=FACE_OUTER_BOUND('',#22465,.T.) ;
#18182=FACE_OUTER_BOUND('',#22466,.T.) ;
#18183=FACE_OUTER_BOUND('',#22467,.T.) ;
#18184=FACE_OUTER_BOUND('',#22468,.T.) ;
#18185=FACE_OUTER_BOUND('',#22469,.T.) ;
#18186=FACE_OUTER_BOUND('',#22470,.T.) ;
#18187=FACE_OUTER_BOUND('',#22471,.T.) ;
#18188=FACE_OUTER_BOUND('',#22472,.T.) ;
#18189=FACE_OUTER_BOUND('',#22473,.T.) ;
#18190=FACE_OUTER_BOUND('',#22474,.T.) ;
#18191=FACE_OUTER_BOUND('',#22475,.T.) ;
#18192=FACE_OUTER_BOUND('',#22476,.T.) ;
#18193=FACE_OUTER_BOUND('',#22477,.T.) ;
#18194=FACE_OUTER_BOUND('',#22478,.T.) ;
#18195=FACE_OUTER_BOUND('',#22479,.T.) ;
#18196=FACE_OUTER_BOUND('',#22480,.T.) ;
#18197=FACE_OUTER_BOUND('',#22481,.T.) ;
#18198=FACE_OUTER_BOUND('',#22482,.T.) ;
#18199=FACE_OUTER_BOUND('',#22483,.T.) ;
#18200=FACE_OUTER_BOUND('',#22484,.T.) ;
#18201=FACE_OUTER_BOUND('',#22485,.T.) ;
#18202=FACE_OUTER_BOUND('',#22486,.T.) ;
#18203=FACE_OUTER_BOUND('',#22497,.T.) ;
#18204=FACE_OUTER_BOUND('',#22498,.T.) ;
#18205=FACE_OUTER_BOUND('',#22499,.T.) ;
#18206=FACE_OUTER_BOUND('',#22500,.T.) ;
#18207=FACE_OUTER_BOUND('',#22501,.T.) ;
#18208=FACE_OUTER_BOUND('',#22502,.T.) ;
#18209=FACE_OUTER_BOUND('',#22503,.T.) ;
#18210=FACE_OUTER_BOUND('',#22504,.T.) ;
#18211=FACE_OUTER_BOUND('',#22505,.T.) ;
#18212=FACE_OUTER_BOUND('',#22506,.T.) ;
#18213=FACE_OUTER_BOUND('',#22507,.T.) ;
#18214=FACE_OUTER_BOUND('',#22508,.T.) ;
#18215=FACE_OUTER_BOUND('',#22509,.T.) ;
#18216=FACE_OUTER_BOUND('',#22510,.T.) ;
#18217=FACE_OUTER_BOUND('',#22511,.T.) ;
#18218=FACE_OUTER_BOUND('',#22512,.T.) ;
#18219=FACE_OUTER_BOUND('',#22513,.T.) ;
#18220=FACE_OUTER_BOUND('',#22514,.T.) ;
#18221=FACE_OUTER_BOUND('',#22515,.T.) ;
#18222=FACE_OUTER_BOUND('',#22516,.T.) ;
#18223=FACE_OUTER_BOUND('',#22517,.T.) ;
#18224=FACE_OUTER_BOUND('',#22518,.T.) ;
#18225=FACE_OUTER_BOUND('',#22519,.T.) ;
#18226=FACE_OUTER_BOUND('',#22520,.T.) ;
#18227=FACE_OUTER_BOUND('',#22521,.T.) ;
#18228=FACE_OUTER_BOUND('',#22522,.T.) ;
#18229=FACE_OUTER_BOUND('',#22523,.T.) ;
#18230=FACE_OUTER_BOUND('',#22524,.T.) ;
#18231=FACE_OUTER_BOUND('',#22525,.T.) ;
#18232=FACE_OUTER_BOUND('',#22526,.T.) ;
#18233=FACE_OUTER_BOUND('',#22527,.T.) ;
#18234=FACE_OUTER_BOUND('',#22528,.T.) ;
#18235=FACE_OUTER_BOUND('',#22529,.T.) ;
#18236=FACE_OUTER_BOUND('',#22530,.T.) ;
#18237=FACE_OUTER_BOUND('',#22531,.T.) ;
#18238=FACE_OUTER_BOUND('',#22532,.T.) ;
#18239=FACE_OUTER_BOUND('',#22534,.T.) ;
#18240=FACE_OUTER_BOUND('',#22536,.T.) ;
#18241=FACE_OUTER_BOUND('',#22537,.T.) ;
#18242=FACE_OUTER_BOUND('',#22538,.T.) ;
#18243=FACE_OUTER_BOUND('',#22539,.T.) ;
#18244=FACE_OUTER_BOUND('',#22540,.T.) ;
#18245=FACE_OUTER_BOUND('',#22541,.T.) ;
#18246=FACE_OUTER_BOUND('',#22542,.T.) ;
#18247=FACE_OUTER_BOUND('',#22543,.T.) ;
#18248=FACE_OUTER_BOUND('',#22544,.T.) ;
#18249=FACE_OUTER_BOUND('',#22545,.T.) ;
#18250=FACE_OUTER_BOUND('',#22546,.T.) ;
#18251=FACE_OUTER_BOUND('',#22547,.T.) ;
#18252=FACE_OUTER_BOUND('',#22548,.T.) ;
#18253=FACE_OUTER_BOUND('',#22549,.T.) ;
#18254=FACE_OUTER_BOUND('',#22550,.T.) ;
#18255=FACE_OUTER_BOUND('',#22551,.T.) ;
#18256=FACE_OUTER_BOUND('',#22552,.T.) ;
#18257=FACE_OUTER_BOUND('',#22553,.T.) ;
#18258=FACE_OUTER_BOUND('',#22554,.T.) ;
#18259=FACE_OUTER_BOUND('',#22555,.T.) ;
#18260=FACE_OUTER_BOUND('',#22556,.T.) ;
#18261=FACE_OUTER_BOUND('',#22557,.T.) ;
#18262=FACE_OUTER_BOUND('',#22558,.T.) ;
#18263=FACE_OUTER_BOUND('',#22559,.T.) ;
#18264=FACE_OUTER_BOUND('',#22560,.T.) ;
#18265=FACE_OUTER_BOUND('',#22561,.T.) ;
#18266=FACE_OUTER_BOUND('',#22562,.T.) ;
#18267=FACE_OUTER_BOUND('',#22563,.T.) ;
#18268=FACE_OUTER_BOUND('',#22564,.T.) ;
#18269=FACE_OUTER_BOUND('',#22565,.T.) ;
#18270=FACE_OUTER_BOUND('',#22566,.T.) ;
#18271=FACE_OUTER_BOUND('',#22567,.T.) ;
#18272=FACE_OUTER_BOUND('',#22568,.T.) ;
#18273=FACE_OUTER_BOUND('',#22569,.T.) ;
#18274=FACE_OUTER_BOUND('',#22570,.T.) ;
#18275=FACE_OUTER_BOUND('',#22571,.T.) ;
#18276=FACE_OUTER_BOUND('',#22572,.T.) ;
#18277=FACE_OUTER_BOUND('',#22573,.T.) ;
#18278=FACE_OUTER_BOUND('',#22574,.T.) ;
#18279=FACE_OUTER_BOUND('',#22575,.T.) ;
#18280=FACE_OUTER_BOUND('',#22576,.T.) ;
#18281=FACE_OUTER_BOUND('',#22577,.T.) ;
#18282=FACE_OUTER_BOUND('',#22578,.T.) ;
#18283=FACE_OUTER_BOUND('',#22579,.T.) ;
#18284=FACE_OUTER_BOUND('',#22580,.T.) ;
#18285=FACE_OUTER_BOUND('',#22581,.T.) ;
#18286=FACE_OUTER_BOUND('',#22582,.T.) ;
#18287=FACE_OUTER_BOUND('',#22583,.T.) ;
#18288=FACE_OUTER_BOUND('',#22584,.T.) ;
#18289=FACE_OUTER_BOUND('',#22585,.T.) ;
#18290=FACE_OUTER_BOUND('',#22586,.T.) ;
#18291=FACE_OUTER_BOUND('',#22587,.T.) ;
#18292=FACE_OUTER_BOUND('',#22588,.T.) ;
#18293=FACE_OUTER_BOUND('',#22589,.T.) ;
#18294=FACE_OUTER_BOUND('',#22590,.T.) ;
#18295=FACE_OUTER_BOUND('',#22591,.T.) ;
#18296=FACE_OUTER_BOUND('',#22592,.T.) ;
#18297=FACE_OUTER_BOUND('',#22593,.T.) ;
#18298=FACE_OUTER_BOUND('',#22594,.T.) ;
#18299=FACE_OUTER_BOUND('',#22595,.T.) ;
#18300=FACE_OUTER_BOUND('',#22596,.T.) ;
#18301=FACE_OUTER_BOUND('',#22597,.T.) ;
#18302=FACE_OUTER_BOUND('',#22598,.T.) ;
#18303=FACE_OUTER_BOUND('',#22599,.T.) ;
#18304=FACE_OUTER_BOUND('',#22600,.T.) ;
#18305=FACE_OUTER_BOUND('',#22601,.T.) ;
#18306=FACE_OUTER_BOUND('',#22602,.T.) ;
#18307=FACE_OUTER_BOUND('',#22603,.T.) ;
#18308=FACE_OUTER_BOUND('',#22604,.T.) ;
#18309=FACE_OUTER_BOUND('',#22605,.T.) ;
#18310=FACE_OUTER_BOUND('',#22606,.T.) ;
#18311=FACE_OUTER_BOUND('',#22607,.T.) ;
#18312=FACE_OUTER_BOUND('',#22608,.T.) ;
#18313=FACE_OUTER_BOUND('',#22609,.T.) ;
#18314=FACE_OUTER_BOUND('',#22610,.T.) ;
#18315=FACE_OUTER_BOUND('',#22611,.T.) ;
#18316=FACE_OUTER_BOUND('',#22612,.T.) ;
#18317=FACE_OUTER_BOUND('',#22613,.T.) ;
#18318=FACE_OUTER_BOUND('',#22614,.T.) ;
#18319=FACE_OUTER_BOUND('',#22615,.T.) ;
#18320=FACE_OUTER_BOUND('',#22616,.T.) ;
#18321=FACE_OUTER_BOUND('',#22617,.T.) ;
#18322=FACE_OUTER_BOUND('',#22618,.T.) ;
#18323=FACE_OUTER_BOUND('',#22619,.T.) ;
#18324=FACE_OUTER_BOUND('',#22620,.T.) ;
#18325=FACE_OUTER_BOUND('',#22621,.T.) ;
#18326=FACE_OUTER_BOUND('',#22622,.T.) ;
#18327=FACE_OUTER_BOUND('',#22623,.T.) ;
#18328=FACE_OUTER_BOUND('',#22624,.T.) ;
#18329=FACE_OUTER_BOUND('',#22625,.T.) ;
#18330=FACE_OUTER_BOUND('',#22626,.T.) ;
#18331=FACE_OUTER_BOUND('',#22627,.T.) ;
#18332=FACE_OUTER_BOUND('',#22628,.T.) ;
#18333=FACE_OUTER_BOUND('',#22629,.T.) ;
#18334=FACE_OUTER_BOUND('',#22630,.T.) ;
#18335=FACE_OUTER_BOUND('',#22631,.T.) ;
#18336=FACE_OUTER_BOUND('',#22632,.T.) ;
#18337=FACE_OUTER_BOUND('',#22633,.T.) ;
#18338=FACE_OUTER_BOUND('',#22634,.T.) ;
#18339=FACE_OUTER_BOUND('',#22635,.T.) ;
#18340=FACE_OUTER_BOUND('',#22636,.T.) ;
#18341=FACE_OUTER_BOUND('',#22637,.T.) ;
#18342=FACE_OUTER_BOUND('',#22638,.T.) ;
#18343=FACE_OUTER_BOUND('',#22639,.T.) ;
#18344=FACE_OUTER_BOUND('',#22640,.T.) ;
#18345=FACE_OUTER_BOUND('',#22641,.T.) ;
#18346=FACE_OUTER_BOUND('',#22642,.T.) ;
#18347=FACE_OUTER_BOUND('',#22643,.T.) ;
#18348=FACE_OUTER_BOUND('',#22644,.T.) ;
#18349=FACE_OUTER_BOUND('',#22645,.T.) ;
#18350=FACE_OUTER_BOUND('',#22646,.T.) ;
#18351=FACE_OUTER_BOUND('',#22647,.T.) ;
#18352=FACE_OUTER_BOUND('',#22648,.T.) ;
#18353=FACE_OUTER_BOUND('',#22649,.T.) ;
#18354=FACE_OUTER_BOUND('',#22650,.T.) ;
#18355=FACE_OUTER_BOUND('',#22651,.T.) ;
#18356=FACE_OUTER_BOUND('',#22652,.T.) ;
#18357=FACE_OUTER_BOUND('',#22653,.T.) ;
#18358=FACE_OUTER_BOUND('',#22654,.T.) ;
#18359=FACE_OUTER_BOUND('',#22655,.T.) ;
#18360=FACE_OUTER_BOUND('',#22656,.T.) ;
#18361=FACE_OUTER_BOUND('',#22657,.T.) ;
#18362=FACE_OUTER_BOUND('',#22658,.T.) ;
#18363=FACE_OUTER_BOUND('',#22659,.T.) ;
#18364=FACE_OUTER_BOUND('',#22660,.T.) ;
#18365=FACE_OUTER_BOUND('',#22661,.T.) ;
#18366=FACE_OUTER_BOUND('',#22662,.T.) ;
#18367=FACE_OUTER_BOUND('',#22663,.T.) ;
#18368=FACE_OUTER_BOUND('',#22664,.T.) ;
#18369=FACE_OUTER_BOUND('',#22665,.T.) ;
#18370=FACE_OUTER_BOUND('',#22666,.T.) ;
#18371=FACE_OUTER_BOUND('',#22667,.T.) ;
#18372=FACE_OUTER_BOUND('',#22668,.T.) ;
#18373=FACE_OUTER_BOUND('',#22669,.T.) ;
#18374=FACE_OUTER_BOUND('',#22670,.T.) ;
#18375=FACE_OUTER_BOUND('',#22671,.T.) ;
#18376=FACE_OUTER_BOUND('',#22672,.T.) ;
#18377=FACE_OUTER_BOUND('',#22673,.T.) ;
#18378=FACE_OUTER_BOUND('',#22674,.T.) ;
#18379=FACE_OUTER_BOUND('',#22675,.T.) ;
#18380=FACE_OUTER_BOUND('',#22676,.T.) ;
#18381=FACE_OUTER_BOUND('',#22677,.T.) ;
#18382=FACE_OUTER_BOUND('',#22678,.T.) ;
#18383=FACE_OUTER_BOUND('',#22679,.T.) ;
#18384=FACE_OUTER_BOUND('',#22680,.T.) ;
#18385=FACE_OUTER_BOUND('',#22681,.T.) ;
#18386=FACE_OUTER_BOUND('',#22682,.T.) ;
#18387=FACE_OUTER_BOUND('',#22683,.T.) ;
#18388=FACE_OUTER_BOUND('',#22684,.T.) ;
#18389=FACE_OUTER_BOUND('',#22685,.T.) ;
#18390=FACE_OUTER_BOUND('',#22686,.T.) ;
#18391=FACE_OUTER_BOUND('',#22687,.T.) ;
#18392=FACE_OUTER_BOUND('',#22688,.T.) ;
#18393=FACE_OUTER_BOUND('',#22689,.T.) ;
#18394=FACE_OUTER_BOUND('',#22690,.T.) ;
#18395=FACE_OUTER_BOUND('',#22691,.T.) ;
#18396=FACE_OUTER_BOUND('',#22692,.T.) ;
#18397=FACE_OUTER_BOUND('',#22693,.T.) ;
#18398=FACE_OUTER_BOUND('',#22694,.T.) ;
#18399=FACE_OUTER_BOUND('',#22695,.T.) ;
#18400=FACE_OUTER_BOUND('',#22696,.T.) ;
#18401=FACE_OUTER_BOUND('',#22697,.T.) ;
#18402=FACE_OUTER_BOUND('',#22698,.T.) ;
#18403=FACE_OUTER_BOUND('',#22699,.T.) ;
#18404=FACE_OUTER_BOUND('',#22700,.T.) ;
#18405=FACE_OUTER_BOUND('',#22701,.T.) ;
#18406=FACE_OUTER_BOUND('',#22702,.T.) ;
#18407=FACE_OUTER_BOUND('',#22703,.T.) ;
#18408=FACE_OUTER_BOUND('',#22704,.T.) ;
#18409=FACE_OUTER_BOUND('',#22705,.T.) ;
#18410=FACE_OUTER_BOUND('',#22706,.T.) ;
#18411=FACE_OUTER_BOUND('',#22707,.T.) ;
#18412=FACE_OUTER_BOUND('',#22708,.T.) ;
#18413=FACE_OUTER_BOUND('',#22709,.T.) ;
#18414=FACE_OUTER_BOUND('',#22710,.T.) ;
#18415=FACE_OUTER_BOUND('',#22711,.T.) ;
#18416=FACE_OUTER_BOUND('',#22712,.T.) ;
#18417=FACE_OUTER_BOUND('',#22713,.T.) ;
#18418=FACE_OUTER_BOUND('',#22714,.T.) ;
#18419=FACE_OUTER_BOUND('',#22715,.T.) ;
#18420=FACE_OUTER_BOUND('',#22716,.T.) ;
#18421=FACE_OUTER_BOUND('',#22717,.T.) ;
#18422=FACE_OUTER_BOUND('',#22718,.T.) ;
#18423=FACE_OUTER_BOUND('',#22719,.T.) ;
#18424=FACE_OUTER_BOUND('',#22720,.T.) ;
#18425=FACE_OUTER_BOUND('',#22721,.T.) ;
#18426=FACE_OUTER_BOUND('',#22722,.T.) ;
#18427=FACE_OUTER_BOUND('',#22723,.T.) ;
#18428=FACE_OUTER_BOUND('',#22724,.T.) ;
#18429=FACE_OUTER_BOUND('',#22725,.T.) ;
#18430=FACE_OUTER_BOUND('',#22726,.T.) ;
#18431=FACE_OUTER_BOUND('',#22727,.T.) ;
#18432=FACE_OUTER_BOUND('',#22728,.T.) ;
#18433=FACE_OUTER_BOUND('',#22729,.T.) ;
#18434=FACE_OUTER_BOUND('',#22730,.T.) ;
#18435=FACE_OUTER_BOUND('',#22731,.T.) ;
#18436=FACE_OUTER_BOUND('',#22732,.T.) ;
#18437=FACE_OUTER_BOUND('',#22733,.T.) ;
#18438=FACE_OUTER_BOUND('',#22734,.T.) ;
#18439=FACE_OUTER_BOUND('',#22735,.T.) ;
#18440=FACE_OUTER_BOUND('',#22736,.T.) ;
#18441=FACE_OUTER_BOUND('',#22737,.T.) ;
#18442=FACE_OUTER_BOUND('',#22738,.T.) ;
#18443=FACE_OUTER_BOUND('',#22739,.T.) ;
#18444=FACE_OUTER_BOUND('',#22740,.T.) ;
#18445=FACE_OUTER_BOUND('',#22741,.T.) ;
#18446=FACE_OUTER_BOUND('',#22742,.T.) ;
#18447=FACE_OUTER_BOUND('',#22743,.T.) ;
#18448=FACE_OUTER_BOUND('',#22744,.T.) ;
#18449=FACE_OUTER_BOUND('',#22745,.T.) ;
#18450=FACE_OUTER_BOUND('',#22746,.T.) ;
#18451=FACE_OUTER_BOUND('',#22747,.T.) ;
#18452=FACE_OUTER_BOUND('',#22748,.T.) ;
#18453=FACE_OUTER_BOUND('',#22749,.T.) ;
#18454=FACE_OUTER_BOUND('',#22750,.T.) ;
#18455=FACE_OUTER_BOUND('',#22751,.T.) ;
#18456=FACE_OUTER_BOUND('',#22752,.T.) ;
#18457=FACE_OUTER_BOUND('',#22753,.T.) ;
#18458=FACE_OUTER_BOUND('',#22754,.T.) ;
#18459=FACE_OUTER_BOUND('',#22755,.T.) ;
#18460=FACE_OUTER_BOUND('',#22756,.T.) ;
#18461=FACE_OUTER_BOUND('',#22757,.T.) ;
#18462=FACE_OUTER_BOUND('',#22758,.T.) ;
#18463=FACE_OUTER_BOUND('',#22759,.T.) ;
#18464=FACE_OUTER_BOUND('',#22760,.T.) ;
#18465=FACE_OUTER_BOUND('',#22761,.T.) ;
#18466=FACE_OUTER_BOUND('',#22762,.T.) ;
#18467=FACE_OUTER_BOUND('',#22763,.T.) ;
#18468=FACE_OUTER_BOUND('',#22764,.T.) ;
#18469=FACE_OUTER_BOUND('',#22765,.T.) ;
#18470=FACE_OUTER_BOUND('',#22766,.T.) ;
#18471=FACE_OUTER_BOUND('',#22767,.T.) ;
#18472=FACE_OUTER_BOUND('',#22768,.T.) ;
#18473=FACE_OUTER_BOUND('',#22769,.T.) ;
#18474=FACE_OUTER_BOUND('',#22770,.T.) ;
#18475=FACE_OUTER_BOUND('',#22771,.T.) ;
#18476=FACE_OUTER_BOUND('',#22772,.T.) ;
#18477=FACE_OUTER_BOUND('',#22773,.T.) ;
#18478=FACE_OUTER_BOUND('',#22774,.T.) ;
#18479=FACE_OUTER_BOUND('',#22775,.T.) ;
#18480=FACE_OUTER_BOUND('',#22776,.T.) ;
#18481=FACE_OUTER_BOUND('',#22777,.T.) ;
#18482=FACE_OUTER_BOUND('',#22778,.T.) ;
#18483=FACE_OUTER_BOUND('',#22779,.T.) ;
#18484=FACE_OUTER_BOUND('',#22780,.T.) ;
#18485=FACE_OUTER_BOUND('',#22781,.T.) ;
#18486=FACE_OUTER_BOUND('',#22782,.T.) ;
#18487=FACE_OUTER_BOUND('',#22783,.T.) ;
#18488=FACE_OUTER_BOUND('',#22784,.T.) ;
#18489=FACE_OUTER_BOUND('',#22785,.T.) ;
#18490=FACE_OUTER_BOUND('',#22786,.T.) ;
#18491=FACE_OUTER_BOUND('',#22787,.T.) ;
#18492=FACE_OUTER_BOUND('',#22788,.T.) ;
#18493=FACE_OUTER_BOUND('',#22789,.T.) ;
#18494=FACE_OUTER_BOUND('',#22790,.T.) ;
#18495=FACE_OUTER_BOUND('',#22791,.T.) ;
#18496=FACE_OUTER_BOUND('',#22792,.T.) ;
#18497=FACE_OUTER_BOUND('',#22793,.T.) ;
#18498=FACE_OUTER_BOUND('',#22794,.T.) ;
#18499=FACE_OUTER_BOUND('',#22795,.T.) ;
#18500=FACE_OUTER_BOUND('',#22796,.T.) ;
#18501=FACE_OUTER_BOUND('',#22797,.T.) ;
#18502=FACE_OUTER_BOUND('',#22798,.T.) ;
#18503=FACE_OUTER_BOUND('',#22799,.T.) ;
#18504=FACE_OUTER_BOUND('',#22800,.T.) ;
#18505=FACE_OUTER_BOUND('',#22801,.T.) ;
#18506=FACE_OUTER_BOUND('',#22802,.T.) ;
#18507=FACE_OUTER_BOUND('',#22803,.T.) ;
#18508=FACE_OUTER_BOUND('',#22804,.T.) ;
#18509=FACE_OUTER_BOUND('',#22805,.T.) ;
#18510=FACE_OUTER_BOUND('',#22806,.T.) ;
#18511=FACE_OUTER_BOUND('',#22807,.T.) ;
#18512=FACE_OUTER_BOUND('',#22808,.T.) ;
#18513=FACE_OUTER_BOUND('',#22809,.T.) ;
#18514=FACE_OUTER_BOUND('',#22810,.T.) ;
#18515=FACE_OUTER_BOUND('',#22811,.T.) ;
#18516=FACE_OUTER_BOUND('',#22812,.T.) ;
#18517=FACE_OUTER_BOUND('',#22813,.T.) ;
#18518=FACE_OUTER_BOUND('',#22814,.T.) ;
#18519=FACE_OUTER_BOUND('',#22815,.T.) ;
#18520=FACE_OUTER_BOUND('',#22816,.T.) ;
#18521=FACE_OUTER_BOUND('',#22817,.T.) ;
#18522=FACE_OUTER_BOUND('',#22818,.T.) ;
#18523=FACE_OUTER_BOUND('',#22819,.T.) ;
#18524=FACE_OUTER_BOUND('',#22820,.T.) ;
#18525=FACE_OUTER_BOUND('',#22821,.T.) ;
#18526=FACE_OUTER_BOUND('',#22823,.T.) ;
#18527=FACE_OUTER_BOUND('',#22824,.T.) ;
#18528=FACE_OUTER_BOUND('',#22825,.T.) ;
#18529=FACE_OUTER_BOUND('',#22826,.T.) ;
#18530=FACE_OUTER_BOUND('',#22827,.T.) ;
#18531=FACE_OUTER_BOUND('',#22828,.T.) ;
#18532=FACE_OUTER_BOUND('',#22829,.T.) ;
#18533=FACE_OUTER_BOUND('',#22830,.T.) ;
#18534=FACE_OUTER_BOUND('',#22831,.T.) ;
#18535=FACE_OUTER_BOUND('',#22832,.T.) ;
#18536=FACE_OUTER_BOUND('',#22833,.T.) ;
#18537=FACE_OUTER_BOUND('',#22834,.T.) ;
#18538=FACE_OUTER_BOUND('',#22835,.T.) ;
#18539=FACE_OUTER_BOUND('',#22836,.T.) ;
#18540=FACE_OUTER_BOUND('',#22837,.T.) ;
#18541=FACE_OUTER_BOUND('',#22838,.T.) ;
#18542=FACE_OUTER_BOUND('',#22839,.T.) ;
#18543=FACE_OUTER_BOUND('',#22840,.T.) ;
#18544=FACE_OUTER_BOUND('',#22841,.T.) ;
#18545=FACE_OUTER_BOUND('',#22842,.T.) ;
#18546=FACE_OUTER_BOUND('',#22843,.T.) ;
#18547=FACE_OUTER_BOUND('',#22844,.T.) ;
#18548=FACE_OUTER_BOUND('',#22845,.T.) ;
#18549=FACE_OUTER_BOUND('',#22846,.T.) ;
#18550=FACE_OUTER_BOUND('',#22847,.T.) ;
#18551=FACE_OUTER_BOUND('',#22848,.T.) ;
#18552=FACE_OUTER_BOUND('',#22849,.T.) ;
#18553=FACE_OUTER_BOUND('',#22850,.T.) ;
#18554=FACE_OUTER_BOUND('',#22852,.T.) ;
#18555=FACE_OUTER_BOUND('',#22853,.T.) ;
#18556=FACE_OUTER_BOUND('',#22854,.T.) ;
#18557=FACE_OUTER_BOUND('',#22855,.T.) ;
#18558=FACE_OUTER_BOUND('',#22856,.T.) ;
#18559=FACE_OUTER_BOUND('',#22857,.T.) ;
#18560=FACE_OUTER_BOUND('',#22858,.T.) ;
#18561=FACE_OUTER_BOUND('',#22859,.T.) ;
#18562=FACE_OUTER_BOUND('',#22860,.T.) ;
#18563=FACE_OUTER_BOUND('',#22861,.T.) ;
#18564=FACE_OUTER_BOUND('',#22862,.T.) ;
#18565=FACE_OUTER_BOUND('',#22863,.T.) ;
#18566=FACE_OUTER_BOUND('',#22864,.T.) ;
#18567=FACE_OUTER_BOUND('',#22865,.T.) ;
#18568=FACE_OUTER_BOUND('',#22866,.T.) ;
#18569=FACE_OUTER_BOUND('',#22867,.T.) ;
#18570=FACE_OUTER_BOUND('',#22868,.T.) ;
#18571=FACE_OUTER_BOUND('',#22869,.T.) ;
#18572=FACE_OUTER_BOUND('',#22870,.T.) ;
#18573=FACE_OUTER_BOUND('',#22871,.T.) ;
#18574=FACE_OUTER_BOUND('',#22872,.T.) ;
#18575=FACE_OUTER_BOUND('',#22873,.T.) ;
#18576=FACE_OUTER_BOUND('',#22874,.T.) ;
#18577=FACE_OUTER_BOUND('',#22875,.T.) ;
#18578=FACE_OUTER_BOUND('',#22876,.T.) ;
#18579=FACE_OUTER_BOUND('',#22877,.T.) ;
#18580=FACE_OUTER_BOUND('',#22878,.T.) ;
#18581=FACE_OUTER_BOUND('',#22879,.T.) ;
#18582=FACE_OUTER_BOUND('',#22881,.T.) ;
#18583=FACE_OUTER_BOUND('',#22882,.T.) ;
#18584=FACE_OUTER_BOUND('',#22883,.T.) ;
#18585=FACE_OUTER_BOUND('',#22884,.T.) ;
#18586=FACE_OUTER_BOUND('',#22885,.T.) ;
#18587=FACE_OUTER_BOUND('',#22886,.T.) ;
#18588=FACE_OUTER_BOUND('',#22887,.T.) ;
#18589=FACE_OUTER_BOUND('',#22888,.T.) ;
#18590=FACE_OUTER_BOUND('',#22889,.T.) ;
#18591=FACE_OUTER_BOUND('',#22890,.T.) ;
#18592=FACE_OUTER_BOUND('',#22891,.T.) ;
#18593=FACE_OUTER_BOUND('',#22892,.T.) ;
#18594=FACE_OUTER_BOUND('',#22893,.T.) ;
#18595=FACE_OUTER_BOUND('',#22894,.T.) ;
#18596=FACE_OUTER_BOUND('',#22895,.T.) ;
#18597=FACE_OUTER_BOUND('',#22896,.T.) ;
#18598=FACE_OUTER_BOUND('',#22897,.T.) ;
#18599=FACE_OUTER_BOUND('',#22898,.T.) ;
#18600=FACE_OUTER_BOUND('',#22899,.T.) ;
#18601=FACE_OUTER_BOUND('',#22900,.T.) ;
#18602=FACE_OUTER_BOUND('',#22901,.T.) ;
#18603=FACE_OUTER_BOUND('',#22902,.T.) ;
#18604=FACE_OUTER_BOUND('',#22903,.T.) ;
#18605=FACE_OUTER_BOUND('',#22904,.T.) ;
#18606=FACE_OUTER_BOUND('',#22905,.T.) ;
#18607=FACE_OUTER_BOUND('',#22906,.T.) ;
#18608=FACE_OUTER_BOUND('',#22907,.T.) ;
#18609=FACE_OUTER_BOUND('',#22908,.T.) ;
#18610=FACE_OUTER_BOUND('',#22910,.T.) ;
#18611=FACE_OUTER_BOUND('',#22911,.T.) ;
#18612=FACE_OUTER_BOUND('',#22912,.T.) ;
#18613=FACE_OUTER_BOUND('',#22913,.T.) ;
#18614=FACE_OUTER_BOUND('',#22914,.T.) ;
#18615=FACE_OUTER_BOUND('',#22915,.T.) ;
#18616=FACE_OUTER_BOUND('',#22916,.T.) ;
#18617=FACE_OUTER_BOUND('',#22917,.T.) ;
#18618=FACE_OUTER_BOUND('',#22918,.T.) ;
#18619=FACE_OUTER_BOUND('',#22919,.T.) ;
#18620=FACE_OUTER_BOUND('',#22920,.T.) ;
#18621=FACE_OUTER_BOUND('',#22921,.T.) ;
#18622=FACE_OUTER_BOUND('',#22922,.T.) ;
#18623=FACE_OUTER_BOUND('',#22923,.T.) ;
#18624=FACE_OUTER_BOUND('',#22924,.T.) ;
#18625=FACE_OUTER_BOUND('',#22925,.T.) ;
#18626=FACE_OUTER_BOUND('',#22926,.T.) ;
#18627=FACE_OUTER_BOUND('',#22927,.T.) ;
#18628=FACE_OUTER_BOUND('',#22928,.T.) ;
#18629=FACE_OUTER_BOUND('',#22929,.T.) ;
#18630=FACE_OUTER_BOUND('',#22930,.T.) ;
#18631=FACE_OUTER_BOUND('',#22931,.T.) ;
#18632=FACE_OUTER_BOUND('',#22932,.T.) ;
#18633=FACE_OUTER_BOUND('',#22933,.T.) ;
#18634=FACE_OUTER_BOUND('',#22934,.T.) ;
#18635=FACE_OUTER_BOUND('',#22935,.T.) ;
#18636=FACE_OUTER_BOUND('',#22936,.T.) ;
#18637=FACE_OUTER_BOUND('',#22937,.T.) ;
#18638=FACE_OUTER_BOUND('',#22939,.T.) ;
#18639=FACE_OUTER_BOUND('',#22940,.T.) ;
#18640=FACE_OUTER_BOUND('',#22941,.T.) ;
#18641=FACE_OUTER_BOUND('',#22942,.T.) ;
#18642=FACE_OUTER_BOUND('',#22943,.T.) ;
#18643=FACE_OUTER_BOUND('',#22944,.T.) ;
#18644=FACE_OUTER_BOUND('',#22945,.T.) ;
#18645=FACE_OUTER_BOUND('',#22946,.T.) ;
#18646=FACE_OUTER_BOUND('',#22947,.T.) ;
#18647=FACE_OUTER_BOUND('',#22948,.T.) ;
#18648=FACE_OUTER_BOUND('',#22949,.T.) ;
#18649=FACE_OUTER_BOUND('',#22950,.T.) ;
#18650=FACE_OUTER_BOUND('',#22951,.T.) ;
#18651=FACE_OUTER_BOUND('',#22952,.T.) ;
#18652=FACE_OUTER_BOUND('',#22953,.T.) ;
#18653=FACE_OUTER_BOUND('',#22954,.T.) ;
#18654=FACE_OUTER_BOUND('',#22955,.T.) ;
#18655=FACE_OUTER_BOUND('',#22956,.T.) ;
#18656=FACE_OUTER_BOUND('',#22957,.T.) ;
#18657=FACE_OUTER_BOUND('',#22958,.T.) ;
#18658=FACE_OUTER_BOUND('',#22959,.T.) ;
#18659=FACE_OUTER_BOUND('',#22960,.T.) ;
#18660=FACE_OUTER_BOUND('',#22961,.T.) ;
#18661=FACE_OUTER_BOUND('',#22962,.T.) ;
#18662=FACE_OUTER_BOUND('',#22963,.T.) ;
#18663=FACE_OUTER_BOUND('',#22964,.T.) ;
#18664=FACE_OUTER_BOUND('',#22965,.T.) ;
#18665=FACE_OUTER_BOUND('',#22966,.T.) ;
#18666=FACE_OUTER_BOUND('',#22968,.T.) ;
#18667=FACE_OUTER_BOUND('',#22969,.T.) ;
#18668=FACE_OUTER_BOUND('',#22970,.T.) ;
#18669=FACE_OUTER_BOUND('',#22971,.T.) ;
#18670=FACE_OUTER_BOUND('',#22972,.T.) ;
#18671=FACE_OUTER_BOUND('',#22973,.T.) ;
#18672=FACE_OUTER_BOUND('',#22974,.T.) ;
#18673=FACE_OUTER_BOUND('',#22975,.T.) ;
#18674=FACE_OUTER_BOUND('',#22976,.T.) ;
#18675=FACE_OUTER_BOUND('',#22977,.T.) ;
#18676=FACE_OUTER_BOUND('',#22978,.T.) ;
#18677=FACE_OUTER_BOUND('',#22979,.T.) ;
#18678=FACE_OUTER_BOUND('',#22980,.T.) ;
#18679=FACE_OUTER_BOUND('',#22981,.T.) ;
#18680=FACE_OUTER_BOUND('',#22982,.T.) ;
#18681=FACE_OUTER_BOUND('',#22983,.T.) ;
#18682=FACE_OUTER_BOUND('',#22984,.T.) ;
#18683=FACE_OUTER_BOUND('',#22985,.T.) ;
#18684=FACE_OUTER_BOUND('',#22986,.T.) ;
#18685=FACE_OUTER_BOUND('',#22987,.T.) ;
#18686=FACE_OUTER_BOUND('',#22988,.T.) ;
#18687=FACE_OUTER_BOUND('',#22989,.T.) ;
#18688=FACE_OUTER_BOUND('',#22990,.T.) ;
#18689=FACE_OUTER_BOUND('',#22991,.T.) ;
#18690=FACE_OUTER_BOUND('',#22992,.T.) ;
#18691=FACE_OUTER_BOUND('',#22993,.T.) ;
#18692=FACE_OUTER_BOUND('',#22994,.T.) ;
#18693=FACE_OUTER_BOUND('',#22995,.T.) ;
#18694=FACE_OUTER_BOUND('',#22997,.T.) ;
#18695=FACE_OUTER_BOUND('',#22998,.T.) ;
#18696=FACE_OUTER_BOUND('',#22999,.T.) ;
#18697=FACE_OUTER_BOUND('',#23000,.T.) ;
#18698=FACE_OUTER_BOUND('',#23001,.T.) ;
#18699=FACE_OUTER_BOUND('',#23002,.T.) ;
#18700=FACE_OUTER_BOUND('',#23003,.T.) ;
#18701=FACE_OUTER_BOUND('',#23004,.T.) ;
#18702=FACE_OUTER_BOUND('',#23005,.T.) ;
#18703=FACE_OUTER_BOUND('',#23006,.T.) ;
#18704=FACE_OUTER_BOUND('',#23007,.T.) ;
#18705=FACE_OUTER_BOUND('',#23008,.T.) ;
#18706=FACE_OUTER_BOUND('',#23009,.T.) ;
#18707=FACE_OUTER_BOUND('',#23010,.T.) ;
#18708=FACE_OUTER_BOUND('',#23011,.T.) ;
#18709=FACE_OUTER_BOUND('',#23012,.T.) ;
#18710=FACE_OUTER_BOUND('',#23013,.T.) ;
#18711=FACE_OUTER_BOUND('',#23014,.T.) ;
#18712=FACE_OUTER_BOUND('',#23015,.T.) ;
#18713=FACE_OUTER_BOUND('',#23016,.T.) ;
#18714=FACE_OUTER_BOUND('',#23017,.T.) ;
#18715=FACE_OUTER_BOUND('',#23018,.T.) ;
#18716=FACE_OUTER_BOUND('',#23019,.T.) ;
#18717=FACE_OUTER_BOUND('',#23020,.T.) ;
#18718=FACE_OUTER_BOUND('',#23021,.T.) ;
#18719=FACE_OUTER_BOUND('',#23022,.T.) ;
#18720=FACE_OUTER_BOUND('',#23023,.T.) ;
#18721=FACE_OUTER_BOUND('',#23024,.T.) ;
#18722=FACE_OUTER_BOUND('',#23026,.T.) ;
#18723=FACE_OUTER_BOUND('',#23027,.T.) ;
#18724=FACE_OUTER_BOUND('',#23028,.T.) ;
#18725=FACE_OUTER_BOUND('',#23029,.T.) ;
#18726=FACE_OUTER_BOUND('',#23030,.T.) ;
#18727=FACE_OUTER_BOUND('',#23031,.T.) ;
#18728=FACE_OUTER_BOUND('',#23032,.T.) ;
#18729=FACE_OUTER_BOUND('',#23033,.T.) ;
#18730=FACE_OUTER_BOUND('',#23034,.T.) ;
#18731=FACE_OUTER_BOUND('',#23035,.T.) ;
#18732=FACE_OUTER_BOUND('',#23036,.T.) ;
#18733=FACE_OUTER_BOUND('',#23037,.T.) ;
#18734=FACE_OUTER_BOUND('',#23038,.T.) ;
#18735=FACE_OUTER_BOUND('',#23039,.T.) ;
#18736=FACE_OUTER_BOUND('',#23040,.T.) ;
#18737=FACE_OUTER_BOUND('',#23041,.T.) ;
#18738=FACE_OUTER_BOUND('',#23042,.T.) ;
#18739=FACE_OUTER_BOUND('',#23043,.T.) ;
#18740=FACE_OUTER_BOUND('',#23044,.T.) ;
#18741=FACE_OUTER_BOUND('',#23045,.T.) ;
#18742=FACE_OUTER_BOUND('',#23046,.T.) ;
#18743=FACE_OUTER_BOUND('',#23047,.T.) ;
#18744=FACE_OUTER_BOUND('',#23048,.T.) ;
#18745=FACE_OUTER_BOUND('',#23049,.T.) ;
#18746=FACE_OUTER_BOUND('',#23050,.T.) ;
#18747=FACE_OUTER_BOUND('',#23051,.T.) ;
#18748=FACE_OUTER_BOUND('',#23052,.T.) ;
#18749=FACE_OUTER_BOUND('',#23053,.T.) ;
#18750=FACE_OUTER_BOUND('',#23055,.T.) ;
#18751=FACE_OUTER_BOUND('',#23057,.T.) ;
#18752=FACE_OUTER_BOUND('',#23059,.T.) ;
#18753=FACE_OUTER_BOUND('',#23061,.T.) ;
#18754=FACE_OUTER_BOUND('',#23063,.T.) ;
#18755=FACE_OUTER_BOUND('',#23065,.T.) ;
#18756=FACE_OUTER_BOUND('',#23067,.T.) ;
#18757=FACE_OUTER_BOUND('',#23069,.T.) ;
#18758=FACE_OUTER_BOUND('',#23071,.T.) ;
#18759=FACE_OUTER_BOUND('',#23073,.T.) ;
#18760=FACE_OUTER_BOUND('',#23074,.T.) ;
#18761=FACE_OUTER_BOUND('',#23075,.T.) ;
#18762=FACE_OUTER_BOUND('',#23076,.T.) ;
#18763=FACE_OUTER_BOUND('',#23077,.T.) ;
#18764=FACE_OUTER_BOUND('',#23078,.T.) ;
#18765=FACE_OUTER_BOUND('',#23079,.T.) ;
#18766=FACE_OUTER_BOUND('',#23080,.T.) ;
#18767=FACE_OUTER_BOUND('',#23081,.T.) ;
#18768=FACE_OUTER_BOUND('',#23082,.T.) ;
#18769=FACE_OUTER_BOUND('',#23083,.T.) ;
#18770=FACE_OUTER_BOUND('',#23084,.T.) ;
#18771=FACE_OUTER_BOUND('',#23085,.T.) ;
#18772=FACE_OUTER_BOUND('',#23086,.T.) ;
#18773=FACE_OUTER_BOUND('',#23087,.T.) ;
#18774=FACE_OUTER_BOUND('',#23088,.T.) ;
#18775=FACE_OUTER_BOUND('',#23089,.T.) ;
#18776=FACE_OUTER_BOUND('',#23090,.T.) ;
#18777=FACE_OUTER_BOUND('',#23091,.T.) ;
#18778=FACE_OUTER_BOUND('',#23092,.T.) ;
#18779=FACE_OUTER_BOUND('',#23093,.T.) ;
#18780=FACE_OUTER_BOUND('',#23094,.T.) ;
#18781=FACE_OUTER_BOUND('',#23095,.T.) ;
#18782=FACE_OUTER_BOUND('',#23096,.T.) ;
#18783=FACE_OUTER_BOUND('',#23097,.T.) ;
#18784=FACE_OUTER_BOUND('',#23098,.T.) ;
#18785=FACE_OUTER_BOUND('',#23099,.T.) ;
#18786=FACE_OUTER_BOUND('',#23100,.T.) ;
#18787=FACE_OUTER_BOUND('',#23101,.T.) ;
#18788=FACE_OUTER_BOUND('',#23102,.T.) ;
#18789=FACE_OUTER_BOUND('',#23103,.T.) ;
#18790=FACE_OUTER_BOUND('',#23104,.T.) ;
#18791=FACE_OUTER_BOUND('',#23105,.T.) ;
#18792=FACE_OUTER_BOUND('',#23106,.T.) ;
#18793=FACE_OUTER_BOUND('',#23107,.T.) ;
#18794=FACE_OUTER_BOUND('',#23108,.T.) ;
#18795=FACE_OUTER_BOUND('',#23109,.T.) ;
#18796=FACE_OUTER_BOUND('',#23110,.T.) ;
#18797=FACE_OUTER_BOUND('',#23111,.T.) ;
#18798=FACE_OUTER_BOUND('',#23112,.T.) ;
#18799=FACE_OUTER_BOUND('',#23113,.T.) ;
#18800=FACE_OUTER_BOUND('',#23114,.T.) ;
#18801=FACE_OUTER_BOUND('',#23115,.T.) ;
#18802=FACE_OUTER_BOUND('',#23116,.T.) ;
#18803=FACE_OUTER_BOUND('',#23117,.T.) ;
#18804=FACE_OUTER_BOUND('',#23118,.T.) ;
#18805=FACE_OUTER_BOUND('',#23119,.T.) ;
#18806=FACE_OUTER_BOUND('',#23120,.T.) ;
#18807=FACE_OUTER_BOUND('',#23121,.T.) ;
#18808=FACE_OUTER_BOUND('',#23122,.T.) ;
#18809=FACE_OUTER_BOUND('',#23123,.T.) ;
#18810=FACE_OUTER_BOUND('',#23124,.T.) ;
#18811=FACE_OUTER_BOUND('',#23125,.T.) ;
#18812=FACE_OUTER_BOUND('',#23126,.T.) ;
#18813=FACE_OUTER_BOUND('',#23127,.T.) ;
#18814=FACE_OUTER_BOUND('',#23128,.T.) ;
#18815=FACE_OUTER_BOUND('',#23129,.T.) ;
#18816=FACE_OUTER_BOUND('',#23130,.T.) ;
#18817=FACE_OUTER_BOUND('',#23131,.T.) ;
#18818=FACE_OUTER_BOUND('',#23132,.T.) ;
#18819=FACE_OUTER_BOUND('',#23133,.T.) ;
#18820=FACE_OUTER_BOUND('',#23134,.T.) ;
#18821=FACE_OUTER_BOUND('',#23135,.T.) ;
#18822=FACE_OUTER_BOUND('',#23136,.T.) ;
#18823=FACE_OUTER_BOUND('',#23137,.T.) ;
#18824=FACE_OUTER_BOUND('',#23138,.T.) ;
#18825=FACE_OUTER_BOUND('',#23139,.T.) ;
#18826=FACE_OUTER_BOUND('',#23140,.T.) ;
#18827=FACE_OUTER_BOUND('',#23141,.T.) ;
#18828=FACE_OUTER_BOUND('',#23142,.T.) ;
#18829=FACE_OUTER_BOUND('',#23143,.T.) ;
#18830=FACE_OUTER_BOUND('',#23144,.T.) ;
#18831=FACE_OUTER_BOUND('',#23145,.T.) ;
#18832=FACE_OUTER_BOUND('',#23146,.T.) ;
#18833=FACE_OUTER_BOUND('',#23147,.T.) ;
#18834=FACE_OUTER_BOUND('',#23148,.T.) ;
#18835=FACE_OUTER_BOUND('',#23149,.T.) ;
#18836=FACE_OUTER_BOUND('',#23150,.T.) ;
#18837=FACE_OUTER_BOUND('',#23151,.T.) ;
#18838=FACE_OUTER_BOUND('',#23152,.T.) ;
#18839=FACE_OUTER_BOUND('',#23153,.T.) ;
#18840=FACE_OUTER_BOUND('',#23154,.T.) ;
#18841=FACE_OUTER_BOUND('',#23155,.T.) ;
#18842=FACE_OUTER_BOUND('',#23156,.T.) ;
#18843=FACE_OUTER_BOUND('',#23157,.T.) ;
#18844=FACE_OUTER_BOUND('',#23158,.T.) ;
#18845=FACE_OUTER_BOUND('',#23159,.T.) ;
#18846=FACE_OUTER_BOUND('',#23160,.T.) ;
#18847=FACE_OUTER_BOUND('',#23161,.T.) ;
#18848=FACE_OUTER_BOUND('',#23162,.T.) ;
#18849=FACE_OUTER_BOUND('',#23163,.T.) ;
#18850=FACE_OUTER_BOUND('',#23164,.T.) ;
#18851=FACE_OUTER_BOUND('',#23165,.T.) ;
#18852=FACE_OUTER_BOUND('',#23166,.T.) ;
#18853=FACE_OUTER_BOUND('',#23167,.T.) ;
#18854=FACE_OUTER_BOUND('',#23168,.T.) ;
#18855=FACE_OUTER_BOUND('',#23169,.T.) ;
#18856=FACE_OUTER_BOUND('',#23170,.T.) ;
#18857=FACE_OUTER_BOUND('',#23171,.T.) ;
#18858=FACE_OUTER_BOUND('',#23172,.T.) ;
#18859=FACE_OUTER_BOUND('',#23173,.T.) ;
#18860=FACE_OUTER_BOUND('',#23174,.T.) ;
#18861=FACE_OUTER_BOUND('',#23175,.T.) ;
#18862=FACE_OUTER_BOUND('',#23176,.T.) ;
#18863=FACE_OUTER_BOUND('',#23177,.T.) ;
#18864=FACE_OUTER_BOUND('',#23178,.T.) ;
#18865=FACE_OUTER_BOUND('',#23179,.T.) ;
#18866=FACE_OUTER_BOUND('',#23180,.T.) ;
#18867=FACE_OUTER_BOUND('',#23181,.T.) ;
#18868=FACE_OUTER_BOUND('',#23182,.T.) ;
#18869=FACE_OUTER_BOUND('',#23183,.T.) ;
#18870=FACE_OUTER_BOUND('',#23184,.T.) ;
#18871=FACE_OUTER_BOUND('',#23185,.T.) ;
#18872=FACE_OUTER_BOUND('',#23186,.T.) ;
#18873=FACE_OUTER_BOUND('',#23187,.T.) ;
#18874=FACE_OUTER_BOUND('',#23188,.T.) ;
#18875=FACE_OUTER_BOUND('',#23189,.T.) ;
#18876=FACE_OUTER_BOUND('',#23190,.T.) ;
#18877=FACE_OUTER_BOUND('',#23191,.T.) ;
#18878=FACE_OUTER_BOUND('',#23192,.T.) ;
#18879=FACE_OUTER_BOUND('',#23193,.T.) ;
#18880=FACE_OUTER_BOUND('',#23194,.T.) ;
#18881=FACE_OUTER_BOUND('',#23195,.T.) ;
#18882=FACE_OUTER_BOUND('',#23196,.T.) ;
#18883=FACE_OUTER_BOUND('',#23197,.T.) ;
#18884=FACE_OUTER_BOUND('',#23198,.T.) ;
#18885=FACE_OUTER_BOUND('',#23199,.T.) ;
#18886=FACE_OUTER_BOUND('',#23200,.T.) ;
#18887=FACE_OUTER_BOUND('',#23201,.T.) ;
#18888=FACE_OUTER_BOUND('',#23202,.T.) ;
#18889=FACE_OUTER_BOUND('',#23203,.T.) ;
#18890=FACE_OUTER_BOUND('',#23204,.T.) ;
#18891=FACE_OUTER_BOUND('',#23205,.T.) ;
#18892=FACE_OUTER_BOUND('',#23206,.T.) ;
#18893=FACE_OUTER_BOUND('',#23207,.T.) ;
#18894=FACE_OUTER_BOUND('',#23208,.T.) ;
#18895=FACE_OUTER_BOUND('',#23209,.T.) ;
#18896=FACE_OUTER_BOUND('',#23210,.T.) ;
#18897=FACE_OUTER_BOUND('',#23211,.T.) ;
#18898=FACE_OUTER_BOUND('',#23212,.T.) ;
#18899=FACE_OUTER_BOUND('',#23213,.T.) ;
#18900=FACE_OUTER_BOUND('',#23214,.T.) ;
#18901=FACE_OUTER_BOUND('',#23215,.T.) ;
#18902=FACE_OUTER_BOUND('',#23216,.T.) ;
#18903=FACE_OUTER_BOUND('',#23217,.T.) ;
#18904=FACE_OUTER_BOUND('',#23218,.T.) ;
#18905=FACE_OUTER_BOUND('',#23219,.T.) ;
#18906=FACE_OUTER_BOUND('',#23220,.T.) ;
#18907=FACE_OUTER_BOUND('',#23221,.T.) ;
#18908=FACE_OUTER_BOUND('',#23222,.T.) ;
#18909=FACE_OUTER_BOUND('',#23223,.T.) ;
#18910=FACE_OUTER_BOUND('',#23224,.T.) ;
#18911=FACE_OUTER_BOUND('',#23225,.T.) ;
#18912=FACE_OUTER_BOUND('',#23226,.T.) ;
#18913=FACE_OUTER_BOUND('',#23227,.T.) ;
#18914=FACE_OUTER_BOUND('',#23228,.T.) ;
#18915=FACE_OUTER_BOUND('',#23229,.T.) ;
#18916=FACE_OUTER_BOUND('',#23230,.T.) ;
#18917=FACE_OUTER_BOUND('',#23231,.T.) ;
#18918=FACE_OUTER_BOUND('',#23232,.T.) ;
#18919=FACE_OUTER_BOUND('',#23233,.T.) ;
#18920=FACE_OUTER_BOUND('',#23234,.T.) ;
#18921=FACE_OUTER_BOUND('',#23235,.T.) ;
#18922=FACE_OUTER_BOUND('',#23236,.T.) ;
#18923=FACE_OUTER_BOUND('',#23237,.T.) ;
#18924=FACE_OUTER_BOUND('',#23238,.T.) ;
#18925=FACE_OUTER_BOUND('',#23239,.T.) ;
#18926=FACE_OUTER_BOUND('',#23240,.T.) ;
#18927=FACE_OUTER_BOUND('',#23241,.T.) ;
#18928=FACE_OUTER_BOUND('',#23242,.T.) ;
#18929=FACE_OUTER_BOUND('',#23243,.T.) ;
#18930=FACE_OUTER_BOUND('',#23244,.T.) ;
#18931=FACE_OUTER_BOUND('',#23245,.T.) ;
#18932=FACE_OUTER_BOUND('',#23246,.T.) ;
#18933=FACE_OUTER_BOUND('',#23247,.T.) ;
#18934=FACE_OUTER_BOUND('',#23248,.T.) ;
#18935=FACE_OUTER_BOUND('',#23249,.T.) ;
#18936=FACE_OUTER_BOUND('',#23250,.T.) ;
#18937=FACE_OUTER_BOUND('',#23251,.T.) ;
#18938=FACE_OUTER_BOUND('',#23252,.T.) ;
#18939=FACE_OUTER_BOUND('',#23253,.T.) ;
#18940=FACE_OUTER_BOUND('',#23254,.T.) ;
#18941=FACE_OUTER_BOUND('',#23255,.T.) ;
#18942=FACE_OUTER_BOUND('',#23256,.T.) ;
#18943=FACE_OUTER_BOUND('',#23257,.T.) ;
#18944=FACE_OUTER_BOUND('',#23258,.T.) ;
#18945=FACE_OUTER_BOUND('',#23259,.T.) ;
#18946=FACE_OUTER_BOUND('',#23260,.T.) ;
#18947=FACE_OUTER_BOUND('',#23261,.T.) ;
#18948=FACE_OUTER_BOUND('',#23262,.T.) ;
#18949=FACE_OUTER_BOUND('',#23263,.T.) ;
#18950=FACE_OUTER_BOUND('',#23264,.T.) ;
#18951=FACE_OUTER_BOUND('',#23265,.T.) ;
#18952=FACE_OUTER_BOUND('',#23266,.T.) ;
#18953=FACE_OUTER_BOUND('',#23267,.T.) ;
#18954=FACE_OUTER_BOUND('',#23268,.T.) ;
#18955=FACE_OUTER_BOUND('',#23269,.T.) ;
#18956=FACE_OUTER_BOUND('',#23270,.T.) ;
#18957=FACE_OUTER_BOUND('',#23271,.T.) ;
#18958=FACE_OUTER_BOUND('',#23272,.T.) ;
#18959=FACE_OUTER_BOUND('',#23273,.T.) ;
#18960=FACE_OUTER_BOUND('',#23274,.T.) ;
#18961=FACE_OUTER_BOUND('',#23275,.T.) ;
#18962=FACE_OUTER_BOUND('',#23276,.T.) ;
#18963=FACE_OUTER_BOUND('',#23277,.T.) ;
#18964=FACE_OUTER_BOUND('',#23278,.T.) ;
#18965=FACE_OUTER_BOUND('',#23279,.T.) ;
#18966=FACE_OUTER_BOUND('',#23280,.T.) ;
#18967=FACE_OUTER_BOUND('',#23281,.T.) ;
#18968=FACE_OUTER_BOUND('',#23282,.T.) ;
#18969=FACE_OUTER_BOUND('',#23283,.T.) ;
#18970=FACE_OUTER_BOUND('',#23284,.T.) ;
#18971=FACE_OUTER_BOUND('',#23285,.T.) ;
#18972=FACE_OUTER_BOUND('',#23286,.T.) ;
#18973=FACE_OUTER_BOUND('',#23287,.T.) ;
#18974=FACE_OUTER_BOUND('',#23288,.T.) ;
#18975=FACE_OUTER_BOUND('',#23289,.T.) ;
#18976=FACE_OUTER_BOUND('',#23290,.T.) ;
#18977=FACE_OUTER_BOUND('',#23291,.T.) ;
#18978=FACE_OUTER_BOUND('',#23292,.T.) ;
#18979=FACE_OUTER_BOUND('',#23293,.T.) ;
#18980=FACE_OUTER_BOUND('',#23294,.T.) ;
#18981=FACE_OUTER_BOUND('',#23295,.T.) ;
#18982=FACE_OUTER_BOUND('',#23296,.T.) ;
#18983=FACE_OUTER_BOUND('',#23297,.T.) ;
#18984=FACE_OUTER_BOUND('',#23298,.T.) ;
#18985=FACE_OUTER_BOUND('',#23299,.T.) ;
#18986=FACE_OUTER_BOUND('',#23300,.T.) ;
#18987=FACE_OUTER_BOUND('',#23301,.T.) ;
#18988=FACE_OUTER_BOUND('',#23302,.T.) ;
#18989=FACE_OUTER_BOUND('',#23303,.T.) ;
#18990=FACE_OUTER_BOUND('',#23304,.T.) ;
#18991=FACE_OUTER_BOUND('',#23305,.T.) ;
#18992=FACE_OUTER_BOUND('',#23306,.T.) ;
#18993=FACE_OUTER_BOUND('',#23307,.T.) ;
#18994=FACE_OUTER_BOUND('',#23308,.T.) ;
#18995=FACE_OUTER_BOUND('',#23309,.T.) ;
#18996=FACE_OUTER_BOUND('',#23310,.T.) ;
#18997=FACE_OUTER_BOUND('',#23311,.T.) ;
#18998=FACE_OUTER_BOUND('',#23312,.T.) ;
#18999=FACE_OUTER_BOUND('',#23313,.T.) ;
#19000=FACE_OUTER_BOUND('',#23314,.T.) ;
#19001=FACE_OUTER_BOUND('',#23315,.T.) ;
#19002=FACE_OUTER_BOUND('',#23316,.T.) ;
#19003=FACE_OUTER_BOUND('',#23317,.T.) ;
#19004=FACE_OUTER_BOUND('',#23318,.T.) ;
#19005=FACE_OUTER_BOUND('',#23319,.T.) ;
#19006=FACE_OUTER_BOUND('',#23320,.T.) ;
#19007=FACE_OUTER_BOUND('',#23321,.T.) ;
#19008=FACE_OUTER_BOUND('',#23322,.T.) ;
#19009=FACE_OUTER_BOUND('',#23323,.T.) ;
#19010=FACE_OUTER_BOUND('',#23324,.T.) ;
#19011=FACE_OUTER_BOUND('',#23325,.T.) ;
#19012=FACE_OUTER_BOUND('',#23326,.T.) ;
#19013=FACE_OUTER_BOUND('',#23327,.T.) ;
#19014=FACE_OUTER_BOUND('',#23328,.T.) ;
#19015=FACE_OUTER_BOUND('',#23329,.T.) ;
#19016=FACE_OUTER_BOUND('',#23330,.T.) ;
#19017=FACE_OUTER_BOUND('',#23331,.T.) ;
#19018=FACE_OUTER_BOUND('',#23332,.T.) ;
#19019=FACE_OUTER_BOUND('',#23333,.T.) ;
#19020=FACE_OUTER_BOUND('',#23334,.T.) ;
#19021=FACE_OUTER_BOUND('',#23335,.T.) ;
#19022=FACE_OUTER_BOUND('',#23336,.T.) ;
#19023=FACE_OUTER_BOUND('',#23337,.T.) ;
#19024=FACE_OUTER_BOUND('',#23338,.T.) ;
#19025=FACE_OUTER_BOUND('',#23339,.T.) ;
#19026=FACE_OUTER_BOUND('',#23340,.T.) ;
#19027=FACE_OUTER_BOUND('',#23341,.T.) ;
#19028=FACE_OUTER_BOUND('',#23342,.T.) ;
#19029=FACE_OUTER_BOUND('',#23343,.T.) ;
#19030=FACE_OUTER_BOUND('',#23344,.T.) ;
#19031=FACE_OUTER_BOUND('',#23345,.T.) ;
#19032=FACE_OUTER_BOUND('',#23346,.T.) ;
#19033=FACE_OUTER_BOUND('',#23347,.T.) ;
#19034=FACE_OUTER_BOUND('',#23348,.T.) ;
#19035=FACE_OUTER_BOUND('',#23349,.T.) ;
#19036=FACE_OUTER_BOUND('',#23350,.T.) ;
#19037=FACE_OUTER_BOUND('',#23351,.T.) ;
#19038=FACE_OUTER_BOUND('',#23352,.T.) ;
#19039=FACE_OUTER_BOUND('',#23353,.T.) ;
#19040=FACE_OUTER_BOUND('',#23354,.T.) ;
#19041=FACE_OUTER_BOUND('',#23355,.T.) ;
#19042=FACE_OUTER_BOUND('',#23356,.T.) ;
#19043=FACE_OUTER_BOUND('',#23357,.T.) ;
#19044=FACE_OUTER_BOUND('',#23358,.T.) ;
#19045=FACE_OUTER_BOUND('',#23359,.T.) ;
#19046=FACE_OUTER_BOUND('',#23360,.T.) ;
#19047=FACE_OUTER_BOUND('',#23361,.T.) ;
#19048=FACE_OUTER_BOUND('',#23362,.T.) ;
#19049=FACE_OUTER_BOUND('',#23363,.T.) ;
#19050=FACE_OUTER_BOUND('',#23364,.T.) ;
#19051=FACE_OUTER_BOUND('',#23365,.T.) ;
#19052=FACE_OUTER_BOUND('',#23366,.T.) ;
#19053=FACE_OUTER_BOUND('',#23367,.T.) ;
#19054=FACE_OUTER_BOUND('',#23368,.T.) ;
#19055=FACE_OUTER_BOUND('',#23369,.T.) ;
#19056=FACE_OUTER_BOUND('',#23370,.T.) ;
#19057=FACE_OUTER_BOUND('',#23371,.T.) ;
#19058=FACE_OUTER_BOUND('',#23372,.T.) ;
#19059=FACE_OUTER_BOUND('',#23373,.T.) ;
#19060=FACE_OUTER_BOUND('',#23374,.T.) ;
#19061=FACE_OUTER_BOUND('',#23375,.T.) ;
#19062=FACE_OUTER_BOUND('',#23376,.T.) ;
#19063=FACE_OUTER_BOUND('',#23377,.T.) ;
#19064=FACE_OUTER_BOUND('',#23378,.T.) ;
#19065=FACE_OUTER_BOUND('',#23379,.T.) ;
#19066=FACE_OUTER_BOUND('',#23380,.T.) ;
#19067=FACE_OUTER_BOUND('',#23381,.T.) ;
#19068=FACE_OUTER_BOUND('',#23382,.T.) ;
#19069=FACE_OUTER_BOUND('',#23383,.T.) ;
#19070=FACE_OUTER_BOUND('',#23384,.T.) ;
#19071=FACE_OUTER_BOUND('',#23385,.T.) ;
#19072=FACE_OUTER_BOUND('',#23386,.T.) ;
#19073=FACE_OUTER_BOUND('',#23387,.T.) ;
#19074=FACE_OUTER_BOUND('',#23388,.T.) ;
#19075=FACE_OUTER_BOUND('',#23389,.T.) ;
#19076=FACE_OUTER_BOUND('',#23390,.T.) ;
#19077=FACE_OUTER_BOUND('',#23391,.T.) ;
#19078=FACE_OUTER_BOUND('',#23392,.T.) ;
#19079=FACE_OUTER_BOUND('',#23393,.T.) ;
#19080=FACE_OUTER_BOUND('',#23394,.T.) ;
#19081=FACE_OUTER_BOUND('',#23395,.T.) ;
#19082=FACE_OUTER_BOUND('',#23396,.T.) ;
#19083=FACE_OUTER_BOUND('',#23397,.T.) ;
#19084=FACE_OUTER_BOUND('',#23398,.T.) ;
#19085=FACE_OUTER_BOUND('',#23399,.T.) ;
#19086=FACE_OUTER_BOUND('',#23400,.T.) ;
#19087=FACE_OUTER_BOUND('',#23401,.T.) ;
#19088=FACE_OUTER_BOUND('',#23402,.T.) ;
#19089=FACE_OUTER_BOUND('',#23403,.T.) ;
#19090=FACE_OUTER_BOUND('',#23404,.T.) ;
#19091=FACE_OUTER_BOUND('',#23405,.T.) ;
#19092=FACE_OUTER_BOUND('',#23406,.T.) ;
#19093=FACE_OUTER_BOUND('',#23407,.T.) ;
#19094=FACE_OUTER_BOUND('',#23408,.T.) ;
#19095=FACE_OUTER_BOUND('',#23409,.T.) ;
#19096=FACE_OUTER_BOUND('',#23410,.T.) ;
#19097=FACE_OUTER_BOUND('',#23411,.T.) ;
#19098=FACE_OUTER_BOUND('',#23412,.T.) ;
#19099=FACE_OUTER_BOUND('',#23413,.T.) ;
#19100=FACE_OUTER_BOUND('',#23414,.T.) ;
#19101=FACE_OUTER_BOUND('',#23415,.T.) ;
#19102=FACE_OUTER_BOUND('',#23416,.T.) ;
#19103=FACE_OUTER_BOUND('',#23417,.T.) ;
#19104=FACE_OUTER_BOUND('',#23418,.T.) ;
#19105=FACE_OUTER_BOUND('',#23419,.T.) ;
#19106=FACE_OUTER_BOUND('',#23420,.T.) ;
#19107=FACE_OUTER_BOUND('',#23421,.T.) ;
#19108=FACE_OUTER_BOUND('',#23422,.T.) ;
#19109=FACE_OUTER_BOUND('',#23423,.T.) ;
#19110=FACE_OUTER_BOUND('',#23424,.T.) ;
#19111=FACE_OUTER_BOUND('',#23425,.T.) ;
#19112=FACE_OUTER_BOUND('',#23426,.T.) ;
#19113=FACE_OUTER_BOUND('',#23427,.T.) ;
#19114=FACE_OUTER_BOUND('',#23428,.T.) ;
#19115=FACE_OUTER_BOUND('',#23429,.T.) ;
#19116=FACE_OUTER_BOUND('',#23430,.T.) ;
#19117=FACE_OUTER_BOUND('',#23431,.T.) ;
#19118=FACE_OUTER_BOUND('',#23432,.T.) ;
#19119=FACE_OUTER_BOUND('',#23433,.T.) ;
#19120=FACE_OUTER_BOUND('',#23434,.T.) ;
#19121=FACE_OUTER_BOUND('',#23435,.T.) ;
#19122=FACE_OUTER_BOUND('',#23436,.T.) ;
#19123=FACE_OUTER_BOUND('',#23437,.T.) ;
#19124=FACE_OUTER_BOUND('',#23438,.T.) ;
#19125=FACE_OUTER_BOUND('',#23439,.T.) ;
#19126=FACE_OUTER_BOUND('',#23440,.T.) ;
#19127=FACE_OUTER_BOUND('',#23441,.T.) ;
#19128=FACE_OUTER_BOUND('',#23442,.T.) ;
#19129=FACE_OUTER_BOUND('',#23443,.T.) ;
#19130=FACE_OUTER_BOUND('',#23444,.T.) ;
#19131=FACE_OUTER_BOUND('',#23445,.T.) ;
#19132=FACE_OUTER_BOUND('',#23446,.T.) ;
#19133=FACE_OUTER_BOUND('',#23447,.T.) ;
#19134=FACE_OUTER_BOUND('',#23448,.T.) ;
#19135=FACE_OUTER_BOUND('',#23449,.T.) ;
#19136=FACE_OUTER_BOUND('',#23450,.T.) ;
#19137=FACE_OUTER_BOUND('',#23451,.T.) ;
#19138=FACE_OUTER_BOUND('',#23452,.T.) ;
#19139=FACE_OUTER_BOUND('',#23453,.T.) ;
#19140=FACE_OUTER_BOUND('',#23454,.T.) ;
#19141=FACE_OUTER_BOUND('',#23455,.T.) ;
#19142=FACE_OUTER_BOUND('',#23456,.T.) ;
#19143=FACE_OUTER_BOUND('',#23457,.T.) ;
#19144=FACE_OUTER_BOUND('',#23458,.T.) ;
#19145=FACE_OUTER_BOUND('',#23459,.T.) ;
#19146=FACE_OUTER_BOUND('',#23460,.T.) ;
#19147=FACE_OUTER_BOUND('',#23461,.T.) ;
#19148=FACE_OUTER_BOUND('',#23462,.T.) ;
#19149=FACE_OUTER_BOUND('',#23463,.T.) ;
#19150=FACE_OUTER_BOUND('',#23464,.T.) ;
#19151=FACE_OUTER_BOUND('',#23465,.T.) ;
#19152=FACE_OUTER_BOUND('',#23466,.T.) ;
#19153=FACE_OUTER_BOUND('',#23467,.T.) ;
#19154=FACE_OUTER_BOUND('',#23468,.T.) ;
#19155=FACE_OUTER_BOUND('',#23469,.T.) ;
#19156=FACE_OUTER_BOUND('',#23470,.T.) ;
#19157=FACE_OUTER_BOUND('',#23471,.T.) ;
#19158=FACE_OUTER_BOUND('',#23472,.T.) ;
#19159=FACE_OUTER_BOUND('',#23473,.T.) ;
#19160=FACE_OUTER_BOUND('',#23474,.T.) ;
#19161=FACE_OUTER_BOUND('',#23475,.T.) ;
#19162=FACE_OUTER_BOUND('',#23476,.T.) ;
#19163=FACE_OUTER_BOUND('',#23477,.T.) ;
#19164=FACE_OUTER_BOUND('',#23478,.T.) ;
#19165=FACE_OUTER_BOUND('',#23479,.T.) ;
#19166=FACE_OUTER_BOUND('',#23480,.T.) ;
#19167=FACE_OUTER_BOUND('',#23481,.T.) ;
#19168=FACE_OUTER_BOUND('',#23482,.T.) ;
#19169=FACE_OUTER_BOUND('',#23483,.T.) ;
#19170=FACE_OUTER_BOUND('',#23484,.T.) ;
#19171=FACE_OUTER_BOUND('',#23485,.T.) ;
#19172=FACE_OUTER_BOUND('',#23486,.T.) ;
#19173=FACE_OUTER_BOUND('',#23487,.T.) ;
#19174=FACE_OUTER_BOUND('',#23488,.T.) ;
#19175=FACE_OUTER_BOUND('',#23489,.T.) ;
#19176=FACE_OUTER_BOUND('',#23490,.T.) ;
#19177=FACE_OUTER_BOUND('',#23491,.T.) ;
#19178=FACE_OUTER_BOUND('',#23492,.T.) ;
#19179=FACE_OUTER_BOUND('',#23493,.T.) ;
#19180=FACE_OUTER_BOUND('',#23494,.T.) ;
#19181=FACE_OUTER_BOUND('',#23495,.T.) ;
#19182=FACE_OUTER_BOUND('',#23496,.T.) ;
#19183=FACE_OUTER_BOUND('',#23497,.T.) ;
#19184=FACE_OUTER_BOUND('',#23498,.T.) ;
#19185=FACE_OUTER_BOUND('',#23499,.T.) ;
#19186=FACE_OUTER_BOUND('',#23500,.T.) ;
#19187=FACE_OUTER_BOUND('',#23501,.T.) ;
#19188=FACE_OUTER_BOUND('',#23502,.T.) ;
#19189=FACE_OUTER_BOUND('',#23503,.T.) ;
#19190=FACE_OUTER_BOUND('',#23504,.T.) ;
#19191=FACE_OUTER_BOUND('',#23505,.T.) ;
#19192=FACE_OUTER_BOUND('',#23506,.T.) ;
#19193=FACE_OUTER_BOUND('',#23507,.T.) ;
#19194=FACE_OUTER_BOUND('',#23508,.T.) ;
#19195=FACE_OUTER_BOUND('',#23509,.T.) ;
#19196=FACE_OUTER_BOUND('',#23510,.T.) ;
#19197=FACE_OUTER_BOUND('',#23511,.T.) ;
#19198=FACE_OUTER_BOUND('',#23512,.T.) ;
#19199=FACE_OUTER_BOUND('',#23513,.T.) ;
#19200=FACE_OUTER_BOUND('',#23514,.T.) ;
#19201=FACE_OUTER_BOUND('',#23515,.T.) ;
#19202=FACE_OUTER_BOUND('',#23516,.T.) ;
#19203=FACE_OUTER_BOUND('',#23517,.T.) ;
#19204=FACE_OUTER_BOUND('',#23518,.T.) ;
#19205=FACE_OUTER_BOUND('',#23519,.T.) ;
#19206=FACE_OUTER_BOUND('',#23520,.T.) ;
#19207=FACE_OUTER_BOUND('',#23521,.T.) ;
#19208=FACE_OUTER_BOUND('',#23522,.T.) ;
#19209=FACE_OUTER_BOUND('',#23523,.T.) ;
#19210=FACE_OUTER_BOUND('',#23524,.T.) ;
#19211=FACE_OUTER_BOUND('',#23525,.T.) ;
#19212=FACE_OUTER_BOUND('',#23526,.T.) ;
#19213=FACE_OUTER_BOUND('',#23527,.T.) ;
#19214=FACE_OUTER_BOUND('',#23528,.T.) ;
#19215=FACE_OUTER_BOUND('',#23529,.T.) ;
#19216=FACE_OUTER_BOUND('',#23530,.T.) ;
#19217=FACE_OUTER_BOUND('',#23531,.T.) ;
#19218=FACE_OUTER_BOUND('',#23532,.T.) ;
#19219=FACE_OUTER_BOUND('',#23533,.T.) ;
#19220=FACE_OUTER_BOUND('',#23534,.T.) ;
#19221=FACE_OUTER_BOUND('',#23535,.T.) ;
#19222=FACE_OUTER_BOUND('',#23536,.T.) ;
#19223=FACE_OUTER_BOUND('',#23537,.T.) ;
#19224=FACE_OUTER_BOUND('',#23538,.T.) ;
#19225=FACE_OUTER_BOUND('',#23539,.T.) ;
#19226=FACE_OUTER_BOUND('',#23540,.T.) ;
#19227=FACE_OUTER_BOUND('',#23541,.T.) ;
#19228=FACE_OUTER_BOUND('',#23542,.T.) ;
#19229=FACE_OUTER_BOUND('',#23543,.T.) ;
#19230=FACE_OUTER_BOUND('',#23544,.T.) ;
#19231=FACE_OUTER_BOUND('',#23545,.T.) ;
#19232=FACE_OUTER_BOUND('',#23546,.T.) ;
#19233=FACE_OUTER_BOUND('',#23547,.T.) ;
#19234=FACE_OUTER_BOUND('',#23548,.T.) ;
#19235=FACE_OUTER_BOUND('',#23549,.T.) ;
#19236=FACE_OUTER_BOUND('',#23550,.T.) ;
#19237=FACE_OUTER_BOUND('',#23551,.T.) ;
#19238=FACE_OUTER_BOUND('',#23552,.T.) ;
#19239=FACE_OUTER_BOUND('',#23553,.T.) ;
#19240=FACE_OUTER_BOUND('',#23554,.T.) ;
#19241=FACE_OUTER_BOUND('',#23555,.T.) ;
#19242=FACE_OUTER_BOUND('',#23556,.T.) ;
#19243=FACE_OUTER_BOUND('',#23557,.T.) ;
#19244=FACE_OUTER_BOUND('',#23558,.T.) ;
#19245=FACE_OUTER_BOUND('',#23559,.T.) ;
#19246=FACE_OUTER_BOUND('',#23560,.T.) ;
#19247=FACE_OUTER_BOUND('',#23561,.T.) ;
#19248=FACE_OUTER_BOUND('',#23562,.T.) ;
#19249=FACE_OUTER_BOUND('',#23563,.T.) ;
#19250=FACE_OUTER_BOUND('',#23564,.T.) ;
#19251=FACE_OUTER_BOUND('',#23565,.T.) ;
#19252=FACE_OUTER_BOUND('',#23566,.T.) ;
#19253=FACE_OUTER_BOUND('',#23567,.T.) ;
#19254=FACE_OUTER_BOUND('',#23568,.T.) ;
#19255=FACE_OUTER_BOUND('',#23569,.T.) ;
#19256=FACE_OUTER_BOUND('',#23570,.T.) ;
#19257=FACE_OUTER_BOUND('',#23571,.T.) ;
#19258=FACE_OUTER_BOUND('',#23572,.T.) ;
#19259=FACE_OUTER_BOUND('',#23573,.T.) ;
#19260=FACE_OUTER_BOUND('',#23574,.T.) ;
#19261=FACE_OUTER_BOUND('',#23575,.T.) ;
#19262=FACE_OUTER_BOUND('',#23576,.T.) ;
#19263=FACE_OUTER_BOUND('',#23577,.T.) ;
#19264=FACE_OUTER_BOUND('',#23578,.T.) ;
#19265=FACE_OUTER_BOUND('',#23579,.T.) ;
#19266=FACE_OUTER_BOUND('',#23580,.T.) ;
#19267=FACE_OUTER_BOUND('',#23581,.T.) ;
#19268=FACE_OUTER_BOUND('',#23582,.T.) ;
#19269=FACE_OUTER_BOUND('',#23583,.T.) ;
#19270=FACE_OUTER_BOUND('',#23584,.T.) ;
#19271=FACE_OUTER_BOUND('',#23585,.T.) ;
#19272=FACE_OUTER_BOUND('',#23586,.T.) ;
#19273=FACE_OUTER_BOUND('',#23587,.T.) ;
#19274=FACE_OUTER_BOUND('',#23588,.T.) ;
#19275=FACE_OUTER_BOUND('',#23589,.T.) ;
#19276=FACE_OUTER_BOUND('',#23590,.T.) ;
#19277=FACE_OUTER_BOUND('',#23591,.T.) ;
#19278=FACE_OUTER_BOUND('',#23592,.T.) ;
#19279=FACE_OUTER_BOUND('',#23593,.T.) ;
#19280=FACE_OUTER_BOUND('',#23594,.T.) ;
#19281=FACE_OUTER_BOUND('',#23595,.T.) ;
#19282=FACE_OUTER_BOUND('',#23596,.T.) ;
#19283=FACE_OUTER_BOUND('',#23597,.T.) ;
#19284=FACE_OUTER_BOUND('',#23598,.T.) ;
#19285=FACE_OUTER_BOUND('',#23599,.T.) ;
#19286=FACE_OUTER_BOUND('',#23600,.T.) ;
#19287=FACE_OUTER_BOUND('',#23601,.T.) ;
#19288=FACE_OUTER_BOUND('',#23602,.T.) ;
#19289=FACE_OUTER_BOUND('',#23603,.T.) ;
#19290=FACE_OUTER_BOUND('',#23604,.T.) ;
#19291=FACE_OUTER_BOUND('',#23605,.T.) ;
#19292=FACE_OUTER_BOUND('',#23606,.T.) ;
#19293=FACE_OUTER_BOUND('',#23607,.T.) ;
#19294=FACE_OUTER_BOUND('',#23608,.T.) ;
#19295=FACE_OUTER_BOUND('',#23609,.T.) ;
#19296=FACE_OUTER_BOUND('',#23610,.T.) ;
#19297=FACE_OUTER_BOUND('',#23611,.T.) ;
#19298=FACE_OUTER_BOUND('',#23612,.T.) ;
#19299=FACE_OUTER_BOUND('',#23613,.T.) ;
#19300=FACE_OUTER_BOUND('',#23614,.T.) ;
#19301=FACE_OUTER_BOUND('',#23615,.T.) ;
#19302=FACE_OUTER_BOUND('',#23616,.T.) ;
#19303=FACE_OUTER_BOUND('',#23617,.T.) ;
#19304=FACE_OUTER_BOUND('',#23618,.T.) ;
#19305=FACE_OUTER_BOUND('',#23619,.T.) ;
#19306=FACE_OUTER_BOUND('',#23620,.T.) ;
#19307=FACE_OUTER_BOUND('',#23621,.T.) ;
#19308=FACE_OUTER_BOUND('',#23622,.T.) ;
#19309=FACE_OUTER_BOUND('',#23623,.T.) ;
#19310=FACE_OUTER_BOUND('',#23624,.T.) ;
#19311=FACE_OUTER_BOUND('',#23625,.T.) ;
#19312=FACE_OUTER_BOUND('',#23626,.T.) ;
#19313=FACE_OUTER_BOUND('',#23627,.T.) ;
#19314=FACE_OUTER_BOUND('',#23628,.T.) ;
#19315=FACE_OUTER_BOUND('',#23629,.T.) ;
#19316=FACE_OUTER_BOUND('',#23630,.T.) ;
#19317=FACE_OUTER_BOUND('',#23631,.T.) ;
#19318=FACE_OUTER_BOUND('',#23632,.T.) ;
#19319=FACE_OUTER_BOUND('',#23633,.T.) ;
#19320=FACE_OUTER_BOUND('',#23634,.T.) ;
#19321=FACE_OUTER_BOUND('',#23635,.T.) ;
#19322=FACE_OUTER_BOUND('',#23636,.T.) ;
#19323=FACE_OUTER_BOUND('',#23637,.T.) ;
#19324=FACE_OUTER_BOUND('',#23638,.T.) ;
#19325=FACE_OUTER_BOUND('',#23639,.T.) ;
#19326=FACE_OUTER_BOUND('',#23640,.T.) ;
#19327=FACE_OUTER_BOUND('',#23641,.T.) ;
#19328=FACE_OUTER_BOUND('',#23642,.T.) ;
#19329=FACE_OUTER_BOUND('',#23643,.T.) ;
#19330=FACE_OUTER_BOUND('',#23644,.T.) ;
#19331=FACE_OUTER_BOUND('',#23645,.T.) ;
#19332=FACE_OUTER_BOUND('',#23646,.T.) ;
#19333=FACE_OUTER_BOUND('',#23647,.T.) ;
#19334=FACE_OUTER_BOUND('',#23648,.T.) ;
#19335=FACE_OUTER_BOUND('',#23649,.T.) ;
#19336=FACE_OUTER_BOUND('',#23650,.T.) ;
#19337=FACE_OUTER_BOUND('',#23651,.T.) ;
#19338=FACE_OUTER_BOUND('',#23652,.T.) ;
#19339=FACE_OUTER_BOUND('',#23653,.T.) ;
#19340=FACE_OUTER_BOUND('',#23654,.T.) ;
#19341=FACE_OUTER_BOUND('',#23655,.T.) ;
#19342=FACE_OUTER_BOUND('',#23656,.T.) ;
#19343=FACE_OUTER_BOUND('',#23657,.T.) ;
#19344=FACE_OUTER_BOUND('',#23658,.T.) ;
#19345=FACE_OUTER_BOUND('',#23659,.T.) ;
#19346=FACE_OUTER_BOUND('',#23660,.T.) ;
#19347=FACE_OUTER_BOUND('',#23661,.T.) ;
#19348=FACE_OUTER_BOUND('',#23662,.T.) ;
#19349=FACE_OUTER_BOUND('',#23663,.T.) ;
#19350=FACE_OUTER_BOUND('',#23664,.T.) ;
#19351=FACE_OUTER_BOUND('',#23665,.T.) ;
#19352=FACE_OUTER_BOUND('',#23666,.T.) ;
#19353=FACE_OUTER_BOUND('',#23667,.T.) ;
#19354=FACE_OUTER_BOUND('',#23668,.T.) ;
#19355=FACE_OUTER_BOUND('',#23669,.T.) ;
#19356=FACE_OUTER_BOUND('',#23670,.T.) ;
#19357=FACE_OUTER_BOUND('',#23671,.T.) ;
#19358=FACE_OUTER_BOUND('',#23672,.T.) ;
#19359=FACE_OUTER_BOUND('',#23673,.T.) ;
#19360=FACE_OUTER_BOUND('',#23674,.T.) ;
#19361=FACE_OUTER_BOUND('',#23675,.T.) ;
#19362=FACE_OUTER_BOUND('',#23676,.T.) ;
#19363=FACE_OUTER_BOUND('',#23677,.T.) ;
#19364=FACE_OUTER_BOUND('',#23678,.T.) ;
#19365=FACE_OUTER_BOUND('',#23679,.T.) ;
#19366=FACE_OUTER_BOUND('',#23680,.T.) ;
#19367=FACE_OUTER_BOUND('',#23681,.T.) ;
#19368=FACE_OUTER_BOUND('',#23682,.T.) ;
#19369=FACE_OUTER_BOUND('',#23683,.T.) ;
#19370=FACE_OUTER_BOUND('',#23684,.T.) ;
#19371=FACE_OUTER_BOUND('',#23685,.T.) ;
#19372=FACE_OUTER_BOUND('',#23686,.T.) ;
#19373=FACE_OUTER_BOUND('',#23687,.T.) ;
#19374=FACE_OUTER_BOUND('',#23688,.T.) ;
#19375=FACE_OUTER_BOUND('',#23689,.T.) ;
#19376=FACE_OUTER_BOUND('',#23690,.T.) ;
#19377=FACE_OUTER_BOUND('',#23691,.T.) ;
#19378=FACE_OUTER_BOUND('',#23692,.T.) ;
#19379=FACE_OUTER_BOUND('',#23693,.T.) ;
#19380=FACE_OUTER_BOUND('',#23694,.T.) ;
#19381=FACE_OUTER_BOUND('',#23695,.T.) ;
#19382=FACE_OUTER_BOUND('',#23696,.T.) ;
#19383=FACE_OUTER_BOUND('',#23697,.T.) ;
#19384=FACE_OUTER_BOUND('',#23698,.T.) ;
#19385=FACE_OUTER_BOUND('',#23699,.T.) ;
#19386=FACE_OUTER_BOUND('',#23700,.T.) ;
#19387=FACE_OUTER_BOUND('',#23701,.T.) ;
#19388=FACE_OUTER_BOUND('',#23702,.T.) ;
#19389=FACE_OUTER_BOUND('',#23703,.T.) ;
#19390=FACE_OUTER_BOUND('',#23704,.T.) ;
#19391=FACE_OUTER_BOUND('',#23705,.T.) ;
#19392=FACE_OUTER_BOUND('',#23706,.T.) ;
#19393=FACE_OUTER_BOUND('',#23707,.T.) ;
#19394=FACE_OUTER_BOUND('',#23708,.T.) ;
#19395=FACE_OUTER_BOUND('',#23709,.T.) ;
#19396=FACE_OUTER_BOUND('',#23710,.T.) ;
#19397=FACE_OUTER_BOUND('',#23711,.T.) ;
#19398=FACE_OUTER_BOUND('',#23712,.T.) ;
#19399=FACE_OUTER_BOUND('',#23713,.T.) ;
#19400=FACE_OUTER_BOUND('',#23714,.T.) ;
#19401=FACE_OUTER_BOUND('',#23715,.T.) ;
#19402=FACE_OUTER_BOUND('',#23716,.T.) ;
#19403=FACE_OUTER_BOUND('',#23717,.T.) ;
#19404=FACE_OUTER_BOUND('',#23718,.T.) ;
#19405=FACE_OUTER_BOUND('',#23719,.T.) ;
#19406=FACE_OUTER_BOUND('',#23720,.T.) ;
#19407=FACE_OUTER_BOUND('',#23721,.T.) ;
#19408=FACE_OUTER_BOUND('',#23722,.T.) ;
#19409=FACE_OUTER_BOUND('',#23723,.T.) ;
#19410=FACE_OUTER_BOUND('',#23724,.T.) ;
#19411=FACE_OUTER_BOUND('',#23725,.T.) ;
#19412=FACE_OUTER_BOUND('',#23726,.T.) ;
#19413=FACE_OUTER_BOUND('',#23727,.T.) ;
#19414=FACE_OUTER_BOUND('',#23728,.T.) ;
#19415=FACE_OUTER_BOUND('',#23729,.T.) ;
#19416=FACE_OUTER_BOUND('',#23730,.T.) ;
#19417=FACE_OUTER_BOUND('',#23731,.T.) ;
#19418=FACE_OUTER_BOUND('',#23732,.T.) ;
#19419=FACE_OUTER_BOUND('',#23733,.T.) ;
#19420=FACE_OUTER_BOUND('',#23734,.T.) ;
#19421=FACE_OUTER_BOUND('',#23735,.T.) ;
#19422=FACE_OUTER_BOUND('',#23736,.T.) ;
#19423=FACE_OUTER_BOUND('',#23737,.T.) ;
#19424=FACE_OUTER_BOUND('',#23738,.T.) ;
#19425=FACE_OUTER_BOUND('',#23739,.T.) ;
#19426=FACE_OUTER_BOUND('',#23740,.T.) ;
#19427=FACE_OUTER_BOUND('',#23741,.T.) ;
#19428=FACE_OUTER_BOUND('',#23742,.T.) ;
#19429=FACE_OUTER_BOUND('',#23743,.T.) ;
#19430=FACE_OUTER_BOUND('',#23744,.T.) ;
#19431=FACE_OUTER_BOUND('',#23745,.T.) ;
#19432=FACE_OUTER_BOUND('',#23746,.T.) ;
#19433=FACE_OUTER_BOUND('',#23747,.T.) ;
#19434=FACE_OUTER_BOUND('',#23748,.T.) ;
#19435=FACE_OUTER_BOUND('',#23749,.T.) ;
#19436=FACE_OUTER_BOUND('',#23750,.T.) ;
#19437=FACE_OUTER_BOUND('',#23751,.T.) ;
#19438=FACE_OUTER_BOUND('',#23752,.T.) ;
#19439=FACE_OUTER_BOUND('',#23753,.T.) ;
#19440=FACE_OUTER_BOUND('',#23754,.T.) ;
#19441=FACE_OUTER_BOUND('',#23755,.T.) ;
#19442=FACE_OUTER_BOUND('',#23756,.T.) ;
#19443=FACE_OUTER_BOUND('',#23757,.T.) ;
#19444=FACE_OUTER_BOUND('',#23758,.T.) ;
#19445=FACE_OUTER_BOUND('',#23759,.T.) ;
#19446=FACE_OUTER_BOUND('',#23760,.T.) ;
#19447=FACE_OUTER_BOUND('',#23761,.T.) ;
#19448=FACE_OUTER_BOUND('',#23762,.T.) ;
#19449=FACE_OUTER_BOUND('',#23763,.T.) ;
#19450=FACE_OUTER_BOUND('',#23764,.T.) ;
#19451=FACE_OUTER_BOUND('',#23765,.T.) ;
#19452=FACE_OUTER_BOUND('',#23766,.T.) ;
#19453=FACE_OUTER_BOUND('',#23767,.T.) ;
#19454=FACE_OUTER_BOUND('',#23768,.T.) ;
#19455=FACE_OUTER_BOUND('',#23769,.T.) ;
#19456=FACE_OUTER_BOUND('',#23770,.T.) ;
#19457=FACE_OUTER_BOUND('',#23771,.T.) ;
#19458=FACE_OUTER_BOUND('',#23772,.T.) ;
#19459=FACE_OUTER_BOUND('',#23773,.T.) ;
#19460=FACE_OUTER_BOUND('',#23774,.T.) ;
#19461=FACE_OUTER_BOUND('',#23775,.T.) ;
#19462=FACE_OUTER_BOUND('',#23776,.T.) ;
#19463=FACE_OUTER_BOUND('',#23777,.T.) ;
#19464=FACE_OUTER_BOUND('',#23778,.T.) ;
#19465=FACE_OUTER_BOUND('',#23779,.T.) ;
#19466=FACE_OUTER_BOUND('',#23780,.T.) ;
#19467=FACE_OUTER_BOUND('',#23781,.T.) ;
#19468=FACE_OUTER_BOUND('',#23782,.T.) ;
#19469=FACE_OUTER_BOUND('',#23783,.T.) ;
#19470=FACE_OUTER_BOUND('',#23784,.T.) ;
#19471=FACE_OUTER_BOUND('',#23785,.T.) ;
#19472=FACE_OUTER_BOUND('',#23786,.T.) ;
#19473=FACE_OUTER_BOUND('',#23787,.T.) ;
#19474=FACE_OUTER_BOUND('',#23788,.T.) ;
#19475=FACE_OUTER_BOUND('',#23789,.T.) ;
#19476=FACE_OUTER_BOUND('',#23790,.T.) ;
#19477=FACE_OUTER_BOUND('',#23791,.T.) ;
#19478=FACE_OUTER_BOUND('',#23792,.T.) ;
#19479=FACE_OUTER_BOUND('',#23793,.T.) ;
#19480=FACE_OUTER_BOUND('',#23794,.T.) ;
#19481=FACE_OUTER_BOUND('',#23795,.T.) ;
#19482=FACE_OUTER_BOUND('',#23796,.T.) ;
#19483=FACE_OUTER_BOUND('',#23797,.T.) ;
#19484=FACE_OUTER_BOUND('',#23798,.T.) ;
#19485=FACE_OUTER_BOUND('',#23799,.T.) ;
#19486=FACE_OUTER_BOUND('',#23800,.T.) ;
#19487=FACE_OUTER_BOUND('',#23801,.T.) ;
#19488=FACE_OUTER_BOUND('',#23802,.T.) ;
#19489=FACE_OUTER_BOUND('',#23803,.T.) ;
#19490=FACE_OUTER_BOUND('',#23804,.T.) ;
#19491=FACE_OUTER_BOUND('',#23805,.T.) ;
#19492=FACE_OUTER_BOUND('',#23806,.T.) ;
#19493=FACE_OUTER_BOUND('',#23807,.T.) ;
#19494=FACE_OUTER_BOUND('',#23808,.T.) ;
#19495=FACE_OUTER_BOUND('',#23809,.T.) ;
#19496=FACE_OUTER_BOUND('',#23810,.T.) ;
#19497=FACE_OUTER_BOUND('',#23811,.T.) ;
#19498=FACE_OUTER_BOUND('',#23812,.T.) ;
#19499=FACE_OUTER_BOUND('',#23813,.T.) ;
#19500=FACE_OUTER_BOUND('',#23814,.T.) ;
#19501=FACE_OUTER_BOUND('',#23815,.T.) ;
#19502=FACE_OUTER_BOUND('',#23816,.T.) ;
#19503=FACE_OUTER_BOUND('',#23817,.T.) ;
#19504=FACE_OUTER_BOUND('',#23818,.T.) ;
#19505=FACE_OUTER_BOUND('',#23819,.T.) ;
#19506=FACE_OUTER_BOUND('',#23820,.T.) ;
#19507=FACE_OUTER_BOUND('',#23821,.T.) ;
#19508=FACE_OUTER_BOUND('',#23822,.T.) ;
#19509=FACE_OUTER_BOUND('',#23823,.T.) ;
#19510=FACE_OUTER_BOUND('',#23824,.T.) ;
#19511=FACE_OUTER_BOUND('',#23825,.T.) ;
#19512=FACE_OUTER_BOUND('',#23826,.T.) ;
#19513=FACE_OUTER_BOUND('',#23827,.T.) ;
#19514=FACE_OUTER_BOUND('',#23828,.T.) ;
#19515=FACE_OUTER_BOUND('',#23829,.T.) ;
#19516=FACE_OUTER_BOUND('',#23830,.T.) ;
#19517=FACE_OUTER_BOUND('',#23831,.T.) ;
#19518=FACE_OUTER_BOUND('',#23832,.T.) ;
#19519=FACE_OUTER_BOUND('',#23833,.T.) ;
#19520=FACE_OUTER_BOUND('',#23834,.T.) ;
#19521=FACE_OUTER_BOUND('',#23835,.T.) ;
#19522=FACE_OUTER_BOUND('',#23836,.T.) ;
#19523=FACE_OUTER_BOUND('',#23837,.T.) ;
#19524=FACE_OUTER_BOUND('',#23838,.T.) ;
#19525=FACE_OUTER_BOUND('',#23839,.T.) ;
#19526=FACE_OUTER_BOUND('',#23840,.T.) ;
#19527=FACE_OUTER_BOUND('',#23841,.T.) ;
#19528=FACE_OUTER_BOUND('',#23842,.T.) ;
#19529=FACE_OUTER_BOUND('',#23843,.T.) ;
#19530=FACE_OUTER_BOUND('',#23844,.T.) ;
#19531=FACE_OUTER_BOUND('',#23845,.T.) ;
#19532=FACE_OUTER_BOUND('',#23846,.T.) ;
#19533=FACE_OUTER_BOUND('',#23847,.T.) ;
#19534=FACE_OUTER_BOUND('',#23848,.T.) ;
#19535=FACE_OUTER_BOUND('',#23849,.T.) ;
#19536=FACE_OUTER_BOUND('',#23850,.T.) ;
#19537=FACE_OUTER_BOUND('',#23851,.T.) ;
#19538=FACE_OUTER_BOUND('',#23852,.T.) ;
#19539=FACE_OUTER_BOUND('',#23853,.T.) ;
#19540=FACE_OUTER_BOUND('',#23854,.T.) ;
#19541=FACE_OUTER_BOUND('',#23855,.T.) ;
#19542=FACE_OUTER_BOUND('',#23856,.T.) ;
#19543=FACE_OUTER_BOUND('',#23857,.T.) ;
#19544=FACE_OUTER_BOUND('',#23858,.T.) ;
#19545=FACE_OUTER_BOUND('',#23859,.T.) ;
#19546=FACE_OUTER_BOUND('',#23860,.T.) ;
#19547=FACE_OUTER_BOUND('',#23861,.T.) ;
#19548=FACE_OUTER_BOUND('',#23862,.T.) ;
#19549=FACE_OUTER_BOUND('',#23863,.T.) ;
#19550=FACE_OUTER_BOUND('',#23864,.T.) ;
#19551=FACE_OUTER_BOUND('',#23865,.T.) ;
#19552=FACE_OUTER_BOUND('',#23866,.T.) ;
#19553=FACE_OUTER_BOUND('',#23867,.T.) ;
#19554=FACE_OUTER_BOUND('',#23868,.T.) ;
#19555=FACE_OUTER_BOUND('',#23869,.T.) ;
#19556=FACE_OUTER_BOUND('',#23870,.T.) ;
#19557=FACE_OUTER_BOUND('',#23871,.T.) ;
#19558=FACE_OUTER_BOUND('',#23872,.T.) ;
#19559=FACE_OUTER_BOUND('',#23873,.T.) ;
#19560=FACE_OUTER_BOUND('',#23874,.T.) ;
#19561=FACE_OUTER_BOUND('',#23875,.T.) ;
#19562=FACE_OUTER_BOUND('',#23876,.T.) ;
#19563=FACE_OUTER_BOUND('',#23877,.T.) ;
#19564=FACE_OUTER_BOUND('',#23878,.T.) ;
#19565=FACE_OUTER_BOUND('',#23879,.T.) ;
#19566=FACE_OUTER_BOUND('',#23880,.T.) ;
#19567=FACE_OUTER_BOUND('',#23881,.T.) ;
#19568=FACE_OUTER_BOUND('',#23882,.T.) ;
#19569=FACE_OUTER_BOUND('',#23883,.T.) ;
#19570=FACE_OUTER_BOUND('',#23884,.T.) ;
#19571=FACE_OUTER_BOUND('',#23885,.T.) ;
#19572=FACE_OUTER_BOUND('',#23886,.T.) ;
#19573=FACE_OUTER_BOUND('',#23887,.T.) ;
#19574=FACE_OUTER_BOUND('',#23888,.T.) ;
#19575=FACE_OUTER_BOUND('',#23889,.T.) ;
#19576=FACE_OUTER_BOUND('',#23890,.T.) ;
#19577=FACE_OUTER_BOUND('',#23891,.T.) ;
#19578=FACE_OUTER_BOUND('',#23892,.T.) ;
#19579=FACE_OUTER_BOUND('',#23893,.T.) ;
#19580=FACE_OUTER_BOUND('',#23894,.T.) ;
#19581=FACE_OUTER_BOUND('',#23895,.T.) ;
#19582=FACE_OUTER_BOUND('',#23896,.T.) ;
#19583=FACE_OUTER_BOUND('',#23897,.T.) ;
#19584=FACE_OUTER_BOUND('',#23898,.T.) ;
#19585=FACE_OUTER_BOUND('',#23899,.T.) ;
#19586=FACE_OUTER_BOUND('',#23900,.T.) ;
#19587=FACE_OUTER_BOUND('',#23901,.T.) ;
#19588=FACE_OUTER_BOUND('',#23902,.T.) ;
#19589=FACE_OUTER_BOUND('',#23903,.T.) ;
#19590=FACE_OUTER_BOUND('',#23904,.T.) ;
#19591=FACE_OUTER_BOUND('',#23905,.T.) ;
#19592=FACE_OUTER_BOUND('',#23906,.T.) ;
#19593=FACE_OUTER_BOUND('',#23907,.T.) ;
#19594=FACE_OUTER_BOUND('',#23908,.T.) ;
#19595=FACE_OUTER_BOUND('',#23909,.T.) ;
#19596=FACE_OUTER_BOUND('',#23910,.T.) ;
#19597=FACE_OUTER_BOUND('',#23911,.T.) ;
#19598=FACE_OUTER_BOUND('',#23912,.T.) ;
#19599=FACE_OUTER_BOUND('',#23913,.T.) ;
#19600=FACE_OUTER_BOUND('',#23914,.T.) ;
#19601=FACE_OUTER_BOUND('',#23915,.T.) ;
#19602=FACE_OUTER_BOUND('',#23916,.T.) ;
#19603=FACE_OUTER_BOUND('',#23917,.T.) ;
#19604=FACE_OUTER_BOUND('',#23918,.T.) ;
#19605=FACE_OUTER_BOUND('',#23919,.T.) ;
#19606=FACE_OUTER_BOUND('',#23920,.T.) ;
#19607=FACE_OUTER_BOUND('',#23921,.T.) ;
#19608=FACE_OUTER_BOUND('',#23922,.T.) ;
#19609=FACE_OUTER_BOUND('',#23923,.T.) ;
#19610=FACE_OUTER_BOUND('',#23924,.T.) ;
#19611=FACE_OUTER_BOUND('',#23925,.T.) ;
#19612=FACE_OUTER_BOUND('',#23926,.T.) ;
#19613=FACE_OUTER_BOUND('',#23927,.T.) ;
#19614=FACE_OUTER_BOUND('',#23928,.T.) ;
#19615=FACE_OUTER_BOUND('',#23929,.T.) ;
#19616=FACE_OUTER_BOUND('',#23930,.T.) ;
#19617=FACE_OUTER_BOUND('',#23931,.T.) ;
#19618=FACE_OUTER_BOUND('',#23932,.T.) ;
#19619=FACE_OUTER_BOUND('',#23933,.T.) ;
#19620=FACE_OUTER_BOUND('',#23934,.T.) ;
#19621=FACE_OUTER_BOUND('',#23935,.T.) ;
#19622=FACE_OUTER_BOUND('',#23936,.T.) ;
#19623=FACE_OUTER_BOUND('',#23937,.T.) ;
#19624=FACE_OUTER_BOUND('',#23938,.T.) ;
#19625=FACE_OUTER_BOUND('',#23939,.T.) ;
#19626=FACE_OUTER_BOUND('',#23940,.T.) ;
#19627=FACE_OUTER_BOUND('',#23941,.T.) ;
#19628=FACE_OUTER_BOUND('',#23942,.T.) ;
#19629=FACE_OUTER_BOUND('',#23943,.T.) ;
#19630=FACE_OUTER_BOUND('',#23944,.T.) ;
#19631=FACE_OUTER_BOUND('',#23945,.T.) ;
#19632=FACE_OUTER_BOUND('',#23946,.T.) ;
#19633=FACE_OUTER_BOUND('',#23947,.T.) ;
#19634=FACE_OUTER_BOUND('',#23948,.T.) ;
#19635=FACE_OUTER_BOUND('',#23949,.T.) ;
#19636=FACE_OUTER_BOUND('',#23950,.T.) ;
#19637=FACE_OUTER_BOUND('',#23951,.T.) ;
#19638=FACE_OUTER_BOUND('',#23952,.T.) ;
#19639=FACE_OUTER_BOUND('',#23953,.T.) ;
#19640=FACE_OUTER_BOUND('',#23954,.T.) ;
#19641=FACE_OUTER_BOUND('',#23955,.T.) ;
#19642=FACE_OUTER_BOUND('',#23956,.T.) ;
#19643=FACE_OUTER_BOUND('',#23957,.T.) ;
#19644=FACE_OUTER_BOUND('',#23958,.T.) ;
#19645=FACE_OUTER_BOUND('',#23959,.T.) ;
#19646=FACE_OUTER_BOUND('',#23960,.T.) ;
#19647=FACE_OUTER_BOUND('',#23961,.T.) ;
#19648=FACE_OUTER_BOUND('',#23962,.T.) ;
#19649=FACE_OUTER_BOUND('',#23963,.T.) ;
#19650=FACE_OUTER_BOUND('',#23964,.T.) ;
#19651=FACE_OUTER_BOUND('',#23965,.T.) ;
#19652=FACE_OUTER_BOUND('',#23966,.T.) ;
#19653=FACE_OUTER_BOUND('',#23967,.T.) ;
#19654=FACE_OUTER_BOUND('',#23968,.T.) ;
#19655=FACE_OUTER_BOUND('',#23969,.T.) ;
#19656=FACE_OUTER_BOUND('',#23970,.T.) ;
#19657=FACE_OUTER_BOUND('',#23971,.T.) ;
#19658=FACE_OUTER_BOUND('',#23972,.T.) ;
#19659=FACE_OUTER_BOUND('',#23973,.T.) ;
#19660=FACE_OUTER_BOUND('',#23974,.T.) ;
#19661=FACE_OUTER_BOUND('',#23975,.T.) ;
#19662=FACE_OUTER_BOUND('',#23976,.T.) ;
#19663=FACE_OUTER_BOUND('',#23977,.T.) ;
#19664=FACE_OUTER_BOUND('',#23978,.T.) ;
#19665=FACE_OUTER_BOUND('',#23979,.T.) ;
#19666=FACE_OUTER_BOUND('',#23980,.T.) ;
#19667=FACE_OUTER_BOUND('',#23981,.T.) ;
#19668=FACE_OUTER_BOUND('',#23982,.T.) ;
#19669=FACE_OUTER_BOUND('',#23983,.T.) ;
#19670=FACE_OUTER_BOUND('',#23984,.T.) ;
#19671=FACE_OUTER_BOUND('',#23985,.T.) ;
#19672=FACE_OUTER_BOUND('',#23986,.T.) ;
#19673=FACE_OUTER_BOUND('',#23987,.T.) ;
#19674=FACE_OUTER_BOUND('',#23988,.T.) ;
#19675=FACE_OUTER_BOUND('',#23989,.T.) ;
#19676=FACE_OUTER_BOUND('',#23990,.T.) ;
#19677=FACE_OUTER_BOUND('',#23991,.T.) ;
#19678=FACE_OUTER_BOUND('',#23992,.T.) ;
#19679=FACE_OUTER_BOUND('',#23993,.T.) ;
#19680=FACE_OUTER_BOUND('',#23994,.T.) ;
#19681=FACE_OUTER_BOUND('',#23995,.T.) ;
#19682=FACE_OUTER_BOUND('',#23996,.T.) ;
#19683=FACE_OUTER_BOUND('',#23997,.T.) ;
#19684=FACE_OUTER_BOUND('',#23998,.T.) ;
#19685=FACE_OUTER_BOUND('',#23999,.T.) ;
#19686=FACE_OUTER_BOUND('',#24000,.T.) ;
#19687=FACE_OUTER_BOUND('',#24001,.T.) ;
#19688=FACE_OUTER_BOUND('',#24002,.T.) ;
#19689=FACE_OUTER_BOUND('',#24003,.T.) ;
#19690=FACE_OUTER_BOUND('',#24004,.T.) ;
#19691=FACE_OUTER_BOUND('',#24005,.T.) ;
#19692=FACE_OUTER_BOUND('',#24006,.T.) ;
#19693=FACE_OUTER_BOUND('',#24007,.T.) ;
#19694=FACE_OUTER_BOUND('',#24008,.T.) ;
#19695=FACE_OUTER_BOUND('',#24009,.T.) ;
#19696=FACE_OUTER_BOUND('',#24010,.T.) ;
#19697=FACE_OUTER_BOUND('',#24011,.T.) ;
#19698=FACE_OUTER_BOUND('',#24012,.T.) ;
#19699=FACE_OUTER_BOUND('',#24013,.T.) ;
#19700=FACE_OUTER_BOUND('',#24014,.T.) ;
#19701=FACE_OUTER_BOUND('',#24015,.T.) ;
#19702=FACE_OUTER_BOUND('',#24016,.T.) ;
#19703=FACE_OUTER_BOUND('',#24017,.T.) ;
#19704=FACE_OUTER_BOUND('',#24018,.T.) ;
#19705=FACE_OUTER_BOUND('',#24019,.T.) ;
#19706=FACE_OUTER_BOUND('',#24020,.T.) ;
#19707=FACE_OUTER_BOUND('',#24021,.T.) ;
#19708=FACE_OUTER_BOUND('',#24022,.T.) ;
#19709=FACE_OUTER_BOUND('',#24023,.T.) ;
#19710=FACE_OUTER_BOUND('',#24024,.T.) ;
#19711=FACE_OUTER_BOUND('',#24025,.T.) ;
#19712=FACE_OUTER_BOUND('',#24026,.T.) ;
#19713=FACE_OUTER_BOUND('',#24027,.T.) ;
#19714=FACE_OUTER_BOUND('',#24028,.T.) ;
#19715=FACE_OUTER_BOUND('',#24029,.T.) ;
#19716=FACE_OUTER_BOUND('',#24030,.T.) ;
#19717=FACE_OUTER_BOUND('',#24031,.T.) ;
#19718=FACE_OUTER_BOUND('',#24032,.T.) ;
#19719=FACE_OUTER_BOUND('',#24033,.T.) ;
#19720=FACE_OUTER_BOUND('',#24034,.T.) ;
#19721=FACE_OUTER_BOUND('',#24035,.T.) ;
#19722=FACE_OUTER_BOUND('',#24036,.T.) ;
#19723=FACE_OUTER_BOUND('',#24037,.T.) ;
#19724=FACE_OUTER_BOUND('',#24038,.T.) ;
#19725=FACE_OUTER_BOUND('',#24039,.T.) ;
#19726=FACE_OUTER_BOUND('',#24040,.T.) ;
#19727=FACE_OUTER_BOUND('',#24041,.T.) ;
#19728=FACE_OUTER_BOUND('',#24042,.T.) ;
#19729=FACE_OUTER_BOUND('',#24043,.T.) ;
#19730=FACE_OUTER_BOUND('',#24044,.T.) ;
#19731=FACE_OUTER_BOUND('',#24045,.T.) ;
#19732=FACE_OUTER_BOUND('',#24046,.T.) ;
#19733=FACE_OUTER_BOUND('',#24047,.T.) ;
#19734=FACE_OUTER_BOUND('',#24048,.T.) ;
#19735=FACE_OUTER_BOUND('',#24049,.T.) ;
#19736=FACE_OUTER_BOUND('',#24050,.T.) ;
#19737=FACE_OUTER_BOUND('',#24051,.T.) ;
#19738=FACE_OUTER_BOUND('',#24052,.T.) ;
#19739=FACE_OUTER_BOUND('',#24053,.T.) ;
#19740=FACE_OUTER_BOUND('',#24054,.T.) ;
#19741=FACE_OUTER_BOUND('',#24055,.T.) ;
#19742=FACE_OUTER_BOUND('',#24056,.T.) ;
#19743=FACE_OUTER_BOUND('',#24057,.T.) ;
#19744=FACE_OUTER_BOUND('',#24058,.T.) ;
#19745=FACE_OUTER_BOUND('',#24059,.T.) ;
#19746=FACE_OUTER_BOUND('',#24060,.T.) ;
#19747=FACE_OUTER_BOUND('',#24061,.T.) ;
#19748=FACE_OUTER_BOUND('',#24062,.T.) ;
#19749=FACE_OUTER_BOUND('',#24063,.T.) ;
#19750=FACE_OUTER_BOUND('',#24064,.T.) ;
#19751=FACE_OUTER_BOUND('',#24065,.T.) ;
#19752=FACE_OUTER_BOUND('',#24066,.T.) ;
#19753=FACE_OUTER_BOUND('',#24067,.T.) ;
#19754=FACE_OUTER_BOUND('',#24068,.T.) ;
#19755=FACE_OUTER_BOUND('',#24069,.T.) ;
#19756=FACE_OUTER_BOUND('',#24070,.T.) ;
#19757=FACE_OUTER_BOUND('',#24071,.T.) ;
#19758=FACE_OUTER_BOUND('',#24072,.T.) ;
#19759=FACE_OUTER_BOUND('',#24073,.T.) ;
#19760=FACE_OUTER_BOUND('',#24074,.T.) ;
#19761=FACE_OUTER_BOUND('',#24075,.T.) ;
#19762=FACE_OUTER_BOUND('',#24076,.T.) ;
#19763=FACE_OUTER_BOUND('',#24077,.T.) ;
#19764=FACE_OUTER_BOUND('',#24078,.T.) ;
#19765=FACE_OUTER_BOUND('',#24079,.T.) ;
#19766=FACE_OUTER_BOUND('',#24080,.T.) ;
#19767=FACE_OUTER_BOUND('',#24081,.T.) ;
#19768=FACE_OUTER_BOUND('',#24082,.T.) ;
#19769=FACE_OUTER_BOUND('',#24083,.T.) ;
#19770=FACE_OUTER_BOUND('',#24084,.T.) ;
#19771=FACE_OUTER_BOUND('',#24085,.T.) ;
#19772=FACE_OUTER_BOUND('',#24086,.T.) ;
#19773=FACE_OUTER_BOUND('',#24087,.T.) ;
#19774=FACE_OUTER_BOUND('',#24088,.T.) ;
#19775=FACE_OUTER_BOUND('',#24089,.T.) ;
#19776=FACE_OUTER_BOUND('',#24090,.T.) ;
#19777=FACE_OUTER_BOUND('',#24091,.T.) ;
#19778=FACE_OUTER_BOUND('',#24092,.T.) ;
#19779=FACE_OUTER_BOUND('',#24093,.T.) ;
#19780=FACE_OUTER_BOUND('',#24094,.T.) ;
#19781=FACE_OUTER_BOUND('',#24095,.T.) ;
#19782=FACE_OUTER_BOUND('',#24096,.T.) ;
#19783=FACE_OUTER_BOUND('',#24097,.T.) ;
#19784=FACE_OUTER_BOUND('',#24098,.T.) ;
#19785=FACE_OUTER_BOUND('',#24099,.T.) ;
#19786=FACE_OUTER_BOUND('',#24100,.T.) ;
#19787=FACE_OUTER_BOUND('',#24101,.T.) ;
#19788=FACE_OUTER_BOUND('',#24102,.T.) ;
#19789=FACE_OUTER_BOUND('',#24103,.T.) ;
#19790=FACE_OUTER_BOUND('',#24104,.T.) ;
#19791=FACE_OUTER_BOUND('',#24105,.T.) ;
#19792=FACE_OUTER_BOUND('',#24106,.T.) ;
#19793=FACE_OUTER_BOUND('',#24107,.T.) ;
#19794=FACE_OUTER_BOUND('',#24108,.T.) ;
#19795=FACE_OUTER_BOUND('',#24109,.T.) ;
#19796=FACE_OUTER_BOUND('',#24110,.T.) ;
#19797=FACE_OUTER_BOUND('',#24111,.T.) ;
#19798=FACE_OUTER_BOUND('',#24112,.T.) ;
#19799=FACE_OUTER_BOUND('',#24113,.T.) ;
#19800=FACE_OUTER_BOUND('',#24114,.T.) ;
#19801=FACE_OUTER_BOUND('',#24115,.T.) ;
#19802=FACE_OUTER_BOUND('',#24116,.T.) ;
#19803=FACE_OUTER_BOUND('',#24117,.T.) ;
#19804=FACE_OUTER_BOUND('',#24118,.T.) ;
#19805=FACE_OUTER_BOUND('',#24119,.T.) ;
#19806=FACE_OUTER_BOUND('',#24120,.T.) ;
#19807=FACE_OUTER_BOUND('',#24121,.T.) ;
#19808=FACE_OUTER_BOUND('',#24122,.T.) ;
#19809=FACE_OUTER_BOUND('',#24123,.T.) ;
#19810=FACE_OUTER_BOUND('',#24124,.T.) ;
#19811=FACE_OUTER_BOUND('',#24125,.T.) ;
#19812=FACE_OUTER_BOUND('',#24126,.T.) ;
#19813=FACE_OUTER_BOUND('',#24127,.T.) ;
#19814=FACE_OUTER_BOUND('',#24128,.T.) ;
#19815=FACE_OUTER_BOUND('',#24129,.T.) ;
#19816=FACE_OUTER_BOUND('',#24130,.T.) ;
#19817=FACE_OUTER_BOUND('',#24131,.T.) ;
#19818=FACE_OUTER_BOUND('',#24132,.T.) ;
#19819=FACE_OUTER_BOUND('',#24133,.T.) ;
#19820=FACE_OUTER_BOUND('',#24134,.T.) ;
#19821=FACE_OUTER_BOUND('',#24135,.T.) ;
#19822=FACE_OUTER_BOUND('',#24136,.T.) ;
#19823=FACE_OUTER_BOUND('',#24137,.T.) ;
#19824=FACE_OUTER_BOUND('',#24138,.T.) ;
#19825=FACE_OUTER_BOUND('',#24139,.T.) ;
#19826=FACE_OUTER_BOUND('',#24140,.T.) ;
#19827=FACE_OUTER_BOUND('',#24141,.T.) ;
#19828=FACE_OUTER_BOUND('',#24142,.T.) ;
#19829=FACE_OUTER_BOUND('',#24143,.T.) ;
#19830=FACE_OUTER_BOUND('',#24144,.T.) ;
#19831=FACE_OUTER_BOUND('',#24145,.T.) ;
#19832=FACE_OUTER_BOUND('',#24146,.T.) ;
#19833=FACE_OUTER_BOUND('',#24147,.T.) ;
#19834=FACE_OUTER_BOUND('',#24148,.T.) ;
#19835=FACE_OUTER_BOUND('',#24149,.T.) ;
#19836=FACE_OUTER_BOUND('',#24150,.T.) ;
#19837=FACE_OUTER_BOUND('',#24151,.T.) ;
#19838=FACE_OUTER_BOUND('',#24152,.T.) ;
#19839=FACE_OUTER_BOUND('',#24153,.T.) ;
#19840=FACE_OUTER_BOUND('',#24154,.T.) ;
#19841=FACE_OUTER_BOUND('',#24155,.T.) ;
#19842=FACE_OUTER_BOUND('',#24156,.T.) ;
#19843=FACE_OUTER_BOUND('',#24157,.T.) ;
#19844=FACE_OUTER_BOUND('',#24158,.T.) ;
#19845=FACE_OUTER_BOUND('',#24159,.T.) ;
#19846=FACE_OUTER_BOUND('',#24160,.T.) ;
#19847=FACE_OUTER_BOUND('',#24161,.T.) ;
#19848=FACE_OUTER_BOUND('',#24162,.T.) ;
#19849=FACE_OUTER_BOUND('',#24163,.T.) ;
#19850=FACE_OUTER_BOUND('',#24164,.T.) ;
#19851=FACE_OUTER_BOUND('',#24165,.T.) ;
#19852=FACE_OUTER_BOUND('',#24166,.T.) ;
#19853=FACE_OUTER_BOUND('',#24167,.T.) ;
#19854=FACE_OUTER_BOUND('',#24168,.T.) ;
#19855=FACE_OUTER_BOUND('',#24169,.T.) ;
#19856=FACE_OUTER_BOUND('',#24170,.T.) ;
#19857=FACE_OUTER_BOUND('',#24171,.T.) ;
#19858=FACE_OUTER_BOUND('',#24172,.T.) ;
#19859=FACE_OUTER_BOUND('',#24173,.T.) ;
#19860=FACE_OUTER_BOUND('',#24174,.T.) ;
#19861=FACE_OUTER_BOUND('',#24175,.T.) ;
#19862=FACE_OUTER_BOUND('',#24176,.T.) ;
#19863=FACE_OUTER_BOUND('',#24177,.T.) ;
#19864=FACE_OUTER_BOUND('',#24178,.T.) ;
#19865=FACE_OUTER_BOUND('',#24179,.T.) ;
#19866=FACE_OUTER_BOUND('',#24180,.T.) ;
#19867=FACE_OUTER_BOUND('',#24181,.T.) ;
#19868=FACE_OUTER_BOUND('',#24182,.T.) ;
#19869=FACE_OUTER_BOUND('',#24183,.T.) ;
#19870=FACE_OUTER_BOUND('',#24184,.T.) ;
#19871=FACE_OUTER_BOUND('',#24185,.T.) ;
#19872=FACE_OUTER_BOUND('',#24186,.T.) ;
#19873=FACE_OUTER_BOUND('',#24187,.T.) ;
#19874=FACE_OUTER_BOUND('',#24188,.T.) ;
#19875=FACE_OUTER_BOUND('',#24189,.T.) ;
#19876=FACE_OUTER_BOUND('',#24190,.T.) ;
#19877=FACE_OUTER_BOUND('',#24191,.T.) ;
#19878=FACE_OUTER_BOUND('',#24192,.T.) ;
#19879=FACE_OUTER_BOUND('',#24193,.T.) ;
#19880=FACE_OUTER_BOUND('',#24194,.T.) ;
#19881=FACE_OUTER_BOUND('',#24195,.T.) ;
#19882=FACE_OUTER_BOUND('',#24196,.T.) ;
#19883=FACE_OUTER_BOUND('',#24197,.T.) ;
#19884=FACE_OUTER_BOUND('',#24198,.T.) ;
#19885=FACE_OUTER_BOUND('',#24199,.T.) ;
#19886=FACE_OUTER_BOUND('',#24200,.T.) ;
#19887=FACE_OUTER_BOUND('',#24201,.T.) ;
#19888=FACE_OUTER_BOUND('',#24202,.T.) ;
#19889=FACE_OUTER_BOUND('',#24203,.T.) ;
#19890=FACE_OUTER_BOUND('',#24204,.T.) ;
#19891=FACE_OUTER_BOUND('',#24205,.T.) ;
#19892=FACE_OUTER_BOUND('',#24206,.T.) ;
#19893=FACE_OUTER_BOUND('',#24207,.T.) ;
#19894=FACE_OUTER_BOUND('',#24208,.T.) ;
#19895=FACE_OUTER_BOUND('',#24209,.T.) ;
#19896=FACE_OUTER_BOUND('',#24210,.T.) ;
#19897=FACE_OUTER_BOUND('',#24211,.T.) ;
#19898=FACE_OUTER_BOUND('',#24212,.T.) ;
#19899=FACE_OUTER_BOUND('',#24213,.T.) ;
#19900=FACE_OUTER_BOUND('',#24214,.T.) ;
#19901=FACE_OUTER_BOUND('',#24215,.T.) ;
#19902=FACE_OUTER_BOUND('',#24216,.T.) ;
#19903=FACE_OUTER_BOUND('',#24217,.T.) ;
#19904=FACE_OUTER_BOUND('',#24218,.T.) ;
#19905=FACE_OUTER_BOUND('',#24219,.T.) ;
#19906=FACE_OUTER_BOUND('',#24220,.T.) ;
#19907=FACE_OUTER_BOUND('',#24221,.T.) ;
#19908=FACE_OUTER_BOUND('',#24222,.T.) ;
#19909=FACE_OUTER_BOUND('',#24223,.T.) ;
#19910=FACE_OUTER_BOUND('',#24224,.T.) ;
#19911=FACE_OUTER_BOUND('',#24225,.T.) ;
#19912=FACE_OUTER_BOUND('',#24226,.T.) ;
#19913=FACE_OUTER_BOUND('',#24227,.T.) ;
#19914=FACE_OUTER_BOUND('',#24228,.T.) ;
#19915=FACE_OUTER_BOUND('',#24229,.T.) ;
#19916=FACE_OUTER_BOUND('',#24230,.T.) ;
#19917=FACE_OUTER_BOUND('',#24231,.T.) ;
#19918=FACE_OUTER_BOUND('',#24232,.T.) ;
#19919=FACE_OUTER_BOUND('',#24233,.T.) ;
#19920=FACE_OUTER_BOUND('',#24234,.T.) ;
#19921=FACE_OUTER_BOUND('',#24235,.T.) ;
#19922=FACE_OUTER_BOUND('',#24236,.T.) ;
#19923=FACE_OUTER_BOUND('',#24237,.T.) ;
#19924=FACE_OUTER_BOUND('',#24238,.T.) ;
#19925=FACE_OUTER_BOUND('',#24239,.T.) ;
#19926=FACE_OUTER_BOUND('',#24240,.T.) ;
#19927=FACE_OUTER_BOUND('',#24241,.T.) ;
#19928=FACE_OUTER_BOUND('',#24242,.T.) ;
#19929=FACE_OUTER_BOUND('',#24243,.T.) ;
#19930=FACE_OUTER_BOUND('',#24244,.T.) ;
#19931=FACE_OUTER_BOUND('',#24245,.T.) ;
#19932=FACE_OUTER_BOUND('',#24246,.T.) ;
#19933=FACE_OUTER_BOUND('',#24247,.T.) ;
#19934=FACE_OUTER_BOUND('',#24248,.T.) ;
#19935=FACE_OUTER_BOUND('',#24249,.T.) ;
#19936=FACE_OUTER_BOUND('',#24250,.T.) ;
#19937=FACE_OUTER_BOUND('',#24251,.T.) ;
#19938=FACE_OUTER_BOUND('',#24252,.T.) ;
#19939=FACE_OUTER_BOUND('',#24253,.T.) ;
#19940=FACE_OUTER_BOUND('',#24254,.T.) ;
#19941=FACE_OUTER_BOUND('',#24255,.T.) ;
#19942=FACE_OUTER_BOUND('',#24256,.T.) ;
#19943=FACE_OUTER_BOUND('',#24257,.T.) ;
#19944=FACE_OUTER_BOUND('',#24258,.T.) ;
#19945=FACE_OUTER_BOUND('',#24259,.T.) ;
#19946=FACE_OUTER_BOUND('',#24260,.T.) ;
#19947=FACE_OUTER_BOUND('',#24261,.T.) ;
#19948=FACE_OUTER_BOUND('',#24262,.T.) ;
#19949=FACE_OUTER_BOUND('',#24263,.T.) ;
#19950=FACE_OUTER_BOUND('',#24264,.T.) ;
#19951=FACE_OUTER_BOUND('',#24265,.T.) ;
#19952=FACE_OUTER_BOUND('',#24266,.T.) ;
#19953=FACE_OUTER_BOUND('',#24267,.T.) ;
#19954=FACE_OUTER_BOUND('',#24268,.T.) ;
#19955=FACE_OUTER_BOUND('',#24269,.T.) ;
#19956=FACE_OUTER_BOUND('',#24270,.T.) ;
#19957=FACE_OUTER_BOUND('',#24271,.T.) ;
#19958=FACE_OUTER_BOUND('',#24272,.T.) ;
#19959=FACE_OUTER_BOUND('',#24273,.T.) ;
#19960=FACE_OUTER_BOUND('',#24274,.T.) ;
#19961=FACE_OUTER_BOUND('',#24275,.T.) ;
#19962=FACE_OUTER_BOUND('',#24276,.T.) ;
#19963=FACE_OUTER_BOUND('',#24277,.T.) ;
#19964=FACE_OUTER_BOUND('',#24278,.T.) ;
#19965=FACE_OUTER_BOUND('',#24279,.T.) ;
#19966=FACE_OUTER_BOUND('',#24280,.T.) ;
#19967=FACE_OUTER_BOUND('',#24281,.T.) ;
#19968=FACE_OUTER_BOUND('',#24282,.T.) ;
#19969=FACE_OUTER_BOUND('',#24283,.T.) ;
#19970=FACE_OUTER_BOUND('',#24284,.T.) ;
#19971=FACE_OUTER_BOUND('',#24285,.T.) ;
#19972=FACE_OUTER_BOUND('',#24286,.T.) ;
#19973=FACE_OUTER_BOUND('',#24287,.T.) ;
#19974=FACE_OUTER_BOUND('',#24288,.T.) ;
#19975=FACE_OUTER_BOUND('',#24289,.T.) ;
#19976=FACE_OUTER_BOUND('',#24290,.T.) ;
#19977=FACE_OUTER_BOUND('',#24291,.T.) ;
#19978=FACE_OUTER_BOUND('',#24292,.T.) ;
#19979=FACE_OUTER_BOUND('',#24293,.T.) ;
#19980=FACE_OUTER_BOUND('',#24294,.T.) ;
#19981=FACE_OUTER_BOUND('',#24295,.T.) ;
#19982=FACE_OUTER_BOUND('',#24296,.T.) ;
#19983=FACE_OUTER_BOUND('',#24297,.T.) ;
#19984=FACE_OUTER_BOUND('',#24298,.T.) ;
#19985=FACE_OUTER_BOUND('',#24299,.T.) ;
#19986=FACE_OUTER_BOUND('',#24300,.T.) ;
#19987=FACE_OUTER_BOUND('',#24301,.T.) ;
#19988=FACE_OUTER_BOUND('',#24302,.T.) ;
#19989=FACE_OUTER_BOUND('',#24303,.T.) ;
#19990=FACE_OUTER_BOUND('',#24304,.T.) ;
#19991=FACE_OUTER_BOUND('',#24305,.T.) ;
#19992=FACE_OUTER_BOUND('',#24306,.T.) ;
#19993=FACE_OUTER_BOUND('',#24307,.T.) ;
#19994=FACE_OUTER_BOUND('',#24308,.T.) ;
#19995=FACE_OUTER_BOUND('',#24309,.T.) ;
#19996=FACE_OUTER_BOUND('',#24310,.T.) ;
#19997=FACE_OUTER_BOUND('',#24311,.T.) ;
#19998=FACE_OUTER_BOUND('',#24312,.T.) ;
#19999=FACE_OUTER_BOUND('',#24313,.T.) ;
#20000=FACE_OUTER_BOUND('',#24314,.T.) ;
#20001=FACE_OUTER_BOUND('',#24315,.T.) ;
#20002=FACE_OUTER_BOUND('',#24316,.T.) ;
#20003=FACE_OUTER_BOUND('',#24317,.T.) ;
#20004=FACE_OUTER_BOUND('',#24318,.T.) ;
#20005=FACE_OUTER_BOUND('',#24319,.T.) ;
#20006=FACE_OUTER_BOUND('',#24320,.T.) ;
#20007=FACE_OUTER_BOUND('',#24321,.T.) ;
#20008=FACE_OUTER_BOUND('',#24322,.T.) ;
#20009=FACE_OUTER_BOUND('',#24323,.T.) ;
#20010=FACE_OUTER_BOUND('',#24324,.T.) ;
#20011=FACE_OUTER_BOUND('',#24325,.T.) ;
#20012=FACE_OUTER_BOUND('',#24326,.T.) ;
#20013=FACE_OUTER_BOUND('',#24327,.T.) ;
#20014=FACE_OUTER_BOUND('',#24328,.T.) ;
#20015=FACE_OUTER_BOUND('',#24329,.T.) ;
#20016=FACE_OUTER_BOUND('',#24330,.T.) ;
#20017=FACE_OUTER_BOUND('',#24331,.T.) ;
#20018=FACE_OUTER_BOUND('',#24332,.T.) ;
#20019=FACE_OUTER_BOUND('',#24333,.T.) ;
#20020=FACE_OUTER_BOUND('',#24334,.T.) ;
#20021=FACE_OUTER_BOUND('',#24335,.T.) ;
#20022=FACE_OUTER_BOUND('',#24336,.T.) ;
#20023=FACE_OUTER_BOUND('',#24337,.T.) ;
#20024=FACE_OUTER_BOUND('',#24338,.T.) ;
#20025=FACE_OUTER_BOUND('',#24339,.T.) ;
#20026=FACE_OUTER_BOUND('',#24340,.T.) ;
#20027=FACE_OUTER_BOUND('',#24341,.T.) ;
#20028=FACE_OUTER_BOUND('',#24342,.T.) ;
#20029=FACE_OUTER_BOUND('',#24343,.T.) ;
#20030=FACE_OUTER_BOUND('',#24344,.T.) ;
#20031=FACE_OUTER_BOUND('',#24345,.T.) ;
#20032=FACE_OUTER_BOUND('',#24346,.T.) ;
#20033=FACE_OUTER_BOUND('',#24347,.T.) ;
#20034=FACE_OUTER_BOUND('',#24348,.T.) ;
#20035=FACE_OUTER_BOUND('',#24349,.T.) ;
#20036=FACE_OUTER_BOUND('',#24350,.T.) ;
#20037=FACE_OUTER_BOUND('',#24351,.T.) ;
#20038=FACE_OUTER_BOUND('',#24352,.T.) ;
#20039=FACE_OUTER_BOUND('',#24353,.T.) ;
#20040=FACE_OUTER_BOUND('',#24354,.T.) ;
#20041=FACE_OUTER_BOUND('',#24355,.T.) ;
#20042=FACE_OUTER_BOUND('',#24356,.T.) ;
#20043=FACE_OUTER_BOUND('',#24357,.T.) ;
#20044=FACE_OUTER_BOUND('',#24358,.T.) ;
#20045=FACE_OUTER_BOUND('',#24359,.T.) ;
#20046=FACE_OUTER_BOUND('',#24360,.T.) ;
#20047=FACE_OUTER_BOUND('',#24361,.T.) ;
#20048=FACE_OUTER_BOUND('',#24362,.T.) ;
#20049=FACE_OUTER_BOUND('',#24363,.T.) ;
#20050=FACE_OUTER_BOUND('',#24364,.T.) ;
#20051=FACE_OUTER_BOUND('',#24365,.T.) ;
#20052=FACE_OUTER_BOUND('',#24366,.T.) ;
#20053=FACE_OUTER_BOUND('',#24367,.T.) ;
#20054=FACE_OUTER_BOUND('',#24368,.T.) ;
#20055=FACE_OUTER_BOUND('',#24369,.T.) ;
#20056=FACE_OUTER_BOUND('',#24370,.T.) ;
#20057=FACE_OUTER_BOUND('',#24371,.T.) ;
#20058=FACE_OUTER_BOUND('',#24372,.T.) ;
#20059=FACE_OUTER_BOUND('',#24373,.T.) ;
#20060=FACE_OUTER_BOUND('',#24374,.T.) ;
#20061=FACE_OUTER_BOUND('',#24375,.T.) ;
#20062=FACE_OUTER_BOUND('',#24376,.T.) ;
#20063=FACE_OUTER_BOUND('',#24377,.T.) ;
#20064=FACE_OUTER_BOUND('',#24378,.T.) ;
#20065=FACE_OUTER_BOUND('',#24379,.T.) ;
#20066=FACE_OUTER_BOUND('',#24380,.T.) ;
#20067=FACE_OUTER_BOUND('',#24381,.T.) ;
#20068=FACE_OUTER_BOUND('',#24382,.T.) ;
#20069=FACE_OUTER_BOUND('',#24383,.T.) ;
#20070=FACE_OUTER_BOUND('',#24384,.T.) ;
#20071=FACE_OUTER_BOUND('',#24385,.T.) ;
#20072=FACE_OUTER_BOUND('',#24386,.T.) ;
#20073=FACE_OUTER_BOUND('',#24387,.T.) ;
#20074=FACE_OUTER_BOUND('',#24388,.T.) ;
#20075=FACE_OUTER_BOUND('',#24389,.T.) ;
#20076=FACE_OUTER_BOUND('',#24390,.T.) ;
#20077=FACE_OUTER_BOUND('',#24391,.T.) ;
#20078=FACE_OUTER_BOUND('',#24392,.T.) ;
#20079=FACE_OUTER_BOUND('',#24393,.T.) ;
#20080=FACE_OUTER_BOUND('',#24394,.T.) ;
#20081=FACE_OUTER_BOUND('',#24395,.T.) ;
#20082=FACE_OUTER_BOUND('',#24396,.T.) ;
#20083=FACE_OUTER_BOUND('',#24397,.T.) ;
#20084=FACE_OUTER_BOUND('',#24398,.T.) ;
#20085=FACE_OUTER_BOUND('',#24399,.T.) ;
#20086=FACE_OUTER_BOUND('',#24400,.T.) ;
#20087=FACE_OUTER_BOUND('',#24401,.T.) ;
#20088=FACE_OUTER_BOUND('',#24402,.T.) ;
#20089=FACE_OUTER_BOUND('',#24403,.T.) ;
#20090=FACE_OUTER_BOUND('',#24404,.T.) ;
#20091=FACE_OUTER_BOUND('',#24405,.T.) ;
#20092=FACE_OUTER_BOUND('',#24406,.T.) ;
#20093=FACE_OUTER_BOUND('',#24407,.T.) ;
#20094=FACE_OUTER_BOUND('',#24408,.T.) ;
#20095=FACE_OUTER_BOUND('',#24409,.T.) ;
#20096=FACE_OUTER_BOUND('',#24410,.T.) ;
#20097=FACE_OUTER_BOUND('',#24411,.T.) ;
#20098=FACE_OUTER_BOUND('',#24412,.T.) ;
#20099=FACE_OUTER_BOUND('',#24413,.T.) ;
#20100=FACE_OUTER_BOUND('',#24414,.T.) ;
#20101=FACE_OUTER_BOUND('',#24415,.T.) ;
#20102=FACE_OUTER_BOUND('',#24416,.T.) ;
#20103=FACE_OUTER_BOUND('',#24417,.T.) ;
#20104=FACE_OUTER_BOUND('',#24418,.T.) ;
#20105=FACE_OUTER_BOUND('',#24419,.T.) ;
#20106=FACE_OUTER_BOUND('',#24420,.T.) ;
#20107=FACE_OUTER_BOUND('',#24421,.T.) ;
#20108=FACE_OUTER_BOUND('',#24422,.T.) ;
#20109=FACE_OUTER_BOUND('',#24423,.T.) ;
#20110=FACE_OUTER_BOUND('',#24424,.T.) ;
#20111=FACE_OUTER_BOUND('',#24425,.T.) ;
#20112=FACE_OUTER_BOUND('',#24426,.T.) ;
#20113=FACE_OUTER_BOUND('',#24427,.T.) ;
#20114=FACE_OUTER_BOUND('',#24428,.T.) ;
#20115=FACE_OUTER_BOUND('',#24429,.T.) ;
#20116=FACE_OUTER_BOUND('',#24430,.T.) ;
#20117=FACE_OUTER_BOUND('',#24431,.T.) ;
#20118=FACE_OUTER_BOUND('',#24432,.T.) ;
#20119=FACE_OUTER_BOUND('',#24433,.T.) ;
#20120=FACE_OUTER_BOUND('',#24434,.T.) ;
#20121=FACE_OUTER_BOUND('',#24435,.T.) ;
#20122=FACE_OUTER_BOUND('',#24436,.T.) ;
#20123=FACE_OUTER_BOUND('',#24437,.T.) ;
#20124=FACE_OUTER_BOUND('',#24438,.T.) ;
#20125=FACE_OUTER_BOUND('',#24439,.T.) ;
#20126=FACE_OUTER_BOUND('',#24440,.T.) ;
#20127=FACE_OUTER_BOUND('',#24441,.T.) ;
#20128=FACE_OUTER_BOUND('',#24442,.T.) ;
#20129=FACE_OUTER_BOUND('',#24443,.T.) ;
#20130=FACE_OUTER_BOUND('',#24444,.T.) ;
#20131=FACE_OUTER_BOUND('',#24445,.T.) ;
#20132=FACE_OUTER_BOUND('',#24446,.T.) ;
#20133=FACE_OUTER_BOUND('',#24447,.T.) ;
#20134=FACE_OUTER_BOUND('',#24448,.T.) ;
#20135=FACE_OUTER_BOUND('',#24449,.T.) ;
#20136=FACE_OUTER_BOUND('',#24450,.T.) ;
#20137=FACE_OUTER_BOUND('',#24451,.T.) ;
#20138=FACE_OUTER_BOUND('',#24452,.T.) ;
#20139=FACE_OUTER_BOUND('',#24453,.T.) ;
#20140=FACE_OUTER_BOUND('',#24454,.T.) ;
#20141=FACE_OUTER_BOUND('',#24455,.T.) ;
#20142=FACE_OUTER_BOUND('',#24456,.T.) ;
#20143=FACE_OUTER_BOUND('',#24457,.T.) ;
#20144=FACE_OUTER_BOUND('',#24458,.T.) ;
#20145=FACE_OUTER_BOUND('',#24459,.T.) ;
#20146=FACE_OUTER_BOUND('',#24460,.T.) ;
#20147=FACE_OUTER_BOUND('',#24461,.T.) ;
#20148=FACE_OUTER_BOUND('',#24462,.T.) ;
#20149=FACE_OUTER_BOUND('',#24463,.T.) ;
#20150=FACE_OUTER_BOUND('',#24464,.T.) ;
#20151=FACE_OUTER_BOUND('',#24465,.T.) ;
#20152=FACE_OUTER_BOUND('',#24466,.T.) ;
#20153=FACE_OUTER_BOUND('',#24467,.T.) ;
#20154=FACE_OUTER_BOUND('',#24468,.T.) ;
#20155=FACE_OUTER_BOUND('',#24469,.T.) ;
#20156=FACE_OUTER_BOUND('',#24470,.T.) ;
#20157=FACE_OUTER_BOUND('',#24471,.T.) ;
#20158=FACE_OUTER_BOUND('',#24472,.T.) ;
#20159=FACE_OUTER_BOUND('',#24473,.T.) ;
#20160=FACE_OUTER_BOUND('',#24474,.T.) ;
#20161=FACE_OUTER_BOUND('',#24475,.T.) ;
#20162=FACE_OUTER_BOUND('',#24476,.T.) ;
#20163=FACE_OUTER_BOUND('',#24477,.T.) ;
#20164=FACE_OUTER_BOUND('',#24478,.T.) ;
#20165=FACE_OUTER_BOUND('',#24479,.T.) ;
#20166=FACE_OUTER_BOUND('',#24480,.T.) ;
#20167=FACE_OUTER_BOUND('',#24481,.T.) ;
#20168=FACE_OUTER_BOUND('',#24482,.T.) ;
#20169=FACE_OUTER_BOUND('',#24483,.T.) ;
#20170=FACE_OUTER_BOUND('',#24484,.T.) ;
#20171=FACE_OUTER_BOUND('',#24485,.T.) ;
#20172=FACE_OUTER_BOUND('',#24486,.T.) ;
#20173=FACE_OUTER_BOUND('',#24487,.T.) ;
#20174=FACE_OUTER_BOUND('',#24488,.T.) ;
#20175=FACE_OUTER_BOUND('',#24489,.T.) ;
#20176=FACE_OUTER_BOUND('',#24490,.T.) ;
#20177=FACE_OUTER_BOUND('',#24491,.T.) ;
#20178=FACE_OUTER_BOUND('',#24492,.T.) ;
#20179=FACE_OUTER_BOUND('',#24493,.T.) ;
#20180=FACE_OUTER_BOUND('',#24494,.T.) ;
#20181=FACE_OUTER_BOUND('',#24495,.T.) ;
#20182=FACE_OUTER_BOUND('',#24496,.T.) ;
#20183=FACE_OUTER_BOUND('',#24497,.T.) ;
#20184=FACE_OUTER_BOUND('',#24498,.T.) ;
#20185=FACE_OUTER_BOUND('',#24499,.T.) ;
#20186=FACE_OUTER_BOUND('',#24500,.T.) ;
#20187=FACE_OUTER_BOUND('',#24501,.T.) ;
#20188=FACE_OUTER_BOUND('',#24502,.T.) ;
#20189=FACE_OUTER_BOUND('',#24503,.T.) ;
#20190=FACE_OUTER_BOUND('',#24504,.T.) ;
#20191=FACE_OUTER_BOUND('',#24505,.T.) ;
#20192=FACE_OUTER_BOUND('',#24506,.T.) ;
#20193=FACE_OUTER_BOUND('',#24507,.T.) ;
#20194=FACE_OUTER_BOUND('',#24508,.T.) ;
#20195=FACE_OUTER_BOUND('',#24509,.T.) ;
#20196=FACE_OUTER_BOUND('',#24510,.T.) ;
#20197=FACE_OUTER_BOUND('',#24511,.T.) ;
#20198=FACE_OUTER_BOUND('',#24512,.T.) ;
#20199=FACE_OUTER_BOUND('',#24513,.T.) ;
#20200=FACE_OUTER_BOUND('',#24514,.T.) ;
#20201=FACE_OUTER_BOUND('',#24515,.T.) ;
#20202=FACE_OUTER_BOUND('',#24516,.T.) ;
#20203=FACE_OUTER_BOUND('',#24517,.T.) ;
#20204=FACE_OUTER_BOUND('',#24518,.T.) ;
#20205=FACE_OUTER_BOUND('',#24519,.T.) ;
#20206=FACE_OUTER_BOUND('',#24520,.T.) ;
#20207=FACE_OUTER_BOUND('',#24521,.T.) ;
#20208=FACE_OUTER_BOUND('',#24522,.T.) ;
#20209=FACE_OUTER_BOUND('',#24523,.T.) ;
#20210=FACE_OUTER_BOUND('',#24524,.T.) ;
#20211=FACE_OUTER_BOUND('',#24525,.T.) ;
#20212=FACE_OUTER_BOUND('',#24526,.T.) ;
#20213=FACE_OUTER_BOUND('',#24527,.T.) ;
#20214=FACE_OUTER_BOUND('',#24528,.T.) ;
#20215=FACE_OUTER_BOUND('',#24529,.T.) ;
#20216=FACE_OUTER_BOUND('',#24530,.T.) ;
#20217=FACE_OUTER_BOUND('',#24531,.T.) ;
#20218=FACE_OUTER_BOUND('',#24532,.T.) ;
#20219=FACE_OUTER_BOUND('',#24533,.T.) ;
#20220=FACE_OUTER_BOUND('',#24534,.T.) ;
#20221=FACE_OUTER_BOUND('',#24535,.T.) ;
#20222=FACE_OUTER_BOUND('',#24536,.T.) ;
#20223=FACE_OUTER_BOUND('',#24537,.T.) ;
#20224=FACE_OUTER_BOUND('',#24538,.T.) ;
#20225=FACE_OUTER_BOUND('',#24539,.T.) ;
#20226=FACE_OUTER_BOUND('',#24540,.T.) ;
#20227=FACE_OUTER_BOUND('',#24541,.T.) ;
#20228=FACE_OUTER_BOUND('',#24542,.T.) ;
#20229=FACE_OUTER_BOUND('',#24543,.T.) ;
#20230=FACE_OUTER_BOUND('',#24544,.T.) ;
#20231=FACE_OUTER_BOUND('',#24545,.T.) ;
#20232=FACE_OUTER_BOUND('',#24546,.T.) ;
#20233=FACE_OUTER_BOUND('',#24547,.T.) ;
#20234=FACE_OUTER_BOUND('',#24548,.T.) ;
#20235=FACE_OUTER_BOUND('',#24549,.T.) ;
#20236=FACE_OUTER_BOUND('',#24550,.T.) ;
#20237=FACE_OUTER_BOUND('',#24551,.T.) ;
#20238=FACE_OUTER_BOUND('',#24552,.T.) ;
#20239=FACE_OUTER_BOUND('',#24553,.T.) ;
#20240=FACE_OUTER_BOUND('',#24554,.T.) ;
#20241=FACE_OUTER_BOUND('',#24555,.T.) ;
#20242=FACE_OUTER_BOUND('',#24556,.T.) ;
#20243=FACE_OUTER_BOUND('',#24557,.T.) ;
#20244=FACE_OUTER_BOUND('',#24558,.T.) ;
#20245=FACE_OUTER_BOUND('',#24559,.T.) ;
#20246=FACE_OUTER_BOUND('',#24560,.T.) ;
#20247=FACE_OUTER_BOUND('',#24561,.T.) ;
#20248=FACE_OUTER_BOUND('',#24562,.T.) ;
#20249=FACE_OUTER_BOUND('',#24563,.T.) ;
#20250=FACE_OUTER_BOUND('',#24564,.T.) ;
#20251=FACE_OUTER_BOUND('',#24565,.T.) ;
#20252=FACE_OUTER_BOUND('',#24566,.T.) ;
#20253=FACE_OUTER_BOUND('',#24567,.T.) ;
#20254=FACE_OUTER_BOUND('',#24568,.T.) ;
#20255=FACE_OUTER_BOUND('',#24569,.T.) ;
#20256=FACE_OUTER_BOUND('',#24570,.T.) ;
#20257=FACE_OUTER_BOUND('',#24571,.T.) ;
#20258=FACE_OUTER_BOUND('',#24572,.T.) ;
#20259=FACE_OUTER_BOUND('',#24573,.T.) ;
#20260=FACE_OUTER_BOUND('',#24574,.T.) ;
#20261=FACE_OUTER_BOUND('',#24575,.T.) ;
#20262=FACE_OUTER_BOUND('',#24576,.T.) ;
#20263=FACE_OUTER_BOUND('',#24577,.T.) ;
#20264=FACE_OUTER_BOUND('',#24578,.T.) ;
#20265=FACE_OUTER_BOUND('',#24579,.T.) ;
#20266=FACE_OUTER_BOUND('',#24580,.T.) ;
#20267=FACE_OUTER_BOUND('',#24581,.T.) ;
#20268=FACE_OUTER_BOUND('',#24582,.T.) ;
#20269=FACE_OUTER_BOUND('',#24583,.T.) ;
#20270=FACE_OUTER_BOUND('',#24584,.T.) ;
#20271=FACE_OUTER_BOUND('',#24585,.T.) ;
#20272=FACE_OUTER_BOUND('',#24586,.T.) ;
#20273=FACE_OUTER_BOUND('',#24587,.T.) ;
#20274=FACE_OUTER_BOUND('',#24588,.T.) ;
#20275=FACE_OUTER_BOUND('',#24589,.T.) ;
#20276=FACE_OUTER_BOUND('',#24590,.T.) ;
#20277=FACE_OUTER_BOUND('',#24591,.T.) ;
#20278=FACE_OUTER_BOUND('',#24592,.T.) ;
#20279=FACE_OUTER_BOUND('',#24593,.T.) ;
#20280=FACE_OUTER_BOUND('',#24594,.T.) ;
#20281=FACE_OUTER_BOUND('',#24595,.T.) ;
#20282=FACE_OUTER_BOUND('',#24596,.T.) ;
#20283=FACE_OUTER_BOUND('',#24597,.T.) ;
#20284=FACE_OUTER_BOUND('',#24598,.T.) ;
#20285=FACE_OUTER_BOUND('',#24599,.T.) ;
#20286=FACE_OUTER_BOUND('',#24600,.T.) ;
#20287=FACE_OUTER_BOUND('',#24601,.T.) ;
#20288=FACE_OUTER_BOUND('',#24602,.T.) ;
#20289=FACE_OUTER_BOUND('',#24603,.T.) ;
#20290=FACE_OUTER_BOUND('',#24604,.T.) ;
#20291=FACE_OUTER_BOUND('',#24605,.T.) ;
#20292=FACE_OUTER_BOUND('',#24606,.T.) ;
#20293=FACE_OUTER_BOUND('',#24607,.T.) ;
#20294=FACE_OUTER_BOUND('',#24608,.T.) ;
#20295=FACE_OUTER_BOUND('',#24609,.T.) ;
#20296=FACE_OUTER_BOUND('',#24610,.T.) ;
#20297=FACE_OUTER_BOUND('',#24611,.T.) ;
#20298=FACE_OUTER_BOUND('',#24612,.T.) ;
#20299=FACE_OUTER_BOUND('',#24613,.T.) ;
#20300=FACE_OUTER_BOUND('',#24614,.T.) ;
#20301=FACE_OUTER_BOUND('',#24615,.T.) ;
#20302=FACE_OUTER_BOUND('',#24616,.T.) ;
#20303=FACE_OUTER_BOUND('',#24617,.T.) ;
#20304=FACE_OUTER_BOUND('',#24618,.T.) ;
#20305=FACE_OUTER_BOUND('',#24619,.T.) ;
#20306=FACE_OUTER_BOUND('',#24620,.T.) ;
#22361=EDGE_LOOP('',(#52858,#52859,#52860,#52861,#52862)) ;
#22362=EDGE_LOOP('',(#52863,#52864,#52865,#52866)) ;
#22363=EDGE_LOOP('',(#52867,#52868,#52869)) ;
#22364=EDGE_LOOP('',(#52870,#52871,#52872,#52873,#52874,#52875,#52876)) ;
#22365=EDGE_LOOP('',(#52877,#52878,#52879,#52880,#52881)) ;
#22366=EDGE_LOOP('',(#52882,#52883,#52884,#52885)) ;
#22367=EDGE_LOOP('',(#52886,#52887,#52888)) ;
#22368=EDGE_LOOP('',(#52889,#52890,#52891,#52892,#52893,#52894,#52895)) ;
#22369=EDGE_LOOP('',(#52896,#52897,#52898,#52899,#52900)) ;
#22370=EDGE_LOOP('',(#52901,#52902,#52903,#52904)) ;
#22371=EDGE_LOOP('',(#52905,#52906,#52907)) ;
#22372=EDGE_LOOP('',(#52908,#52909,#52910,#52911,#52912,#52913,#52914)) ;
#22373=EDGE_LOOP('',(#52915,#52916,#52917,#52918,#52919)) ;
#22374=EDGE_LOOP('',(#52920,#52921,#52922,#52923)) ;
#22375=EDGE_LOOP('',(#52924,#52925,#52926)) ;
#22376=EDGE_LOOP('',(#52927,#52928,#52929,#52930,#52931,#52932,#52933)) ;
#22377=EDGE_LOOP('',(#52934,#52935,#52936,#52937,#52938)) ;
#22378=EDGE_LOOP('',(#52939,#52940,#52941,#52942)) ;
#22379=EDGE_LOOP('',(#52943,#52944,#52945)) ;
#22380=EDGE_LOOP('',(#52946,#52947,#52948,#52949,#52950,#52951,#52952)) ;
#22381=EDGE_LOOP('',(#52953,#52954,#52955,#52956,#52957)) ;
#22382=EDGE_LOOP('',(#52958,#52959,#52960,#52961)) ;
#22383=EDGE_LOOP('',(#52962,#52963,#52964)) ;
#22384=EDGE_LOOP('',(#52965,#52966,#52967,#52968,#52969,#52970,#52971)) ;
#22385=EDGE_LOOP('',(#52972,#52973,#52974,#52975,#52976)) ;
#22386=EDGE_LOOP('',(#52977,#52978,#52979,#52980)) ;
#22387=EDGE_LOOP('',(#52981,#52982,#52983)) ;
#22388=EDGE_LOOP('',(#52984,#52985,#52986,#52987,#52988,#52989,#52990)) ;
#22389=EDGE_LOOP('',(#52991,#52992,#52993,#52994,#52995)) ;
#22390=EDGE_LOOP('',(#52996,#52997,#52998,#52999)) ;
#22391=EDGE_LOOP('',(#53000,#53001,#53002)) ;
#22392=EDGE_LOOP('',(#53003,#53004,#53005,#53006,#53007,#53008,#53009)) ;
#22393=EDGE_LOOP('',(#53010,#53011,#53012,#53013,#53014)) ;
#22394=EDGE_LOOP('',(#53015,#53016,#53017,#53018)) ;
#22395=EDGE_LOOP('',(#53019,#53020,#53021,#53022)) ;
#22396=EDGE_LOOP('',(#53023,#53024,#53025,#53026)) ;
#22397=EDGE_LOOP('',(#53027,#53028,#53029,#53030)) ;
#22398=EDGE_LOOP('',(#53031,#53032,#53033,#53034)) ;
#22399=EDGE_LOOP('',(#53035,#53036,#53037,#53038)) ;
#22400=EDGE_LOOP('',(#53039,#53040,#53041,#53042)) ;
#22401=EDGE_LOOP('',(#53043,#53044,#53045,#53046)) ;
#22402=EDGE_LOOP('',(#53047,#53048,#53049,#53050)) ;
#22403=EDGE_LOOP('',(#53051,#53052,#53053,#53054)) ;
#22404=EDGE_LOOP('',(#53055,#53056,#53057)) ;
#22405=EDGE_LOOP('',(#53058,#53059,#53060,#53061,#53062,#53063,#53064)) ;
#22406=EDGE_LOOP('',(#53065,#53066,#53067,#53068,#53069)) ;
#22407=EDGE_LOOP('',(#53070,#53071,#53072,#53073,#53074)) ;
#22408=EDGE_LOOP('',(#53075,#53076,#53077,#53078,#53079)) ;
#22409=EDGE_LOOP('',(#53080,#53081,#53082,#53083,#53084)) ;
#22410=EDGE_LOOP('',(#53085,#53086,#53087,#53088,#53089)) ;
#22411=EDGE_LOOP('',(#53090,#53091,#53092,#53093,#53094)) ;
#22412=EDGE_LOOP('',(#53095,#53096,#53097,#53098,#53099)) ;
#22413=EDGE_LOOP('',(#53100,#53101,#53102,#53103,#53104)) ;
#22414=EDGE_LOOP('',(#53105,#53106,#53107,#53108,#53109)) ;
#22415=EDGE_LOOP('',(#53110,#53111,#53112,#53113)) ;
#22416=EDGE_LOOP('',(#53114,#53115,#53116,#53117)) ;
#22417=EDGE_LOOP('',(#53118,#53119,#53120,#53121)) ;
#22418=EDGE_LOOP('',(#53122,#53123,#53124,#53125)) ;
#22419=EDGE_LOOP('',(#53126,#53127,#53128,#53129)) ;
#22420=EDGE_LOOP('',(#53130,#53131,#53132,#53133)) ;
#22421=EDGE_LOOP('',(#53134,#53135,#53136,#53137)) ;
#22422=EDGE_LOOP('',(#53138,#53139,#53140,#53141)) ;
#22423=EDGE_LOOP('',(#53142,#53143,#53144,#53145)) ;
#22424=EDGE_LOOP('',(#53146,#53147,#53148,#53149,#53150)) ;
#22425=EDGE_LOOP('',(#53151,#53152,#53153,#53154)) ;
#22426=EDGE_LOOP('',(#53155,#53156,#53157,#53158)) ;
#22427=EDGE_LOOP('',(#53159,#53160,#53161)) ;
#22428=EDGE_LOOP('',(#53162,#53163,#53164,#53165,#53166,#53167,#53168)) ;
#22429=EDGE_LOOP('',(#53169,#53170,#53171,#53172,#53173)) ;
#22430=EDGE_LOOP('',(#53174,#53175,#53176,#53177)) ;
#22431=EDGE_LOOP('',(#53178,#53179,#53180,#53181,#53182,#53183,#53184,#53185,
#53186,#53187,#53188,#53189)) ;
#22432=EDGE_LOOP('',(#53190,#53191,#53192,#53193,#53194,#53195,#53196,#53197,
#53198,#53199,#53200,#53201)) ;
#22433=EDGE_LOOP('',(#53202,#53203,#53204,#53205,#53206,#53207,#53208,#53209,
#53210,#53211,#53212,#53213)) ;
#22434=EDGE_LOOP('',(#53214,#53215,#53216,#53217,#53218,#53219,#53220,#53221,
#53222,#53223,#53224,#53225)) ;
#22435=EDGE_LOOP('',(#53226,#53227,#53228,#53229,#53230,#53231,#53232,#53233,
#53234,#53235,#53236,#53237)) ;
#22436=EDGE_LOOP('',(#53238,#53239,#53240,#53241,#53242,#53243,#53244,#53245,
#53246,#53247,#53248,#53249)) ;
#22437=EDGE_LOOP('',(#53250,#53251,#53252,#53253,#53254,#53255,#53256,#53257,
#53258,#53259,#53260,#53261)) ;
#22438=EDGE_LOOP('',(#53262,#53263,#53264,#53265,#53266,#53267,#53268,#53269,
#53270,#53271,#53272,#53273)) ;
#22439=EDGE_LOOP('',(#53274,#53275,#53276,#53277,#53278,#53279,#53280,#53281,
#53282,#53283,#53284,#53285)) ;
#22440=EDGE_LOOP('',(#53286,#53287,#53288,#53289,#53290)) ;
#22441=EDGE_LOOP('',(#53291,#53292,#53293,#53294,#53295)) ;
#22442=EDGE_LOOP('',(#53296,#53297,#53298,#53299,#53300)) ;
#22443=EDGE_LOOP('',(#53301,#53302,#53303,#53304,#53305)) ;
#22444=EDGE_LOOP('',(#53306,#53307,#53308,#53309,#53310)) ;
#22445=EDGE_LOOP('',(#53311,#53312,#53313,#53314,#53315)) ;
#22446=EDGE_LOOP('',(#53316,#53317,#53318,#53319,#53320)) ;
#22447=EDGE_LOOP('',(#53321,#53322,#53323,#53324,#53325)) ;
#22448=EDGE_LOOP('',(#53326,#53327,#53328,#53329,#53330)) ;
#22449=EDGE_LOOP('',(#53331,#53332,#53333,#53334,#53335)) ;
#22450=EDGE_LOOP('',(#53336,#53337,#53338,#53339,#53340)) ;
#22451=EDGE_LOOP('',(#53341,#53342,#53343,#53344,#53345)) ;
#22452=EDGE_LOOP('',(#53346,#53347,#53348,#53349,#53350)) ;
#22453=EDGE_LOOP('',(#53351,#53352,#53353,#53354,#53355)) ;
#22454=EDGE_LOOP('',(#53356,#53357,#53358,#53359,#53360)) ;
#22455=EDGE_LOOP('',(#53361,#53362,#53363,#53364,#53365)) ;
#22456=EDGE_LOOP('',(#53366,#53367,#53368,#53369,#53370)) ;
#22457=EDGE_LOOP('',(#53371,#53372,#53373,#53374,#53375)) ;
#22458=EDGE_LOOP('',(#53376,#53377,#53378,#53379)) ;
#22459=EDGE_LOOP('',(#53380,#53381,#53382,#53383)) ;
#22460=EDGE_LOOP('',(#53384,#53385,#53386,#53387)) ;
#22461=EDGE_LOOP('',(#53388,#53389,#53390,#53391)) ;
#22462=EDGE_LOOP('',(#53392,#53393,#53394,#53395)) ;
#22463=EDGE_LOOP('',(#53396,#53397,#53398,#53399)) ;
#22464=EDGE_LOOP('',(#53400,#53401,#53402,#53403)) ;
#22465=EDGE_LOOP('',(#53404,#53405,#53406,#53407)) ;
#22466=EDGE_LOOP('',(#53408,#53409,#53410,#53411)) ;
#22467=EDGE_LOOP('',(#53412,#53413,#53414,#53415,#53416,#53417,#53418,#53419,
#53420,#53421,#53422,#53423)) ;
#22468=EDGE_LOOP('',(#53424,#53425,#53426,#53427,#53428)) ;
#22469=EDGE_LOOP('',(#53429,#53430,#53431,#53432,#53433)) ;
#22470=EDGE_LOOP('',(#53434,#53435,#53436,#53437)) ;
#22471=EDGE_LOOP('',(#53438,#53439,#53440,#53441)) ;
#22472=EDGE_LOOP('',(#53442,#53443,#53444,#53445,#53446,#53447,#53448,#53449,
#53450,#53451,#53452,#53453,#53454,#53455,#53456,#53457,#53458,#53459,#53460,
#53461,#53462,#53463,#53464,#53465,#53466,#53467,#53468,#53469,#53470,#53471,
#53472,#53473,#53474,#53475,#53476,#53477,#53478,#53479,#53480,#53481,#53482,
#53483,#53484,#53485,#53486,#53487,#53488,#53489,#53490,#53491,#53492,#53493,
#53494,#53495,#53496,#53497,#53498,#53499,#53500,#53501,#53502,#53503,#53504,
#53505)) ;
#22473=EDGE_LOOP('',(#53506,#53507,#53508,#53509)) ;
#22474=EDGE_LOOP('',(#53510,#53511,#53512,#53513,#53514,#53515,#53516,#53517,
#53518,#53519,#53520,#53521,#53522,#53523,#53524,#53525,#53526,#53527,#53528,
#53529,#53530,#53531,#53532,#53533,#53534,#53535,#53536,#53537,#53538,#53539,
#53540,#53541,#53542,#53543,#53544,#53545,#53546,#53547,#53548,#53549,#53550,
#53551,#53552,#53553,#53554,#53555,#53556,#53557,#53558,#53559,#53560,#53561,
#53562,#53563,#53564,#53565,#53566,#53567,#53568,#53569,#53570,#53571,#53572,
#53573)) ;
#22475=EDGE_LOOP('',(#53574,#53575,#53576,#53577)) ;
#22476=EDGE_LOOP('',(#53578,#53579,#53580,#53581)) ;
#22477=EDGE_LOOP('',(#53582,#53583,#53584,#53585)) ;
#22478=EDGE_LOOP('',(#53586,#53587,#53588,#53589)) ;
#22479=EDGE_LOOP('',(#53590,#53591,#53592,#53593)) ;
#22480=EDGE_LOOP('',(#53594,#53595,#53596,#53597)) ;
#22481=EDGE_LOOP('',(#53598,#53599,#53600,#53601)) ;
#22482=EDGE_LOOP('',(#53602,#53603,#53604,#53605)) ;
#22483=EDGE_LOOP('',(#53606,#53607,#53608,#53609)) ;
#22484=EDGE_LOOP('',(#53610,#53611,#53612,#53613)) ;
#22485=EDGE_LOOP('',(#53614,#53615,#53616,#53617)) ;
#22486=EDGE_LOOP('',(#53618,#53619,#53620,#53621)) ;
#22487=EDGE_LOOP('',(#53622,#53623,#53624,#53625,#53626,#53627,#53628,#53629,
#53630,#53631,#53632,#53633,#53634,#53635,#53636,#53637,#53638,#53639,#53640,
#53641,#53642,#53643,#53644,#53645)) ;
#22488=EDGE_LOOP('',(#53646,#53647,#53648,#53649,#53650,#53651,#53652,#53653,
#53654,#53655,#53656,#53657,#53658,#53659,#53660,#53661,#53662,#53663,#53664,
#53665,#53666,#53667,#53668,#53669)) ;
#22489=EDGE_LOOP('',(#53670,#53671,#53672,#53673,#53674,#53675,#53676,#53677,
#53678,#53679,#53680,#53681,#53682,#53683,#53684,#53685,#53686,#53687,#53688,
#53689,#53690,#53691,#53692,#53693)) ;
#22490=EDGE_LOOP('',(#53694,#53695,#53696,#53697,#53698,#53699,#53700,#53701,
#53702,#53703,#53704,#53705,#53706,#53707,#53708,#53709,#53710,#53711,#53712,
#53713,#53714,#53715,#53716,#53717)) ;
#22491=EDGE_LOOP('',(#53718,#53719,#53720,#53721,#53722,#53723,#53724,#53725,
#53726,#53727,#53728,#53729,#53730,#53731,#53732,#53733,#53734,#53735,#53736,
#53737,#53738,#53739,#53740,#53741)) ;
#22492=EDGE_LOOP('',(#53742,#53743,#53744,#53745,#53746,#53747,#53748,#53749,
#53750,#53751,#53752,#53753,#53754,#53755,#53756,#53757,#53758,#53759,#53760,
#53761,#53762,#53763,#53764,#53765)) ;
#22493=EDGE_LOOP('',(#53766,#53767,#53768,#53769,#53770,#53771,#53772,#53773,
#53774,#53775,#53776,#53777,#53778,#53779,#53780,#53781,#53782,#53783,#53784,
#53785,#53786,#53787,#53788,#53789)) ;
#22494=EDGE_LOOP('',(#53790,#53791,#53792,#53793,#53794,#53795,#53796,#53797,
#53798,#53799,#53800,#53801,#53802,#53803,#53804,#53805,#53806,#53807,#53808,
#53809,#53810,#53811,#53812,#53813)) ;
#22495=EDGE_LOOP('',(#53814,#53815,#53816,#53817,#53818,#53819,#53820,#53821,
#53822,#53823,#53824,#53825,#53826,#53827,#53828,#53829,#53830,#53831,#53832,
#53833,#53834,#53835,#53836,#53837)) ;
#22496=EDGE_LOOP('',(#53838,#53839,#53840,#53841,#53842,#53843,#53844,#53845,
#53846,#53847,#53848,#53849,#53850,#53851,#53852,#53853,#53854,#53855,#53856,
#53857,#53858,#53859,#53860,#53861)) ;
#22497=EDGE_LOOP('',(#53862,#53863,#53864,#53865,#53866,#53867,#53868,#53869,
#53870,#53871)) ;
#22498=EDGE_LOOP('',(#53872,#53873,#53874,#53875,#53876,#53877,#53878,#53879,
#53880,#53881)) ;
#22499=EDGE_LOOP('',(#53882,#53883,#53884,#53885,#53886,#53887,#53888,#53889,
#53890,#53891)) ;
#22500=EDGE_LOOP('',(#53892,#53893,#53894,#53895)) ;
#22501=EDGE_LOOP('',(#53896,#53897,#53898,#53899)) ;
#22502=EDGE_LOOP('',(#53900,#53901,#53902,#53903)) ;
#22503=EDGE_LOOP('',(#53904,#53905,#53906,#53907)) ;
#22504=EDGE_LOOP('',(#53908,#53909,#53910,#53911)) ;
#22505=EDGE_LOOP('',(#53912,#53913,#53914,#53915)) ;
#22506=EDGE_LOOP('',(#53916,#53917,#53918,#53919)) ;
#22507=EDGE_LOOP('',(#53920,#53921,#53922,#53923)) ;
#22508=EDGE_LOOP('',(#53924,#53925,#53926,#53927)) ;
#22509=EDGE_LOOP('',(#53928,#53929,#53930,#53931)) ;
#22510=EDGE_LOOP('',(#53932,#53933,#53934,#53935)) ;
#22511=EDGE_LOOP('',(#53936,#53937,#53938,#53939)) ;
#22512=EDGE_LOOP('',(#53940,#53941,#53942,#53943)) ;
#22513=EDGE_LOOP('',(#53944,#53945,#53946,#53947)) ;
#22514=EDGE_LOOP('',(#53948,#53949,#53950,#53951)) ;
#22515=EDGE_LOOP('',(#53952,#53953,#53954,#53955)) ;
#22516=EDGE_LOOP('',(#53956,#53957,#53958,#53959)) ;
#22517=EDGE_LOOP('',(#53960,#53961,#53962,#53963)) ;
#22518=EDGE_LOOP('',(#53964,#53965,#53966,#53967)) ;
#22519=EDGE_LOOP('',(#53968,#53969,#53970,#53971)) ;
#22520=EDGE_LOOP('',(#53972,#53973,#53974,#53975)) ;
#22521=EDGE_LOOP('',(#53976,#53977,#53978,#53979)) ;
#22522=EDGE_LOOP('',(#53980,#53981,#53982,#53983)) ;
#22523=EDGE_LOOP('',(#53984,#53985,#53986,#53987)) ;
#22524=EDGE_LOOP('',(#53988,#53989,#53990,#53991)) ;
#22525=EDGE_LOOP('',(#53992,#53993,#53994,#53995)) ;
#22526=EDGE_LOOP('',(#53996,#53997,#53998,#53999)) ;
#22527=EDGE_LOOP('',(#54000,#54001,#54002,#54003)) ;
#22528=EDGE_LOOP('',(#54004,#54005,#54006,#54007)) ;
#22529=EDGE_LOOP('',(#54008,#54009,#54010,#54011)) ;
#22530=EDGE_LOOP('',(#54012,#54013,#54014,#54015)) ;
#22531=EDGE_LOOP('',(#54016,#54017,#54018,#54019)) ;
#22532=EDGE_LOOP('',(#54020,#54021,#54022,#54023,#54024,#54025,#54026,#54027,
#54028,#54029,#54030,#54031,#54032,#54033,#54034,#54035,#54036,#54037)) ;
#22533=EDGE_LOOP('',(#54038)) ;
#22534=EDGE_LOOP('',(#54039)) ;
#22535=EDGE_LOOP('',(#54040,#54041,#54042,#54043,#54044,#54045,#54046,#54047)) ;
#22536=EDGE_LOOP('',(#54048,#54049,#54050,#54051)) ;
#22537=EDGE_LOOP('',(#54052,#54053,#54054,#54055)) ;
#22538=EDGE_LOOP('',(#54056,#54057,#54058)) ;
#22539=EDGE_LOOP('',(#54059,#54060,#54061)) ;
#22540=EDGE_LOOP('',(#54062,#54063,#54064,#54065)) ;
#22541=EDGE_LOOP('',(#54066,#54067,#54068,#54069,#54070,#54071)) ;
#22542=EDGE_LOOP('',(#54072,#54073,#54074,#54075,#54076,#54077,#54078)) ;
#22543=EDGE_LOOP('',(#54079,#54080,#54081,#54082)) ;
#22544=EDGE_LOOP('',(#54083,#54084,#54085,#54086)) ;
#22545=EDGE_LOOP('',(#54087,#54088,#54089,#54090)) ;
#22546=EDGE_LOOP('',(#54091,#54092,#54093,#54094)) ;
#22547=EDGE_LOOP('',(#54095,#54096,#54097)) ;
#22548=EDGE_LOOP('',(#54098,#54099,#54100,#54101)) ;
#22549=EDGE_LOOP('',(#54102,#54103,#54104,#54105)) ;
#22550=EDGE_LOOP('',(#54106,#54107,#54108,#54109)) ;
#22551=EDGE_LOOP('',(#54110,#54111,#54112,#54113)) ;
#22552=EDGE_LOOP('',(#54114,#54115,#54116,#54117)) ;
#22553=EDGE_LOOP('',(#54118,#54119,#54120,#54121)) ;
#22554=EDGE_LOOP('',(#54122,#54123,#54124,#54125)) ;
#22555=EDGE_LOOP('',(#54126,#54127,#54128,#54129)) ;
#22556=EDGE_LOOP('',(#54130,#54131,#54132,#54133)) ;
#22557=EDGE_LOOP('',(#54134,#54135,#54136)) ;
#22558=EDGE_LOOP('',(#54137,#54138,#54139)) ;
#22559=EDGE_LOOP('',(#54140,#54141,#54142,#54143,#54144)) ;
#22560=EDGE_LOOP('',(#54145,#54146,#54147)) ;
#22561=EDGE_LOOP('',(#54148,#54149,#54150)) ;
#22562=EDGE_LOOP('',(#54151,#54152,#54153,#54154)) ;
#22563=EDGE_LOOP('',(#54155,#54156,#54157,#54158)) ;
#22564=EDGE_LOOP('',(#54159,#54160,#54161,#54162)) ;
#22565=EDGE_LOOP('',(#54163,#54164,#54165,#54166)) ;
#22566=EDGE_LOOP('',(#54167,#54168,#54169,#54170)) ;
#22567=EDGE_LOOP('',(#54171,#54172,#54173,#54174)) ;
#22568=EDGE_LOOP('',(#54175,#54176,#54177,#54178)) ;
#22569=EDGE_LOOP('',(#54179,#54180,#54181)) ;
#22570=EDGE_LOOP('',(#54182,#54183,#54184,#54185)) ;
#22571=EDGE_LOOP('',(#54186,#54187,#54188,#54189)) ;
#22572=EDGE_LOOP('',(#54190,#54191,#54192)) ;
#22573=EDGE_LOOP('',(#54193,#54194,#54195,#54196)) ;
#22574=EDGE_LOOP('',(#54197,#54198,#54199,#54200)) ;
#22575=EDGE_LOOP('',(#54201,#54202,#54203,#54204)) ;
#22576=EDGE_LOOP('',(#54205,#54206,#54207,#54208)) ;
#22577=EDGE_LOOP('',(#54209,#54210,#54211,#54212)) ;
#22578=EDGE_LOOP('',(#54213,#54214,#54215,#54216)) ;
#22579=EDGE_LOOP('',(#54217,#54218,#54219,#54220,#54221)) ;
#22580=EDGE_LOOP('',(#54222,#54223,#54224,#54225)) ;
#22581=EDGE_LOOP('',(#54226,#54227,#54228)) ;
#22582=EDGE_LOOP('',(#54229,#54230,#54231)) ;
#22583=EDGE_LOOP('',(#54232,#54233,#54234,#54235)) ;
#22584=EDGE_LOOP('',(#54236,#54237,#54238,#54239)) ;
#22585=EDGE_LOOP('',(#54240,#54241,#54242,#54243)) ;
#22586=EDGE_LOOP('',(#54244,#54245,#54246)) ;
#22587=EDGE_LOOP('',(#54247,#54248,#54249,#54250)) ;
#22588=EDGE_LOOP('',(#54251,#54252,#54253,#54254)) ;
#22589=EDGE_LOOP('',(#54255,#54256,#54257)) ;
#22590=EDGE_LOOP('',(#54258,#54259,#54260,#54261)) ;
#22591=EDGE_LOOP('',(#54262,#54263,#54264,#54265)) ;
#22592=EDGE_LOOP('',(#54266,#54267,#54268,#54269)) ;
#22593=EDGE_LOOP('',(#54270,#54271,#54272)) ;
#22594=EDGE_LOOP('',(#54273,#54274,#54275)) ;
#22595=EDGE_LOOP('',(#54276,#54277,#54278,#54279)) ;
#22596=EDGE_LOOP('',(#54280,#54281,#54282,#54283)) ;
#22597=EDGE_LOOP('',(#54284,#54285,#54286)) ;
#22598=EDGE_LOOP('',(#54287,#54288,#54289)) ;
#22599=EDGE_LOOP('',(#54290,#54291,#54292,#54293)) ;
#22600=EDGE_LOOP('',(#54294,#54295,#54296,#54297)) ;
#22601=EDGE_LOOP('',(#54298,#54299,#54300,#54301)) ;
#22602=EDGE_LOOP('',(#54302,#54303,#54304)) ;
#22603=EDGE_LOOP('',(#54305,#54306,#54307,#54308)) ;
#22604=EDGE_LOOP('',(#54309,#54310,#54311,#54312)) ;
#22605=EDGE_LOOP('',(#54313,#54314,#54315)) ;
#22606=EDGE_LOOP('',(#54316,#54317,#54318,#54319)) ;
#22607=EDGE_LOOP('',(#54320,#54321,#54322,#54323)) ;
#22608=EDGE_LOOP('',(#54324,#54325,#54326,#54327)) ;
#22609=EDGE_LOOP('',(#54328,#54329,#54330)) ;
#22610=EDGE_LOOP('',(#54331,#54332,#54333)) ;
#22611=EDGE_LOOP('',(#54334,#54335,#54336,#54337)) ;
#22612=EDGE_LOOP('',(#54338,#54339,#54340,#54341)) ;
#22613=EDGE_LOOP('',(#54342,#54343,#54344)) ;
#22614=EDGE_LOOP('',(#54345,#54346,#54347,#54348)) ;
#22615=EDGE_LOOP('',(#54349,#54350,#54351,#54352)) ;
#22616=EDGE_LOOP('',(#54353,#54354,#54355)) ;
#22617=EDGE_LOOP('',(#54356,#54357,#54358,#54359)) ;
#22618=EDGE_LOOP('',(#54360,#54361,#54362,#54363)) ;
#22619=EDGE_LOOP('',(#54364,#54365,#54366,#54367)) ;
#22620=EDGE_LOOP('',(#54368,#54369,#54370)) ;
#22621=EDGE_LOOP('',(#54371,#54372,#54373,#54374)) ;
#22622=EDGE_LOOP('',(#54375,#54376,#54377,#54378)) ;
#22623=EDGE_LOOP('',(#54379,#54380,#54381)) ;
#22624=EDGE_LOOP('',(#54382,#54383,#54384)) ;
#22625=EDGE_LOOP('',(#54385,#54386,#54387,#54388)) ;
#22626=EDGE_LOOP('',(#54389,#54390,#54391,#54392)) ;
#22627=EDGE_LOOP('',(#54393,#54394,#54395)) ;
#22628=EDGE_LOOP('',(#54396,#54397,#54398)) ;
#22629=EDGE_LOOP('',(#54399,#54400,#54401,#54402)) ;
#22630=EDGE_LOOP('',(#54403,#54404,#54405,#54406)) ;
#22631=EDGE_LOOP('',(#54407,#54408,#54409)) ;
#22632=EDGE_LOOP('',(#54410,#54411,#54412,#54413)) ;
#22633=EDGE_LOOP('',(#54414,#54415,#54416,#54417)) ;
#22634=EDGE_LOOP('',(#54418,#54419,#54420)) ;
#22635=EDGE_LOOP('',(#54421,#54422,#54423)) ;
#22636=EDGE_LOOP('',(#54424,#54425,#54426,#54427)) ;
#22637=EDGE_LOOP('',(#54428,#54429,#54430,#54431)) ;
#22638=EDGE_LOOP('',(#54432,#54433,#54434,#54435)) ;
#22639=EDGE_LOOP('',(#54436,#54437,#54438,#54439)) ;
#22640=EDGE_LOOP('',(#54440,#54441,#54442,#54443)) ;
#22641=EDGE_LOOP('',(#54444,#54445,#54446,#54447)) ;
#22642=EDGE_LOOP('',(#54448,#54449,#54450)) ;
#22643=EDGE_LOOP('',(#54451,#54452,#54453)) ;
#22644=EDGE_LOOP('',(#54454,#54455,#54456,#54457)) ;
#22645=EDGE_LOOP('',(#54458,#54459,#54460,#54461)) ;
#22646=EDGE_LOOP('',(#54462,#54463,#54464,#54465)) ;
#22647=EDGE_LOOP('',(#54466,#54467,#54468,#54469)) ;
#22648=EDGE_LOOP('',(#54470,#54471,#54472,#54473)) ;
#22649=EDGE_LOOP('',(#54474,#54475,#54476,#54477)) ;
#22650=EDGE_LOOP('',(#54478,#54479,#54480,#54481)) ;
#22651=EDGE_LOOP('',(#54482,#54483,#54484,#54485)) ;
#22652=EDGE_LOOP('',(#54486,#54487,#54488,#54489)) ;
#22653=EDGE_LOOP('',(#54490,#54491,#54492,#54493)) ;
#22654=EDGE_LOOP('',(#54494,#54495,#54496,#54497)) ;
#22655=EDGE_LOOP('',(#54498,#54499,#54500,#54501)) ;
#22656=EDGE_LOOP('',(#54502,#54503,#54504,#54505)) ;
#22657=EDGE_LOOP('',(#54506,#54507,#54508,#54509)) ;
#22658=EDGE_LOOP('',(#54510,#54511,#54512,#54513)) ;
#22659=EDGE_LOOP('',(#54514,#54515,#54516,#54517)) ;
#22660=EDGE_LOOP('',(#54518,#54519,#54520,#54521)) ;
#22661=EDGE_LOOP('',(#54522,#54523,#54524)) ;
#22662=EDGE_LOOP('',(#54525,#54526,#54527,#54528)) ;
#22663=EDGE_LOOP('',(#54529,#54530,#54531,#54532)) ;
#22664=EDGE_LOOP('',(#54533,#54534,#54535,#54536)) ;
#22665=EDGE_LOOP('',(#54537,#54538,#54539)) ;
#22666=EDGE_LOOP('',(#54540,#54541,#54542,#54543)) ;
#22667=EDGE_LOOP('',(#54544,#54545,#54546,#54547)) ;
#22668=EDGE_LOOP('',(#54548,#54549,#54550,#54551)) ;
#22669=EDGE_LOOP('',(#54552,#54553,#54554,#54555)) ;
#22670=EDGE_LOOP('',(#54556,#54557,#54558,#54559)) ;
#22671=EDGE_LOOP('',(#54560,#54561,#54562,#54563)) ;
#22672=EDGE_LOOP('',(#54564,#54565,#54566,#54567)) ;
#22673=EDGE_LOOP('',(#54568,#54569,#54570,#54571,#54572,#54573)) ;
#22674=EDGE_LOOP('',(#54574,#54575,#54576,#54577,#54578,#54579)) ;
#22675=EDGE_LOOP('',(#54580,#54581,#54582,#54583,#54584)) ;
#22676=EDGE_LOOP('',(#54585,#54586,#54587,#54588)) ;
#22677=EDGE_LOOP('',(#54589,#54590,#54591,#54592)) ;
#22678=EDGE_LOOP('',(#54593,#54594,#54595,#54596)) ;
#22679=EDGE_LOOP('',(#54597,#54598,#54599,#54600)) ;
#22680=EDGE_LOOP('',(#54601,#54602,#54603,#54604)) ;
#22681=EDGE_LOOP('',(#54605,#54606,#54607,#54608)) ;
#22682=EDGE_LOOP('',(#54609,#54610,#54611,#54612)) ;
#22683=EDGE_LOOP('',(#54613,#54614,#54615,#54616)) ;
#22684=EDGE_LOOP('',(#54617,#54618,#54619,#54620)) ;
#22685=EDGE_LOOP('',(#54621,#54622,#54623,#54624)) ;
#22686=EDGE_LOOP('',(#54625,#54626,#54627,#54628)) ;
#22687=EDGE_LOOP('',(#54629,#54630,#54631,#54632)) ;
#22688=EDGE_LOOP('',(#54633,#54634,#54635,#54636)) ;
#22689=EDGE_LOOP('',(#54637,#54638,#54639,#54640)) ;
#22690=EDGE_LOOP('',(#54641,#54642,#54643)) ;
#22691=EDGE_LOOP('',(#54644,#54645,#54646,#54647)) ;
#22692=EDGE_LOOP('',(#54648,#54649,#54650,#54651)) ;
#22693=EDGE_LOOP('',(#54652,#54653,#54654,#54655)) ;
#22694=EDGE_LOOP('',(#54656,#54657,#54658)) ;
#22695=EDGE_LOOP('',(#54659,#54660,#54661)) ;
#22696=EDGE_LOOP('',(#54662,#54663,#54664,#54665)) ;
#22697=EDGE_LOOP('',(#54666,#54667,#54668,#54669)) ;
#22698=EDGE_LOOP('',(#54670,#54671,#54672,#54673)) ;
#22699=EDGE_LOOP('',(#54674,#54675,#54676)) ;
#22700=EDGE_LOOP('',(#54677,#54678,#54679,#54680)) ;
#22701=EDGE_LOOP('',(#54681,#54682,#54683,#54684)) ;
#22702=EDGE_LOOP('',(#54685,#54686,#54687,#54688)) ;
#22703=EDGE_LOOP('',(#54689,#54690,#54691,#54692)) ;
#22704=EDGE_LOOP('',(#54693,#54694,#54695)) ;
#22705=EDGE_LOOP('',(#54696,#54697,#54698,#54699)) ;
#22706=EDGE_LOOP('',(#54700,#54701,#54702,#54703)) ;
#22707=EDGE_LOOP('',(#54704,#54705,#54706,#54707)) ;
#22708=EDGE_LOOP('',(#54708,#54709,#54710)) ;
#22709=EDGE_LOOP('',(#54711,#54712,#54713)) ;
#22710=EDGE_LOOP('',(#54714,#54715,#54716,#54717)) ;
#22711=EDGE_LOOP('',(#54718,#54719,#54720,#54721)) ;
#22712=EDGE_LOOP('',(#54722,#54723,#54724,#54725)) ;
#22713=EDGE_LOOP('',(#54726,#54727,#54728)) ;
#22714=EDGE_LOOP('',(#54729,#54730,#54731,#54732)) ;
#22715=EDGE_LOOP('',(#54733,#54734,#54735,#54736)) ;
#22716=EDGE_LOOP('',(#54737,#54738,#54739,#54740)) ;
#22717=EDGE_LOOP('',(#54741,#54742,#54743,#54744)) ;
#22718=EDGE_LOOP('',(#54745,#54746,#54747,#54748)) ;
#22719=EDGE_LOOP('',(#54749,#54750,#54751,#54752)) ;
#22720=EDGE_LOOP('',(#54753,#54754,#54755,#54756)) ;
#22721=EDGE_LOOP('',(#54757,#54758,#54759,#54760)) ;
#22722=EDGE_LOOP('',(#54761,#54762,#54763,#54764,#54765)) ;
#22723=EDGE_LOOP('',(#54766,#54767,#54768,#54769)) ;
#22724=EDGE_LOOP('',(#54770,#54771,#54772,#54773)) ;
#22725=EDGE_LOOP('',(#54774,#54775,#54776,#54777)) ;
#22726=EDGE_LOOP('',(#54778,#54779,#54780,#54781)) ;
#22727=EDGE_LOOP('',(#54782,#54783,#54784,#54785)) ;
#22728=EDGE_LOOP('',(#54786,#54787,#54788,#54789)) ;
#22729=EDGE_LOOP('',(#54790,#54791,#54792,#54793)) ;
#22730=EDGE_LOOP('',(#54794,#54795,#54796,#54797)) ;
#22731=EDGE_LOOP('',(#54798,#54799,#54800,#54801)) ;
#22732=EDGE_LOOP('',(#54802,#54803,#54804,#54805)) ;
#22733=EDGE_LOOP('',(#54806,#54807,#54808,#54809)) ;
#22734=EDGE_LOOP('',(#54810,#54811,#54812,#54813)) ;
#22735=EDGE_LOOP('',(#54814,#54815,#54816,#54817)) ;
#22736=EDGE_LOOP('',(#54818,#54819,#54820,#54821)) ;
#22737=EDGE_LOOP('',(#54822,#54823,#54824,#54825)) ;
#22738=EDGE_LOOP('',(#54826,#54827,#54828,#54829)) ;
#22739=EDGE_LOOP('',(#54830,#54831,#54832,#54833)) ;
#22740=EDGE_LOOP('',(#54834,#54835,#54836,#54837,#54838,#54839,#54840,#54841,
#54842,#54843)) ;
#22741=EDGE_LOOP('',(#54844,#54845,#54846,#54847,#54848,#54849,#54850,#54851,
#54852,#54853)) ;
#22742=EDGE_LOOP('',(#54854,#54855,#54856,#54857,#54858,#54859,#54860,#54861,
#54862,#54863)) ;
#22743=EDGE_LOOP('',(#54864,#54865,#54866,#54867,#54868,#54869,#54870,#54871,
#54872,#54873)) ;
#22744=EDGE_LOOP('',(#54874,#54875,#54876,#54877,#54878,#54879,#54880,#54881,
#54882,#54883)) ;
#22745=EDGE_LOOP('',(#54884,#54885,#54886,#54887,#54888,#54889,#54890,#54891,
#54892,#54893)) ;
#22746=EDGE_LOOP('',(#54894,#54895,#54896,#54897,#54898,#54899,#54900,#54901,
#54902,#54903)) ;
#22747=EDGE_LOOP('',(#54904,#54905,#54906,#54907,#54908,#54909,#54910,#54911,
#54912,#54913)) ;
#22748=EDGE_LOOP('',(#54914,#54915,#54916,#54917,#54918,#54919,#54920,#54921,
#54922,#54923)) ;
#22749=EDGE_LOOP('',(#54924,#54925,#54926,#54927)) ;
#22750=EDGE_LOOP('',(#54928,#54929,#54930,#54931)) ;
#22751=EDGE_LOOP('',(#54932,#54933,#54934,#54935)) ;
#22752=EDGE_LOOP('',(#54936,#54937,#54938,#54939)) ;
#22753=EDGE_LOOP('',(#54940,#54941,#54942,#54943)) ;
#22754=EDGE_LOOP('',(#54944,#54945,#54946,#54947)) ;
#22755=EDGE_LOOP('',(#54948,#54949,#54950,#54951)) ;
#22756=EDGE_LOOP('',(#54952,#54953,#54954,#54955)) ;
#22757=EDGE_LOOP('',(#54956,#54957,#54958,#54959)) ;
#22758=EDGE_LOOP('',(#54960,#54961,#54962,#54963)) ;
#22759=EDGE_LOOP('',(#54964,#54965,#54966,#54967)) ;
#22760=EDGE_LOOP('',(#54968,#54969,#54970,#54971)) ;
#22761=EDGE_LOOP('',(#54972,#54973,#54974,#54975)) ;
#22762=EDGE_LOOP('',(#54976,#54977,#54978,#54979)) ;
#22763=EDGE_LOOP('',(#54980,#54981,#54982,#54983)) ;
#22764=EDGE_LOOP('',(#54984,#54985,#54986,#54987)) ;
#22765=EDGE_LOOP('',(#54988,#54989,#54990,#54991)) ;
#22766=EDGE_LOOP('',(#54992,#54993,#54994,#54995)) ;
#22767=EDGE_LOOP('',(#54996,#54997,#54998,#54999)) ;
#22768=EDGE_LOOP('',(#55000,#55001,#55002,#55003)) ;
#22769=EDGE_LOOP('',(#55004,#55005,#55006,#55007)) ;
#22770=EDGE_LOOP('',(#55008,#55009,#55010,#55011)) ;
#22771=EDGE_LOOP('',(#55012,#55013,#55014,#55015)) ;
#22772=EDGE_LOOP('',(#55016,#55017,#55018,#55019)) ;
#22773=EDGE_LOOP('',(#55020,#55021,#55022,#55023)) ;
#22774=EDGE_LOOP('',(#55024,#55025,#55026,#55027)) ;
#22775=EDGE_LOOP('',(#55028,#55029,#55030,#55031)) ;
#22776=EDGE_LOOP('',(#55032,#55033,#55034,#55035)) ;
#22777=EDGE_LOOP('',(#55036,#55037,#55038,#55039)) ;
#22778=EDGE_LOOP('',(#55040,#55041,#55042,#55043)) ;
#22779=EDGE_LOOP('',(#55044,#55045,#55046,#55047)) ;
#22780=EDGE_LOOP('',(#55048,#55049,#55050,#55051)) ;
#22781=EDGE_LOOP('',(#55052,#55053,#55054,#55055)) ;
#22782=EDGE_LOOP('',(#55056,#55057,#55058,#55059)) ;
#22783=EDGE_LOOP('',(#55060,#55061,#55062,#55063)) ;
#22784=EDGE_LOOP('',(#55064,#55065,#55066,#55067)) ;
#22785=EDGE_LOOP('',(#55068,#55069,#55070,#55071)) ;
#22786=EDGE_LOOP('',(#55072,#55073,#55074,#55075)) ;
#22787=EDGE_LOOP('',(#55076,#55077,#55078,#55079)) ;
#22788=EDGE_LOOP('',(#55080,#55081,#55082,#55083)) ;
#22789=EDGE_LOOP('',(#55084,#55085,#55086,#55087)) ;
#22790=EDGE_LOOP('',(#55088,#55089,#55090,#55091)) ;
#22791=EDGE_LOOP('',(#55092,#55093,#55094,#55095)) ;
#22792=EDGE_LOOP('',(#55096,#55097,#55098,#55099)) ;
#22793=EDGE_LOOP('',(#55100,#55101,#55102,#55103)) ;
#22794=EDGE_LOOP('',(#55104,#55105,#55106,#55107)) ;
#22795=EDGE_LOOP('',(#55108,#55109,#55110,#55111)) ;
#22796=EDGE_LOOP('',(#55112,#55113,#55114,#55115)) ;
#22797=EDGE_LOOP('',(#55116,#55117,#55118,#55119)) ;
#22798=EDGE_LOOP('',(#55120,#55121,#55122,#55123)) ;
#22799=EDGE_LOOP('',(#55124,#55125,#55126,#55127)) ;
#22800=EDGE_LOOP('',(#55128,#55129,#55130,#55131)) ;
#22801=EDGE_LOOP('',(#55132,#55133,#55134,#55135)) ;
#22802=EDGE_LOOP('',(#55136,#55137,#55138,#55139)) ;
#22803=EDGE_LOOP('',(#55140,#55141,#55142,#55143)) ;
#22804=EDGE_LOOP('',(#55144,#55145,#55146,#55147)) ;
#22805=EDGE_LOOP('',(#55148,#55149,#55150,#55151)) ;
#22806=EDGE_LOOP('',(#55152,#55153,#55154,#55155)) ;
#22807=EDGE_LOOP('',(#55156,#55157,#55158,#55159)) ;
#22808=EDGE_LOOP('',(#55160,#55161,#55162,#55163)) ;
#22809=EDGE_LOOP('',(#55164,#55165,#55166,#55167)) ;
#22810=EDGE_LOOP('',(#55168,#55169,#55170,#55171)) ;
#22811=EDGE_LOOP('',(#55172,#55173,#55174,#55175)) ;
#22812=EDGE_LOOP('',(#55176,#55177,#55178,#55179)) ;
#22813=EDGE_LOOP('',(#55180,#55181,#55182,#55183)) ;
#22814=EDGE_LOOP('',(#55184,#55185,#55186,#55187)) ;
#22815=EDGE_LOOP('',(#55188,#55189,#55190,#55191)) ;
#22816=EDGE_LOOP('',(#55192,#55193,#55194,#55195)) ;
#22817=EDGE_LOOP('',(#55196,#55197,#55198,#55199)) ;
#22818=EDGE_LOOP('',(#55200,#55201,#55202,#55203)) ;
#22819=EDGE_LOOP('',(#55204,#55205,#55206,#55207)) ;
#22820=EDGE_LOOP('',(#55208,#55209,#55210,#55211)) ;
#22821=EDGE_LOOP('',(#55212,#55213,#55214,#55215,#55216,#55217,#55218,#55219,
#55220,#55221,#55222,#55223,#55224,#55225,#55226,#55227,#55228,#55229)) ;
#22822=EDGE_LOOP('',(#55230)) ;
#22823=EDGE_LOOP('',(#55231,#55232,#55233,#55234)) ;
#22824=EDGE_LOOP('',(#55235,#55236,#55237,#55238)) ;
#22825=EDGE_LOOP('',(#55239,#55240,#55241,#55242)) ;
#22826=EDGE_LOOP('',(#55243,#55244,#55245,#55246)) ;
#22827=EDGE_LOOP('',(#55247,#55248,#55249,#55250)) ;
#22828=EDGE_LOOP('',(#55251,#55252,#55253,#55254)) ;
#22829=EDGE_LOOP('',(#55255,#55256,#55257,#55258)) ;
#22830=EDGE_LOOP('',(#55259,#55260,#55261,#55262)) ;
#22831=EDGE_LOOP('',(#55263,#55264,#55265,#55266)) ;
#22832=EDGE_LOOP('',(#55267,#55268,#55269,#55270)) ;
#22833=EDGE_LOOP('',(#55271,#55272,#55273,#55274)) ;
#22834=EDGE_LOOP('',(#55275,#55276,#55277,#55278)) ;
#22835=EDGE_LOOP('',(#55279,#55280,#55281,#55282)) ;
#22836=EDGE_LOOP('',(#55283,#55284,#55285,#55286)) ;
#22837=EDGE_LOOP('',(#55287,#55288,#55289,#55290)) ;
#22838=EDGE_LOOP('',(#55291,#55292,#55293,#55294)) ;
#22839=EDGE_LOOP('',(#55295,#55296,#55297,#55298)) ;
#22840=EDGE_LOOP('',(#55299,#55300,#55301,#55302)) ;
#22841=EDGE_LOOP('',(#55303,#55304,#55305,#55306)) ;
#22842=EDGE_LOOP('',(#55307,#55308,#55309,#55310)) ;
#22843=EDGE_LOOP('',(#55311,#55312,#55313,#55314)) ;
#22844=EDGE_LOOP('',(#55315,#55316,#55317,#55318)) ;
#22845=EDGE_LOOP('',(#55319,#55320,#55321,#55322)) ;
#22846=EDGE_LOOP('',(#55323,#55324,#55325,#55326)) ;
#22847=EDGE_LOOP('',(#55327,#55328,#55329,#55330)) ;
#22848=EDGE_LOOP('',(#55331,#55332,#55333,#55334)) ;
#22849=EDGE_LOOP('',(#55335,#55336,#55337,#55338)) ;
#22850=EDGE_LOOP('',(#55339,#55340,#55341,#55342,#55343,#55344,#55345,#55346,
#55347,#55348,#55349,#55350,#55351,#55352,#55353,#55354,#55355,#55356)) ;
#22851=EDGE_LOOP('',(#55357)) ;
#22852=EDGE_LOOP('',(#55358,#55359,#55360,#55361)) ;
#22853=EDGE_LOOP('',(#55362,#55363,#55364,#55365)) ;
#22854=EDGE_LOOP('',(#55366,#55367,#55368,#55369)) ;
#22855=EDGE_LOOP('',(#55370,#55371,#55372,#55373)) ;
#22856=EDGE_LOOP('',(#55374,#55375,#55376,#55377)) ;
#22857=EDGE_LOOP('',(#55378,#55379,#55380,#55381)) ;
#22858=EDGE_LOOP('',(#55382,#55383,#55384,#55385)) ;
#22859=EDGE_LOOP('',(#55386,#55387,#55388,#55389)) ;
#22860=EDGE_LOOP('',(#55390,#55391,#55392,#55393)) ;
#22861=EDGE_LOOP('',(#55394,#55395,#55396,#55397)) ;
#22862=EDGE_LOOP('',(#55398,#55399,#55400,#55401)) ;
#22863=EDGE_LOOP('',(#55402,#55403,#55404,#55405)) ;
#22864=EDGE_LOOP('',(#55406,#55407,#55408,#55409)) ;
#22865=EDGE_LOOP('',(#55410,#55411,#55412,#55413)) ;
#22866=EDGE_LOOP('',(#55414,#55415,#55416,#55417)) ;
#22867=EDGE_LOOP('',(#55418,#55419,#55420,#55421)) ;
#22868=EDGE_LOOP('',(#55422,#55423,#55424,#55425)) ;
#22869=EDGE_LOOP('',(#55426,#55427,#55428,#55429)) ;
#22870=EDGE_LOOP('',(#55430,#55431,#55432,#55433)) ;
#22871=EDGE_LOOP('',(#55434,#55435,#55436,#55437)) ;
#22872=EDGE_LOOP('',(#55438,#55439,#55440,#55441)) ;
#22873=EDGE_LOOP('',(#55442,#55443,#55444,#55445)) ;
#22874=EDGE_LOOP('',(#55446,#55447,#55448,#55449)) ;
#22875=EDGE_LOOP('',(#55450,#55451,#55452,#55453)) ;
#22876=EDGE_LOOP('',(#55454,#55455,#55456,#55457)) ;
#22877=EDGE_LOOP('',(#55458,#55459,#55460,#55461)) ;
#22878=EDGE_LOOP('',(#55462,#55463,#55464,#55465)) ;
#22879=EDGE_LOOP('',(#55466,#55467,#55468,#55469,#55470,#55471,#55472,#55473,
#55474,#55475,#55476,#55477,#55478,#55479,#55480,#55481,#55482,#55483)) ;
#22880=EDGE_LOOP('',(#55484)) ;
#22881=EDGE_LOOP('',(#55485,#55486,#55487,#55488)) ;
#22882=EDGE_LOOP('',(#55489,#55490,#55491,#55492)) ;
#22883=EDGE_LOOP('',(#55493,#55494,#55495,#55496)) ;
#22884=EDGE_LOOP('',(#55497,#55498,#55499,#55500)) ;
#22885=EDGE_LOOP('',(#55501,#55502,#55503,#55504)) ;
#22886=EDGE_LOOP('',(#55505,#55506,#55507,#55508)) ;
#22887=EDGE_LOOP('',(#55509,#55510,#55511,#55512)) ;
#22888=EDGE_LOOP('',(#55513,#55514,#55515,#55516)) ;
#22889=EDGE_LOOP('',(#55517,#55518,#55519,#55520)) ;
#22890=EDGE_LOOP('',(#55521,#55522,#55523,#55524)) ;
#22891=EDGE_LOOP('',(#55525,#55526,#55527,#55528)) ;
#22892=EDGE_LOOP('',(#55529,#55530,#55531,#55532)) ;
#22893=EDGE_LOOP('',(#55533,#55534,#55535,#55536)) ;
#22894=EDGE_LOOP('',(#55537,#55538,#55539,#55540)) ;
#22895=EDGE_LOOP('',(#55541,#55542,#55543,#55544)) ;
#22896=EDGE_LOOP('',(#55545,#55546,#55547,#55548)) ;
#22897=EDGE_LOOP('',(#55549,#55550,#55551,#55552)) ;
#22898=EDGE_LOOP('',(#55553,#55554,#55555,#55556)) ;
#22899=EDGE_LOOP('',(#55557,#55558,#55559,#55560)) ;
#22900=EDGE_LOOP('',(#55561,#55562,#55563,#55564)) ;
#22901=EDGE_LOOP('',(#55565,#55566,#55567,#55568)) ;
#22902=EDGE_LOOP('',(#55569,#55570,#55571,#55572)) ;
#22903=EDGE_LOOP('',(#55573,#55574,#55575,#55576)) ;
#22904=EDGE_LOOP('',(#55577,#55578,#55579,#55580)) ;
#22905=EDGE_LOOP('',(#55581,#55582,#55583,#55584)) ;
#22906=EDGE_LOOP('',(#55585,#55586,#55587,#55588)) ;
#22907=EDGE_LOOP('',(#55589,#55590,#55591,#55592)) ;
#22908=EDGE_LOOP('',(#55593,#55594,#55595,#55596,#55597,#55598,#55599,#55600,
#55601,#55602,#55603,#55604,#55605,#55606,#55607,#55608,#55609,#55610)) ;
#22909=EDGE_LOOP('',(#55611)) ;
#22910=EDGE_LOOP('',(#55612,#55613,#55614,#55615)) ;
#22911=EDGE_LOOP('',(#55616,#55617,#55618,#55619)) ;
#22912=EDGE_LOOP('',(#55620,#55621,#55622,#55623)) ;
#22913=EDGE_LOOP('',(#55624,#55625,#55626,#55627)) ;
#22914=EDGE_LOOP('',(#55628,#55629,#55630,#55631)) ;
#22915=EDGE_LOOP('',(#55632,#55633,#55634,#55635)) ;
#22916=EDGE_LOOP('',(#55636,#55637,#55638,#55639)) ;
#22917=EDGE_LOOP('',(#55640,#55641,#55642,#55643)) ;
#22918=EDGE_LOOP('',(#55644,#55645,#55646,#55647)) ;
#22919=EDGE_LOOP('',(#55648,#55649,#55650,#55651)) ;
#22920=EDGE_LOOP('',(#55652,#55653,#55654,#55655)) ;
#22921=EDGE_LOOP('',(#55656,#55657,#55658,#55659)) ;
#22922=EDGE_LOOP('',(#55660,#55661,#55662,#55663)) ;
#22923=EDGE_LOOP('',(#55664,#55665,#55666,#55667)) ;
#22924=EDGE_LOOP('',(#55668,#55669,#55670,#55671)) ;
#22925=EDGE_LOOP('',(#55672,#55673,#55674,#55675)) ;
#22926=EDGE_LOOP('',(#55676,#55677,#55678,#55679)) ;
#22927=EDGE_LOOP('',(#55680,#55681,#55682,#55683)) ;
#22928=EDGE_LOOP('',(#55684,#55685,#55686,#55687)) ;
#22929=EDGE_LOOP('',(#55688,#55689,#55690,#55691)) ;
#22930=EDGE_LOOP('',(#55692,#55693,#55694,#55695)) ;
#22931=EDGE_LOOP('',(#55696,#55697,#55698,#55699)) ;
#22932=EDGE_LOOP('',(#55700,#55701,#55702,#55703)) ;
#22933=EDGE_LOOP('',(#55704,#55705,#55706,#55707)) ;
#22934=EDGE_LOOP('',(#55708,#55709,#55710,#55711)) ;
#22935=EDGE_LOOP('',(#55712,#55713,#55714,#55715)) ;
#22936=EDGE_LOOP('',(#55716,#55717,#55718,#55719)) ;
#22937=EDGE_LOOP('',(#55720,#55721,#55722,#55723,#55724,#55725,#55726,#55727,
#55728,#55729,#55730,#55731,#55732,#55733,#55734,#55735,#55736,#55737)) ;
#22938=EDGE_LOOP('',(#55738)) ;
#22939=EDGE_LOOP('',(#55739,#55740,#55741,#55742)) ;
#22940=EDGE_LOOP('',(#55743,#55744,#55745,#55746)) ;
#22941=EDGE_LOOP('',(#55747,#55748,#55749,#55750)) ;
#22942=EDGE_LOOP('',(#55751,#55752,#55753,#55754)) ;
#22943=EDGE_LOOP('',(#55755,#55756,#55757,#55758)) ;
#22944=EDGE_LOOP('',(#55759,#55760,#55761,#55762)) ;
#22945=EDGE_LOOP('',(#55763,#55764,#55765,#55766)) ;
#22946=EDGE_LOOP('',(#55767,#55768,#55769,#55770)) ;
#22947=EDGE_LOOP('',(#55771,#55772,#55773,#55774)) ;
#22948=EDGE_LOOP('',(#55775,#55776,#55777,#55778)) ;
#22949=EDGE_LOOP('',(#55779,#55780,#55781,#55782)) ;
#22950=EDGE_LOOP('',(#55783,#55784,#55785,#55786)) ;
#22951=EDGE_LOOP('',(#55787,#55788,#55789,#55790)) ;
#22952=EDGE_LOOP('',(#55791,#55792,#55793,#55794)) ;
#22953=EDGE_LOOP('',(#55795,#55796,#55797,#55798)) ;
#22954=EDGE_LOOP('',(#55799,#55800,#55801,#55802)) ;
#22955=EDGE_LOOP('',(#55803,#55804,#55805,#55806)) ;
#22956=EDGE_LOOP('',(#55807,#55808,#55809,#55810)) ;
#22957=EDGE_LOOP('',(#55811,#55812,#55813,#55814)) ;
#22958=EDGE_LOOP('',(#55815,#55816,#55817,#55818)) ;
#22959=EDGE_LOOP('',(#55819,#55820,#55821,#55822)) ;
#22960=EDGE_LOOP('',(#55823,#55824,#55825,#55826)) ;
#22961=EDGE_LOOP('',(#55827,#55828,#55829,#55830)) ;
#22962=EDGE_LOOP('',(#55831,#55832,#55833,#55834)) ;
#22963=EDGE_LOOP('',(#55835,#55836,#55837,#55838)) ;
#22964=EDGE_LOOP('',(#55839,#55840,#55841,#55842)) ;
#22965=EDGE_LOOP('',(#55843,#55844,#55845,#55846)) ;
#22966=EDGE_LOOP('',(#55847,#55848,#55849,#55850,#55851,#55852,#55853,#55854,
#55855,#55856,#55857,#55858,#55859,#55860,#55861,#55862,#55863,#55864)) ;
#22967=EDGE_LOOP('',(#55865)) ;
#22968=EDGE_LOOP('',(#55866,#55867,#55868,#55869)) ;
#22969=EDGE_LOOP('',(#55870,#55871,#55872,#55873)) ;
#22970=EDGE_LOOP('',(#55874,#55875,#55876,#55877)) ;
#22971=EDGE_LOOP('',(#55878,#55879,#55880,#55881)) ;
#22972=EDGE_LOOP('',(#55882,#55883,#55884,#55885)) ;
#22973=EDGE_LOOP('',(#55886,#55887,#55888,#55889)) ;
#22974=EDGE_LOOP('',(#55890,#55891,#55892,#55893)) ;
#22975=EDGE_LOOP('',(#55894,#55895,#55896,#55897)) ;
#22976=EDGE_LOOP('',(#55898,#55899,#55900,#55901)) ;
#22977=EDGE_LOOP('',(#55902,#55903,#55904,#55905)) ;
#22978=EDGE_LOOP('',(#55906,#55907,#55908,#55909)) ;
#22979=EDGE_LOOP('',(#55910,#55911,#55912,#55913)) ;
#22980=EDGE_LOOP('',(#55914,#55915,#55916,#55917)) ;
#22981=EDGE_LOOP('',(#55918,#55919,#55920,#55921)) ;
#22982=EDGE_LOOP('',(#55922,#55923,#55924,#55925)) ;
#22983=EDGE_LOOP('',(#55926,#55927,#55928,#55929)) ;
#22984=EDGE_LOOP('',(#55930,#55931,#55932,#55933)) ;
#22985=EDGE_LOOP('',(#55934,#55935,#55936,#55937)) ;
#22986=EDGE_LOOP('',(#55938,#55939,#55940,#55941)) ;
#22987=EDGE_LOOP('',(#55942,#55943,#55944,#55945)) ;
#22988=EDGE_LOOP('',(#55946,#55947,#55948,#55949)) ;
#22989=EDGE_LOOP('',(#55950,#55951,#55952,#55953)) ;
#22990=EDGE_LOOP('',(#55954,#55955,#55956,#55957)) ;
#22991=EDGE_LOOP('',(#55958,#55959,#55960,#55961)) ;
#22992=EDGE_LOOP('',(#55962,#55963,#55964,#55965)) ;
#22993=EDGE_LOOP('',(#55966,#55967,#55968,#55969)) ;
#22994=EDGE_LOOP('',(#55970,#55971,#55972,#55973)) ;
#22995=EDGE_LOOP('',(#55974,#55975,#55976,#55977,#55978,#55979,#55980,#55981,
#55982,#55983,#55984,#55985,#55986,#55987,#55988,#55989,#55990,#55991)) ;
#22996=EDGE_LOOP('',(#55992)) ;
#22997=EDGE_LOOP('',(#55993,#55994,#55995,#55996)) ;
#22998=EDGE_LOOP('',(#55997,#55998,#55999,#56000)) ;
#22999=EDGE_LOOP('',(#56001,#56002,#56003,#56004)) ;
#23000=EDGE_LOOP('',(#56005,#56006,#56007,#56008)) ;
#23001=EDGE_LOOP('',(#56009,#56010,#56011,#56012)) ;
#23002=EDGE_LOOP('',(#56013,#56014,#56015,#56016)) ;
#23003=EDGE_LOOP('',(#56017,#56018,#56019,#56020)) ;
#23004=EDGE_LOOP('',(#56021,#56022,#56023,#56024)) ;
#23005=EDGE_LOOP('',(#56025,#56026,#56027,#56028)) ;
#23006=EDGE_LOOP('',(#56029,#56030,#56031,#56032)) ;
#23007=EDGE_LOOP('',(#56033,#56034,#56035,#56036)) ;
#23008=EDGE_LOOP('',(#56037,#56038,#56039,#56040)) ;
#23009=EDGE_LOOP('',(#56041,#56042,#56043,#56044)) ;
#23010=EDGE_LOOP('',(#56045,#56046,#56047,#56048)) ;
#23011=EDGE_LOOP('',(#56049,#56050,#56051,#56052)) ;
#23012=EDGE_LOOP('',(#56053,#56054,#56055,#56056)) ;
#23013=EDGE_LOOP('',(#56057,#56058,#56059,#56060)) ;
#23014=EDGE_LOOP('',(#56061,#56062,#56063,#56064)) ;
#23015=EDGE_LOOP('',(#56065,#56066,#56067,#56068)) ;
#23016=EDGE_LOOP('',(#56069,#56070,#56071,#56072)) ;
#23017=EDGE_LOOP('',(#56073,#56074,#56075,#56076)) ;
#23018=EDGE_LOOP('',(#56077,#56078,#56079,#56080)) ;
#23019=EDGE_LOOP('',(#56081,#56082,#56083,#56084)) ;
#23020=EDGE_LOOP('',(#56085,#56086,#56087,#56088)) ;
#23021=EDGE_LOOP('',(#56089,#56090,#56091,#56092)) ;
#23022=EDGE_LOOP('',(#56093,#56094,#56095,#56096)) ;
#23023=EDGE_LOOP('',(#56097,#56098,#56099,#56100)) ;
#23024=EDGE_LOOP('',(#56101,#56102,#56103,#56104,#56105,#56106,#56107,#56108,
#56109,#56110,#56111,#56112,#56113,#56114,#56115,#56116,#56117,#56118)) ;
#23025=EDGE_LOOP('',(#56119)) ;
#23026=EDGE_LOOP('',(#56120,#56121,#56122,#56123)) ;
#23027=EDGE_LOOP('',(#56124,#56125,#56126,#56127)) ;
#23028=EDGE_LOOP('',(#56128,#56129,#56130,#56131)) ;
#23029=EDGE_LOOP('',(#56132,#56133,#56134,#56135)) ;
#23030=EDGE_LOOP('',(#56136,#56137,#56138,#56139)) ;
#23031=EDGE_LOOP('',(#56140,#56141,#56142,#56143)) ;
#23032=EDGE_LOOP('',(#56144,#56145,#56146,#56147)) ;
#23033=EDGE_LOOP('',(#56148,#56149,#56150,#56151)) ;
#23034=EDGE_LOOP('',(#56152,#56153,#56154,#56155)) ;
#23035=EDGE_LOOP('',(#56156,#56157,#56158,#56159)) ;
#23036=EDGE_LOOP('',(#56160,#56161,#56162,#56163)) ;
#23037=EDGE_LOOP('',(#56164,#56165,#56166,#56167)) ;
#23038=EDGE_LOOP('',(#56168,#56169,#56170,#56171)) ;
#23039=EDGE_LOOP('',(#56172,#56173,#56174,#56175)) ;
#23040=EDGE_LOOP('',(#56176,#56177,#56178,#56179)) ;
#23041=EDGE_LOOP('',(#56180,#56181,#56182,#56183)) ;
#23042=EDGE_LOOP('',(#56184,#56185,#56186,#56187)) ;
#23043=EDGE_LOOP('',(#56188,#56189,#56190,#56191)) ;
#23044=EDGE_LOOP('',(#56192,#56193,#56194,#56195)) ;
#23045=EDGE_LOOP('',(#56196,#56197,#56198,#56199)) ;
#23046=EDGE_LOOP('',(#56200,#56201,#56202,#56203)) ;
#23047=EDGE_LOOP('',(#56204,#56205,#56206,#56207)) ;
#23048=EDGE_LOOP('',(#56208,#56209,#56210,#56211)) ;
#23049=EDGE_LOOP('',(#56212,#56213,#56214,#56215)) ;
#23050=EDGE_LOOP('',(#56216,#56217,#56218,#56219)) ;
#23051=EDGE_LOOP('',(#56220,#56221,#56222,#56223)) ;
#23052=EDGE_LOOP('',(#56224,#56225,#56226,#56227)) ;
#23053=EDGE_LOOP('',(#56228,#56229,#56230,#56231,#56232,#56233,#56234,#56235,
#56236,#56237,#56238,#56239,#56240,#56241,#56242,#56243,#56244,#56245)) ;
#23054=EDGE_LOOP('',(#56246)) ;
#23055=EDGE_LOOP('',(#56247)) ;
#23056=EDGE_LOOP('',(#56248,#56249,#56250,#56251,#56252,#56253,#56254,#56255)) ;
#23057=EDGE_LOOP('',(#56256)) ;
#23058=EDGE_LOOP('',(#56257,#56258,#56259,#56260,#56261,#56262,#56263,#56264)) ;
#23059=EDGE_LOOP('',(#56265)) ;
#23060=EDGE_LOOP('',(#56266,#56267,#56268,#56269,#56270,#56271,#56272,#56273)) ;
#23061=EDGE_LOOP('',(#56274)) ;
#23062=EDGE_LOOP('',(#56275,#56276,#56277,#56278,#56279,#56280,#56281,#56282)) ;
#23063=EDGE_LOOP('',(#56283)) ;
#23064=EDGE_LOOP('',(#56284,#56285,#56286,#56287,#56288,#56289,#56290,#56291)) ;
#23065=EDGE_LOOP('',(#56292)) ;
#23066=EDGE_LOOP('',(#56293,#56294,#56295,#56296,#56297,#56298,#56299,#56300)) ;
#23067=EDGE_LOOP('',(#56301)) ;
#23068=EDGE_LOOP('',(#56302,#56303,#56304,#56305,#56306,#56307,#56308,#56309)) ;
#23069=EDGE_LOOP('',(#56310)) ;
#23070=EDGE_LOOP('',(#56311,#56312,#56313,#56314,#56315,#56316,#56317,#56318)) ;
#23071=EDGE_LOOP('',(#56319)) ;
#23072=EDGE_LOOP('',(#56320,#56321,#56322,#56323,#56324,#56325,#56326,#56327)) ;
#23073=EDGE_LOOP('',(#56328,#56329,#56330,#56331)) ;
#23074=EDGE_LOOP('',(#56332,#56333,#56334,#56335)) ;
#23075=EDGE_LOOP('',(#56336,#56337,#56338)) ;
#23076=EDGE_LOOP('',(#56339,#56340,#56341)) ;
#23077=EDGE_LOOP('',(#56342,#56343,#56344,#56345)) ;
#23078=EDGE_LOOP('',(#56346,#56347,#56348,#56349,#56350,#56351)) ;
#23079=EDGE_LOOP('',(#56352,#56353,#56354,#56355,#56356,#56357,#56358)) ;
#23080=EDGE_LOOP('',(#56359,#56360,#56361,#56362)) ;
#23081=EDGE_LOOP('',(#56363,#56364,#56365,#56366)) ;
#23082=EDGE_LOOP('',(#56367,#56368,#56369,#56370)) ;
#23083=EDGE_LOOP('',(#56371,#56372,#56373,#56374)) ;
#23084=EDGE_LOOP('',(#56375,#56376,#56377)) ;
#23085=EDGE_LOOP('',(#56378,#56379,#56380,#56381)) ;
#23086=EDGE_LOOP('',(#56382,#56383,#56384,#56385)) ;
#23087=EDGE_LOOP('',(#56386,#56387,#56388,#56389)) ;
#23088=EDGE_LOOP('',(#56390,#56391,#56392,#56393)) ;
#23089=EDGE_LOOP('',(#56394,#56395,#56396,#56397)) ;
#23090=EDGE_LOOP('',(#56398,#56399,#56400,#56401)) ;
#23091=EDGE_LOOP('',(#56402,#56403,#56404,#56405)) ;
#23092=EDGE_LOOP('',(#56406,#56407,#56408,#56409)) ;
#23093=EDGE_LOOP('',(#56410,#56411,#56412,#56413)) ;
#23094=EDGE_LOOP('',(#56414,#56415,#56416)) ;
#23095=EDGE_LOOP('',(#56417,#56418,#56419)) ;
#23096=EDGE_LOOP('',(#56420,#56421,#56422,#56423,#56424)) ;
#23097=EDGE_LOOP('',(#56425,#56426,#56427)) ;
#23098=EDGE_LOOP('',(#56428,#56429,#56430)) ;
#23099=EDGE_LOOP('',(#56431,#56432,#56433,#56434)) ;
#23100=EDGE_LOOP('',(#56435,#56436,#56437,#56438)) ;
#23101=EDGE_LOOP('',(#56439,#56440,#56441,#56442)) ;
#23102=EDGE_LOOP('',(#56443,#56444,#56445,#56446)) ;
#23103=EDGE_LOOP('',(#56447,#56448,#56449,#56450)) ;
#23104=EDGE_LOOP('',(#56451,#56452,#56453,#56454)) ;
#23105=EDGE_LOOP('',(#56455,#56456,#56457,#56458)) ;
#23106=EDGE_LOOP('',(#56459,#56460,#56461)) ;
#23107=EDGE_LOOP('',(#56462,#56463,#56464,#56465)) ;
#23108=EDGE_LOOP('',(#56466,#56467,#56468,#56469)) ;
#23109=EDGE_LOOP('',(#56470,#56471,#56472)) ;
#23110=EDGE_LOOP('',(#56473,#56474,#56475,#56476)) ;
#23111=EDGE_LOOP('',(#56477,#56478,#56479,#56480)) ;
#23112=EDGE_LOOP('',(#56481,#56482,#56483,#56484)) ;
#23113=EDGE_LOOP('',(#56485,#56486,#56487,#56488)) ;
#23114=EDGE_LOOP('',(#56489,#56490,#56491,#56492)) ;
#23115=EDGE_LOOP('',(#56493,#56494,#56495,#56496)) ;
#23116=EDGE_LOOP('',(#56497,#56498,#56499,#56500,#56501)) ;
#23117=EDGE_LOOP('',(#56502,#56503,#56504,#56505)) ;
#23118=EDGE_LOOP('',(#56506,#56507,#56508)) ;
#23119=EDGE_LOOP('',(#56509,#56510,#56511,#56512)) ;
#23120=EDGE_LOOP('',(#56513,#56514,#56515,#56516)) ;
#23121=EDGE_LOOP('',(#56517,#56518,#56519)) ;
#23122=EDGE_LOOP('',(#56520,#56521,#56522,#56523)) ;
#23123=EDGE_LOOP('',(#56524,#56525,#56526,#56527)) ;
#23124=EDGE_LOOP('',(#56528,#56529,#56530,#56531)) ;
#23125=EDGE_LOOP('',(#56532,#56533,#56534)) ;
#23126=EDGE_LOOP('',(#56535,#56536,#56537,#56538)) ;
#23127=EDGE_LOOP('',(#56539,#56540,#56541,#56542)) ;
#23128=EDGE_LOOP('',(#56543,#56544,#56545)) ;
#23129=EDGE_LOOP('',(#56546,#56547,#56548)) ;
#23130=EDGE_LOOP('',(#56549,#56550,#56551,#56552)) ;
#23131=EDGE_LOOP('',(#56553,#56554,#56555,#56556)) ;
#23132=EDGE_LOOP('',(#56557,#56558,#56559)) ;
#23133=EDGE_LOOP('',(#56560,#56561,#56562)) ;
#23134=EDGE_LOOP('',(#56563,#56564,#56565,#56566)) ;
#23135=EDGE_LOOP('',(#56567,#56568,#56569,#56570)) ;
#23136=EDGE_LOOP('',(#56571,#56572,#56573)) ;
#23137=EDGE_LOOP('',(#56574,#56575,#56576,#56577)) ;
#23138=EDGE_LOOP('',(#56578,#56579,#56580,#56581)) ;
#23139=EDGE_LOOP('',(#56582,#56583,#56584)) ;
#23140=EDGE_LOOP('',(#56585,#56586,#56587)) ;
#23141=EDGE_LOOP('',(#56588,#56589,#56590,#56591)) ;
#23142=EDGE_LOOP('',(#56592,#56593,#56594,#56595)) ;
#23143=EDGE_LOOP('',(#56596,#56597,#56598,#56599)) ;
#23144=EDGE_LOOP('',(#56600,#56601,#56602,#56603)) ;
#23145=EDGE_LOOP('',(#56604,#56605,#56606,#56607)) ;
#23146=EDGE_LOOP('',(#56608,#56609,#56610,#56611)) ;
#23147=EDGE_LOOP('',(#56612,#56613,#56614)) ;
#23148=EDGE_LOOP('',(#56615,#56616,#56617)) ;
#23149=EDGE_LOOP('',(#56618,#56619,#56620,#56621)) ;
#23150=EDGE_LOOP('',(#56622,#56623,#56624,#56625)) ;
#23151=EDGE_LOOP('',(#56626,#56627,#56628,#56629)) ;
#23152=EDGE_LOOP('',(#56630,#56631,#56632,#56633)) ;
#23153=EDGE_LOOP('',(#56634,#56635,#56636,#56637)) ;
#23154=EDGE_LOOP('',(#56638,#56639,#56640,#56641)) ;
#23155=EDGE_LOOP('',(#56642,#56643,#56644,#56645)) ;
#23156=EDGE_LOOP('',(#56646,#56647,#56648,#56649)) ;
#23157=EDGE_LOOP('',(#56650,#56651,#56652,#56653)) ;
#23158=EDGE_LOOP('',(#56654,#56655,#56656,#56657)) ;
#23159=EDGE_LOOP('',(#56658,#56659,#56660,#56661)) ;
#23160=EDGE_LOOP('',(#56662,#56663,#56664,#56665)) ;
#23161=EDGE_LOOP('',(#56666,#56667,#56668,#56669)) ;
#23162=EDGE_LOOP('',(#56670,#56671,#56672,#56673)) ;
#23163=EDGE_LOOP('',(#56674,#56675,#56676,#56677)) ;
#23164=EDGE_LOOP('',(#56678,#56679,#56680,#56681)) ;
#23165=EDGE_LOOP('',(#56682,#56683,#56684,#56685)) ;
#23166=EDGE_LOOP('',(#56686,#56687,#56688)) ;
#23167=EDGE_LOOP('',(#56689,#56690,#56691,#56692)) ;
#23168=EDGE_LOOP('',(#56693,#56694,#56695,#56696)) ;
#23169=EDGE_LOOP('',(#56697,#56698,#56699,#56700)) ;
#23170=EDGE_LOOP('',(#56701,#56702,#56703)) ;
#23171=EDGE_LOOP('',(#56704,#56705,#56706,#56707)) ;
#23172=EDGE_LOOP('',(#56708,#56709,#56710,#56711)) ;
#23173=EDGE_LOOP('',(#56712,#56713,#56714,#56715)) ;
#23174=EDGE_LOOP('',(#56716,#56717,#56718)) ;
#23175=EDGE_LOOP('',(#56719,#56720,#56721)) ;
#23176=EDGE_LOOP('',(#56722,#56723,#56724,#56725)) ;
#23177=EDGE_LOOP('',(#56726,#56727,#56728,#56729)) ;
#23178=EDGE_LOOP('',(#56730,#56731,#56732,#56733)) ;
#23179=EDGE_LOOP('',(#56734,#56735,#56736,#56737)) ;
#23180=EDGE_LOOP('',(#56738,#56739,#56740,#56741)) ;
#23181=EDGE_LOOP('',(#56742,#56743,#56744,#56745)) ;
#23182=EDGE_LOOP('',(#56746,#56747,#56748,#56749)) ;
#23183=EDGE_LOOP('',(#56750,#56751,#56752,#56753)) ;
#23184=EDGE_LOOP('',(#56754,#56755,#56756,#56757)) ;
#23185=EDGE_LOOP('',(#56758,#56759,#56760,#56761)) ;
#23186=EDGE_LOOP('',(#56762,#56763,#56764,#56765)) ;
#23187=EDGE_LOOP('',(#56766,#56767,#56768,#56769)) ;
#23188=EDGE_LOOP('',(#56770,#56771,#56772,#56773)) ;
#23189=EDGE_LOOP('',(#56774,#56775,#56776,#56777)) ;
#23190=EDGE_LOOP('',(#56778,#56779,#56780,#56781)) ;
#23191=EDGE_LOOP('',(#56782,#56783,#56784,#56785)) ;
#23192=EDGE_LOOP('',(#56786,#56787,#56788,#56789)) ;
#23193=EDGE_LOOP('',(#56790,#56791,#56792)) ;
#23194=EDGE_LOOP('',(#56793,#56794,#56795,#56796)) ;
#23195=EDGE_LOOP('',(#56797,#56798,#56799,#56800)) ;
#23196=EDGE_LOOP('',(#56801,#56802,#56803,#56804)) ;
#23197=EDGE_LOOP('',(#56805,#56806,#56807)) ;
#23198=EDGE_LOOP('',(#56808,#56809,#56810,#56811)) ;
#23199=EDGE_LOOP('',(#56812,#56813,#56814,#56815)) ;
#23200=EDGE_LOOP('',(#56816,#56817,#56818,#56819)) ;
#23201=EDGE_LOOP('',(#56820,#56821,#56822)) ;
#23202=EDGE_LOOP('',(#56823,#56824,#56825)) ;
#23203=EDGE_LOOP('',(#56826,#56827,#56828,#56829)) ;
#23204=EDGE_LOOP('',(#56830,#56831,#56832,#56833)) ;
#23205=EDGE_LOOP('',(#56834,#56835,#56836,#56837)) ;
#23206=EDGE_LOOP('',(#56838,#56839,#56840,#56841)) ;
#23207=EDGE_LOOP('',(#56842,#56843,#56844,#56845)) ;
#23208=EDGE_LOOP('',(#56846,#56847,#56848,#56849)) ;
#23209=EDGE_LOOP('',(#56850,#56851,#56852,#56853)) ;
#23210=EDGE_LOOP('',(#56854,#56855,#56856,#56857)) ;
#23211=EDGE_LOOP('',(#56858,#56859,#56860,#56861)) ;
#23212=EDGE_LOOP('',(#56862,#56863,#56864,#56865)) ;
#23213=EDGE_LOOP('',(#56866,#56867,#56868,#56869)) ;
#23214=EDGE_LOOP('',(#56870,#56871,#56872,#56873)) ;
#23215=EDGE_LOOP('',(#56874,#56875,#56876,#56877)) ;
#23216=EDGE_LOOP('',(#56878,#56879,#56880,#56881)) ;
#23217=EDGE_LOOP('',(#56882,#56883,#56884,#56885)) ;
#23218=EDGE_LOOP('',(#56886,#56887,#56888,#56889)) ;
#23219=EDGE_LOOP('',(#56890,#56891,#56892,#56893)) ;
#23220=EDGE_LOOP('',(#56894,#56895,#56896)) ;
#23221=EDGE_LOOP('',(#56897,#56898,#56899,#56900)) ;
#23222=EDGE_LOOP('',(#56901,#56902,#56903,#56904)) ;
#23223=EDGE_LOOP('',(#56905,#56906,#56907,#56908)) ;
#23224=EDGE_LOOP('',(#56909,#56910,#56911)) ;
#23225=EDGE_LOOP('',(#56912,#56913,#56914,#56915)) ;
#23226=EDGE_LOOP('',(#56916,#56917,#56918,#56919)) ;
#23227=EDGE_LOOP('',(#56920,#56921,#56922,#56923)) ;
#23228=EDGE_LOOP('',(#56924,#56925,#56926)) ;
#23229=EDGE_LOOP('',(#56927,#56928,#56929)) ;
#23230=EDGE_LOOP('',(#56930,#56931,#56932,#56933)) ;
#23231=EDGE_LOOP('',(#56934,#56935,#56936,#56937)) ;
#23232=EDGE_LOOP('',(#56938,#56939,#56940,#56941)) ;
#23233=EDGE_LOOP('',(#56942,#56943,#56944,#56945)) ;
#23234=EDGE_LOOP('',(#56946,#56947,#56948,#56949)) ;
#23235=EDGE_LOOP('',(#56950,#56951,#56952,#56953)) ;
#23236=EDGE_LOOP('',(#56954,#56955,#56956,#56957)) ;
#23237=EDGE_LOOP('',(#56958,#56959,#56960,#56961)) ;
#23238=EDGE_LOOP('',(#56962,#56963,#56964,#56965)) ;
#23239=EDGE_LOOP('',(#56966,#56967,#56968,#56969)) ;
#23240=EDGE_LOOP('',(#56970,#56971,#56972,#56973)) ;
#23241=EDGE_LOOP('',(#56974,#56975,#56976,#56977)) ;
#23242=EDGE_LOOP('',(#56978,#56979,#56980,#56981)) ;
#23243=EDGE_LOOP('',(#56982,#56983,#56984,#56985)) ;
#23244=EDGE_LOOP('',(#56986,#56987,#56988,#56989)) ;
#23245=EDGE_LOOP('',(#56990,#56991,#56992,#56993)) ;
#23246=EDGE_LOOP('',(#56994,#56995,#56996,#56997)) ;
#23247=EDGE_LOOP('',(#56998,#56999,#57000)) ;
#23248=EDGE_LOOP('',(#57001,#57002,#57003,#57004)) ;
#23249=EDGE_LOOP('',(#57005,#57006,#57007,#57008)) ;
#23250=EDGE_LOOP('',(#57009,#57010,#57011,#57012)) ;
#23251=EDGE_LOOP('',(#57013,#57014,#57015)) ;
#23252=EDGE_LOOP('',(#57016,#57017,#57018,#57019)) ;
#23253=EDGE_LOOP('',(#57020,#57021,#57022,#57023)) ;
#23254=EDGE_LOOP('',(#57024,#57025,#57026,#57027)) ;
#23255=EDGE_LOOP('',(#57028,#57029,#57030)) ;
#23256=EDGE_LOOP('',(#57031,#57032,#57033)) ;
#23257=EDGE_LOOP('',(#57034,#57035,#57036,#57037)) ;
#23258=EDGE_LOOP('',(#57038,#57039,#57040,#57041)) ;
#23259=EDGE_LOOP('',(#57042,#57043,#57044,#57045)) ;
#23260=EDGE_LOOP('',(#57046,#57047,#57048,#57049)) ;
#23261=EDGE_LOOP('',(#57050,#57051,#57052,#57053)) ;
#23262=EDGE_LOOP('',(#57054,#57055,#57056,#57057)) ;
#23263=EDGE_LOOP('',(#57058,#57059,#57060,#57061)) ;
#23264=EDGE_LOOP('',(#57062,#57063,#57064,#57065)) ;
#23265=EDGE_LOOP('',(#57066,#57067,#57068,#57069)) ;
#23266=EDGE_LOOP('',(#57070,#57071,#57072,#57073)) ;
#23267=EDGE_LOOP('',(#57074,#57075,#57076,#57077)) ;
#23268=EDGE_LOOP('',(#57078,#57079,#57080,#57081)) ;
#23269=EDGE_LOOP('',(#57082,#57083,#57084,#57085)) ;
#23270=EDGE_LOOP('',(#57086,#57087,#57088,#57089)) ;
#23271=EDGE_LOOP('',(#57090,#57091,#57092,#57093)) ;
#23272=EDGE_LOOP('',(#57094,#57095,#57096,#57097)) ;
#23273=EDGE_LOOP('',(#57098,#57099,#57100,#57101)) ;
#23274=EDGE_LOOP('',(#57102,#57103,#57104)) ;
#23275=EDGE_LOOP('',(#57105,#57106,#57107,#57108)) ;
#23276=EDGE_LOOP('',(#57109,#57110,#57111,#57112)) ;
#23277=EDGE_LOOP('',(#57113,#57114,#57115,#57116)) ;
#23278=EDGE_LOOP('',(#57117,#57118,#57119)) ;
#23279=EDGE_LOOP('',(#57120,#57121,#57122,#57123)) ;
#23280=EDGE_LOOP('',(#57124,#57125,#57126,#57127)) ;
#23281=EDGE_LOOP('',(#57128,#57129,#57130,#57131)) ;
#23282=EDGE_LOOP('',(#57132,#57133,#57134)) ;
#23283=EDGE_LOOP('',(#57135,#57136,#57137)) ;
#23284=EDGE_LOOP('',(#57138,#57139,#57140,#57141)) ;
#23285=EDGE_LOOP('',(#57142,#57143,#57144,#57145)) ;
#23286=EDGE_LOOP('',(#57146,#57147,#57148,#57149)) ;
#23287=EDGE_LOOP('',(#57150,#57151,#57152,#57153)) ;
#23288=EDGE_LOOP('',(#57154,#57155,#57156,#57157)) ;
#23289=EDGE_LOOP('',(#57158,#57159,#57160,#57161)) ;
#23290=EDGE_LOOP('',(#57162,#57163,#57164,#57165)) ;
#23291=EDGE_LOOP('',(#57166,#57167,#57168,#57169)) ;
#23292=EDGE_LOOP('',(#57170,#57171,#57172,#57173)) ;
#23293=EDGE_LOOP('',(#57174,#57175,#57176,#57177)) ;
#23294=EDGE_LOOP('',(#57178,#57179,#57180,#57181)) ;
#23295=EDGE_LOOP('',(#57182,#57183,#57184,#57185)) ;
#23296=EDGE_LOOP('',(#57186,#57187,#57188,#57189)) ;
#23297=EDGE_LOOP('',(#57190,#57191,#57192,#57193)) ;
#23298=EDGE_LOOP('',(#57194,#57195,#57196,#57197)) ;
#23299=EDGE_LOOP('',(#57198,#57199,#57200,#57201)) ;
#23300=EDGE_LOOP('',(#57202,#57203,#57204,#57205)) ;
#23301=EDGE_LOOP('',(#57206,#57207,#57208)) ;
#23302=EDGE_LOOP('',(#57209,#57210,#57211,#57212)) ;
#23303=EDGE_LOOP('',(#57213,#57214,#57215,#57216)) ;
#23304=EDGE_LOOP('',(#57217,#57218,#57219,#57220)) ;
#23305=EDGE_LOOP('',(#57221,#57222,#57223)) ;
#23306=EDGE_LOOP('',(#57224,#57225,#57226,#57227)) ;
#23307=EDGE_LOOP('',(#57228,#57229,#57230,#57231)) ;
#23308=EDGE_LOOP('',(#57232,#57233,#57234,#57235)) ;
#23309=EDGE_LOOP('',(#57236,#57237,#57238)) ;
#23310=EDGE_LOOP('',(#57239,#57240,#57241)) ;
#23311=EDGE_LOOP('',(#57242,#57243,#57244,#57245)) ;
#23312=EDGE_LOOP('',(#57246,#57247,#57248,#57249)) ;
#23313=EDGE_LOOP('',(#57250,#57251,#57252,#57253)) ;
#23314=EDGE_LOOP('',(#57254,#57255,#57256,#57257)) ;
#23315=EDGE_LOOP('',(#57258,#57259,#57260,#57261)) ;
#23316=EDGE_LOOP('',(#57262,#57263,#57264,#57265)) ;
#23317=EDGE_LOOP('',(#57266,#57267,#57268,#57269)) ;
#23318=EDGE_LOOP('',(#57270,#57271,#57272,#57273)) ;
#23319=EDGE_LOOP('',(#57274,#57275,#57276,#57277)) ;
#23320=EDGE_LOOP('',(#57278,#57279,#57280,#57281)) ;
#23321=EDGE_LOOP('',(#57282,#57283,#57284,#57285)) ;
#23322=EDGE_LOOP('',(#57286,#57287,#57288,#57289)) ;
#23323=EDGE_LOOP('',(#57290,#57291,#57292,#57293)) ;
#23324=EDGE_LOOP('',(#57294,#57295,#57296,#57297)) ;
#23325=EDGE_LOOP('',(#57298,#57299,#57300,#57301)) ;
#23326=EDGE_LOOP('',(#57302,#57303,#57304,#57305)) ;
#23327=EDGE_LOOP('',(#57306,#57307,#57308,#57309)) ;
#23328=EDGE_LOOP('',(#57310,#57311,#57312)) ;
#23329=EDGE_LOOP('',(#57313,#57314,#57315,#57316)) ;
#23330=EDGE_LOOP('',(#57317,#57318,#57319,#57320)) ;
#23331=EDGE_LOOP('',(#57321,#57322,#57323,#57324)) ;
#23332=EDGE_LOOP('',(#57325,#57326,#57327)) ;
#23333=EDGE_LOOP('',(#57328,#57329,#57330,#57331)) ;
#23334=EDGE_LOOP('',(#57332,#57333,#57334,#57335)) ;
#23335=EDGE_LOOP('',(#57336,#57337,#57338,#57339)) ;
#23336=EDGE_LOOP('',(#57340,#57341,#57342)) ;
#23337=EDGE_LOOP('',(#57343,#57344,#57345)) ;
#23338=EDGE_LOOP('',(#57346,#57347,#57348,#57349)) ;
#23339=EDGE_LOOP('',(#57350,#57351,#57352,#57353)) ;
#23340=EDGE_LOOP('',(#57354,#57355,#57356,#57357)) ;
#23341=EDGE_LOOP('',(#57358,#57359,#57360,#57361)) ;
#23342=EDGE_LOOP('',(#57362,#57363,#57364,#57365)) ;
#23343=EDGE_LOOP('',(#57366,#57367,#57368,#57369)) ;
#23344=EDGE_LOOP('',(#57370,#57371,#57372,#57373)) ;
#23345=EDGE_LOOP('',(#57374,#57375,#57376,#57377)) ;
#23346=EDGE_LOOP('',(#57378,#57379,#57380,#57381)) ;
#23347=EDGE_LOOP('',(#57382,#57383,#57384,#57385)) ;
#23348=EDGE_LOOP('',(#57386,#57387,#57388,#57389)) ;
#23349=EDGE_LOOP('',(#57390,#57391,#57392,#57393)) ;
#23350=EDGE_LOOP('',(#57394,#57395,#57396,#57397)) ;
#23351=EDGE_LOOP('',(#57398,#57399,#57400,#57401)) ;
#23352=EDGE_LOOP('',(#57402,#57403,#57404,#57405)) ;
#23353=EDGE_LOOP('',(#57406,#57407,#57408,#57409)) ;
#23354=EDGE_LOOP('',(#57410,#57411,#57412,#57413)) ;
#23355=EDGE_LOOP('',(#57414,#57415,#57416)) ;
#23356=EDGE_LOOP('',(#57417,#57418,#57419,#57420)) ;
#23357=EDGE_LOOP('',(#57421,#57422,#57423,#57424)) ;
#23358=EDGE_LOOP('',(#57425,#57426,#57427,#57428)) ;
#23359=EDGE_LOOP('',(#57429,#57430,#57431)) ;
#23360=EDGE_LOOP('',(#57432,#57433,#57434,#57435)) ;
#23361=EDGE_LOOP('',(#57436,#57437,#57438,#57439)) ;
#23362=EDGE_LOOP('',(#57440,#57441,#57442,#57443)) ;
#23363=EDGE_LOOP('',(#57444,#57445,#57446)) ;
#23364=EDGE_LOOP('',(#57447,#57448,#57449)) ;
#23365=EDGE_LOOP('',(#57450,#57451,#57452,#57453)) ;
#23366=EDGE_LOOP('',(#57454,#57455,#57456,#57457)) ;
#23367=EDGE_LOOP('',(#57458,#57459,#57460,#57461)) ;
#23368=EDGE_LOOP('',(#57462,#57463,#57464,#57465)) ;
#23369=EDGE_LOOP('',(#57466,#57467,#57468,#57469)) ;
#23370=EDGE_LOOP('',(#57470,#57471,#57472,#57473)) ;
#23371=EDGE_LOOP('',(#57474,#57475,#57476,#57477)) ;
#23372=EDGE_LOOP('',(#57478,#57479,#57480,#57481)) ;
#23373=EDGE_LOOP('',(#57482,#57483,#57484,#57485)) ;
#23374=EDGE_LOOP('',(#57486,#57487,#57488,#57489)) ;
#23375=EDGE_LOOP('',(#57490,#57491,#57492,#57493)) ;
#23376=EDGE_LOOP('',(#57494,#57495,#57496,#57497)) ;
#23377=EDGE_LOOP('',(#57498,#57499,#57500,#57501)) ;
#23378=EDGE_LOOP('',(#57502,#57503,#57504,#57505)) ;
#23379=EDGE_LOOP('',(#57506,#57507,#57508,#57509)) ;
#23380=EDGE_LOOP('',(#57510,#57511,#57512,#57513)) ;
#23381=EDGE_LOOP('',(#57514,#57515,#57516,#57517)) ;
#23382=EDGE_LOOP('',(#57518,#57519,#57520)) ;
#23383=EDGE_LOOP('',(#57521,#57522,#57523,#57524)) ;
#23384=EDGE_LOOP('',(#57525,#57526,#57527,#57528)) ;
#23385=EDGE_LOOP('',(#57529,#57530,#57531,#57532)) ;
#23386=EDGE_LOOP('',(#57533,#57534,#57535)) ;
#23387=EDGE_LOOP('',(#57536,#57537,#57538,#57539)) ;
#23388=EDGE_LOOP('',(#57540,#57541,#57542,#57543)) ;
#23389=EDGE_LOOP('',(#57544,#57545,#57546,#57547)) ;
#23390=EDGE_LOOP('',(#57548,#57549,#57550,#57551)) ;
#23391=EDGE_LOOP('',(#57552,#57553,#57554)) ;
#23392=EDGE_LOOP('',(#57555,#57556,#57557)) ;
#23393=EDGE_LOOP('',(#57558,#57559,#57560,#57561)) ;
#23394=EDGE_LOOP('',(#57562,#57563,#57564,#57565,#57566,#57567)) ;
#23395=EDGE_LOOP('',(#57568,#57569,#57570,#57571,#57572,#57573,#57574)) ;
#23396=EDGE_LOOP('',(#57575,#57576,#57577,#57578)) ;
#23397=EDGE_LOOP('',(#57579,#57580,#57581,#57582)) ;
#23398=EDGE_LOOP('',(#57583,#57584,#57585,#57586)) ;
#23399=EDGE_LOOP('',(#57587,#57588,#57589,#57590)) ;
#23400=EDGE_LOOP('',(#57591,#57592,#57593)) ;
#23401=EDGE_LOOP('',(#57594,#57595,#57596,#57597)) ;
#23402=EDGE_LOOP('',(#57598,#57599,#57600,#57601)) ;
#23403=EDGE_LOOP('',(#57602,#57603,#57604,#57605)) ;
#23404=EDGE_LOOP('',(#57606,#57607,#57608,#57609)) ;
#23405=EDGE_LOOP('',(#57610,#57611,#57612,#57613)) ;
#23406=EDGE_LOOP('',(#57614,#57615,#57616,#57617)) ;
#23407=EDGE_LOOP('',(#57618,#57619,#57620,#57621)) ;
#23408=EDGE_LOOP('',(#57622,#57623,#57624,#57625)) ;
#23409=EDGE_LOOP('',(#57626,#57627,#57628,#57629)) ;
#23410=EDGE_LOOP('',(#57630,#57631,#57632)) ;
#23411=EDGE_LOOP('',(#57633,#57634,#57635)) ;
#23412=EDGE_LOOP('',(#57636,#57637,#57638,#57639,#57640)) ;
#23413=EDGE_LOOP('',(#57641,#57642,#57643)) ;
#23414=EDGE_LOOP('',(#57644,#57645,#57646)) ;
#23415=EDGE_LOOP('',(#57647,#57648,#57649,#57650)) ;
#23416=EDGE_LOOP('',(#57651,#57652,#57653,#57654)) ;
#23417=EDGE_LOOP('',(#57655,#57656,#57657,#57658)) ;
#23418=EDGE_LOOP('',(#57659,#57660,#57661,#57662)) ;
#23419=EDGE_LOOP('',(#57663,#57664,#57665,#57666)) ;
#23420=EDGE_LOOP('',(#57667,#57668,#57669,#57670)) ;
#23421=EDGE_LOOP('',(#57671,#57672,#57673,#57674)) ;
#23422=EDGE_LOOP('',(#57675,#57676,#57677)) ;
#23423=EDGE_LOOP('',(#57678,#57679,#57680,#57681)) ;
#23424=EDGE_LOOP('',(#57682,#57683,#57684,#57685)) ;
#23425=EDGE_LOOP('',(#57686,#57687,#57688)) ;
#23426=EDGE_LOOP('',(#57689,#57690,#57691,#57692)) ;
#23427=EDGE_LOOP('',(#57693,#57694,#57695,#57696)) ;
#23428=EDGE_LOOP('',(#57697,#57698,#57699,#57700)) ;
#23429=EDGE_LOOP('',(#57701,#57702,#57703,#57704)) ;
#23430=EDGE_LOOP('',(#57705,#57706,#57707,#57708)) ;
#23431=EDGE_LOOP('',(#57709,#57710,#57711,#57712)) ;
#23432=EDGE_LOOP('',(#57713,#57714,#57715,#57716,#57717)) ;
#23433=EDGE_LOOP('',(#57718,#57719,#57720,#57721)) ;
#23434=EDGE_LOOP('',(#57722,#57723,#57724)) ;
#23435=EDGE_LOOP('',(#57725,#57726,#57727,#57728)) ;
#23436=EDGE_LOOP('',(#57729,#57730,#57731,#57732)) ;
#23437=EDGE_LOOP('',(#57733,#57734,#57735)) ;
#23438=EDGE_LOOP('',(#57736,#57737,#57738,#57739)) ;
#23439=EDGE_LOOP('',(#57740,#57741,#57742,#57743)) ;
#23440=EDGE_LOOP('',(#57744,#57745,#57746,#57747)) ;
#23441=EDGE_LOOP('',(#57748,#57749,#57750)) ;
#23442=EDGE_LOOP('',(#57751,#57752,#57753,#57754)) ;
#23443=EDGE_LOOP('',(#57755,#57756,#57757,#57758)) ;
#23444=EDGE_LOOP('',(#57759,#57760,#57761)) ;
#23445=EDGE_LOOP('',(#57762,#57763,#57764)) ;
#23446=EDGE_LOOP('',(#57765,#57766,#57767,#57768)) ;
#23447=EDGE_LOOP('',(#57769,#57770,#57771,#57772)) ;
#23448=EDGE_LOOP('',(#57773,#57774,#57775)) ;
#23449=EDGE_LOOP('',(#57776,#57777,#57778)) ;
#23450=EDGE_LOOP('',(#57779,#57780,#57781,#57782)) ;
#23451=EDGE_LOOP('',(#57783,#57784,#57785,#57786)) ;
#23452=EDGE_LOOP('',(#57787,#57788,#57789)) ;
#23453=EDGE_LOOP('',(#57790,#57791,#57792,#57793)) ;
#23454=EDGE_LOOP('',(#57794,#57795,#57796,#57797)) ;
#23455=EDGE_LOOP('',(#57798,#57799,#57800)) ;
#23456=EDGE_LOOP('',(#57801,#57802,#57803)) ;
#23457=EDGE_LOOP('',(#57804,#57805,#57806,#57807)) ;
#23458=EDGE_LOOP('',(#57808,#57809,#57810,#57811)) ;
#23459=EDGE_LOOP('',(#57812,#57813,#57814,#57815)) ;
#23460=EDGE_LOOP('',(#57816,#57817,#57818,#57819)) ;
#23461=EDGE_LOOP('',(#57820,#57821,#57822,#57823)) ;
#23462=EDGE_LOOP('',(#57824,#57825,#57826,#57827)) ;
#23463=EDGE_LOOP('',(#57828,#57829,#57830,#57831)) ;
#23464=EDGE_LOOP('',(#57832,#57833,#57834)) ;
#23465=EDGE_LOOP('',(#57835,#57836,#57837)) ;
#23466=EDGE_LOOP('',(#57838,#57839,#57840,#57841)) ;
#23467=EDGE_LOOP('',(#57842,#57843,#57844,#57845,#57846,#57847)) ;
#23468=EDGE_LOOP('',(#57848,#57849,#57850,#57851,#57852,#57853,#57854)) ;
#23469=EDGE_LOOP('',(#57855,#57856,#57857,#57858)) ;
#23470=EDGE_LOOP('',(#57859,#57860,#57861,#57862)) ;
#23471=EDGE_LOOP('',(#57863,#57864,#57865,#57866)) ;
#23472=EDGE_LOOP('',(#57867,#57868,#57869,#57870)) ;
#23473=EDGE_LOOP('',(#57871,#57872,#57873)) ;
#23474=EDGE_LOOP('',(#57874,#57875,#57876,#57877)) ;
#23475=EDGE_LOOP('',(#57878,#57879,#57880,#57881)) ;
#23476=EDGE_LOOP('',(#57882,#57883,#57884,#57885)) ;
#23477=EDGE_LOOP('',(#57886,#57887,#57888,#57889)) ;
#23478=EDGE_LOOP('',(#57890,#57891,#57892,#57893)) ;
#23479=EDGE_LOOP('',(#57894,#57895,#57896,#57897)) ;
#23480=EDGE_LOOP('',(#57898,#57899,#57900,#57901)) ;
#23481=EDGE_LOOP('',(#57902,#57903,#57904,#57905)) ;
#23482=EDGE_LOOP('',(#57906,#57907,#57908,#57909)) ;
#23483=EDGE_LOOP('',(#57910,#57911,#57912)) ;
#23484=EDGE_LOOP('',(#57913,#57914,#57915)) ;
#23485=EDGE_LOOP('',(#57916,#57917,#57918,#57919,#57920)) ;
#23486=EDGE_LOOP('',(#57921,#57922,#57923)) ;
#23487=EDGE_LOOP('',(#57924,#57925,#57926)) ;
#23488=EDGE_LOOP('',(#57927,#57928,#57929,#57930)) ;
#23489=EDGE_LOOP('',(#57931,#57932,#57933,#57934)) ;
#23490=EDGE_LOOP('',(#57935,#57936,#57937,#57938)) ;
#23491=EDGE_LOOP('',(#57939,#57940,#57941,#57942)) ;
#23492=EDGE_LOOP('',(#57943,#57944,#57945,#57946)) ;
#23493=EDGE_LOOP('',(#57947,#57948,#57949,#57950)) ;
#23494=EDGE_LOOP('',(#57951,#57952,#57953,#57954)) ;
#23495=EDGE_LOOP('',(#57955,#57956,#57957)) ;
#23496=EDGE_LOOP('',(#57958,#57959,#57960,#57961)) ;
#23497=EDGE_LOOP('',(#57962,#57963,#57964,#57965)) ;
#23498=EDGE_LOOP('',(#57966,#57967,#57968)) ;
#23499=EDGE_LOOP('',(#57969,#57970,#57971,#57972)) ;
#23500=EDGE_LOOP('',(#57973,#57974,#57975,#57976)) ;
#23501=EDGE_LOOP('',(#57977,#57978,#57979,#57980)) ;
#23502=EDGE_LOOP('',(#57981,#57982,#57983,#57984)) ;
#23503=EDGE_LOOP('',(#57985,#57986,#57987,#57988)) ;
#23504=EDGE_LOOP('',(#57989,#57990,#57991,#57992)) ;
#23505=EDGE_LOOP('',(#57993,#57994,#57995,#57996,#57997)) ;
#23506=EDGE_LOOP('',(#57998,#57999,#58000,#58001)) ;
#23507=EDGE_LOOP('',(#58002,#58003,#58004)) ;
#23508=EDGE_LOOP('',(#58005,#58006,#58007,#58008)) ;
#23509=EDGE_LOOP('',(#58009,#58010,#58011,#58012)) ;
#23510=EDGE_LOOP('',(#58013,#58014,#58015)) ;
#23511=EDGE_LOOP('',(#58016,#58017,#58018,#58019)) ;
#23512=EDGE_LOOP('',(#58020,#58021,#58022,#58023)) ;
#23513=EDGE_LOOP('',(#58024,#58025,#58026,#58027)) ;
#23514=EDGE_LOOP('',(#58028,#58029,#58030)) ;
#23515=EDGE_LOOP('',(#58031,#58032,#58033,#58034)) ;
#23516=EDGE_LOOP('',(#58035,#58036,#58037,#58038)) ;
#23517=EDGE_LOOP('',(#58039,#58040,#58041)) ;
#23518=EDGE_LOOP('',(#58042,#58043,#58044)) ;
#23519=EDGE_LOOP('',(#58045,#58046,#58047,#58048)) ;
#23520=EDGE_LOOP('',(#58049,#58050,#58051,#58052)) ;
#23521=EDGE_LOOP('',(#58053,#58054,#58055)) ;
#23522=EDGE_LOOP('',(#58056,#58057,#58058)) ;
#23523=EDGE_LOOP('',(#58059,#58060,#58061,#58062)) ;
#23524=EDGE_LOOP('',(#58063,#58064,#58065,#58066)) ;
#23525=EDGE_LOOP('',(#58067,#58068,#58069)) ;
#23526=EDGE_LOOP('',(#58070,#58071,#58072,#58073)) ;
#23527=EDGE_LOOP('',(#58074,#58075,#58076,#58077)) ;
#23528=EDGE_LOOP('',(#58078,#58079,#58080)) ;
#23529=EDGE_LOOP('',(#58081,#58082,#58083)) ;
#23530=EDGE_LOOP('',(#58084,#58085,#58086,#58087)) ;
#23531=EDGE_LOOP('',(#58088,#58089,#58090,#58091)) ;
#23532=EDGE_LOOP('',(#58092,#58093,#58094,#58095)) ;
#23533=EDGE_LOOP('',(#58096,#58097,#58098,#58099)) ;
#23534=EDGE_LOOP('',(#58100,#58101,#58102,#58103)) ;
#23535=EDGE_LOOP('',(#58104,#58105,#58106,#58107)) ;
#23536=EDGE_LOOP('',(#58108,#58109,#58110,#58111)) ;
#23537=EDGE_LOOP('',(#58112,#58113,#58114)) ;
#23538=EDGE_LOOP('',(#58115,#58116,#58117)) ;
#23539=EDGE_LOOP('',(#58118,#58119,#58120,#58121)) ;
#23540=EDGE_LOOP('',(#58122,#58123,#58124,#58125,#58126,#58127)) ;
#23541=EDGE_LOOP('',(#58128,#58129,#58130,#58131,#58132,#58133,#58134)) ;
#23542=EDGE_LOOP('',(#58135,#58136,#58137,#58138)) ;
#23543=EDGE_LOOP('',(#58139,#58140,#58141,#58142)) ;
#23544=EDGE_LOOP('',(#58143,#58144,#58145,#58146)) ;
#23545=EDGE_LOOP('',(#58147,#58148,#58149,#58150)) ;
#23546=EDGE_LOOP('',(#58151,#58152,#58153)) ;
#23547=EDGE_LOOP('',(#58154,#58155,#58156,#58157)) ;
#23548=EDGE_LOOP('',(#58158,#58159,#58160,#58161)) ;
#23549=EDGE_LOOP('',(#58162,#58163,#58164,#58165)) ;
#23550=EDGE_LOOP('',(#58166,#58167,#58168,#58169)) ;
#23551=EDGE_LOOP('',(#58170,#58171,#58172,#58173)) ;
#23552=EDGE_LOOP('',(#58174,#58175,#58176,#58177)) ;
#23553=EDGE_LOOP('',(#58178,#58179,#58180,#58181)) ;
#23554=EDGE_LOOP('',(#58182,#58183,#58184,#58185)) ;
#23555=EDGE_LOOP('',(#58186,#58187,#58188,#58189)) ;
#23556=EDGE_LOOP('',(#58190,#58191,#58192)) ;
#23557=EDGE_LOOP('',(#58193,#58194,#58195)) ;
#23558=EDGE_LOOP('',(#58196,#58197,#58198,#58199,#58200)) ;
#23559=EDGE_LOOP('',(#58201,#58202,#58203)) ;
#23560=EDGE_LOOP('',(#58204,#58205,#58206)) ;
#23561=EDGE_LOOP('',(#58207,#58208,#58209,#58210)) ;
#23562=EDGE_LOOP('',(#58211,#58212,#58213,#58214)) ;
#23563=EDGE_LOOP('',(#58215,#58216,#58217,#58218)) ;
#23564=EDGE_LOOP('',(#58219,#58220,#58221,#58222)) ;
#23565=EDGE_LOOP('',(#58223,#58224,#58225,#58226)) ;
#23566=EDGE_LOOP('',(#58227,#58228,#58229,#58230)) ;
#23567=EDGE_LOOP('',(#58231,#58232,#58233,#58234)) ;
#23568=EDGE_LOOP('',(#58235,#58236,#58237)) ;
#23569=EDGE_LOOP('',(#58238,#58239,#58240,#58241)) ;
#23570=EDGE_LOOP('',(#58242,#58243,#58244,#58245)) ;
#23571=EDGE_LOOP('',(#58246,#58247,#58248)) ;
#23572=EDGE_LOOP('',(#58249,#58250,#58251,#58252)) ;
#23573=EDGE_LOOP('',(#58253,#58254,#58255,#58256)) ;
#23574=EDGE_LOOP('',(#58257,#58258,#58259,#58260)) ;
#23575=EDGE_LOOP('',(#58261,#58262,#58263,#58264)) ;
#23576=EDGE_LOOP('',(#58265,#58266,#58267,#58268)) ;
#23577=EDGE_LOOP('',(#58269,#58270,#58271,#58272)) ;
#23578=EDGE_LOOP('',(#58273,#58274,#58275,#58276,#58277)) ;
#23579=EDGE_LOOP('',(#58278,#58279,#58280,#58281)) ;
#23580=EDGE_LOOP('',(#58282,#58283,#58284)) ;
#23581=EDGE_LOOP('',(#58285,#58286,#58287,#58288)) ;
#23582=EDGE_LOOP('',(#58289,#58290,#58291,#58292)) ;
#23583=EDGE_LOOP('',(#58293,#58294,#58295)) ;
#23584=EDGE_LOOP('',(#58296,#58297,#58298,#58299)) ;
#23585=EDGE_LOOP('',(#58300,#58301,#58302,#58303)) ;
#23586=EDGE_LOOP('',(#58304,#58305,#58306,#58307)) ;
#23587=EDGE_LOOP('',(#58308,#58309,#58310)) ;
#23588=EDGE_LOOP('',(#58311,#58312,#58313,#58314)) ;
#23589=EDGE_LOOP('',(#58315,#58316,#58317,#58318)) ;
#23590=EDGE_LOOP('',(#58319,#58320,#58321)) ;
#23591=EDGE_LOOP('',(#58322,#58323,#58324)) ;
#23592=EDGE_LOOP('',(#58325,#58326,#58327,#58328)) ;
#23593=EDGE_LOOP('',(#58329,#58330,#58331,#58332)) ;
#23594=EDGE_LOOP('',(#58333,#58334,#58335)) ;
#23595=EDGE_LOOP('',(#58336,#58337,#58338)) ;
#23596=EDGE_LOOP('',(#58339,#58340,#58341,#58342)) ;
#23597=EDGE_LOOP('',(#58343,#58344,#58345,#58346)) ;
#23598=EDGE_LOOP('',(#58347,#58348,#58349)) ;
#23599=EDGE_LOOP('',(#58350,#58351,#58352,#58353)) ;
#23600=EDGE_LOOP('',(#58354,#58355,#58356,#58357)) ;
#23601=EDGE_LOOP('',(#58358,#58359,#58360)) ;
#23602=EDGE_LOOP('',(#58361,#58362,#58363)) ;
#23603=EDGE_LOOP('',(#58364,#58365,#58366,#58367)) ;
#23604=EDGE_LOOP('',(#58368,#58369,#58370,#58371)) ;
#23605=EDGE_LOOP('',(#58372,#58373,#58374,#58375)) ;
#23606=EDGE_LOOP('',(#58376,#58377,#58378,#58379)) ;
#23607=EDGE_LOOP('',(#58380,#58381,#58382,#58383)) ;
#23608=EDGE_LOOP('',(#58384,#58385,#58386,#58387)) ;
#23609=EDGE_LOOP('',(#58388,#58389,#58390,#58391)) ;
#23610=EDGE_LOOP('',(#58392,#58393,#58394)) ;
#23611=EDGE_LOOP('',(#58395,#58396,#58397)) ;
#23612=EDGE_LOOP('',(#58398,#58399,#58400,#58401)) ;
#23613=EDGE_LOOP('',(#58402,#58403,#58404,#58405,#58406,#58407)) ;
#23614=EDGE_LOOP('',(#58408,#58409,#58410,#58411,#58412,#58413,#58414)) ;
#23615=EDGE_LOOP('',(#58415,#58416,#58417,#58418)) ;
#23616=EDGE_LOOP('',(#58419,#58420,#58421,#58422)) ;
#23617=EDGE_LOOP('',(#58423,#58424,#58425,#58426)) ;
#23618=EDGE_LOOP('',(#58427,#58428,#58429,#58430)) ;
#23619=EDGE_LOOP('',(#58431,#58432,#58433)) ;
#23620=EDGE_LOOP('',(#58434,#58435,#58436,#58437)) ;
#23621=EDGE_LOOP('',(#58438,#58439,#58440,#58441)) ;
#23622=EDGE_LOOP('',(#58442,#58443,#58444,#58445)) ;
#23623=EDGE_LOOP('',(#58446,#58447,#58448,#58449)) ;
#23624=EDGE_LOOP('',(#58450,#58451,#58452,#58453)) ;
#23625=EDGE_LOOP('',(#58454,#58455,#58456,#58457)) ;
#23626=EDGE_LOOP('',(#58458,#58459,#58460,#58461)) ;
#23627=EDGE_LOOP('',(#58462,#58463,#58464,#58465)) ;
#23628=EDGE_LOOP('',(#58466,#58467,#58468,#58469)) ;
#23629=EDGE_LOOP('',(#58470,#58471,#58472)) ;
#23630=EDGE_LOOP('',(#58473,#58474,#58475)) ;
#23631=EDGE_LOOP('',(#58476,#58477,#58478,#58479,#58480)) ;
#23632=EDGE_LOOP('',(#58481,#58482,#58483)) ;
#23633=EDGE_LOOP('',(#58484,#58485,#58486)) ;
#23634=EDGE_LOOP('',(#58487,#58488,#58489,#58490)) ;
#23635=EDGE_LOOP('',(#58491,#58492,#58493,#58494)) ;
#23636=EDGE_LOOP('',(#58495,#58496,#58497,#58498)) ;
#23637=EDGE_LOOP('',(#58499,#58500,#58501,#58502)) ;
#23638=EDGE_LOOP('',(#58503,#58504,#58505,#58506)) ;
#23639=EDGE_LOOP('',(#58507,#58508,#58509,#58510)) ;
#23640=EDGE_LOOP('',(#58511,#58512,#58513,#58514)) ;
#23641=EDGE_LOOP('',(#58515,#58516,#58517)) ;
#23642=EDGE_LOOP('',(#58518,#58519,#58520,#58521)) ;
#23643=EDGE_LOOP('',(#58522,#58523,#58524,#58525)) ;
#23644=EDGE_LOOP('',(#58526,#58527,#58528)) ;
#23645=EDGE_LOOP('',(#58529,#58530,#58531,#58532)) ;
#23646=EDGE_LOOP('',(#58533,#58534,#58535,#58536)) ;
#23647=EDGE_LOOP('',(#58537,#58538,#58539,#58540)) ;
#23648=EDGE_LOOP('',(#58541,#58542,#58543,#58544)) ;
#23649=EDGE_LOOP('',(#58545,#58546,#58547,#58548)) ;
#23650=EDGE_LOOP('',(#58549,#58550,#58551,#58552)) ;
#23651=EDGE_LOOP('',(#58553,#58554,#58555,#58556,#58557)) ;
#23652=EDGE_LOOP('',(#58558,#58559,#58560,#58561)) ;
#23653=EDGE_LOOP('',(#58562,#58563,#58564)) ;
#23654=EDGE_LOOP('',(#58565,#58566,#58567,#58568)) ;
#23655=EDGE_LOOP('',(#58569,#58570,#58571,#58572)) ;
#23656=EDGE_LOOP('',(#58573,#58574,#58575)) ;
#23657=EDGE_LOOP('',(#58576,#58577,#58578,#58579)) ;
#23658=EDGE_LOOP('',(#58580,#58581,#58582,#58583)) ;
#23659=EDGE_LOOP('',(#58584,#58585,#58586,#58587)) ;
#23660=EDGE_LOOP('',(#58588,#58589,#58590)) ;
#23661=EDGE_LOOP('',(#58591,#58592,#58593,#58594)) ;
#23662=EDGE_LOOP('',(#58595,#58596,#58597,#58598)) ;
#23663=EDGE_LOOP('',(#58599,#58600,#58601)) ;
#23664=EDGE_LOOP('',(#58602,#58603,#58604)) ;
#23665=EDGE_LOOP('',(#58605,#58606,#58607,#58608)) ;
#23666=EDGE_LOOP('',(#58609,#58610,#58611,#58612)) ;
#23667=EDGE_LOOP('',(#58613,#58614,#58615)) ;
#23668=EDGE_LOOP('',(#58616,#58617,#58618)) ;
#23669=EDGE_LOOP('',(#58619,#58620,#58621,#58622)) ;
#23670=EDGE_LOOP('',(#58623,#58624,#58625,#58626)) ;
#23671=EDGE_LOOP('',(#58627,#58628,#58629)) ;
#23672=EDGE_LOOP('',(#58630,#58631,#58632,#58633)) ;
#23673=EDGE_LOOP('',(#58634,#58635,#58636,#58637)) ;
#23674=EDGE_LOOP('',(#58638,#58639,#58640)) ;
#23675=EDGE_LOOP('',(#58641,#58642,#58643)) ;
#23676=EDGE_LOOP('',(#58644,#58645,#58646,#58647)) ;
#23677=EDGE_LOOP('',(#58648,#58649,#58650,#58651)) ;
#23678=EDGE_LOOP('',(#58652,#58653,#58654,#58655)) ;
#23679=EDGE_LOOP('',(#58656,#58657,#58658,#58659)) ;
#23680=EDGE_LOOP('',(#58660,#58661,#58662,#58663)) ;
#23681=EDGE_LOOP('',(#58664,#58665,#58666,#58667)) ;
#23682=EDGE_LOOP('',(#58668,#58669,#58670,#58671)) ;
#23683=EDGE_LOOP('',(#58672,#58673,#58674)) ;
#23684=EDGE_LOOP('',(#58675,#58676,#58677)) ;
#23685=EDGE_LOOP('',(#58678,#58679,#58680,#58681)) ;
#23686=EDGE_LOOP('',(#58682,#58683,#58684,#58685,#58686,#58687)) ;
#23687=EDGE_LOOP('',(#58688,#58689,#58690,#58691,#58692,#58693,#58694)) ;
#23688=EDGE_LOOP('',(#58695,#58696,#58697,#58698)) ;
#23689=EDGE_LOOP('',(#58699,#58700,#58701,#58702)) ;
#23690=EDGE_LOOP('',(#58703,#58704,#58705,#58706)) ;
#23691=EDGE_LOOP('',(#58707,#58708,#58709,#58710)) ;
#23692=EDGE_LOOP('',(#58711,#58712,#58713)) ;
#23693=EDGE_LOOP('',(#58714,#58715,#58716,#58717)) ;
#23694=EDGE_LOOP('',(#58718,#58719,#58720,#58721)) ;
#23695=EDGE_LOOP('',(#58722,#58723,#58724,#58725)) ;
#23696=EDGE_LOOP('',(#58726,#58727,#58728,#58729)) ;
#23697=EDGE_LOOP('',(#58730,#58731,#58732,#58733)) ;
#23698=EDGE_LOOP('',(#58734,#58735,#58736,#58737)) ;
#23699=EDGE_LOOP('',(#58738,#58739,#58740,#58741)) ;
#23700=EDGE_LOOP('',(#58742,#58743,#58744,#58745)) ;
#23701=EDGE_LOOP('',(#58746,#58747,#58748,#58749)) ;
#23702=EDGE_LOOP('',(#58750,#58751,#58752)) ;
#23703=EDGE_LOOP('',(#58753,#58754,#58755)) ;
#23704=EDGE_LOOP('',(#58756,#58757,#58758,#58759,#58760)) ;
#23705=EDGE_LOOP('',(#58761,#58762,#58763)) ;
#23706=EDGE_LOOP('',(#58764,#58765,#58766)) ;
#23707=EDGE_LOOP('',(#58767,#58768,#58769,#58770)) ;
#23708=EDGE_LOOP('',(#58771,#58772,#58773,#58774)) ;
#23709=EDGE_LOOP('',(#58775,#58776,#58777,#58778)) ;
#23710=EDGE_LOOP('',(#58779,#58780,#58781,#58782)) ;
#23711=EDGE_LOOP('',(#58783,#58784,#58785,#58786)) ;
#23712=EDGE_LOOP('',(#58787,#58788,#58789,#58790)) ;
#23713=EDGE_LOOP('',(#58791,#58792,#58793,#58794)) ;
#23714=EDGE_LOOP('',(#58795,#58796,#58797)) ;
#23715=EDGE_LOOP('',(#58798,#58799,#58800,#58801)) ;
#23716=EDGE_LOOP('',(#58802,#58803,#58804,#58805)) ;
#23717=EDGE_LOOP('',(#58806,#58807,#58808)) ;
#23718=EDGE_LOOP('',(#58809,#58810,#58811,#58812)) ;
#23719=EDGE_LOOP('',(#58813,#58814,#58815,#58816)) ;
#23720=EDGE_LOOP('',(#58817,#58818,#58819,#58820)) ;
#23721=EDGE_LOOP('',(#58821,#58822,#58823,#58824)) ;
#23722=EDGE_LOOP('',(#58825,#58826,#58827,#58828)) ;
#23723=EDGE_LOOP('',(#58829,#58830,#58831,#58832)) ;
#23724=EDGE_LOOP('',(#58833,#58834,#58835,#58836,#58837)) ;
#23725=EDGE_LOOP('',(#58838,#58839,#58840,#58841)) ;
#23726=EDGE_LOOP('',(#58842,#58843,#58844)) ;
#23727=EDGE_LOOP('',(#58845,#58846,#58847,#58848)) ;
#23728=EDGE_LOOP('',(#58849,#58850,#58851,#58852)) ;
#23729=EDGE_LOOP('',(#58853,#58854,#58855)) ;
#23730=EDGE_LOOP('',(#58856,#58857,#58858,#58859)) ;
#23731=EDGE_LOOP('',(#58860,#58861,#58862,#58863)) ;
#23732=EDGE_LOOP('',(#58864,#58865,#58866,#58867)) ;
#23733=EDGE_LOOP('',(#58868,#58869,#58870)) ;
#23734=EDGE_LOOP('',(#58871,#58872,#58873,#58874)) ;
#23735=EDGE_LOOP('',(#58875,#58876,#58877,#58878)) ;
#23736=EDGE_LOOP('',(#58879,#58880,#58881)) ;
#23737=EDGE_LOOP('',(#58882,#58883,#58884)) ;
#23738=EDGE_LOOP('',(#58885,#58886,#58887,#58888)) ;
#23739=EDGE_LOOP('',(#58889,#58890,#58891,#58892)) ;
#23740=EDGE_LOOP('',(#58893,#58894,#58895)) ;
#23741=EDGE_LOOP('',(#58896,#58897,#58898)) ;
#23742=EDGE_LOOP('',(#58899,#58900,#58901,#58902)) ;
#23743=EDGE_LOOP('',(#58903,#58904,#58905,#58906)) ;
#23744=EDGE_LOOP('',(#58907,#58908,#58909)) ;
#23745=EDGE_LOOP('',(#58910,#58911,#58912,#58913)) ;
#23746=EDGE_LOOP('',(#58914,#58915,#58916,#58917)) ;
#23747=EDGE_LOOP('',(#58918,#58919,#58920)) ;
#23748=EDGE_LOOP('',(#58921,#58922,#58923)) ;
#23749=EDGE_LOOP('',(#58924,#58925,#58926,#58927)) ;
#23750=EDGE_LOOP('',(#58928,#58929,#58930,#58931)) ;
#23751=EDGE_LOOP('',(#58932,#58933,#58934,#58935)) ;
#23752=EDGE_LOOP('',(#58936,#58937,#58938,#58939)) ;
#23753=EDGE_LOOP('',(#58940,#58941,#58942,#58943)) ;
#23754=EDGE_LOOP('',(#58944,#58945,#58946,#58947)) ;
#23755=EDGE_LOOP('',(#58948,#58949,#58950,#58951)) ;
#23756=EDGE_LOOP('',(#58952,#58953,#58954)) ;
#23757=EDGE_LOOP('',(#58955,#58956,#58957)) ;
#23758=EDGE_LOOP('',(#58958,#58959,#58960,#58961)) ;
#23759=EDGE_LOOP('',(#58962,#58963,#58964,#58965,#58966,#58967)) ;
#23760=EDGE_LOOP('',(#58968,#58969,#58970,#58971,#58972,#58973,#58974)) ;
#23761=EDGE_LOOP('',(#58975,#58976,#58977,#58978)) ;
#23762=EDGE_LOOP('',(#58979,#58980,#58981,#58982)) ;
#23763=EDGE_LOOP('',(#58983,#58984,#58985,#58986)) ;
#23764=EDGE_LOOP('',(#58987,#58988,#58989,#58990)) ;
#23765=EDGE_LOOP('',(#58991,#58992,#58993)) ;
#23766=EDGE_LOOP('',(#58994,#58995,#58996,#58997)) ;
#23767=EDGE_LOOP('',(#58998,#58999,#59000,#59001)) ;
#23768=EDGE_LOOP('',(#59002,#59003,#59004,#59005)) ;
#23769=EDGE_LOOP('',(#59006,#59007,#59008,#59009)) ;
#23770=EDGE_LOOP('',(#59010,#59011,#59012,#59013)) ;
#23771=EDGE_LOOP('',(#59014,#59015,#59016,#59017)) ;
#23772=EDGE_LOOP('',(#59018,#59019,#59020,#59021)) ;
#23773=EDGE_LOOP('',(#59022,#59023,#59024,#59025)) ;
#23774=EDGE_LOOP('',(#59026,#59027,#59028,#59029)) ;
#23775=EDGE_LOOP('',(#59030,#59031,#59032)) ;
#23776=EDGE_LOOP('',(#59033,#59034,#59035)) ;
#23777=EDGE_LOOP('',(#59036,#59037,#59038,#59039,#59040)) ;
#23778=EDGE_LOOP('',(#59041,#59042,#59043)) ;
#23779=EDGE_LOOP('',(#59044,#59045,#59046)) ;
#23780=EDGE_LOOP('',(#59047,#59048,#59049,#59050)) ;
#23781=EDGE_LOOP('',(#59051,#59052,#59053,#59054)) ;
#23782=EDGE_LOOP('',(#59055,#59056,#59057,#59058)) ;
#23783=EDGE_LOOP('',(#59059,#59060,#59061,#59062)) ;
#23784=EDGE_LOOP('',(#59063,#59064,#59065,#59066)) ;
#23785=EDGE_LOOP('',(#59067,#59068,#59069,#59070)) ;
#23786=EDGE_LOOP('',(#59071,#59072,#59073,#59074)) ;
#23787=EDGE_LOOP('',(#59075,#59076,#59077)) ;
#23788=EDGE_LOOP('',(#59078,#59079,#59080,#59081)) ;
#23789=EDGE_LOOP('',(#59082,#59083,#59084,#59085)) ;
#23790=EDGE_LOOP('',(#59086,#59087,#59088)) ;
#23791=EDGE_LOOP('',(#59089,#59090,#59091,#59092)) ;
#23792=EDGE_LOOP('',(#59093,#59094,#59095,#59096)) ;
#23793=EDGE_LOOP('',(#59097,#59098,#59099,#59100)) ;
#23794=EDGE_LOOP('',(#59101,#59102,#59103,#59104)) ;
#23795=EDGE_LOOP('',(#59105,#59106,#59107,#59108)) ;
#23796=EDGE_LOOP('',(#59109,#59110,#59111,#59112)) ;
#23797=EDGE_LOOP('',(#59113,#59114,#59115,#59116,#59117)) ;
#23798=EDGE_LOOP('',(#59118,#59119,#59120,#59121)) ;
#23799=EDGE_LOOP('',(#59122,#59123,#59124)) ;
#23800=EDGE_LOOP('',(#59125,#59126,#59127,#59128)) ;
#23801=EDGE_LOOP('',(#59129,#59130,#59131,#59132)) ;
#23802=EDGE_LOOP('',(#59133,#59134,#59135)) ;
#23803=EDGE_LOOP('',(#59136,#59137,#59138,#59139)) ;
#23804=EDGE_LOOP('',(#59140,#59141,#59142,#59143)) ;
#23805=EDGE_LOOP('',(#59144,#59145,#59146,#59147)) ;
#23806=EDGE_LOOP('',(#59148,#59149,#59150)) ;
#23807=EDGE_LOOP('',(#59151,#59152,#59153,#59154)) ;
#23808=EDGE_LOOP('',(#59155,#59156,#59157,#59158)) ;
#23809=EDGE_LOOP('',(#59159,#59160,#59161)) ;
#23810=EDGE_LOOP('',(#59162,#59163,#59164)) ;
#23811=EDGE_LOOP('',(#59165,#59166,#59167,#59168)) ;
#23812=EDGE_LOOP('',(#59169,#59170,#59171,#59172)) ;
#23813=EDGE_LOOP('',(#59173,#59174,#59175)) ;
#23814=EDGE_LOOP('',(#59176,#59177,#59178)) ;
#23815=EDGE_LOOP('',(#59179,#59180,#59181,#59182)) ;
#23816=EDGE_LOOP('',(#59183,#59184,#59185,#59186)) ;
#23817=EDGE_LOOP('',(#59187,#59188,#59189)) ;
#23818=EDGE_LOOP('',(#59190,#59191,#59192,#59193)) ;
#23819=EDGE_LOOP('',(#59194,#59195,#59196,#59197)) ;
#23820=EDGE_LOOP('',(#59198,#59199,#59200)) ;
#23821=EDGE_LOOP('',(#59201,#59202,#59203)) ;
#23822=EDGE_LOOP('',(#59204,#59205,#59206,#59207)) ;
#23823=EDGE_LOOP('',(#59208,#59209,#59210,#59211)) ;
#23824=EDGE_LOOP('',(#59212,#59213,#59214,#59215)) ;
#23825=EDGE_LOOP('',(#59216,#59217,#59218,#59219)) ;
#23826=EDGE_LOOP('',(#59220,#59221,#59222,#59223)) ;
#23827=EDGE_LOOP('',(#59224,#59225,#59226,#59227)) ;
#23828=EDGE_LOOP('',(#59228,#59229,#59230,#59231)) ;
#23829=EDGE_LOOP('',(#59232,#59233,#59234)) ;
#23830=EDGE_LOOP('',(#59235,#59236,#59237)) ;
#23831=EDGE_LOOP('',(#59238,#59239,#59240,#59241)) ;
#23832=EDGE_LOOP('',(#59242,#59243,#59244,#59245,#59246,#59247)) ;
#23833=EDGE_LOOP('',(#59248,#59249,#59250,#59251,#59252,#59253,#59254)) ;
#23834=EDGE_LOOP('',(#59255,#59256,#59257,#59258)) ;
#23835=EDGE_LOOP('',(#59259,#59260,#59261,#59262)) ;
#23836=EDGE_LOOP('',(#59263,#59264,#59265,#59266)) ;
#23837=EDGE_LOOP('',(#59267,#59268,#59269,#59270)) ;
#23838=EDGE_LOOP('',(#59271,#59272,#59273)) ;
#23839=EDGE_LOOP('',(#59274,#59275,#59276,#59277)) ;
#23840=EDGE_LOOP('',(#59278,#59279,#59280,#59281)) ;
#23841=EDGE_LOOP('',(#59282,#59283,#59284,#59285)) ;
#23842=EDGE_LOOP('',(#59286,#59287,#59288,#59289)) ;
#23843=EDGE_LOOP('',(#59290,#59291,#59292,#59293)) ;
#23844=EDGE_LOOP('',(#59294,#59295,#59296,#59297)) ;
#23845=EDGE_LOOP('',(#59298,#59299,#59300,#59301)) ;
#23846=EDGE_LOOP('',(#59302,#59303,#59304,#59305)) ;
#23847=EDGE_LOOP('',(#59306,#59307,#59308,#59309)) ;
#23848=EDGE_LOOP('',(#59310,#59311,#59312)) ;
#23849=EDGE_LOOP('',(#59313,#59314,#59315)) ;
#23850=EDGE_LOOP('',(#59316,#59317,#59318,#59319,#59320)) ;
#23851=EDGE_LOOP('',(#59321,#59322,#59323)) ;
#23852=EDGE_LOOP('',(#59324,#59325,#59326)) ;
#23853=EDGE_LOOP('',(#59327,#59328,#59329,#59330)) ;
#23854=EDGE_LOOP('',(#59331,#59332,#59333,#59334)) ;
#23855=EDGE_LOOP('',(#59335,#59336,#59337,#59338)) ;
#23856=EDGE_LOOP('',(#59339,#59340,#59341,#59342)) ;
#23857=EDGE_LOOP('',(#59343,#59344,#59345,#59346)) ;
#23858=EDGE_LOOP('',(#59347,#59348,#59349,#59350)) ;
#23859=EDGE_LOOP('',(#59351,#59352,#59353,#59354)) ;
#23860=EDGE_LOOP('',(#59355,#59356,#59357)) ;
#23861=EDGE_LOOP('',(#59358,#59359,#59360,#59361)) ;
#23862=EDGE_LOOP('',(#59362,#59363,#59364,#59365)) ;
#23863=EDGE_LOOP('',(#59366,#59367,#59368)) ;
#23864=EDGE_LOOP('',(#59369,#59370,#59371,#59372)) ;
#23865=EDGE_LOOP('',(#59373,#59374,#59375,#59376)) ;
#23866=EDGE_LOOP('',(#59377,#59378,#59379,#59380)) ;
#23867=EDGE_LOOP('',(#59381,#59382,#59383,#59384)) ;
#23868=EDGE_LOOP('',(#59385,#59386,#59387,#59388)) ;
#23869=EDGE_LOOP('',(#59389,#59390,#59391,#59392)) ;
#23870=EDGE_LOOP('',(#59393,#59394,#59395,#59396,#59397)) ;
#23871=EDGE_LOOP('',(#59398,#59399,#59400,#59401)) ;
#23872=EDGE_LOOP('',(#59402,#59403,#59404)) ;
#23873=EDGE_LOOP('',(#59405,#59406,#59407,#59408)) ;
#23874=EDGE_LOOP('',(#59409,#59410,#59411,#59412)) ;
#23875=EDGE_LOOP('',(#59413,#59414,#59415)) ;
#23876=EDGE_LOOP('',(#59416,#59417,#59418,#59419)) ;
#23877=EDGE_LOOP('',(#59420,#59421,#59422,#59423)) ;
#23878=EDGE_LOOP('',(#59424,#59425,#59426,#59427)) ;
#23879=EDGE_LOOP('',(#59428,#59429,#59430)) ;
#23880=EDGE_LOOP('',(#59431,#59432,#59433,#59434)) ;
#23881=EDGE_LOOP('',(#59435,#59436,#59437,#59438)) ;
#23882=EDGE_LOOP('',(#59439,#59440,#59441)) ;
#23883=EDGE_LOOP('',(#59442,#59443,#59444)) ;
#23884=EDGE_LOOP('',(#59445,#59446,#59447,#59448)) ;
#23885=EDGE_LOOP('',(#59449,#59450,#59451,#59452)) ;
#23886=EDGE_LOOP('',(#59453,#59454,#59455)) ;
#23887=EDGE_LOOP('',(#59456,#59457,#59458)) ;
#23888=EDGE_LOOP('',(#59459,#59460,#59461,#59462)) ;
#23889=EDGE_LOOP('',(#59463,#59464,#59465,#59466)) ;
#23890=EDGE_LOOP('',(#59467,#59468,#59469)) ;
#23891=EDGE_LOOP('',(#59470,#59471,#59472,#59473)) ;
#23892=EDGE_LOOP('',(#59474,#59475,#59476,#59477)) ;
#23893=EDGE_LOOP('',(#59478,#59479,#59480)) ;
#23894=EDGE_LOOP('',(#59481,#59482,#59483)) ;
#23895=EDGE_LOOP('',(#59484,#59485,#59486,#59487)) ;
#23896=EDGE_LOOP('',(#59488,#59489,#59490,#59491)) ;
#23897=EDGE_LOOP('',(#59492,#59493,#59494,#59495)) ;
#23898=EDGE_LOOP('',(#59496,#59497,#59498,#59499)) ;
#23899=EDGE_LOOP('',(#59500,#59501,#59502,#59503)) ;
#23900=EDGE_LOOP('',(#59504,#59505,#59506,#59507)) ;
#23901=EDGE_LOOP('',(#59508,#59509,#59510,#59511)) ;
#23902=EDGE_LOOP('',(#59512,#59513,#59514)) ;
#23903=EDGE_LOOP('',(#59515,#59516,#59517)) ;
#23904=EDGE_LOOP('',(#59518,#59519,#59520,#59521)) ;
#23905=EDGE_LOOP('',(#59522,#59523,#59524,#59525,#59526,#59527)) ;
#23906=EDGE_LOOP('',(#59528,#59529,#59530,#59531,#59532,#59533,#59534)) ;
#23907=EDGE_LOOP('',(#59535,#59536,#59537,#59538)) ;
#23908=EDGE_LOOP('',(#59539,#59540,#59541,#59542)) ;
#23909=EDGE_LOOP('',(#59543,#59544,#59545,#59546)) ;
#23910=EDGE_LOOP('',(#59547,#59548,#59549,#59550)) ;
#23911=EDGE_LOOP('',(#59551,#59552,#59553)) ;
#23912=EDGE_LOOP('',(#59554,#59555,#59556,#59557)) ;
#23913=EDGE_LOOP('',(#59558,#59559,#59560,#59561)) ;
#23914=EDGE_LOOP('',(#59562,#59563,#59564,#59565)) ;
#23915=EDGE_LOOP('',(#59566,#59567,#59568,#59569)) ;
#23916=EDGE_LOOP('',(#59570,#59571,#59572,#59573)) ;
#23917=EDGE_LOOP('',(#59574,#59575,#59576,#59577)) ;
#23918=EDGE_LOOP('',(#59578,#59579,#59580,#59581)) ;
#23919=EDGE_LOOP('',(#59582,#59583,#59584,#59585)) ;
#23920=EDGE_LOOP('',(#59586,#59587,#59588,#59589)) ;
#23921=EDGE_LOOP('',(#59590,#59591,#59592)) ;
#23922=EDGE_LOOP('',(#59593,#59594,#59595)) ;
#23923=EDGE_LOOP('',(#59596,#59597,#59598,#59599,#59600)) ;
#23924=EDGE_LOOP('',(#59601,#59602,#59603)) ;
#23925=EDGE_LOOP('',(#59604,#59605,#59606)) ;
#23926=EDGE_LOOP('',(#59607,#59608,#59609,#59610)) ;
#23927=EDGE_LOOP('',(#59611,#59612,#59613,#59614)) ;
#23928=EDGE_LOOP('',(#59615,#59616,#59617,#59618)) ;
#23929=EDGE_LOOP('',(#59619,#59620,#59621,#59622)) ;
#23930=EDGE_LOOP('',(#59623,#59624,#59625,#59626)) ;
#23931=EDGE_LOOP('',(#59627,#59628,#59629,#59630)) ;
#23932=EDGE_LOOP('',(#59631,#59632,#59633,#59634)) ;
#23933=EDGE_LOOP('',(#59635,#59636,#59637)) ;
#23934=EDGE_LOOP('',(#59638,#59639,#59640,#59641)) ;
#23935=EDGE_LOOP('',(#59642,#59643,#59644,#59645)) ;
#23936=EDGE_LOOP('',(#59646,#59647,#59648)) ;
#23937=EDGE_LOOP('',(#59649,#59650,#59651,#59652)) ;
#23938=EDGE_LOOP('',(#59653,#59654,#59655,#59656)) ;
#23939=EDGE_LOOP('',(#59657,#59658,#59659,#59660)) ;
#23940=EDGE_LOOP('',(#59661,#59662,#59663,#59664)) ;
#23941=EDGE_LOOP('',(#59665,#59666,#59667,#59668)) ;
#23942=EDGE_LOOP('',(#59669,#59670,#59671,#59672)) ;
#23943=EDGE_LOOP('',(#59673,#59674,#59675,#59676,#59677)) ;
#23944=EDGE_LOOP('',(#59678,#59679,#59680,#59681)) ;
#23945=EDGE_LOOP('',(#59682,#59683,#59684)) ;
#23946=EDGE_LOOP('',(#59685,#59686,#59687,#59688)) ;
#23947=EDGE_LOOP('',(#59689,#59690,#59691,#59692)) ;
#23948=EDGE_LOOP('',(#59693,#59694,#59695)) ;
#23949=EDGE_LOOP('',(#59696,#59697,#59698,#59699)) ;
#23950=EDGE_LOOP('',(#59700,#59701,#59702,#59703)) ;
#23951=EDGE_LOOP('',(#59704,#59705,#59706,#59707)) ;
#23952=EDGE_LOOP('',(#59708,#59709,#59710)) ;
#23953=EDGE_LOOP('',(#59711,#59712,#59713,#59714)) ;
#23954=EDGE_LOOP('',(#59715,#59716,#59717,#59718)) ;
#23955=EDGE_LOOP('',(#59719,#59720,#59721)) ;
#23956=EDGE_LOOP('',(#59722,#59723,#59724)) ;
#23957=EDGE_LOOP('',(#59725,#59726,#59727,#59728)) ;
#23958=EDGE_LOOP('',(#59729,#59730,#59731,#59732)) ;
#23959=EDGE_LOOP('',(#59733,#59734,#59735)) ;
#23960=EDGE_LOOP('',(#59736,#59737,#59738)) ;
#23961=EDGE_LOOP('',(#59739,#59740,#59741,#59742)) ;
#23962=EDGE_LOOP('',(#59743,#59744,#59745,#59746)) ;
#23963=EDGE_LOOP('',(#59747,#59748,#59749)) ;
#23964=EDGE_LOOP('',(#59750,#59751,#59752,#59753)) ;
#23965=EDGE_LOOP('',(#59754,#59755,#59756,#59757)) ;
#23966=EDGE_LOOP('',(#59758,#59759,#59760)) ;
#23967=EDGE_LOOP('',(#59761,#59762,#59763)) ;
#23968=EDGE_LOOP('',(#59764,#59765,#59766,#59767)) ;
#23969=EDGE_LOOP('',(#59768,#59769,#59770,#59771)) ;
#23970=EDGE_LOOP('',(#59772,#59773,#59774,#59775)) ;
#23971=EDGE_LOOP('',(#59776,#59777,#59778,#59779)) ;
#23972=EDGE_LOOP('',(#59780,#59781,#59782,#59783)) ;
#23973=EDGE_LOOP('',(#59784,#59785,#59786,#59787)) ;
#23974=EDGE_LOOP('',(#59788,#59789,#59790,#59791)) ;
#23975=EDGE_LOOP('',(#59792,#59793,#59794,#59795)) ;
#23976=EDGE_LOOP('',(#59796,#59797,#59798,#59799)) ;
#23977=EDGE_LOOP('',(#59800,#59801,#59802,#59803)) ;
#23978=EDGE_LOOP('',(#59804,#59805,#59806,#59807,#59808,#59809)) ;
#23979=EDGE_LOOP('',(#59810,#59811,#59812,#59813,#59814,#59815)) ;
#23980=EDGE_LOOP('',(#59816,#59817,#59818,#59819,#59820)) ;
#23981=EDGE_LOOP('',(#59821,#59822,#59823,#59824)) ;
#23982=EDGE_LOOP('',(#59825,#59826,#59827,#59828)) ;
#23983=EDGE_LOOP('',(#59829,#59830,#59831,#59832)) ;
#23984=EDGE_LOOP('',(#59833,#59834,#59835,#59836)) ;
#23985=EDGE_LOOP('',(#59837,#59838,#59839,#59840)) ;
#23986=EDGE_LOOP('',(#59841,#59842,#59843,#59844)) ;
#23987=EDGE_LOOP('',(#59845,#59846,#59847,#59848)) ;
#23988=EDGE_LOOP('',(#59849,#59850,#59851,#59852)) ;
#23989=EDGE_LOOP('',(#59853,#59854,#59855,#59856)) ;
#23990=EDGE_LOOP('',(#59857,#59858,#59859,#59860)) ;
#23991=EDGE_LOOP('',(#59861,#59862,#59863,#59864)) ;
#23992=EDGE_LOOP('',(#59865,#59866,#59867,#59868)) ;
#23993=EDGE_LOOP('',(#59869,#59870,#59871,#59872)) ;
#23994=EDGE_LOOP('',(#59873,#59874,#59875,#59876,#59877,#59878)) ;
#23995=EDGE_LOOP('',(#59879,#59880,#59881,#59882,#59883,#59884)) ;
#23996=EDGE_LOOP('',(#59885,#59886,#59887,#59888,#59889)) ;
#23997=EDGE_LOOP('',(#59890,#59891,#59892,#59893)) ;
#23998=EDGE_LOOP('',(#59894,#59895,#59896,#59897)) ;
#23999=EDGE_LOOP('',(#59898,#59899,#59900,#59901)) ;
#24000=EDGE_LOOP('',(#59902,#59903,#59904,#59905)) ;
#24001=EDGE_LOOP('',(#59906,#59907,#59908,#59909)) ;
#24002=EDGE_LOOP('',(#59910,#59911,#59912,#59913)) ;
#24003=EDGE_LOOP('',(#59914,#59915,#59916,#59917)) ;
#24004=EDGE_LOOP('',(#59918,#59919,#59920,#59921)) ;
#24005=EDGE_LOOP('',(#59922,#59923,#59924,#59925)) ;
#24006=EDGE_LOOP('',(#59926,#59927,#59928,#59929)) ;
#24007=EDGE_LOOP('',(#59930,#59931,#59932,#59933)) ;
#24008=EDGE_LOOP('',(#59934,#59935,#59936,#59937)) ;
#24009=EDGE_LOOP('',(#59938,#59939,#59940,#59941)) ;
#24010=EDGE_LOOP('',(#59942,#59943,#59944,#59945,#59946,#59947)) ;
#24011=EDGE_LOOP('',(#59948,#59949,#59950,#59951,#59952,#59953)) ;
#24012=EDGE_LOOP('',(#59954,#59955,#59956,#59957,#59958)) ;
#24013=EDGE_LOOP('',(#59959,#59960,#59961,#59962)) ;
#24014=EDGE_LOOP('',(#59963,#59964,#59965,#59966)) ;
#24015=EDGE_LOOP('',(#59967,#59968,#59969,#59970)) ;
#24016=EDGE_LOOP('',(#59971,#59972,#59973,#59974)) ;
#24017=EDGE_LOOP('',(#59975,#59976,#59977,#59978)) ;
#24018=EDGE_LOOP('',(#59979,#59980,#59981,#59982)) ;
#24019=EDGE_LOOP('',(#59983,#59984,#59985,#59986)) ;
#24020=EDGE_LOOP('',(#59987,#59988,#59989,#59990)) ;
#24021=EDGE_LOOP('',(#59991,#59992,#59993,#59994)) ;
#24022=EDGE_LOOP('',(#59995,#59996,#59997,#59998)) ;
#24023=EDGE_LOOP('',(#59999,#60000,#60001,#60002)) ;
#24024=EDGE_LOOP('',(#60003,#60004,#60005,#60006)) ;
#24025=EDGE_LOOP('',(#60007,#60008,#60009,#60010)) ;
#24026=EDGE_LOOP('',(#60011,#60012,#60013,#60014,#60015,#60016)) ;
#24027=EDGE_LOOP('',(#60017,#60018,#60019,#60020,#60021,#60022)) ;
#24028=EDGE_LOOP('',(#60023,#60024,#60025,#60026,#60027)) ;
#24029=EDGE_LOOP('',(#60028,#60029,#60030,#60031)) ;
#24030=EDGE_LOOP('',(#60032,#60033,#60034,#60035)) ;
#24031=EDGE_LOOP('',(#60036,#60037,#60038,#60039)) ;
#24032=EDGE_LOOP('',(#60040,#60041,#60042,#60043)) ;
#24033=EDGE_LOOP('',(#60044,#60045,#60046,#60047)) ;
#24034=EDGE_LOOP('',(#60048,#60049,#60050,#60051)) ;
#24035=EDGE_LOOP('',(#60052,#60053,#60054,#60055)) ;
#24036=EDGE_LOOP('',(#60056,#60057,#60058,#60059)) ;
#24037=EDGE_LOOP('',(#60060,#60061,#60062,#60063)) ;
#24038=EDGE_LOOP('',(#60064,#60065,#60066,#60067)) ;
#24039=EDGE_LOOP('',(#60068,#60069,#60070,#60071)) ;
#24040=EDGE_LOOP('',(#60072,#60073,#60074,#60075)) ;
#24041=EDGE_LOOP('',(#60076,#60077,#60078,#60079)) ;
#24042=EDGE_LOOP('',(#60080,#60081,#60082,#60083,#60084,#60085)) ;
#24043=EDGE_LOOP('',(#60086,#60087,#60088,#60089,#60090,#60091)) ;
#24044=EDGE_LOOP('',(#60092,#60093,#60094,#60095,#60096)) ;
#24045=EDGE_LOOP('',(#60097,#60098,#60099,#60100)) ;
#24046=EDGE_LOOP('',(#60101,#60102,#60103,#60104)) ;
#24047=EDGE_LOOP('',(#60105,#60106,#60107,#60108)) ;
#24048=EDGE_LOOP('',(#60109,#60110,#60111,#60112)) ;
#24049=EDGE_LOOP('',(#60113,#60114,#60115,#60116)) ;
#24050=EDGE_LOOP('',(#60117,#60118,#60119,#60120)) ;
#24051=EDGE_LOOP('',(#60121,#60122,#60123,#60124)) ;
#24052=EDGE_LOOP('',(#60125,#60126,#60127,#60128)) ;
#24053=EDGE_LOOP('',(#60129,#60130,#60131,#60132)) ;
#24054=EDGE_LOOP('',(#60133,#60134,#60135,#60136)) ;
#24055=EDGE_LOOP('',(#60137,#60138,#60139,#60140)) ;
#24056=EDGE_LOOP('',(#60141,#60142,#60143,#60144)) ;
#24057=EDGE_LOOP('',(#60145,#60146,#60147,#60148)) ;
#24058=EDGE_LOOP('',(#60149,#60150,#60151,#60152,#60153,#60154)) ;
#24059=EDGE_LOOP('',(#60155,#60156,#60157,#60158,#60159,#60160)) ;
#24060=EDGE_LOOP('',(#60161,#60162,#60163,#60164,#60165)) ;
#24061=EDGE_LOOP('',(#60166,#60167,#60168,#60169)) ;
#24062=EDGE_LOOP('',(#60170,#60171,#60172,#60173)) ;
#24063=EDGE_LOOP('',(#60174,#60175,#60176,#60177)) ;
#24064=EDGE_LOOP('',(#60178,#60179,#60180,#60181)) ;
#24065=EDGE_LOOP('',(#60182,#60183,#60184,#60185)) ;
#24066=EDGE_LOOP('',(#60186,#60187,#60188,#60189)) ;
#24067=EDGE_LOOP('',(#60190,#60191,#60192,#60193)) ;
#24068=EDGE_LOOP('',(#60194,#60195,#60196,#60197)) ;
#24069=EDGE_LOOP('',(#60198,#60199,#60200,#60201)) ;
#24070=EDGE_LOOP('',(#60202,#60203,#60204,#60205)) ;
#24071=EDGE_LOOP('',(#60206,#60207,#60208,#60209)) ;
#24072=EDGE_LOOP('',(#60210,#60211,#60212,#60213)) ;
#24073=EDGE_LOOP('',(#60214,#60215,#60216,#60217)) ;
#24074=EDGE_LOOP('',(#60218,#60219,#60220,#60221,#60222,#60223)) ;
#24075=EDGE_LOOP('',(#60224,#60225,#60226,#60227,#60228,#60229)) ;
#24076=EDGE_LOOP('',(#60230,#60231,#60232,#60233,#60234)) ;
#24077=EDGE_LOOP('',(#60235,#60236,#60237,#60238)) ;
#24078=EDGE_LOOP('',(#60239,#60240,#60241,#60242)) ;
#24079=EDGE_LOOP('',(#60243,#60244,#60245,#60246)) ;
#24080=EDGE_LOOP('',(#60247,#60248,#60249,#60250)) ;
#24081=EDGE_LOOP('',(#60251,#60252,#60253,#60254)) ;
#24082=EDGE_LOOP('',(#60255,#60256,#60257,#60258)) ;
#24083=EDGE_LOOP('',(#60259,#60260,#60261,#60262)) ;
#24084=EDGE_LOOP('',(#60263,#60264,#60265,#60266)) ;
#24085=EDGE_LOOP('',(#60267,#60268,#60269,#60270)) ;
#24086=EDGE_LOOP('',(#60271,#60272,#60273,#60274)) ;
#24087=EDGE_LOOP('',(#60275,#60276,#60277,#60278)) ;
#24088=EDGE_LOOP('',(#60279,#60280,#60281,#60282)) ;
#24089=EDGE_LOOP('',(#60283,#60284,#60285,#60286)) ;
#24090=EDGE_LOOP('',(#60287,#60288,#60289,#60290,#60291,#60292)) ;
#24091=EDGE_LOOP('',(#60293,#60294,#60295,#60296,#60297,#60298)) ;
#24092=EDGE_LOOP('',(#60299,#60300,#60301,#60302,#60303)) ;
#24093=EDGE_LOOP('',(#60304,#60305,#60306,#60307)) ;
#24094=EDGE_LOOP('',(#60308,#60309,#60310,#60311)) ;
#24095=EDGE_LOOP('',(#60312,#60313,#60314,#60315)) ;
#24096=EDGE_LOOP('',(#60316,#60317,#60318,#60319)) ;
#24097=EDGE_LOOP('',(#60320,#60321,#60322,#60323)) ;
#24098=EDGE_LOOP('',(#60324,#60325,#60326,#60327)) ;
#24099=EDGE_LOOP('',(#60328,#60329,#60330,#60331)) ;
#24100=EDGE_LOOP('',(#60332,#60333,#60334,#60335)) ;
#24101=EDGE_LOOP('',(#60336,#60337,#60338,#60339)) ;
#24102=EDGE_LOOP('',(#60340,#60341,#60342,#60343)) ;
#24103=EDGE_LOOP('',(#60344,#60345,#60346,#60347)) ;
#24104=EDGE_LOOP('',(#60348,#60349,#60350,#60351)) ;
#24105=EDGE_LOOP('',(#60352,#60353,#60354,#60355)) ;
#24106=EDGE_LOOP('',(#60356,#60357,#60358,#60359,#60360,#60361)) ;
#24107=EDGE_LOOP('',(#60362,#60363,#60364,#60365,#60366,#60367)) ;
#24108=EDGE_LOOP('',(#60368,#60369,#60370,#60371,#60372)) ;
#24109=EDGE_LOOP('',(#60373,#60374,#60375,#60376)) ;
#24110=EDGE_LOOP('',(#60377,#60378,#60379,#60380)) ;
#24111=EDGE_LOOP('',(#60381,#60382,#60383,#60384)) ;
#24112=EDGE_LOOP('',(#60385,#60386,#60387,#60388)) ;
#24113=EDGE_LOOP('',(#60389,#60390,#60391,#60392)) ;
#24114=EDGE_LOOP('',(#60393,#60394,#60395,#60396)) ;
#24115=EDGE_LOOP('',(#60397,#60398,#60399,#60400)) ;
#24116=EDGE_LOOP('',(#60401,#60402,#60403,#60404)) ;
#24117=EDGE_LOOP('',(#60405,#60406,#60407,#60408)) ;
#24118=EDGE_LOOP('',(#60409,#60410,#60411,#60412)) ;
#24119=EDGE_LOOP('',(#60413,#60414,#60415,#60416)) ;
#24120=EDGE_LOOP('',(#60417,#60418,#60419,#60420)) ;
#24121=EDGE_LOOP('',(#60421,#60422,#60423,#60424)) ;
#24122=EDGE_LOOP('',(#60425,#60426,#60427,#60428)) ;
#24123=EDGE_LOOP('',(#60429,#60430,#60431,#60432)) ;
#24124=EDGE_LOOP('',(#60433,#60434,#60435,#60436)) ;
#24125=EDGE_LOOP('',(#60437,#60438,#60439,#60440)) ;
#24126=EDGE_LOOP('',(#60441,#60442,#60443,#60444)) ;
#24127=EDGE_LOOP('',(#60445,#60446,#60447,#60448)) ;
#24128=EDGE_LOOP('',(#60449,#60450,#60451,#60452)) ;
#24129=EDGE_LOOP('',(#60453,#60454,#60455,#60456)) ;
#24130=EDGE_LOOP('',(#60457,#60458,#60459,#60460)) ;
#24131=EDGE_LOOP('',(#60461,#60462,#60463,#60464)) ;
#24132=EDGE_LOOP('',(#60465,#60466,#60467,#60468)) ;
#24133=EDGE_LOOP('',(#60469,#60470,#60471,#60472)) ;
#24134=EDGE_LOOP('',(#60473,#60474,#60475,#60476)) ;
#24135=EDGE_LOOP('',(#60477,#60478,#60479,#60480)) ;
#24136=EDGE_LOOP('',(#60481,#60482,#60483,#60484)) ;
#24137=EDGE_LOOP('',(#60485,#60486,#60487,#60488)) ;
#24138=EDGE_LOOP('',(#60489,#60490,#60491,#60492)) ;
#24139=EDGE_LOOP('',(#60493,#60494,#60495,#60496)) ;
#24140=EDGE_LOOP('',(#60497,#60498,#60499,#60500)) ;
#24141=EDGE_LOOP('',(#60501,#60502,#60503,#60504)) ;
#24142=EDGE_LOOP('',(#60505,#60506,#60507,#60508)) ;
#24143=EDGE_LOOP('',(#60509,#60510,#60511,#60512)) ;
#24144=EDGE_LOOP('',(#60513,#60514,#60515,#60516)) ;
#24145=EDGE_LOOP('',(#60517,#60518,#60519,#60520)) ;
#24146=EDGE_LOOP('',(#60521,#60522,#60523,#60524)) ;
#24147=EDGE_LOOP('',(#60525,#60526,#60527,#60528)) ;
#24148=EDGE_LOOP('',(#60529,#60530,#60531,#60532)) ;
#24149=EDGE_LOOP('',(#60533,#60534,#60535,#60536)) ;
#24150=EDGE_LOOP('',(#60537,#60538,#60539,#60540)) ;
#24151=EDGE_LOOP('',(#60541,#60542,#60543,#60544)) ;
#24152=EDGE_LOOP('',(#60545,#60546,#60547,#60548)) ;
#24153=EDGE_LOOP('',(#60549,#60550,#60551,#60552)) ;
#24154=EDGE_LOOP('',(#60553,#60554,#60555,#60556)) ;
#24155=EDGE_LOOP('',(#60557,#60558,#60559)) ;
#24156=EDGE_LOOP('',(#60560,#60561,#60562,#60563)) ;
#24157=EDGE_LOOP('',(#60564,#60565,#60566,#60567)) ;
#24158=EDGE_LOOP('',(#60568,#60569,#60570,#60571)) ;
#24159=EDGE_LOOP('',(#60572,#60573,#60574)) ;
#24160=EDGE_LOOP('',(#60575,#60576,#60577)) ;
#24161=EDGE_LOOP('',(#60578,#60579,#60580,#60581)) ;
#24162=EDGE_LOOP('',(#60582,#60583,#60584,#60585)) ;
#24163=EDGE_LOOP('',(#60586,#60587,#60588,#60589)) ;
#24164=EDGE_LOOP('',(#60590,#60591,#60592)) ;
#24165=EDGE_LOOP('',(#60593,#60594,#60595,#60596)) ;
#24166=EDGE_LOOP('',(#60597,#60598,#60599,#60600)) ;
#24167=EDGE_LOOP('',(#60601,#60602,#60603,#60604)) ;
#24168=EDGE_LOOP('',(#60605,#60606,#60607,#60608)) ;
#24169=EDGE_LOOP('',(#60609,#60610,#60611)) ;
#24170=EDGE_LOOP('',(#60612,#60613,#60614,#60615)) ;
#24171=EDGE_LOOP('',(#60616,#60617,#60618,#60619)) ;
#24172=EDGE_LOOP('',(#60620,#60621,#60622,#60623)) ;
#24173=EDGE_LOOP('',(#60624,#60625,#60626)) ;
#24174=EDGE_LOOP('',(#60627,#60628,#60629)) ;
#24175=EDGE_LOOP('',(#60630,#60631,#60632,#60633)) ;
#24176=EDGE_LOOP('',(#60634,#60635,#60636,#60637)) ;
#24177=EDGE_LOOP('',(#60638,#60639,#60640,#60641)) ;
#24178=EDGE_LOOP('',(#60642,#60643,#60644)) ;
#24179=EDGE_LOOP('',(#60645,#60646,#60647,#60648)) ;
#24180=EDGE_LOOP('',(#60649,#60650,#60651,#60652)) ;
#24181=EDGE_LOOP('',(#60653,#60654,#60655,#60656)) ;
#24182=EDGE_LOOP('',(#60657,#60658,#60659,#60660)) ;
#24183=EDGE_LOOP('',(#60661,#60662,#60663)) ;
#24184=EDGE_LOOP('',(#60664,#60665,#60666,#60667)) ;
#24185=EDGE_LOOP('',(#60668,#60669,#60670,#60671)) ;
#24186=EDGE_LOOP('',(#60672,#60673,#60674,#60675)) ;
#24187=EDGE_LOOP('',(#60676,#60677,#60678)) ;
#24188=EDGE_LOOP('',(#60679,#60680,#60681)) ;
#24189=EDGE_LOOP('',(#60682,#60683,#60684,#60685)) ;
#24190=EDGE_LOOP('',(#60686,#60687,#60688,#60689)) ;
#24191=EDGE_LOOP('',(#60690,#60691,#60692,#60693)) ;
#24192=EDGE_LOOP('',(#60694,#60695,#60696)) ;
#24193=EDGE_LOOP('',(#60697,#60698,#60699,#60700)) ;
#24194=EDGE_LOOP('',(#60701,#60702,#60703,#60704)) ;
#24195=EDGE_LOOP('',(#60705,#60706,#60707,#60708)) ;
#24196=EDGE_LOOP('',(#60709,#60710,#60711,#60712)) ;
#24197=EDGE_LOOP('',(#60713,#60714,#60715)) ;
#24198=EDGE_LOOP('',(#60716,#60717,#60718,#60719)) ;
#24199=EDGE_LOOP('',(#60720,#60721,#60722,#60723)) ;
#24200=EDGE_LOOP('',(#60724,#60725,#60726,#60727)) ;
#24201=EDGE_LOOP('',(#60728,#60729,#60730)) ;
#24202=EDGE_LOOP('',(#60731,#60732,#60733)) ;
#24203=EDGE_LOOP('',(#60734,#60735,#60736,#60737)) ;
#24204=EDGE_LOOP('',(#60738,#60739,#60740,#60741)) ;
#24205=EDGE_LOOP('',(#60742,#60743,#60744,#60745)) ;
#24206=EDGE_LOOP('',(#60746,#60747,#60748)) ;
#24207=EDGE_LOOP('',(#60749,#60750,#60751,#60752)) ;
#24208=EDGE_LOOP('',(#60753,#60754,#60755,#60756)) ;
#24209=EDGE_LOOP('',(#60757,#60758,#60759,#60760)) ;
#24210=EDGE_LOOP('',(#60761,#60762,#60763,#60764)) ;
#24211=EDGE_LOOP('',(#60765,#60766,#60767)) ;
#24212=EDGE_LOOP('',(#60768,#60769,#60770,#60771)) ;
#24213=EDGE_LOOP('',(#60772,#60773,#60774,#60775)) ;
#24214=EDGE_LOOP('',(#60776,#60777,#60778,#60779)) ;
#24215=EDGE_LOOP('',(#60780,#60781,#60782)) ;
#24216=EDGE_LOOP('',(#60783,#60784,#60785)) ;
#24217=EDGE_LOOP('',(#60786,#60787,#60788,#60789)) ;
#24218=EDGE_LOOP('',(#60790,#60791,#60792,#60793)) ;
#24219=EDGE_LOOP('',(#60794,#60795,#60796,#60797)) ;
#24220=EDGE_LOOP('',(#60798,#60799,#60800)) ;
#24221=EDGE_LOOP('',(#60801,#60802,#60803,#60804)) ;
#24222=EDGE_LOOP('',(#60805,#60806,#60807,#60808)) ;
#24223=EDGE_LOOP('',(#60809,#60810,#60811,#60812)) ;
#24224=EDGE_LOOP('',(#60813,#60814,#60815,#60816)) ;
#24225=EDGE_LOOP('',(#60817,#60818,#60819)) ;
#24226=EDGE_LOOP('',(#60820,#60821,#60822,#60823)) ;
#24227=EDGE_LOOP('',(#60824,#60825,#60826,#60827)) ;
#24228=EDGE_LOOP('',(#60828,#60829,#60830,#60831)) ;
#24229=EDGE_LOOP('',(#60832,#60833,#60834)) ;
#24230=EDGE_LOOP('',(#60835,#60836,#60837)) ;
#24231=EDGE_LOOP('',(#60838,#60839,#60840,#60841)) ;
#24232=EDGE_LOOP('',(#60842,#60843,#60844,#60845)) ;
#24233=EDGE_LOOP('',(#60846,#60847,#60848,#60849)) ;
#24234=EDGE_LOOP('',(#60850,#60851,#60852)) ;
#24235=EDGE_LOOP('',(#60853,#60854,#60855,#60856)) ;
#24236=EDGE_LOOP('',(#60857,#60858,#60859,#60860)) ;
#24237=EDGE_LOOP('',(#60861,#60862,#60863,#60864)) ;
#24238=EDGE_LOOP('',(#60865,#60866,#60867,#60868)) ;
#24239=EDGE_LOOP('',(#60869,#60870,#60871)) ;
#24240=EDGE_LOOP('',(#60872,#60873,#60874,#60875)) ;
#24241=EDGE_LOOP('',(#60876,#60877,#60878,#60879)) ;
#24242=EDGE_LOOP('',(#60880,#60881,#60882,#60883)) ;
#24243=EDGE_LOOP('',(#60884,#60885,#60886)) ;
#24244=EDGE_LOOP('',(#60887,#60888,#60889)) ;
#24245=EDGE_LOOP('',(#60890,#60891,#60892,#60893)) ;
#24246=EDGE_LOOP('',(#60894,#60895,#60896,#60897)) ;
#24247=EDGE_LOOP('',(#60898,#60899,#60900,#60901)) ;
#24248=EDGE_LOOP('',(#60902,#60903,#60904)) ;
#24249=EDGE_LOOP('',(#60905,#60906,#60907,#60908)) ;
#24250=EDGE_LOOP('',(#60909,#60910,#60911,#60912)) ;
#24251=EDGE_LOOP('',(#60913,#60914,#60915,#60916)) ;
#24252=EDGE_LOOP('',(#60917,#60918,#60919,#60920)) ;
#24253=EDGE_LOOP('',(#60921,#60922,#60923)) ;
#24254=EDGE_LOOP('',(#60924,#60925,#60926,#60927)) ;
#24255=EDGE_LOOP('',(#60928,#60929,#60930,#60931)) ;
#24256=EDGE_LOOP('',(#60932,#60933,#60934,#60935)) ;
#24257=EDGE_LOOP('',(#60936,#60937,#60938)) ;
#24258=EDGE_LOOP('',(#60939,#60940,#60941)) ;
#24259=EDGE_LOOP('',(#60942,#60943,#60944,#60945)) ;
#24260=EDGE_LOOP('',(#60946,#60947,#60948,#60949)) ;
#24261=EDGE_LOOP('',(#60950,#60951,#60952,#60953)) ;
#24262=EDGE_LOOP('',(#60954,#60955,#60956)) ;
#24263=EDGE_LOOP('',(#60957,#60958,#60959,#60960)) ;
#24264=EDGE_LOOP('',(#60961,#60962,#60963,#60964)) ;
#24265=EDGE_LOOP('',(#60965,#60966,#60967,#60968)) ;
#24266=EDGE_LOOP('',(#60969,#60970,#60971,#60972)) ;
#24267=EDGE_LOOP('',(#60973,#60974,#60975)) ;
#24268=EDGE_LOOP('',(#60976,#60977,#60978,#60979)) ;
#24269=EDGE_LOOP('',(#60980,#60981,#60982,#60983)) ;
#24270=EDGE_LOOP('',(#60984,#60985,#60986,#60987)) ;
#24271=EDGE_LOOP('',(#60988,#60989,#60990)) ;
#24272=EDGE_LOOP('',(#60991,#60992,#60993)) ;
#24273=EDGE_LOOP('',(#60994,#60995,#60996,#60997)) ;
#24274=EDGE_LOOP('',(#60998,#60999,#61000,#61001)) ;
#24275=EDGE_LOOP('',(#61002,#61003,#61004,#61005)) ;
#24276=EDGE_LOOP('',(#61006,#61007,#61008)) ;
#24277=EDGE_LOOP('',(#61009,#61010,#61011,#61012)) ;
#24278=EDGE_LOOP('',(#61013,#61014,#61015,#61016)) ;
#24279=EDGE_LOOP('',(#61017,#61018,#61019,#61020)) ;
#24280=EDGE_LOOP('',(#61021,#61022,#61023,#61024)) ;
#24281=EDGE_LOOP('',(#61025,#61026,#61027)) ;
#24282=EDGE_LOOP('',(#61028,#61029,#61030,#61031)) ;
#24283=EDGE_LOOP('',(#61032,#61033,#61034,#61035)) ;
#24284=EDGE_LOOP('',(#61036,#61037,#61038,#61039)) ;
#24285=EDGE_LOOP('',(#61040,#61041,#61042)) ;
#24286=EDGE_LOOP('',(#61043,#61044,#61045)) ;
#24287=EDGE_LOOP('',(#61046,#61047,#61048,#61049)) ;
#24288=EDGE_LOOP('',(#61050,#61051,#61052,#61053)) ;
#24289=EDGE_LOOP('',(#61054,#61055,#61056,#61057)) ;
#24290=EDGE_LOOP('',(#61058,#61059,#61060)) ;
#24291=EDGE_LOOP('',(#61061,#61062,#61063,#61064)) ;
#24292=EDGE_LOOP('',(#61065,#61066,#61067,#61068)) ;
#24293=EDGE_LOOP('',(#61069,#61070,#61071,#61072)) ;
#24294=EDGE_LOOP('',(#61073,#61074,#61075,#61076)) ;
#24295=EDGE_LOOP('',(#61077,#61078,#61079)) ;
#24296=EDGE_LOOP('',(#61080,#61081,#61082,#61083)) ;
#24297=EDGE_LOOP('',(#61084,#61085,#61086,#61087)) ;
#24298=EDGE_LOOP('',(#61088,#61089,#61090,#61091)) ;
#24299=EDGE_LOOP('',(#61092,#61093,#61094)) ;
#24300=EDGE_LOOP('',(#61095,#61096,#61097)) ;
#24301=EDGE_LOOP('',(#61098,#61099,#61100,#61101)) ;
#24302=EDGE_LOOP('',(#61102,#61103,#61104,#61105)) ;
#24303=EDGE_LOOP('',(#61106,#61107,#61108,#61109)) ;
#24304=EDGE_LOOP('',(#61110,#61111,#61112)) ;
#24305=EDGE_LOOP('',(#61113,#61114,#61115,#61116)) ;
#24306=EDGE_LOOP('',(#61117,#61118,#61119,#61120)) ;
#24307=EDGE_LOOP('',(#61121,#61122,#61123,#61124)) ;
#24308=EDGE_LOOP('',(#61125,#61126,#61127,#61128)) ;
#24309=EDGE_LOOP('',(#61129,#61130,#61131)) ;
#24310=EDGE_LOOP('',(#61132,#61133,#61134,#61135)) ;
#24311=EDGE_LOOP('',(#61136,#61137,#61138,#61139)) ;
#24312=EDGE_LOOP('',(#61140,#61141,#61142,#61143)) ;
#24313=EDGE_LOOP('',(#61144,#61145,#61146)) ;
#24314=EDGE_LOOP('',(#61147,#61148,#61149)) ;
#24315=EDGE_LOOP('',(#61150,#61151,#61152,#61153)) ;
#24316=EDGE_LOOP('',(#61154,#61155,#61156,#61157)) ;
#24317=EDGE_LOOP('',(#61158,#61159,#61160,#61161)) ;
#24318=EDGE_LOOP('',(#61162,#61163,#61164)) ;
#24319=EDGE_LOOP('',(#61165,#61166,#61167,#61168)) ;
#24320=EDGE_LOOP('',(#61169,#61170,#61171,#61172)) ;
#24321=EDGE_LOOP('',(#61173,#61174,#61175,#61176)) ;
#24322=EDGE_LOOP('',(#61177,#61178,#61179,#61180)) ;
#24323=EDGE_LOOP('',(#61181,#61182,#61183)) ;
#24324=EDGE_LOOP('',(#61184,#61185,#61186,#61187)) ;
#24325=EDGE_LOOP('',(#61188,#61189,#61190,#61191)) ;
#24326=EDGE_LOOP('',(#61192,#61193,#61194,#61195)) ;
#24327=EDGE_LOOP('',(#61196,#61197,#61198)) ;
#24328=EDGE_LOOP('',(#61199,#61200,#61201)) ;
#24329=EDGE_LOOP('',(#61202,#61203,#61204,#61205)) ;
#24330=EDGE_LOOP('',(#61206,#61207,#61208,#61209)) ;
#24331=EDGE_LOOP('',(#61210,#61211,#61212,#61213)) ;
#24332=EDGE_LOOP('',(#61214,#61215,#61216)) ;
#24333=EDGE_LOOP('',(#61217,#61218,#61219,#61220)) ;
#24334=EDGE_LOOP('',(#61221,#61222,#61223,#61224)) ;
#24335=EDGE_LOOP('',(#61225,#61226,#61227,#61228)) ;
#24336=EDGE_LOOP('',(#61229,#61230,#61231,#61232)) ;
#24337=EDGE_LOOP('',(#61233,#61234,#61235)) ;
#24338=EDGE_LOOP('',(#61236,#61237,#61238,#61239)) ;
#24339=EDGE_LOOP('',(#61240,#61241,#61242,#61243)) ;
#24340=EDGE_LOOP('',(#61244,#61245,#61246,#61247)) ;
#24341=EDGE_LOOP('',(#61248,#61249,#61250)) ;
#24342=EDGE_LOOP('',(#61251,#61252,#61253)) ;
#24343=EDGE_LOOP('',(#61254,#61255,#61256,#61257)) ;
#24344=EDGE_LOOP('',(#61258,#61259,#61260,#61261)) ;
#24345=EDGE_LOOP('',(#61262,#61263,#61264,#61265)) ;
#24346=EDGE_LOOP('',(#61266,#61267,#61268)) ;
#24347=EDGE_LOOP('',(#61269,#61270,#61271,#61272)) ;
#24348=EDGE_LOOP('',(#61273,#61274,#61275,#61276)) ;
#24349=EDGE_LOOP('',(#61277,#61278,#61279,#61280)) ;
#24350=EDGE_LOOP('',(#61281,#61282,#61283,#61284)) ;
#24351=EDGE_LOOP('',(#61285,#61286,#61287)) ;
#24352=EDGE_LOOP('',(#61288,#61289,#61290,#61291)) ;
#24353=EDGE_LOOP('',(#61292,#61293,#61294,#61295)) ;
#24354=EDGE_LOOP('',(#61296,#61297,#61298,#61299)) ;
#24355=EDGE_LOOP('',(#61300,#61301,#61302)) ;
#24356=EDGE_LOOP('',(#61303,#61304,#61305)) ;
#24357=EDGE_LOOP('',(#61306,#61307,#61308,#61309)) ;
#24358=EDGE_LOOP('',(#61310,#61311,#61312,#61313)) ;
#24359=EDGE_LOOP('',(#61314,#61315,#61316,#61317)) ;
#24360=EDGE_LOOP('',(#61318,#61319,#61320)) ;
#24361=EDGE_LOOP('',(#61321,#61322,#61323,#61324)) ;
#24362=EDGE_LOOP('',(#61325,#61326,#61327,#61328)) ;
#24363=EDGE_LOOP('',(#61329,#61330,#61331,#61332)) ;
#24364=EDGE_LOOP('',(#61333,#61334,#61335,#61336)) ;
#24365=EDGE_LOOP('',(#61337,#61338,#61339)) ;
#24366=EDGE_LOOP('',(#61340,#61341,#61342,#61343)) ;
#24367=EDGE_LOOP('',(#61344,#61345,#61346,#61347)) ;
#24368=EDGE_LOOP('',(#61348,#61349,#61350,#61351)) ;
#24369=EDGE_LOOP('',(#61352,#61353,#61354)) ;
#24370=EDGE_LOOP('',(#61355,#61356,#61357)) ;
#24371=EDGE_LOOP('',(#61358,#61359,#61360,#61361)) ;
#24372=EDGE_LOOP('',(#61362,#61363,#61364,#61365)) ;
#24373=EDGE_LOOP('',(#61366,#61367,#61368,#61369)) ;
#24374=EDGE_LOOP('',(#61370,#61371,#61372)) ;
#24375=EDGE_LOOP('',(#61373,#61374,#61375,#61376)) ;
#24376=EDGE_LOOP('',(#61377,#61378,#61379,#61380)) ;
#24377=EDGE_LOOP('',(#61381,#61382,#61383,#61384)) ;
#24378=EDGE_LOOP('',(#61385,#61386,#61387,#61388)) ;
#24379=EDGE_LOOP('',(#61389,#61390,#61391)) ;
#24380=EDGE_LOOP('',(#61392,#61393,#61394,#61395)) ;
#24381=EDGE_LOOP('',(#61396,#61397,#61398,#61399)) ;
#24382=EDGE_LOOP('',(#61400,#61401,#61402,#61403)) ;
#24383=EDGE_LOOP('',(#61404,#61405,#61406)) ;
#24384=EDGE_LOOP('',(#61407,#61408,#61409)) ;
#24385=EDGE_LOOP('',(#61410,#61411,#61412,#61413)) ;
#24386=EDGE_LOOP('',(#61414,#61415,#61416,#61417)) ;
#24387=EDGE_LOOP('',(#61418,#61419,#61420,#61421)) ;
#24388=EDGE_LOOP('',(#61422,#61423,#61424)) ;
#24389=EDGE_LOOP('',(#61425,#61426,#61427,#61428)) ;
#24390=EDGE_LOOP('',(#61429,#61430,#61431,#61432)) ;
#24391=EDGE_LOOP('',(#61433,#61434,#61435,#61436)) ;
#24392=EDGE_LOOP('',(#61437,#61438,#61439,#61440)) ;
#24393=EDGE_LOOP('',(#61441,#61442,#61443)) ;
#24394=EDGE_LOOP('',(#61444,#61445,#61446,#61447)) ;
#24395=EDGE_LOOP('',(#61448,#61449,#61450,#61451)) ;
#24396=EDGE_LOOP('',(#61452,#61453,#61454,#61455)) ;
#24397=EDGE_LOOP('',(#61456,#61457,#61458)) ;
#24398=EDGE_LOOP('',(#61459,#61460,#61461)) ;
#24399=EDGE_LOOP('',(#61462,#61463,#61464,#61465)) ;
#24400=EDGE_LOOP('',(#61466,#61467,#61468,#61469)) ;
#24401=EDGE_LOOP('',(#61470,#61471,#61472,#61473)) ;
#24402=EDGE_LOOP('',(#61474,#61475,#61476)) ;
#24403=EDGE_LOOP('',(#61477,#61478,#61479,#61480)) ;
#24404=EDGE_LOOP('',(#61481,#61482,#61483,#61484)) ;
#24405=EDGE_LOOP('',(#61485,#61486,#61487,#61488)) ;
#24406=EDGE_LOOP('',(#61489,#61490,#61491,#61492)) ;
#24407=EDGE_LOOP('',(#61493,#61494,#61495,#61496)) ;
#24408=EDGE_LOOP('',(#61497,#61498,#61499,#61500)) ;
#24409=EDGE_LOOP('',(#61501,#61502,#61503,#61504)) ;
#24410=EDGE_LOOP('',(#61505,#61506,#61507,#61508)) ;
#24411=EDGE_LOOP('',(#61509,#61510,#61511,#61512,#61513)) ;
#24412=EDGE_LOOP('',(#61514,#61515,#61516,#61517)) ;
#24413=EDGE_LOOP('',(#61518,#61519,#61520,#61521)) ;
#24414=EDGE_LOOP('',(#61522,#61523,#61524,#61525)) ;
#24415=EDGE_LOOP('',(#61526,#61527,#61528,#61529)) ;
#24416=EDGE_LOOP('',(#61530,#61531,#61532,#61533)) ;
#24417=EDGE_LOOP('',(#61534,#61535,#61536,#61537)) ;
#24418=EDGE_LOOP('',(#61538,#61539,#61540,#61541)) ;
#24419=EDGE_LOOP('',(#61542,#61543,#61544,#61545)) ;
#24420=EDGE_LOOP('',(#61546,#61547,#61548,#61549)) ;
#24421=EDGE_LOOP('',(#61550,#61551,#61552,#61553)) ;
#24422=EDGE_LOOP('',(#61554,#61555,#61556,#61557)) ;
#24423=EDGE_LOOP('',(#61558,#61559,#61560,#61561)) ;
#24424=EDGE_LOOP('',(#61562,#61563,#61564,#61565)) ;
#24425=EDGE_LOOP('',(#61566,#61567,#61568,#61569)) ;
#24426=EDGE_LOOP('',(#61570,#61571,#61572,#61573)) ;
#24427=EDGE_LOOP('',(#61574,#61575,#61576,#61577)) ;
#24428=EDGE_LOOP('',(#61578,#61579,#61580,#61581)) ;
#24429=EDGE_LOOP('',(#61582,#61583,#61584,#61585)) ;
#24430=EDGE_LOOP('',(#61586,#61587,#61588,#61589)) ;
#24431=EDGE_LOOP('',(#61590,#61591,#61592,#61593)) ;
#24432=EDGE_LOOP('',(#61594,#61595,#61596,#61597)) ;
#24433=EDGE_LOOP('',(#61598,#61599,#61600,#61601)) ;
#24434=EDGE_LOOP('',(#61602,#61603,#61604,#61605)) ;
#24435=EDGE_LOOP('',(#61606,#61607,#61608,#61609,#61610)) ;
#24436=EDGE_LOOP('',(#61611,#61612,#61613,#61614)) ;
#24437=EDGE_LOOP('',(#61615,#61616,#61617,#61618)) ;
#24438=EDGE_LOOP('',(#61619,#61620,#61621,#61622)) ;
#24439=EDGE_LOOP('',(#61623,#61624,#61625,#61626)) ;
#24440=EDGE_LOOP('',(#61627,#61628,#61629,#61630)) ;
#24441=EDGE_LOOP('',(#61631,#61632,#61633,#61634)) ;
#24442=EDGE_LOOP('',(#61635,#61636,#61637,#61638)) ;
#24443=EDGE_LOOP('',(#61639,#61640,#61641,#61642)) ;
#24444=EDGE_LOOP('',(#61643,#61644,#61645,#61646)) ;
#24445=EDGE_LOOP('',(#61647,#61648,#61649,#61650)) ;
#24446=EDGE_LOOP('',(#61651,#61652,#61653,#61654)) ;
#24447=EDGE_LOOP('',(#61655,#61656,#61657,#61658)) ;
#24448=EDGE_LOOP('',(#61659,#61660,#61661,#61662)) ;
#24449=EDGE_LOOP('',(#61663,#61664,#61665,#61666)) ;
#24450=EDGE_LOOP('',(#61667,#61668,#61669,#61670)) ;
#24451=EDGE_LOOP('',(#61671,#61672,#61673,#61674)) ;
#24452=EDGE_LOOP('',(#61675,#61676,#61677,#61678)) ;
#24453=EDGE_LOOP('',(#61679,#61680,#61681,#61682)) ;
#24454=EDGE_LOOP('',(#61683,#61684,#61685,#61686)) ;
#24455=EDGE_LOOP('',(#61687,#61688,#61689,#61690)) ;
#24456=EDGE_LOOP('',(#61691,#61692,#61693,#61694)) ;
#24457=EDGE_LOOP('',(#61695,#61696,#61697,#61698)) ;
#24458=EDGE_LOOP('',(#61699,#61700,#61701,#61702)) ;
#24459=EDGE_LOOP('',(#61703,#61704,#61705,#61706,#61707)) ;
#24460=EDGE_LOOP('',(#61708,#61709,#61710,#61711)) ;
#24461=EDGE_LOOP('',(#61712,#61713,#61714,#61715)) ;
#24462=EDGE_LOOP('',(#61716,#61717,#61718,#61719)) ;
#24463=EDGE_LOOP('',(#61720,#61721,#61722,#61723)) ;
#24464=EDGE_LOOP('',(#61724,#61725,#61726,#61727)) ;
#24465=EDGE_LOOP('',(#61728,#61729,#61730,#61731)) ;
#24466=EDGE_LOOP('',(#61732,#61733,#61734,#61735)) ;
#24467=EDGE_LOOP('',(#61736,#61737,#61738,#61739)) ;
#24468=EDGE_LOOP('',(#61740,#61741,#61742,#61743)) ;
#24469=EDGE_LOOP('',(#61744,#61745,#61746,#61747)) ;
#24470=EDGE_LOOP('',(#61748,#61749,#61750,#61751)) ;
#24471=EDGE_LOOP('',(#61752,#61753,#61754,#61755)) ;
#24472=EDGE_LOOP('',(#61756,#61757,#61758,#61759)) ;
#24473=EDGE_LOOP('',(#61760,#61761,#61762,#61763)) ;
#24474=EDGE_LOOP('',(#61764,#61765,#61766,#61767)) ;
#24475=EDGE_LOOP('',(#61768,#61769,#61770,#61771)) ;
#24476=EDGE_LOOP('',(#61772,#61773,#61774,#61775)) ;
#24477=EDGE_LOOP('',(#61776,#61777,#61778,#61779)) ;
#24478=EDGE_LOOP('',(#61780,#61781,#61782,#61783)) ;
#24479=EDGE_LOOP('',(#61784,#61785,#61786,#61787)) ;
#24480=EDGE_LOOP('',(#61788,#61789,#61790,#61791)) ;
#24481=EDGE_LOOP('',(#61792,#61793,#61794,#61795)) ;
#24482=EDGE_LOOP('',(#61796,#61797,#61798,#61799)) ;
#24483=EDGE_LOOP('',(#61800,#61801,#61802,#61803,#61804)) ;
#24484=EDGE_LOOP('',(#61805,#61806,#61807,#61808)) ;
#24485=EDGE_LOOP('',(#61809,#61810,#61811,#61812)) ;
#24486=EDGE_LOOP('',(#61813,#61814,#61815,#61816)) ;
#24487=EDGE_LOOP('',(#61817,#61818,#61819,#61820)) ;
#24488=EDGE_LOOP('',(#61821,#61822,#61823,#61824)) ;
#24489=EDGE_LOOP('',(#61825,#61826,#61827,#61828)) ;
#24490=EDGE_LOOP('',(#61829,#61830,#61831,#61832)) ;
#24491=EDGE_LOOP('',(#61833,#61834,#61835,#61836)) ;
#24492=EDGE_LOOP('',(#61837,#61838,#61839,#61840)) ;
#24493=EDGE_LOOP('',(#61841,#61842,#61843,#61844)) ;
#24494=EDGE_LOOP('',(#61845,#61846,#61847,#61848)) ;
#24495=EDGE_LOOP('',(#61849,#61850,#61851,#61852)) ;
#24496=EDGE_LOOP('',(#61853,#61854,#61855,#61856)) ;
#24497=EDGE_LOOP('',(#61857,#61858,#61859,#61860)) ;
#24498=EDGE_LOOP('',(#61861,#61862,#61863,#61864)) ;
#24499=EDGE_LOOP('',(#61865,#61866,#61867,#61868)) ;
#24500=EDGE_LOOP('',(#61869,#61870,#61871,#61872)) ;
#24501=EDGE_LOOP('',(#61873,#61874,#61875,#61876)) ;
#24502=EDGE_LOOP('',(#61877,#61878,#61879,#61880)) ;
#24503=EDGE_LOOP('',(#61881,#61882,#61883,#61884)) ;
#24504=EDGE_LOOP('',(#61885,#61886,#61887,#61888)) ;
#24505=EDGE_LOOP('',(#61889,#61890,#61891,#61892)) ;
#24506=EDGE_LOOP('',(#61893,#61894,#61895,#61896)) ;
#24507=EDGE_LOOP('',(#61897,#61898,#61899,#61900,#61901)) ;
#24508=EDGE_LOOP('',(#61902,#61903,#61904,#61905)) ;
#24509=EDGE_LOOP('',(#61906,#61907,#61908,#61909)) ;
#24510=EDGE_LOOP('',(#61910,#61911,#61912,#61913)) ;
#24511=EDGE_LOOP('',(#61914,#61915,#61916,#61917)) ;
#24512=EDGE_LOOP('',(#61918,#61919,#61920,#61921)) ;
#24513=EDGE_LOOP('',(#61922,#61923,#61924,#61925)) ;
#24514=EDGE_LOOP('',(#61926,#61927,#61928,#61929)) ;
#24515=EDGE_LOOP('',(#61930,#61931,#61932,#61933)) ;
#24516=EDGE_LOOP('',(#61934,#61935,#61936,#61937)) ;
#24517=EDGE_LOOP('',(#61938,#61939,#61940,#61941)) ;
#24518=EDGE_LOOP('',(#61942,#61943,#61944,#61945)) ;
#24519=EDGE_LOOP('',(#61946,#61947,#61948,#61949)) ;
#24520=EDGE_LOOP('',(#61950,#61951,#61952,#61953)) ;
#24521=EDGE_LOOP('',(#61954,#61955,#61956,#61957)) ;
#24522=EDGE_LOOP('',(#61958,#61959,#61960,#61961)) ;
#24523=EDGE_LOOP('',(#61962,#61963,#61964,#61965)) ;
#24524=EDGE_LOOP('',(#61966,#61967,#61968,#61969)) ;
#24525=EDGE_LOOP('',(#61970,#61971,#61972,#61973)) ;
#24526=EDGE_LOOP('',(#61974,#61975,#61976,#61977)) ;
#24527=EDGE_LOOP('',(#61978,#61979,#61980,#61981)) ;
#24528=EDGE_LOOP('',(#61982,#61983,#61984,#61985)) ;
#24529=EDGE_LOOP('',(#61986,#61987,#61988,#61989)) ;
#24530=EDGE_LOOP('',(#61990,#61991,#61992,#61993)) ;
#24531=EDGE_LOOP('',(#61994,#61995,#61996,#61997,#61998)) ;
#24532=EDGE_LOOP('',(#61999,#62000,#62001,#62002)) ;
#24533=EDGE_LOOP('',(#62003,#62004,#62005,#62006)) ;
#24534=EDGE_LOOP('',(#62007,#62008,#62009,#62010)) ;
#24535=EDGE_LOOP('',(#62011,#62012,#62013,#62014)) ;
#24536=EDGE_LOOP('',(#62015,#62016,#62017,#62018)) ;
#24537=EDGE_LOOP('',(#62019,#62020,#62021,#62022)) ;
#24538=EDGE_LOOP('',(#62023,#62024,#62025,#62026)) ;
#24539=EDGE_LOOP('',(#62027,#62028,#62029,#62030)) ;
#24540=EDGE_LOOP('',(#62031,#62032,#62033,#62034)) ;
#24541=EDGE_LOOP('',(#62035,#62036,#62037,#62038)) ;
#24542=EDGE_LOOP('',(#62039,#62040,#62041,#62042)) ;
#24543=EDGE_LOOP('',(#62043,#62044,#62045,#62046)) ;
#24544=EDGE_LOOP('',(#62047,#62048,#62049,#62050)) ;
#24545=EDGE_LOOP('',(#62051,#62052,#62053,#62054)) ;
#24546=EDGE_LOOP('',(#62055,#62056,#62057,#62058)) ;
#24547=EDGE_LOOP('',(#62059,#62060,#62061,#62062)) ;
#24548=EDGE_LOOP('',(#62063,#62064,#62065,#62066)) ;
#24549=EDGE_LOOP('',(#62067,#62068,#62069,#62070)) ;
#24550=EDGE_LOOP('',(#62071,#62072,#62073,#62074)) ;
#24551=EDGE_LOOP('',(#62075,#62076,#62077,#62078)) ;
#24552=EDGE_LOOP('',(#62079,#62080,#62081,#62082)) ;
#24553=EDGE_LOOP('',(#62083,#62084,#62085,#62086)) ;
#24554=EDGE_LOOP('',(#62087,#62088,#62089,#62090)) ;
#24555=EDGE_LOOP('',(#62091,#62092,#62093,#62094,#62095)) ;
#24556=EDGE_LOOP('',(#62096,#62097,#62098,#62099)) ;
#24557=EDGE_LOOP('',(#62100,#62101,#62102,#62103)) ;
#24558=EDGE_LOOP('',(#62104,#62105,#62106,#62107)) ;
#24559=EDGE_LOOP('',(#62108,#62109,#62110,#62111)) ;
#24560=EDGE_LOOP('',(#62112,#62113,#62114,#62115)) ;
#24561=EDGE_LOOP('',(#62116,#62117,#62118,#62119)) ;
#24562=EDGE_LOOP('',(#62120,#62121,#62122,#62123)) ;
#24563=EDGE_LOOP('',(#62124,#62125,#62126,#62127)) ;
#24564=EDGE_LOOP('',(#62128,#62129,#62130,#62131)) ;
#24565=EDGE_LOOP('',(#62132,#62133,#62134,#62135)) ;
#24566=EDGE_LOOP('',(#62136,#62137,#62138,#62139)) ;
#24567=EDGE_LOOP('',(#62140,#62141,#62142,#62143)) ;
#24568=EDGE_LOOP('',(#62144,#62145,#62146,#62147)) ;
#24569=EDGE_LOOP('',(#62148,#62149,#62150,#62151)) ;
#24570=EDGE_LOOP('',(#62152,#62153,#62154,#62155)) ;
#24571=EDGE_LOOP('',(#62156,#62157,#62158,#62159)) ;
#24572=EDGE_LOOP('',(#62160,#62161,#62162,#62163)) ;
#24573=EDGE_LOOP('',(#62164,#62165,#62166,#62167)) ;
#24574=EDGE_LOOP('',(#62168,#62169,#62170,#62171)) ;
#24575=EDGE_LOOP('',(#62172,#62173,#62174,#62175)) ;
#24576=EDGE_LOOP('',(#62176,#62177,#62178,#62179)) ;
#24577=EDGE_LOOP('',(#62180,#62181,#62182,#62183)) ;
#24578=EDGE_LOOP('',(#62184,#62185,#62186,#62187)) ;
#24579=EDGE_LOOP('',(#62188,#62189,#62190,#62191,#62192)) ;
#24580=EDGE_LOOP('',(#62193,#62194,#62195,#62196)) ;
#24581=EDGE_LOOP('',(#62197,#62198,#62199,#62200)) ;
#24582=EDGE_LOOP('',(#62201,#62202,#62203,#62204)) ;
#24583=EDGE_LOOP('',(#62205,#62206,#62207,#62208)) ;
#24584=EDGE_LOOP('',(#62209,#62210,#62211,#62212)) ;
#24585=EDGE_LOOP('',(#62213,#62214,#62215,#62216)) ;
#24586=EDGE_LOOP('',(#62217,#62218,#62219,#62220)) ;
#24587=EDGE_LOOP('',(#62221,#62222,#62223,#62224)) ;
#24588=EDGE_LOOP('',(#62225,#62226,#62227,#62228)) ;
#24589=EDGE_LOOP('',(#62229,#62230,#62231,#62232)) ;
#24590=EDGE_LOOP('',(#62233,#62234,#62235,#62236)) ;
#24591=EDGE_LOOP('',(#62237,#62238,#62239,#62240)) ;
#24592=EDGE_LOOP('',(#62241,#62242,#62243,#62244)) ;
#24593=EDGE_LOOP('',(#62245,#62246,#62247,#62248)) ;
#24594=EDGE_LOOP('',(#62249,#62250,#62251,#62252)) ;
#24595=EDGE_LOOP('',(#62253,#62254,#62255,#62256)) ;
#24596=EDGE_LOOP('',(#62257,#62258,#62259,#62260)) ;
#24597=EDGE_LOOP('',(#62261,#62262,#62263,#62264)) ;
#24598=EDGE_LOOP('',(#62265,#62266,#62267,#62268)) ;
#24599=EDGE_LOOP('',(#62269,#62270,#62271,#62272)) ;
#24600=EDGE_LOOP('',(#62273,#62274,#62275,#62276)) ;
#24601=EDGE_LOOP('',(#62277,#62278,#62279,#62280)) ;
#24602=EDGE_LOOP('',(#62281,#62282,#62283,#62284)) ;
#24603=EDGE_LOOP('',(#62285,#62286,#62287,#62288,#62289)) ;
#24604=EDGE_LOOP('',(#62290,#62291,#62292,#62293)) ;
#24605=EDGE_LOOP('',(#62294,#62295,#62296,#62297)) ;
#24606=EDGE_LOOP('',(#62298,#62299,#62300,#62301)) ;
#24607=EDGE_LOOP('',(#62302,#62303,#62304,#62305)) ;
#24608=EDGE_LOOP('',(#62306,#62307,#62308,#62309)) ;
#24609=EDGE_LOOP('',(#62310,#62311,#62312,#62313)) ;
#24610=EDGE_LOOP('',(#62314,#62315,#62316,#62317)) ;
#24611=EDGE_LOOP('',(#62318,#62319,#62320,#62321)) ;
#24612=EDGE_LOOP('',(#62322,#62323,#62324,#62325)) ;
#24613=EDGE_LOOP('',(#62326,#62327,#62328,#62329)) ;
#24614=EDGE_LOOP('',(#62330,#62331,#62332,#62333)) ;
#24615=EDGE_LOOP('',(#62334,#62335,#62336,#62337)) ;
#24616=EDGE_LOOP('',(#62338,#62339,#62340,#62341)) ;
#24617=EDGE_LOOP('',(#62342,#62343,#62344,#62345)) ;
#24618=EDGE_LOOP('',(#62346,#62347,#62348,#62349)) ;
#24619=EDGE_LOOP('',(#62350,#62351,#62352,#62353)) ;
#24620=EDGE_LOOP('',(#62354,#62355,#62356,#62357)) ;
#26857=CIRCLE('',#71868,0.899999999999998) ;
#26858=CIRCLE('',#71869,0.1) ;
#26859=CIRCLE('',#71870,1.) ;
#26860=CIRCLE('',#71871,1.) ;
#26861=CIRCLE('',#71873,1.1) ;
#26862=CIRCLE('',#71874,0.1) ;
#26863=CIRCLE('',#71875,1.) ;
#26864=CIRCLE('',#71877,0.100000000000003) ;
#26865=CIRCLE('',#71878,0.0999999999999999) ;
#26866=CIRCLE('',#71879,0.1) ;
#26867=CIRCLE('',#71882,0.1) ;
#26868=CIRCLE('',#71883,0.100000000000003) ;
#26869=CIRCLE('',#71885,0.899999999999998) ;
#26870=CIRCLE('',#71886,0.1) ;
#26871=CIRCLE('',#71887,1.) ;
#26872=CIRCLE('',#71888,1.) ;
#26873=CIRCLE('',#71890,1.1) ;
#26874=CIRCLE('',#71891,0.1) ;
#26875=CIRCLE('',#71892,1.) ;
#26876=CIRCLE('',#71894,0.0999999999999994) ;
#26877=CIRCLE('',#71895,0.1) ;
#26878=CIRCLE('',#71896,0.1) ;
#26879=CIRCLE('',#71899,0.1) ;
#26880=CIRCLE('',#71900,0.0999999999999994) ;
#26881=CIRCLE('',#71902,0.899999999999998) ;
#26882=CIRCLE('',#71903,0.1) ;
#26883=CIRCLE('',#71904,1.) ;
#26884=CIRCLE('',#71905,1.) ;
#26885=CIRCLE('',#71907,1.1) ;
#26886=CIRCLE('',#71908,0.1) ;
#26887=CIRCLE('',#71909,1.) ;
#26888=CIRCLE('',#71911,0.0999999999999994) ;
#26889=CIRCLE('',#71912,0.1) ;
#26890=CIRCLE('',#71913,0.1) ;
#26891=CIRCLE('',#71916,0.1) ;
#26892=CIRCLE('',#71917,0.0999999999999994) ;
#26893=CIRCLE('',#71919,0.899999999999998) ;
#26894=CIRCLE('',#71920,0.1) ;
#26895=CIRCLE('',#71921,1.) ;
#26896=CIRCLE('',#71922,1.) ;
#26897=CIRCLE('',#71924,1.1) ;
#26898=CIRCLE('',#71925,0.1) ;
#26899=CIRCLE('',#71926,1.) ;
#26900=CIRCLE('',#71928,0.0999999999999994) ;
#26901=CIRCLE('',#71929,0.1) ;
#26902=CIRCLE('',#71930,0.1) ;
#26903=CIRCLE('',#71933,0.1) ;
#26904=CIRCLE('',#71934,0.0999999999999994) ;
#26905=CIRCLE('',#71936,0.900000000000001) ;
#26906=CIRCLE('',#71937,0.1) ;
#26907=CIRCLE('',#71938,1.) ;
#26908=CIRCLE('',#71939,1.) ;
#26909=CIRCLE('',#71941,1.1) ;
#26910=CIRCLE('',#71942,0.1) ;
#26911=CIRCLE('',#71943,1.) ;
#26912=CIRCLE('',#71945,0.0999999999999994) ;
#26913=CIRCLE('',#71946,0.1) ;
#26914=CIRCLE('',#71947,0.1) ;
#26915=CIRCLE('',#71950,0.1) ;
#26916=CIRCLE('',#71951,0.0999999999999994) ;
#26917=CIRCLE('',#71953,0.900000000000001) ;
#26918=CIRCLE('',#71954,0.1) ;
#26919=CIRCLE('',#71955,1.) ;
#26920=CIRCLE('',#71956,1.) ;
#26921=CIRCLE('',#71958,1.1) ;
#26922=CIRCLE('',#71959,0.1) ;
#26923=CIRCLE('',#71960,0.999999999999999) ;
#26924=CIRCLE('',#71962,0.100000000000001) ;
#26925=CIRCLE('',#71963,0.1) ;
#26926=CIRCLE('',#71964,0.1) ;
#26927=CIRCLE('',#71967,0.1) ;
#26928=CIRCLE('',#71968,0.0999999999999994) ;
#26929=CIRCLE('',#71970,0.9) ;
#26930=CIRCLE('',#71971,0.1) ;
#26931=CIRCLE('',#71972,0.999999999999999) ;
#26932=CIRCLE('',#71973,0.999999999999999) ;
#26933=CIRCLE('',#71975,1.1) ;
#26934=CIRCLE('',#71976,0.1) ;
#26935=CIRCLE('',#71977,0.999999999999999) ;
#26936=CIRCLE('',#71979,0.100000000000001) ;
#26937=CIRCLE('',#71980,0.1) ;
#26938=CIRCLE('',#71981,0.1) ;
#26939=CIRCLE('',#71984,0.1) ;
#26940=CIRCLE('',#71985,0.0999999999999994) ;
#26941=CIRCLE('',#71987,0.9) ;
#26942=CIRCLE('',#71988,0.1) ;
#26943=CIRCLE('',#71989,0.999999999999999) ;
#26944=CIRCLE('',#71990,0.999999999999999) ;
#26945=CIRCLE('',#71992,1.1) ;
#26946=CIRCLE('',#71993,0.1) ;
#26947=CIRCLE('',#71994,1.) ;
#26948=CIRCLE('',#71996,0.1) ;
#26949=CIRCLE('',#71997,0.1) ;
#26950=CIRCLE('',#71998,0.1) ;
#26951=CIRCLE('',#72001,0.1) ;
#26952=CIRCLE('',#72002,0.0999999999999994) ;
#26953=CIRCLE('',#72004,0.9) ;
#26954=CIRCLE('',#72005,0.1) ;
#26955=CIRCLE('',#72006,1.) ;
#26956=CIRCLE('',#72007,1.) ;
#26957=CIRCLE('',#72009,0.200000000000001) ;
#26958=CIRCLE('',#72010,0.0999999999999994) ;
#26959=CIRCLE('',#72011,0.1) ;
#26960=CIRCLE('',#72012,0.1) ;
#26961=CIRCLE('',#72014,0.200000000000001) ;
#26962=CIRCLE('',#72015,0.0999999999999994) ;
#26963=CIRCLE('',#72016,0.100000000000001) ;
#26964=CIRCLE('',#72017,0.1) ;
#26965=CIRCLE('',#72019,0.200000000000001) ;
#26966=CIRCLE('',#72020,0.0999999999999994) ;
#26967=CIRCLE('',#72021,0.100000000000001) ;
#26968=CIRCLE('',#72022,0.1) ;
#26969=CIRCLE('',#72024,0.199999999999999) ;
#26970=CIRCLE('',#72025,0.0999999999999994) ;
#26971=CIRCLE('',#72026,0.0999999999999994) ;
#26972=CIRCLE('',#72027,0.0999999999999995) ;
#26973=CIRCLE('',#72029,0.199999999999999) ;
#26974=CIRCLE('',#72030,0.0999999999999994) ;
#26975=CIRCLE('',#72031,0.0999999999999994) ;
#26976=CIRCLE('',#72032,0.0999999999999995) ;
#26977=CIRCLE('',#72034,0.199999999999999) ;
#26978=CIRCLE('',#72035,0.0999999999999994) ;
#26979=CIRCLE('',#72036,0.0999999999999994) ;
#26980=CIRCLE('',#72037,0.0999999999999995) ;
#26981=CIRCLE('',#72039,0.199999999999999) ;
#26982=CIRCLE('',#72040,0.0999999999999994) ;
#26983=CIRCLE('',#72041,0.0999999999999994) ;
#26984=CIRCLE('',#72042,0.0999999999999995) ;
#26985=CIRCLE('',#72044,0.199999999999999) ;
#26986=CIRCLE('',#72045,0.0999999999999994) ;
#26987=CIRCLE('',#72046,0.100000000000003) ;
#26988=CIRCLE('',#72047,0.0999999999999995) ;
#26989=CIRCLE('',#72049,0.199999999999999) ;
#26990=CIRCLE('',#72050,0.0999999999999994) ;
#26991=CIRCLE('',#72051,0.100000000000003) ;
#26992=CIRCLE('',#72052,0.0999999999999995) ;
#26993=CIRCLE('',#72054,1.1) ;
#26994=CIRCLE('',#72055,0.1) ;
#26995=CIRCLE('',#72056,1.) ;
#26996=CIRCLE('',#72058,0.100000000000001) ;
#26997=CIRCLE('',#72059,0.0999999999999998) ;
#26998=CIRCLE('',#72060,0.1) ;
#26999=CIRCLE('',#72063,0.1) ;
#27000=CIRCLE('',#72064,0.1) ;
#27001=CIRCLE('',#72075,0.1) ;
#27002=CIRCLE('',#72077,0.100000000000001) ;
#27003=CIRCLE('',#72079,0.100000000000001) ;
#27004=CIRCLE('',#72081,0.0999999999999994) ;
#27005=CIRCLE('',#72083,0.0999999999999994) ;
#27006=CIRCLE('',#72085,0.0999999999999994) ;
#27007=CIRCLE('',#72087,0.0999999999999994) ;
#27008=CIRCLE('',#72089,0.100000000000003) ;
#27009=CIRCLE('',#72091,0.100000000000003) ;
#27010=CIRCLE('',#72093,0.9) ;
#27011=CIRCLE('',#72094,0.1) ;
#27012=CIRCLE('',#72095,1.) ;
#27013=CIRCLE('',#72096,1.) ;
#27014=CIRCLE('',#72098,0.200000000000001) ;
#27015=CIRCLE('',#72099,0.0999999999999994) ;
#27016=CIRCLE('',#72100,0.1) ;
#27017=CIRCLE('',#72101,0.1) ;
#27018=CIRCLE('',#72103,1.1) ;
#27019=CIRCLE('',#72104,0.1) ;
#27020=CIRCLE('',#72105,1.) ;
#27021=CIRCLE('',#72107,0.1) ;
#27022=CIRCLE('',#72108,0.1) ;
#27023=CIRCLE('',#72109,0.1) ;
#27024=CIRCLE('',#72112,0.1) ;
#27025=CIRCLE('',#72113,0.1) ;
#27026=CIRCLE('',#72116,0.1) ;
#27027=CIRCLE('',#72118,0.1) ;
#27028=CIRCLE('',#72119,0.1) ;
#27029=CIRCLE('',#72120,0.2) ;
#27030=CIRCLE('',#72121,0.2) ;
#27031=CIRCLE('',#72123,0.1) ;
#27032=CIRCLE('',#72124,0.1) ;
#27033=CIRCLE('',#72125,0.2) ;
#27034=CIRCLE('',#72126,0.2) ;
#27035=CIRCLE('',#72128,0.1) ;
#27036=CIRCLE('',#72129,0.1) ;
#27037=CIRCLE('',#72130,0.2) ;
#27038=CIRCLE('',#72131,0.2) ;
#27039=CIRCLE('',#72133,0.1) ;
#27040=CIRCLE('',#72134,0.1) ;
#27041=CIRCLE('',#72135,0.2) ;
#27042=CIRCLE('',#72136,0.2) ;
#27043=CIRCLE('',#72138,0.1) ;
#27044=CIRCLE('',#72139,0.1) ;
#27045=CIRCLE('',#72140,0.2) ;
#27046=CIRCLE('',#72141,0.2) ;
#27047=CIRCLE('',#72143,0.1) ;
#27048=CIRCLE('',#72144,0.1) ;
#27049=CIRCLE('',#72145,0.2) ;
#27050=CIRCLE('',#72146,0.2) ;
#27051=CIRCLE('',#72148,0.1) ;
#27052=CIRCLE('',#72149,0.1) ;
#27053=CIRCLE('',#72150,0.2) ;
#27054=CIRCLE('',#72151,0.2) ;
#27055=CIRCLE('',#72153,0.1) ;
#27056=CIRCLE('',#72154,0.1) ;
#27057=CIRCLE('',#72155,0.2) ;
#27058=CIRCLE('',#72156,0.2) ;
#27059=CIRCLE('',#72158,0.1) ;
#27060=CIRCLE('',#72159,0.1) ;
#27061=CIRCLE('',#72160,0.2) ;
#27062=CIRCLE('',#72161,0.2) ;
#27063=CIRCLE('',#72163,0.2) ;
#27064=CIRCLE('',#72165,0.2) ;
#27065=CIRCLE('',#72167,0.2) ;
#27066=CIRCLE('',#72169,0.2) ;
#27067=CIRCLE('',#72171,0.2) ;
#27068=CIRCLE('',#72173,0.2) ;
#27069=CIRCLE('',#72175,0.2) ;
#27070=CIRCLE('',#72177,0.2) ;
#27071=CIRCLE('',#72179,0.2) ;
#27072=CIRCLE('',#72181,0.2) ;
#27073=CIRCLE('',#72183,0.2) ;
#27074=CIRCLE('',#72185,0.2) ;
#27075=CIRCLE('',#72187,0.2) ;
#27076=CIRCLE('',#72189,0.2) ;
#27077=CIRCLE('',#72191,0.2) ;
#27078=CIRCLE('',#72193,0.2) ;
#27079=CIRCLE('',#72195,0.2) ;
#27080=CIRCLE('',#72197,0.2) ;
#27081=CIRCLE('',#72199,0.1) ;
#27082=CIRCLE('',#72200,0.1) ;
#27083=CIRCLE('',#72202,0.1) ;
#27084=CIRCLE('',#72203,0.1) ;
#27085=CIRCLE('',#72205,0.1) ;
#27086=CIRCLE('',#72206,0.1) ;
#27087=CIRCLE('',#72208,0.1) ;
#27088=CIRCLE('',#72209,0.1) ;
#27089=CIRCLE('',#72211,0.1) ;
#27090=CIRCLE('',#72212,0.1) ;
#27091=CIRCLE('',#72214,0.1) ;
#27092=CIRCLE('',#72215,0.1) ;
#27093=CIRCLE('',#72217,0.1) ;
#27094=CIRCLE('',#72218,0.1) ;
#27095=CIRCLE('',#72220,0.1) ;
#27096=CIRCLE('',#72221,0.1) ;
#27097=CIRCLE('',#72223,0.1) ;
#27098=CIRCLE('',#72224,0.1) ;
#27099=CIRCLE('',#72226,0.1) ;
#27100=CIRCLE('',#72227,0.1) ;
#27101=CIRCLE('',#72228,0.2) ;
#27102=CIRCLE('',#72229,0.2) ;
#27103=CIRCLE('',#72231,0.2) ;
#27104=CIRCLE('',#72233,0.2) ;
#27105=CIRCLE('',#72235,0.1) ;
#27106=CIRCLE('',#72236,0.1) ;
#27107=CIRCLE('',#72238,0.0999999999999994) ;
#27108=CIRCLE('',#72239,0.0999999999999994) ;
#27109=CIRCLE('',#72241,0.199999999999999) ;
#27110=CIRCLE('',#72242,0.2) ;
#27111=CIRCLE('',#72243,0.2) ;
#27112=CIRCLE('',#72244,0.2) ;
#27113=CIRCLE('',#72245,0.2) ;
#27114=CIRCLE('',#72246,0.2) ;
#27115=CIRCLE('',#72247,0.200000000000001) ;
#27116=CIRCLE('',#72248,0.200000000000001) ;
#27117=CIRCLE('',#72249,0.200000000000001) ;
#27118=CIRCLE('',#72250,0.200000000000001) ;
#27119=CIRCLE('',#72251,0.199999999999999) ;
#27120=CIRCLE('',#72252,0.199999999999999) ;
#27121=CIRCLE('',#72253,0.199999999999999) ;
#27122=CIRCLE('',#72254,0.199999999999999) ;
#27123=CIRCLE('',#72255,0.199999999999999) ;
#27124=CIRCLE('',#72256,0.199999999999999) ;
#27125=CIRCLE('',#72257,0.199999999999999) ;
#27126=CIRCLE('',#72258,0.199999999999999) ;
#27127=CIRCLE('',#72259,0.199999999999999) ;
#27128=CIRCLE('',#72260,0.199999999999999) ;
#27129=CIRCLE('',#72262,0.1) ;
#27130=CIRCLE('',#72263,0.1) ;
#27131=CIRCLE('',#72265,0.2) ;
#27132=CIRCLE('',#72266,0.2) ;
#27133=CIRCLE('',#72267,0.2) ;
#27134=CIRCLE('',#72268,0.2) ;
#27135=CIRCLE('',#72269,0.2) ;
#27136=CIRCLE('',#72270,0.2) ;
#27137=CIRCLE('',#72271,0.2) ;
#27138=CIRCLE('',#72272,0.2) ;
#27139=CIRCLE('',#72273,0.2) ;
#27140=CIRCLE('',#72274,0.2) ;
#27141=CIRCLE('',#72275,0.2) ;
#27142=CIRCLE('',#72276,0.2) ;
#27143=CIRCLE('',#72277,0.2) ;
#27144=CIRCLE('',#72278,0.2) ;
#27145=CIRCLE('',#72279,0.2) ;
#27146=CIRCLE('',#72280,0.2) ;
#27147=CIRCLE('',#72281,0.2) ;
#27148=CIRCLE('',#72282,0.2) ;
#27149=CIRCLE('',#72283,0.2) ;
#27150=CIRCLE('',#72284,0.2) ;
#27151=CIRCLE('',#72286,0.1) ;
#27152=CIRCLE('',#72287,0.1) ;
#27153=CIRCLE('',#72290,0.1) ;
#27154=CIRCLE('',#72291,0.1) ;
#27155=CIRCLE('',#72294,0.1) ;
#27156=CIRCLE('',#72295,0.1) ;
#27157=CIRCLE('',#72298,0.100000000000001) ;
#27158=CIRCLE('',#72299,0.100000000000001) ;
#27159=CIRCLE('',#72302,0.1) ;
#27160=CIRCLE('',#72303,0.1) ;
#27161=CIRCLE('',#72306,0.0999999999999994) ;
#27162=CIRCLE('',#72307,0.0999999999999994) ;
#27163=CIRCLE('',#72309,0.199999999999999) ;
#27164=CIRCLE('',#72310,0.199999999999999) ;
#27165=CIRCLE('',#72311,0.199999999999999) ;
#27166=CIRCLE('',#72312,0.199999999999999) ;
#27167=CIRCLE('',#72313,0.199999999999999) ;
#27168=CIRCLE('',#72314,0.199999999999999) ;
#27169=CIRCLE('',#72315,0.199999999999999) ;
#27170=CIRCLE('',#72316,1.55625) ;
#27171=CIRCLE('',#72317,0.199999999999999) ;
#27172=CIRCLE('',#72318,0.199999999999999) ;
#27173=CIRCLE('',#72319,0.199999999999999) ;
#27174=CIRCLE('',#72320,0.199999999999999) ;
#27175=CIRCLE('',#72321,0.199999999999999) ;
#27176=CIRCLE('',#72322,0.199999999999999) ;
#27177=CIRCLE('',#72323,0.199999999999999) ;
#27178=CIRCLE('',#72324,0.199999999999999) ;
#27179=CIRCLE('',#72325,0.199999999999999) ;
#27180=CIRCLE('',#72326,1.55625) ;
#27181=CIRCLE('',#72327,0.199999999999999) ;
#27182=CIRCLE('',#72328,0.199999999999999) ;
#27183=CIRCLE('',#72329,0.199999999999999) ;
#27184=CIRCLE('',#72330,0.199999999999999) ;
#27185=CIRCLE('',#72331,0.199999999999999) ;
#27186=CIRCLE('',#72332,0.199999999999999) ;
#27187=CIRCLE('',#72333,0.199999999999999) ;
#27188=CIRCLE('',#72334,0.199999999999999) ;
#27189=CIRCLE('',#72335,0.199999999999999) ;
#27190=CIRCLE('',#72336,1.55625) ;
#27191=CIRCLE('',#72337,0.199999999999999) ;
#27192=CIRCLE('',#72338,0.199999999999999) ;
#27193=CIRCLE('',#72339,0.199999999999999) ;
#27194=CIRCLE('',#72340,0.199999999999999) ;
#27195=CIRCLE('',#72341,0.199999999999999) ;
#27196=CIRCLE('',#72342,0.199999999999999) ;
#27197=CIRCLE('',#72343,0.199999999999999) ;
#27198=CIRCLE('',#72344,0.199999999999999) ;
#27199=CIRCLE('',#72345,0.199999999999999) ;
#27200=CIRCLE('',#72346,1.55625) ;
#27201=CIRCLE('',#72347,0.199999999999999) ;
#27202=CIRCLE('',#72348,0.199999999999999) ;
#27203=CIRCLE('',#72349,0.199999999999999) ;
#27204=CIRCLE('',#72350,0.199999999999999) ;
#27205=CIRCLE('',#72351,0.199999999999999) ;
#27206=CIRCLE('',#72352,0.199999999999999) ;
#27207=CIRCLE('',#72353,0.199999999999999) ;
#27208=CIRCLE('',#72354,0.199999999999999) ;
#27209=CIRCLE('',#72355,0.199999999999999) ;
#27210=CIRCLE('',#72356,1.55625) ;
#27211=CIRCLE('',#72357,0.199999999999999) ;
#27212=CIRCLE('',#72358,0.199999999999999) ;
#27213=CIRCLE('',#72359,0.200000000000001) ;
#27214=CIRCLE('',#72360,0.199999999999999) ;
#27215=CIRCLE('',#72361,0.200000000000001) ;
#27216=CIRCLE('',#72362,0.199999999999999) ;
#27217=CIRCLE('',#72363,0.199999999999999) ;
#27218=CIRCLE('',#72364,0.199999999999999) ;
#27219=CIRCLE('',#72365,0.199999999999999) ;
#27220=CIRCLE('',#72366,1.55625) ;
#27221=CIRCLE('',#72367,0.200000000000001) ;
#27222=CIRCLE('',#72368,0.200000000000001) ;
#27223=CIRCLE('',#72369,0.200000000000001) ;
#27224=CIRCLE('',#72370,0.199999999999999) ;
#27225=CIRCLE('',#72371,0.200000000000001) ;
#27226=CIRCLE('',#72372,0.200000000000001) ;
#27227=CIRCLE('',#72373,0.200000000000001) ;
#27228=CIRCLE('',#72374,0.200000000000001) ;
#27229=CIRCLE('',#72375,0.200000000000001) ;
#27230=CIRCLE('',#72376,1.55625) ;
#27231=CIRCLE('',#72377,0.200000000000001) ;
#27232=CIRCLE('',#72378,0.200000000000001) ;
#27233=CIRCLE('',#72379,0.2) ;
#27234=CIRCLE('',#72380,0.2) ;
#27235=CIRCLE('',#72381,0.200000000000001) ;
#27236=CIRCLE('',#72382,0.200000000000001) ;
#27237=CIRCLE('',#72383,0.200000000000001) ;
#27238=CIRCLE('',#72384,0.200000000000001) ;
#27239=CIRCLE('',#72385,0.200000000000001) ;
#27240=CIRCLE('',#72386,1.55625) ;
#27241=CIRCLE('',#72387,0.2) ;
#27242=CIRCLE('',#72388,0.2) ;
#27243=CIRCLE('',#72389,0.2) ;
#27244=CIRCLE('',#72390,0.199999999999999) ;
#27245=CIRCLE('',#72391,0.200000000000001) ;
#27246=CIRCLE('',#72392,0.200000000000001) ;
#27247=CIRCLE('',#72393,0.2) ;
#27248=CIRCLE('',#72394,0.2) ;
#27249=CIRCLE('',#72395,0.2) ;
#27250=CIRCLE('',#72396,1.55625) ;
#27251=CIRCLE('',#72397,0.2) ;
#27252=CIRCLE('',#72398,0.2) ;
#27253=CIRCLE('',#72399,0.2) ;
#27254=CIRCLE('',#72400,0.199999999999999) ;
#27255=CIRCLE('',#72401,0.200000000000001) ;
#27256=CIRCLE('',#72402,0.2) ;
#27257=CIRCLE('',#72403,0.2) ;
#27258=CIRCLE('',#72404,0.2) ;
#27259=CIRCLE('',#72405,0.2) ;
#27260=CIRCLE('',#72406,1.55625) ;
#27261=CIRCLE('',#72407,0.2) ;
#27262=CIRCLE('',#72408,0.2) ;
#27263=CIRCLE('',#72410,0.200000000000001) ;
#27264=CIRCLE('',#72411,0.200000000000001) ;
#27265=CIRCLE('',#72413,0.200000000000001) ;
#27266=CIRCLE('',#72414,0.200000000000001) ;
#27267=CIRCLE('',#72416,0.2) ;
#27268=CIRCLE('',#72417,0.2) ;
#27269=CIRCLE('',#72424,0.1) ;
#27270=CIRCLE('',#72425,0.1) ;
#27271=CIRCLE('',#72428,0.1) ;
#27272=CIRCLE('',#72429,0.1) ;
#27273=CIRCLE('',#72432,0.0999999999999994) ;
#27274=CIRCLE('',#72433,0.0999999999999994) ;
#27275=CIRCLE('',#72436,0.1) ;
#27276=CIRCLE('',#72440,0.1) ;
#27277=CIRCLE('',#72441,0.1) ;
#27278=CIRCLE('',#72444,0.1) ;
#27279=CIRCLE('',#72445,0.1) ;
#27280=CIRCLE('',#72448,0.1) ;
#27281=CIRCLE('',#72449,0.1) ;
#27282=CIRCLE('',#72452,0.1) ;
#27283=CIRCLE('',#72453,0.1) ;
#27284=CIRCLE('',#72456,0.1) ;
#27285=CIRCLE('',#72457,0.1) ;
#27286=CIRCLE('',#72460,0.1) ;
#27287=CIRCLE('',#72461,0.1) ;
#27288=CIRCLE('',#72463,1.65625) ;
#27289=CIRCLE('',#72464,1.65625) ;
#27290=CIRCLE('',#72466,0.1) ;
#27291=CIRCLE('',#72467,0.1) ;
#27292=CIRCLE('',#72470,0.1) ;
#27293=CIRCLE('',#72471,0.1) ;
#27294=CIRCLE('',#72474,0.1) ;
#27295=CIRCLE('',#72475,0.1) ;
#27296=CIRCLE('',#72478,0.2) ;
#27297=CIRCLE('',#72479,0.2) ;
#27298=CIRCLE('',#72480,1.75625) ;
#27299=CIRCLE('',#72481,0.2) ;
#27300=CIRCLE('',#72482,0.2) ;
#27301=CIRCLE('',#72484,0.1) ;
#27302=CIRCLE('',#72485,0.1) ;
#27303=CIRCLE('',#72486,0.1) ;
#27304=CIRCLE('',#72487,0.1) ;
#27305=CIRCLE('',#72489,0.1) ;
#27306=CIRCLE('',#72490,0.1) ;
#27307=CIRCLE('',#72492,0.1) ;
#27308=CIRCLE('',#72493,0.1) ;
#27309=CIRCLE('',#72495,0.1) ;
#27310=CIRCLE('',#72496,0.1) ;
#27311=CIRCLE('',#72498,0.1) ;
#27312=CIRCLE('',#72499,0.0999999999999998) ;
#27313=CIRCLE('',#72501,0.1) ;
#27314=CIRCLE('',#72503,0.1) ;
#27315=CIRCLE('',#72505,0.1) ;
#27316=CIRCLE('',#72507,0.1) ;
#27317=CIRCLE('',#72509,0.0999999999999998) ;
#27318=CIRCLE('',#72511,0.1) ;
#27319=CIRCLE('',#72513,0.1) ;
#27320=CIRCLE('',#72514,0.1) ;
#27321=CIRCLE('',#72517,0.1) ;
#27322=CIRCLE('',#72519,0.1) ;
#27323=CIRCLE('',#72520,0.1) ;
#27324=CIRCLE('',#72522,0.1) ;
#27325=CIRCLE('',#72524,0.1) ;
#27326=CIRCLE('',#72526,0.1) ;
#27327=CIRCLE('',#72528,0.1) ;
#27328=CIRCLE('',#72530,0.1) ;
#27329=CIRCLE('',#72532,0.1) ;
#27330=CIRCLE('',#72533,0.1) ;
#27331=CIRCLE('',#72535,0.1) ;
#27332=CIRCLE('',#72537,0.1) ;
#27333=CIRCLE('',#72539,0.0999999999999998) ;
#27334=CIRCLE('',#72540,0.1) ;
#27335=CIRCLE('',#72542,0.1) ;
#27336=CIRCLE('',#72544,0.1) ;
#27337=CIRCLE('',#72545,0.1) ;
#27338=CIRCLE('',#72547,0.1) ;
#27339=CIRCLE('',#72549,0.1) ;
#27340=CIRCLE('',#72551,0.1) ;
#27341=CIRCLE('',#72553,0.1) ;
#27342=CIRCLE('',#72555,0.1) ;
#27343=CIRCLE('',#72557,0.1) ;
#27344=CIRCLE('',#72559,0.1) ;
#27345=CIRCLE('',#72561,0.1) ;
#27346=CIRCLE('',#72562,0.1) ;
#27347=CIRCLE('',#72564,0.1) ;
#27348=CIRCLE('',#72566,0.1) ;
#27349=CIRCLE('',#72568,0.1) ;
#27350=CIRCLE('',#72570,0.1) ;
#27351=CIRCLE('',#72571,0.1) ;
#27352=CIRCLE('',#72573,0.1) ;
#27353=CIRCLE('',#72575,0.1) ;
#27354=CIRCLE('',#72577,0.1) ;
#27355=CIRCLE('',#72579,0.1) ;
#27356=CIRCLE('',#72582,0.1) ;
#27357=CIRCLE('',#72584,0.1) ;
#27358=CIRCLE('',#72586,0.1) ;
#27359=CIRCLE('',#72589,0.100000000000003) ;
#27360=CIRCLE('',#72590,0.100000000000003) ;
#27361=CIRCLE('',#72592,0.100000000000003) ;
#27362=CIRCLE('',#72594,0.100000000000003) ;
#27363=CIRCLE('',#72596,0.1) ;
#27364=CIRCLE('',#72598,0.100000000000003) ;
#27365=CIRCLE('',#72600,0.100000000000003) ;
#27366=CIRCLE('',#72602,0.1) ;
#27367=CIRCLE('',#72604,0.1) ;
#27368=CIRCLE('',#72606,0.1) ;
#27369=CIRCLE('',#72608,0.100000000000003) ;
#27370=CIRCLE('',#72610,0.100000000000003) ;
#27371=CIRCLE('',#72612,0.0999999999999998) ;
#27372=CIRCLE('',#72614,0.100000000000003) ;
#27373=CIRCLE('',#72616,0.100000000000003) ;
#27374=CIRCLE('',#72618,0.0999999999999994) ;
#27375=CIRCLE('',#72621,0.0999999999999998) ;
#27376=CIRCLE('',#72622,0.0999999999999998) ;
#27377=CIRCLE('',#72624,0.0999999999999998) ;
#27378=CIRCLE('',#72626,0.0999999999999998) ;
#27379=CIRCLE('',#72628,0.0999999999999998) ;
#27380=CIRCLE('',#72630,0.0999999999999998) ;
#27381=CIRCLE('',#72632,0.1) ;
#27382=CIRCLE('',#72634,0.1) ;
#27383=CIRCLE('',#72636,0.1) ;
#27384=CIRCLE('',#72638,0.1) ;
#27385=CIRCLE('',#72640,0.1) ;
#27386=CIRCLE('',#72642,0.0999999999999998) ;
#27387=CIRCLE('',#72644,0.0999999999999998) ;
#27388=CIRCLE('',#72646,0.0999999999999998) ;
#27389=CIRCLE('',#72648,0.0999999999999998) ;
#27390=CIRCLE('',#72650,0.0999999999999998) ;
#27391=CIRCLE('',#72653,0.1) ;
#27392=CIRCLE('',#72654,0.1) ;
#27393=CIRCLE('',#72656,0.1) ;
#27394=CIRCLE('',#72658,0.1) ;
#27395=CIRCLE('',#72660,0.1) ;
#27396=CIRCLE('',#72662,0.1) ;
#27397=CIRCLE('',#72664,0.1) ;
#27398=CIRCLE('',#72666,0.0999999999999998) ;
#27399=CIRCLE('',#72668,0.0999999999999998) ;
#27400=CIRCLE('',#72670,0.1) ;
#27401=CIRCLE('',#72672,0.1) ;
#27402=CIRCLE('',#72674,0.1) ;
#27403=CIRCLE('',#72676,0.1) ;
#27404=CIRCLE('',#72678,0.1) ;
#27405=CIRCLE('',#72680,0.1) ;
#27406=CIRCLE('',#72682,0.1) ;
#27407=CIRCLE('',#72685,0.1) ;
#27408=CIRCLE('',#72687,0.1) ;
#27409=CIRCLE('',#72689,0.1) ;
#27410=CIRCLE('',#72691,0.1) ;
#27411=CIRCLE('',#72693,0.0999999999999998) ;
#27412=CIRCLE('',#72695,0.1) ;
#27413=CIRCLE('',#72697,0.1) ;
#27414=CIRCLE('',#72699,0.1) ;
#27415=CIRCLE('',#72701,0.1) ;
#27416=CIRCLE('',#72703,0.1) ;
#27417=CIRCLE('',#72706,0.1) ;
#27418=CIRCLE('',#72707,0.1) ;
#27419=CIRCLE('',#72709,0.0999999999999998) ;
#27420=CIRCLE('',#72711,0.1) ;
#27421=CIRCLE('',#72713,0.1) ;
#27422=CIRCLE('',#72715,0.0999999999999998) ;
#27423=CIRCLE('',#72717,0.1) ;
#27424=CIRCLE('',#72719,0.1) ;
#27425=CIRCLE('',#72722,0.1) ;
#27426=CIRCLE('',#72724,0.0999999999999994) ;
#27427=CIRCLE('',#72726,0.0999999999999994) ;
#27428=CIRCLE('',#72728,0.0999999999999994) ;
#27429=CIRCLE('',#72730,0.1) ;
#27430=CIRCLE('',#72732,0.1) ;
#27431=CIRCLE('',#72734,0.1) ;
#27432=CIRCLE('',#72736,0.1) ;
#27433=CIRCLE('',#72738,0.0999999999999998) ;
#27434=CIRCLE('',#72740,0.0999999999999994) ;
#27435=CIRCLE('',#72742,0.0999999999999998) ;
#27436=CIRCLE('',#72744,0.0999999999999998) ;
#27437=CIRCLE('',#72746,0.1) ;
#27438=CIRCLE('',#72748,0.1) ;
#27439=CIRCLE('',#72750,0.1) ;
#27440=CIRCLE('',#72752,0.1) ;
#27441=CIRCLE('',#72754,0.0999999999999994) ;
#27442=CIRCLE('',#72756,0.1) ;
#27443=CIRCLE('',#72764,0.3) ;
#27444=CIRCLE('',#72765,0.9) ;
#27445=CIRCLE('',#72767,0.9) ;
#27446=CIRCLE('',#72768,0.3) ;
#27447=CIRCLE('',#72770,1.) ;
#27448=CIRCLE('',#72771,1.) ;
#27449=CIRCLE('',#72773,0.2) ;
#27450=CIRCLE('',#72774,0.2) ;
#27451=CIRCLE('',#72787,0.1) ;
#27452=CIRCLE('',#72788,0.1) ;
#27453=CIRCLE('',#72790,0.1) ;
#27454=CIRCLE('',#72791,0.1) ;
#27455=CIRCLE('',#72793,0.1) ;
#27456=CIRCLE('',#72794,0.1) ;
#27457=CIRCLE('',#72796,0.1) ;
#27458=CIRCLE('',#72797,0.1) ;
#27459=CIRCLE('',#72799,0.1) ;
#27460=CIRCLE('',#72801,0.1) ;
#27461=CIRCLE('',#72803,0.1) ;
#27462=CIRCLE('',#72805,0.1) ;
#27463=CIRCLE('',#72806,0.1) ;
#27464=CIRCLE('',#72808,0.1) ;
#27465=CIRCLE('',#72810,0.1) ;
#27466=CIRCLE('',#72812,0.1) ;
#27467=CIRCLE('',#72814,0.1) ;
#27468=CIRCLE('',#72816,0.1) ;
#27469=CIRCLE('',#72817,0.1) ;
#27470=CIRCLE('',#72819,0.1) ;
#27471=CIRCLE('',#72821,0.1) ;
#27472=CIRCLE('',#72822,0.1) ;
#27473=CIRCLE('',#72824,0.1) ;
#27474=CIRCLE('',#72825,0.1) ;
#27475=CIRCLE('',#72827,0.1) ;
#27476=CIRCLE('',#72828,0.1) ;
#27477=CIRCLE('',#72830,0.1) ;
#27478=CIRCLE('',#72831,0.1) ;
#27479=CIRCLE('',#72833,0.1) ;
#27480=CIRCLE('',#72835,0.1) ;
#27481=CIRCLE('',#72837,0.1) ;
#27482=CIRCLE('',#72839,0.1) ;
#27483=CIRCLE('',#72840,0.1) ;
#27484=CIRCLE('',#72842,0.1) ;
#27485=CIRCLE('',#72844,0.1) ;
#27486=CIRCLE('',#72846,0.1) ;
#27487=CIRCLE('',#72848,0.1) ;
#27488=CIRCLE('',#72850,0.1) ;
#27489=CIRCLE('',#72851,0.1) ;
#27490=CIRCLE('',#72853,0.1) ;
#27491=CIRCLE('',#72855,0.1) ;
#27492=CIRCLE('',#72857,0.1) ;
#27493=CIRCLE('',#72859,0.1) ;
#27494=CIRCLE('',#72861,0.1) ;
#27495=CIRCLE('',#72863,0.1) ;
#27496=CIRCLE('',#72865,0.1) ;
#27497=CIRCLE('',#72868,0.1) ;
#27498=CIRCLE('',#72870,0.1) ;
#27499=CIRCLE('',#72872,0.1) ;
#27500=CIRCLE('',#72874,0.1) ;
#27501=CIRCLE('',#72876,0.1) ;
#27502=CIRCLE('',#72878,0.1) ;
#27503=CIRCLE('',#72881,0.1) ;
#27504=CIRCLE('',#72883,0.1) ;
#27505=CIRCLE('',#72885,0.1) ;
#27506=CIRCLE('',#72887,0.1) ;
#27507=CIRCLE('',#72890,0.1) ;
#27508=CIRCLE('',#72892,0.1) ;
#27509=CIRCLE('',#72894,0.1) ;
#27510=CIRCLE('',#72896,0.1) ;
#27511=CIRCLE('',#72899,0.2) ;
#27512=CIRCLE('',#72900,0.2) ;
#27513=CIRCLE('',#72902,0.2) ;
#27514=CIRCLE('',#72903,0.2) ;
#27515=CIRCLE('',#72905,0.2) ;
#27516=CIRCLE('',#72906,0.2) ;
#27517=CIRCLE('',#72908,0.2) ;
#27518=CIRCLE('',#72909,0.2) ;
#27519=CIRCLE('',#72911,0.2) ;
#27520=CIRCLE('',#72912,0.2) ;
#27521=CIRCLE('',#72914,0.2) ;
#27522=CIRCLE('',#72915,0.2) ;
#27523=CIRCLE('',#72917,0.2) ;
#27524=CIRCLE('',#72918,0.2) ;
#27525=CIRCLE('',#72920,0.2) ;
#27526=CIRCLE('',#72921,0.2) ;
#27527=CIRCLE('',#72923,0.2) ;
#27528=CIRCLE('',#72924,0.2) ;
#27529=CIRCLE('',#72971,0.100000000000003) ;
#27530=CIRCLE('',#72972,0.100000000000003) ;
#27531=CIRCLE('',#72975,0.100000000000003) ;
#27532=CIRCLE('',#72976,0.100000000000003) ;
#27533=CIRCLE('',#72979,0.0999999999999959) ;
#27534=CIRCLE('',#72980,0.0999999999999959) ;
#27535=CIRCLE('',#72983,0.100000000000003) ;
#27536=CIRCLE('',#72987,0.100000000000003) ;
#27537=CIRCLE('',#72988,0.100000000000003) ;
#27538=CIRCLE('',#72991,0.100000000000003) ;
#27539=CIRCLE('',#72992,0.100000000000003) ;
#27540=CIRCLE('',#72995,0.100000000000003) ;
#27541=CIRCLE('',#72996,0.100000000000003) ;
#27542=CIRCLE('',#72999,0.100000000000003) ;
#27543=CIRCLE('',#73000,0.100000000000003) ;
#27544=CIRCLE('',#73003,0.100000000000003) ;
#27545=CIRCLE('',#73004,0.100000000000003) ;
#27546=CIRCLE('',#73007,0.100000000000003) ;
#27547=CIRCLE('',#73008,0.100000000000003) ;
#27548=CIRCLE('',#73010,1.65625) ;
#27549=CIRCLE('',#73011,1.65625) ;
#27550=CIRCLE('',#73013,0.100000000000003) ;
#27551=CIRCLE('',#73014,0.100000000000003) ;
#27552=CIRCLE('',#73017,0.100000000000003) ;
#27553=CIRCLE('',#73018,0.100000000000003) ;
#27554=CIRCLE('',#73021,0.100000000000003) ;
#27555=CIRCLE('',#73022,0.100000000000003) ;
#27556=CIRCLE('',#73025,0.199999999999999) ;
#27557=CIRCLE('',#73026,0.199999999999999) ;
#27558=CIRCLE('',#73027,1.75625) ;
#27559=CIRCLE('',#73028,0.199999999999999) ;
#27560=CIRCLE('',#73029,0.199999999999999) ;
#27561=CIRCLE('',#73031,0.0999999999999994) ;
#27562=CIRCLE('',#73032,0.0999999999999994) ;
#27563=CIRCLE('',#73035,0.0999999999999994) ;
#27564=CIRCLE('',#73036,0.0999999999999994) ;
#27565=CIRCLE('',#73039,0.0999999999999994) ;
#27566=CIRCLE('',#73040,0.0999999999999994) ;
#27567=CIRCLE('',#73043,0.0999999999999994) ;
#27568=CIRCLE('',#73047,0.100000000000003) ;
#27569=CIRCLE('',#73048,0.100000000000003) ;
#27570=CIRCLE('',#73051,0.0999999999999994) ;
#27571=CIRCLE('',#73052,0.0999999999999994) ;
#27572=CIRCLE('',#73055,0.0999999999999994) ;
#27573=CIRCLE('',#73056,0.0999999999999994) ;
#27574=CIRCLE('',#73059,0.100000000000003) ;
#27575=CIRCLE('',#73060,0.100000000000003) ;
#27576=CIRCLE('',#73063,0.100000000000003) ;
#27577=CIRCLE('',#73064,0.100000000000003) ;
#27578=CIRCLE('',#73067,0.100000000000003) ;
#27579=CIRCLE('',#73068,0.100000000000003) ;
#27580=CIRCLE('',#73070,1.65625) ;
#27581=CIRCLE('',#73071,1.65625) ;
#27582=CIRCLE('',#73073,0.0999999999999994) ;
#27583=CIRCLE('',#73074,0.0999999999999994) ;
#27584=CIRCLE('',#73077,0.0999999999999994) ;
#27585=CIRCLE('',#73078,0.0999999999999994) ;
#27586=CIRCLE('',#73081,0.0999999999999994) ;
#27587=CIRCLE('',#73082,0.0999999999999994) ;
#27588=CIRCLE('',#73085,0.199999999999999) ;
#27589=CIRCLE('',#73086,0.199999999999999) ;
#27590=CIRCLE('',#73087,1.75625) ;
#27591=CIRCLE('',#73088,0.199999999999999) ;
#27592=CIRCLE('',#73089,0.199999999999999) ;
#27593=CIRCLE('',#73091,0.0999999999999994) ;
#27594=CIRCLE('',#73092,0.0999999999999994) ;
#27595=CIRCLE('',#73095,0.0999999999999994) ;
#27596=CIRCLE('',#73096,0.0999999999999994) ;
#27597=CIRCLE('',#73099,0.0999999999999994) ;
#27598=CIRCLE('',#73100,0.0999999999999994) ;
#27599=CIRCLE('',#73103,0.0999999999999994) ;
#27600=CIRCLE('',#73107,0.0999999999999994) ;
#27601=CIRCLE('',#73108,0.0999999999999994) ;
#27602=CIRCLE('',#73111,0.0999999999999994) ;
#27603=CIRCLE('',#73112,0.0999999999999994) ;
#27604=CIRCLE('',#73115,0.0999999999999994) ;
#27605=CIRCLE('',#73116,0.0999999999999994) ;
#27606=CIRCLE('',#73119,0.0999999999999994) ;
#27607=CIRCLE('',#73120,0.0999999999999994) ;
#27608=CIRCLE('',#73123,0.0999999999999994) ;
#27609=CIRCLE('',#73124,0.0999999999999994) ;
#27610=CIRCLE('',#73127,0.0999999999999994) ;
#27611=CIRCLE('',#73128,0.0999999999999994) ;
#27612=CIRCLE('',#73130,1.65625) ;
#27613=CIRCLE('',#73131,1.65625) ;
#27614=CIRCLE('',#73133,0.0999999999999994) ;
#27615=CIRCLE('',#73134,0.0999999999999994) ;
#27616=CIRCLE('',#73137,0.0999999999999994) ;
#27617=CIRCLE('',#73138,0.0999999999999994) ;
#27618=CIRCLE('',#73141,0.0999999999999994) ;
#27619=CIRCLE('',#73142,0.0999999999999994) ;
#27620=CIRCLE('',#73145,0.199999999999999) ;
#27621=CIRCLE('',#73146,0.199999999999999) ;
#27622=CIRCLE('',#73147,1.75625) ;
#27623=CIRCLE('',#73148,0.199999999999999) ;
#27624=CIRCLE('',#73149,0.199999999999999) ;
#27625=CIRCLE('',#73151,0.0999999999999994) ;
#27626=CIRCLE('',#73152,0.0999999999999994) ;
#27627=CIRCLE('',#73155,0.0999999999999994) ;
#27628=CIRCLE('',#73156,0.0999999999999994) ;
#27629=CIRCLE('',#73159,0.0999999999999994) ;
#27630=CIRCLE('',#73160,0.0999999999999994) ;
#27631=CIRCLE('',#73163,0.0999999999999994) ;
#27632=CIRCLE('',#73167,0.0999999999999994) ;
#27633=CIRCLE('',#73168,0.0999999999999994) ;
#27634=CIRCLE('',#73171,0.0999999999999994) ;
#27635=CIRCLE('',#73172,0.0999999999999994) ;
#27636=CIRCLE('',#73175,0.0999999999999994) ;
#27637=CIRCLE('',#73176,0.0999999999999994) ;
#27638=CIRCLE('',#73179,0.0999999999999994) ;
#27639=CIRCLE('',#73180,0.0999999999999994) ;
#27640=CIRCLE('',#73183,0.0999999999999994) ;
#27641=CIRCLE('',#73184,0.0999999999999994) ;
#27642=CIRCLE('',#73187,0.0999999999999994) ;
#27643=CIRCLE('',#73188,0.0999999999999994) ;
#27644=CIRCLE('',#73190,1.65625) ;
#27645=CIRCLE('',#73191,1.65625) ;
#27646=CIRCLE('',#73193,0.0999999999999994) ;
#27647=CIRCLE('',#73194,0.0999999999999994) ;
#27648=CIRCLE('',#73197,0.0999999999999994) ;
#27649=CIRCLE('',#73198,0.0999999999999994) ;
#27650=CIRCLE('',#73201,0.0999999999999994) ;
#27651=CIRCLE('',#73202,0.0999999999999994) ;
#27652=CIRCLE('',#73205,0.199999999999999) ;
#27653=CIRCLE('',#73206,0.199999999999999) ;
#27654=CIRCLE('',#73207,1.75625) ;
#27655=CIRCLE('',#73208,0.199999999999999) ;
#27656=CIRCLE('',#73209,0.199999999999999) ;
#27657=CIRCLE('',#73211,0.0999999999999994) ;
#27658=CIRCLE('',#73212,0.0999999999999994) ;
#27659=CIRCLE('',#73215,0.0999999999999994) ;
#27660=CIRCLE('',#73216,0.0999999999999994) ;
#27661=CIRCLE('',#73219,0.0999999999999994) ;
#27662=CIRCLE('',#73220,0.0999999999999994) ;
#27663=CIRCLE('',#73223,0.0999999999999994) ;
#27664=CIRCLE('',#73227,0.0999999999999994) ;
#27665=CIRCLE('',#73228,0.0999999999999994) ;
#27666=CIRCLE('',#73231,0.0999999999999994) ;
#27667=CIRCLE('',#73232,0.0999999999999994) ;
#27668=CIRCLE('',#73235,0.0999999999999994) ;
#27669=CIRCLE('',#73236,0.0999999999999994) ;
#27670=CIRCLE('',#73239,0.0999999999999994) ;
#27671=CIRCLE('',#73240,0.0999999999999994) ;
#27672=CIRCLE('',#73243,0.0999999999999994) ;
#27673=CIRCLE('',#73244,0.0999999999999994) ;
#27674=CIRCLE('',#73247,0.0999999999999994) ;
#27675=CIRCLE('',#73248,0.0999999999999994) ;
#27676=CIRCLE('',#73250,1.65625) ;
#27677=CIRCLE('',#73251,1.65625) ;
#27678=CIRCLE('',#73253,0.0999999999999994) ;
#27679=CIRCLE('',#73254,0.0999999999999994) ;
#27680=CIRCLE('',#73257,0.0999999999999994) ;
#27681=CIRCLE('',#73258,0.0999999999999994) ;
#27682=CIRCLE('',#73261,0.0999999999999994) ;
#27683=CIRCLE('',#73262,0.0999999999999994) ;
#27684=CIRCLE('',#73265,0.199999999999999) ;
#27685=CIRCLE('',#73266,0.199999999999999) ;
#27686=CIRCLE('',#73267,1.75625) ;
#27687=CIRCLE('',#73268,0.199999999999999) ;
#27688=CIRCLE('',#73269,0.199999999999999) ;
#27689=CIRCLE('',#73271,0.0999999999999994) ;
#27690=CIRCLE('',#73272,0.0999999999999994) ;
#27691=CIRCLE('',#73275,0.0999999999999994) ;
#27692=CIRCLE('',#73276,0.0999999999999994) ;
#27693=CIRCLE('',#73279,0.0999999999999994) ;
#27694=CIRCLE('',#73280,0.0999999999999994) ;
#27695=CIRCLE('',#73283,0.100000000000001) ;
#27696=CIRCLE('',#73287,0.0999999999999994) ;
#27697=CIRCLE('',#73288,0.0999999999999994) ;
#27698=CIRCLE('',#73291,0.0999999999999994) ;
#27699=CIRCLE('',#73292,0.0999999999999994) ;
#27700=CIRCLE('',#73295,0.0999999999999994) ;
#27701=CIRCLE('',#73296,0.0999999999999994) ;
#27702=CIRCLE('',#73299,0.0999999999999994) ;
#27703=CIRCLE('',#73300,0.0999999999999994) ;
#27704=CIRCLE('',#73303,0.0999999999999994) ;
#27705=CIRCLE('',#73304,0.0999999999999994) ;
#27706=CIRCLE('',#73307,0.0999999999999994) ;
#27707=CIRCLE('',#73308,0.0999999999999994) ;
#27708=CIRCLE('',#73310,1.65625) ;
#27709=CIRCLE('',#73311,1.65625) ;
#27710=CIRCLE('',#73313,0.0999999999999994) ;
#27711=CIRCLE('',#73314,0.0999999999999994) ;
#27712=CIRCLE('',#73317,0.0999999999999994) ;
#27713=CIRCLE('',#73318,0.0999999999999994) ;
#27714=CIRCLE('',#73321,0.0999999999999994) ;
#27715=CIRCLE('',#73322,0.0999999999999994) ;
#27716=CIRCLE('',#73325,0.200000000000001) ;
#27717=CIRCLE('',#73326,0.200000000000001) ;
#27718=CIRCLE('',#73327,1.75625) ;
#27719=CIRCLE('',#73328,0.199999999999999) ;
#27720=CIRCLE('',#73329,0.199999999999999) ;
#27721=CIRCLE('',#73331,0.0999999999999994) ;
#27722=CIRCLE('',#73332,0.0999999999999994) ;
#27723=CIRCLE('',#73335,0.0999999999999994) ;
#27724=CIRCLE('',#73336,0.0999999999999994) ;
#27725=CIRCLE('',#73339,0.0999999999999994) ;
#27726=CIRCLE('',#73340,0.0999999999999994) ;
#27727=CIRCLE('',#73343,0.100000000000001) ;
#27728=CIRCLE('',#73347,0.100000000000001) ;
#27729=CIRCLE('',#73348,0.100000000000001) ;
#27730=CIRCLE('',#73351,0.0999999999999994) ;
#27731=CIRCLE('',#73352,0.0999999999999994) ;
#27732=CIRCLE('',#73355,0.0999999999999994) ;
#27733=CIRCLE('',#73356,0.0999999999999994) ;
#27734=CIRCLE('',#73359,0.0999999999999994) ;
#27735=CIRCLE('',#73360,0.0999999999999994) ;
#27736=CIRCLE('',#73363,0.0999999999999994) ;
#27737=CIRCLE('',#73364,0.0999999999999994) ;
#27738=CIRCLE('',#73367,0.0999999999999994) ;
#27739=CIRCLE('',#73368,0.0999999999999994) ;
#27740=CIRCLE('',#73370,1.65625) ;
#27741=CIRCLE('',#73371,1.65625) ;
#27742=CIRCLE('',#73373,0.0999999999999994) ;
#27743=CIRCLE('',#73374,0.0999999999999994) ;
#27744=CIRCLE('',#73377,0.0999999999999994) ;
#27745=CIRCLE('',#73378,0.0999999999999994) ;
#27746=CIRCLE('',#73381,0.0999999999999994) ;
#27747=CIRCLE('',#73382,0.0999999999999994) ;
#27748=CIRCLE('',#73385,0.200000000000001) ;
#27749=CIRCLE('',#73386,0.200000000000001) ;
#27750=CIRCLE('',#73387,1.75625) ;
#27751=CIRCLE('',#73388,0.200000000000001) ;
#27752=CIRCLE('',#73389,0.200000000000001) ;
#27753=CIRCLE('',#73391,0.1) ;
#27754=CIRCLE('',#73392,0.1) ;
#27755=CIRCLE('',#73395,0.1) ;
#27756=CIRCLE('',#73396,0.1) ;
#27757=CIRCLE('',#73399,0.0999999999999994) ;
#27758=CIRCLE('',#73400,0.0999999999999994) ;
#27759=CIRCLE('',#73403,0.1) ;
#27760=CIRCLE('',#73407,0.100000000000001) ;
#27761=CIRCLE('',#73408,0.100000000000001) ;
#27762=CIRCLE('',#73411,0.0999999999999994) ;
#27763=CIRCLE('',#73412,0.0999999999999994) ;
#27764=CIRCLE('',#73415,0.0999999999999994) ;
#27765=CIRCLE('',#73416,0.0999999999999994) ;
#27766=CIRCLE('',#73419,0.0999999999999994) ;
#27767=CIRCLE('',#73420,0.0999999999999994) ;
#27768=CIRCLE('',#73423,0.0999999999999994) ;
#27769=CIRCLE('',#73424,0.0999999999999994) ;
#27770=CIRCLE('',#73427,0.0999999999999994) ;
#27771=CIRCLE('',#73428,0.0999999999999994) ;
#27772=CIRCLE('',#73430,1.65625) ;
#27773=CIRCLE('',#73431,1.65625) ;
#27774=CIRCLE('',#73433,0.1) ;
#27775=CIRCLE('',#73434,0.1) ;
#27776=CIRCLE('',#73437,0.1) ;
#27777=CIRCLE('',#73438,0.1) ;
#27778=CIRCLE('',#73441,0.1) ;
#27779=CIRCLE('',#73442,0.1) ;
#27780=CIRCLE('',#73445,0.2) ;
#27781=CIRCLE('',#73446,0.2) ;
#27782=CIRCLE('',#73447,1.75625) ;
#27783=CIRCLE('',#73448,0.200000000000001) ;
#27784=CIRCLE('',#73449,0.200000000000001) ;
#27785=CIRCLE('',#73451,0.0999999999999998) ;
#27786=CIRCLE('',#73452,0.0999999999999998) ;
#27787=CIRCLE('',#73455,0.0999999999999998) ;
#27788=CIRCLE('',#73456,0.0999999999999998) ;
#27789=CIRCLE('',#73459,0.0999999999999994) ;
#27790=CIRCLE('',#73460,0.0999999999999994) ;
#27791=CIRCLE('',#73463,0.100000000000001) ;
#27792=CIRCLE('',#73467,0.1) ;
#27793=CIRCLE('',#73468,0.1) ;
#27794=CIRCLE('',#73471,0.1) ;
#27795=CIRCLE('',#73472,0.1) ;
#27796=CIRCLE('',#73475,0.1) ;
#27797=CIRCLE('',#73476,0.1) ;
#27798=CIRCLE('',#73479,0.1) ;
#27799=CIRCLE('',#73480,0.1) ;
#27800=CIRCLE('',#73483,0.1) ;
#27801=CIRCLE('',#73484,0.1) ;
#27802=CIRCLE('',#73487,0.1) ;
#27803=CIRCLE('',#73488,0.1) ;
#27804=CIRCLE('',#73490,1.65625) ;
#27805=CIRCLE('',#73491,1.65625) ;
#27806=CIRCLE('',#73493,0.0999999999999998) ;
#27807=CIRCLE('',#73494,0.0999999999999998) ;
#27808=CIRCLE('',#73497,0.0999999999999998) ;
#27809=CIRCLE('',#73498,0.0999999999999998) ;
#27810=CIRCLE('',#73501,0.1) ;
#27811=CIRCLE('',#73502,0.1) ;
#27812=CIRCLE('',#73505,0.2) ;
#27813=CIRCLE('',#73506,0.2) ;
#27814=CIRCLE('',#73507,1.75625) ;
#27815=CIRCLE('',#73508,0.2) ;
#27816=CIRCLE('',#73509,0.2) ;
#27817=CIRCLE('',#73511,0.0999999999999998) ;
#27818=CIRCLE('',#73512,0.1) ;
#27819=CIRCLE('',#73513,0.1) ;
#27820=CIRCLE('',#73514,0.0999999999999998) ;
#27821=CIRCLE('',#73516,0.1) ;
#27822=CIRCLE('',#73517,0.0999999999999994) ;
#27823=CIRCLE('',#73518,0.0999999999999994) ;
#27824=CIRCLE('',#73519,0.1) ;
#27825=CIRCLE('',#73521,0.0999999999999994) ;
#27826=CIRCLE('',#73522,0.0999999999999994) ;
#27827=CIRCLE('',#73523,0.0999999999999994) ;
#27828=CIRCLE('',#73524,0.0999999999999994) ;
#27829=CIRCLE('',#73526,0.0999999999999994) ;
#27830=CIRCLE('',#73527,0.0999999999999994) ;
#27831=CIRCLE('',#73528,0.0999999999999994) ;
#27832=CIRCLE('',#73529,0.0999999999999994) ;
#27833=CIRCLE('',#73531,0.0999999999999994) ;
#27834=CIRCLE('',#73532,0.0999999999999994) ;
#27835=CIRCLE('',#73533,0.0999999999999994) ;
#27836=CIRCLE('',#73534,0.0999999999999994) ;
#27837=CIRCLE('',#73536,0.0999999999999994) ;
#27838=CIRCLE('',#73537,0.0999999999999994) ;
#27839=CIRCLE('',#73538,0.0999999999999994) ;
#27840=CIRCLE('',#73539,0.0999999999999994) ;
#27841=CIRCLE('',#73541,0.0999999999999994) ;
#27842=CIRCLE('',#73542,0.0999999999999994) ;
#27843=CIRCLE('',#73543,0.0999999999999994) ;
#27844=CIRCLE('',#73544,0.0999999999999994) ;
#27845=CIRCLE('',#73546,0.0999999999999994) ;
#27846=CIRCLE('',#73547,0.0999999999999994) ;
#27847=CIRCLE('',#73548,0.0999999999999994) ;
#27848=CIRCLE('',#73549,0.0999999999999994) ;
#27849=CIRCLE('',#73551,0.100000000000003) ;
#27850=CIRCLE('',#73552,0.100000000000003) ;
#27851=CIRCLE('',#73553,0.100000000000003) ;
#27852=CIRCLE('',#73554,0.100000000000003) ;
#27853=CIRCLE('',#73556,0.0999999999999998) ;
#27854=CIRCLE('',#73557,0.0999999999999998) ;
#27855=CIRCLE('',#73559,0.0999999999999998) ;
#27856=CIRCLE('',#73560,0.1) ;
#27857=CIRCLE('',#73562,0.0999999999999998) ;
#27858=CIRCLE('',#73563,0.1) ;
#27859=CIRCLE('',#73565,0.1) ;
#27860=CIRCLE('',#73566,0.0999999999999998) ;
#27861=CIRCLE('',#73568,0.1) ;
#27862=CIRCLE('',#73570,0.1) ;
#27863=CIRCLE('',#73572,0.0999999999999998) ;
#27864=CIRCLE('',#73574,0.1) ;
#27865=CIRCLE('',#73576,0.0999999999999998) ;
#27866=CIRCLE('',#73578,0.1) ;
#27867=CIRCLE('',#73580,0.1) ;
#27868=CIRCLE('',#73581,0.1) ;
#27869=CIRCLE('',#73584,0.1) ;
#27870=CIRCLE('',#73586,0.0999999999999998) ;
#27871=CIRCLE('',#73587,0.0999999999999998) ;
#27872=CIRCLE('',#73589,0.1) ;
#27873=CIRCLE('',#73591,0.1) ;
#27874=CIRCLE('',#73593,0.0999999999999998) ;
#27875=CIRCLE('',#73595,0.0999999999999998) ;
#27876=CIRCLE('',#73597,0.1) ;
#27877=CIRCLE('',#73599,0.1) ;
#27878=CIRCLE('',#73600,0.1) ;
#27879=CIRCLE('',#73602,0.1) ;
#27880=CIRCLE('',#73604,0.0999999999999998) ;
#27881=CIRCLE('',#73606,0.0999999999999998) ;
#27882=CIRCLE('',#73607,0.1) ;
#27883=CIRCLE('',#73609,0.0999999999999998) ;
#27884=CIRCLE('',#73611,0.1) ;
#27885=CIRCLE('',#73612,0.1) ;
#27886=CIRCLE('',#73614,0.1) ;
#27887=CIRCLE('',#73616,0.1) ;
#27888=CIRCLE('',#73618,0.0999999999999998) ;
#27889=CIRCLE('',#73620,0.0999999999999998) ;
#27890=CIRCLE('',#73622,0.1) ;
#27891=CIRCLE('',#73624,0.1) ;
#27892=CIRCLE('',#73626,0.1) ;
#27893=CIRCLE('',#73628,0.1) ;
#27894=CIRCLE('',#73629,0.1) ;
#27895=CIRCLE('',#73631,0.1) ;
#27896=CIRCLE('',#73633,0.1) ;
#27897=CIRCLE('',#73635,0.1) ;
#27898=CIRCLE('',#73637,0.1) ;
#27899=CIRCLE('',#73638,0.1) ;
#27900=CIRCLE('',#73640,0.1) ;
#27901=CIRCLE('',#73642,0.1) ;
#27902=CIRCLE('',#73644,0.1) ;
#27903=CIRCLE('',#73646,0.1) ;
#27904=CIRCLE('',#73649,0.1) ;
#27905=CIRCLE('',#73651,0.1) ;
#27906=CIRCLE('',#73653,0.1) ;
#27907=CIRCLE('',#73656,0.1) ;
#27908=CIRCLE('',#73657,0.1) ;
#27909=CIRCLE('',#73659,0.1) ;
#27910=CIRCLE('',#73661,0.1) ;
#27911=CIRCLE('',#73663,0.1) ;
#27912=CIRCLE('',#73665,0.1) ;
#27913=CIRCLE('',#73667,0.1) ;
#27914=CIRCLE('',#73669,0.1) ;
#27915=CIRCLE('',#73671,0.1) ;
#27916=CIRCLE('',#73673,0.1) ;
#27917=CIRCLE('',#73675,0.1) ;
#27918=CIRCLE('',#73677,0.1) ;
#27919=CIRCLE('',#73679,0.0999999999999998) ;
#27920=CIRCLE('',#73681,0.1) ;
#27921=CIRCLE('',#73683,0.1) ;
#27922=CIRCLE('',#73685,0.1) ;
#27923=CIRCLE('',#73688,0.1) ;
#27924=CIRCLE('',#73690,0.0999999999999998) ;
#27925=CIRCLE('',#73692,0.0999999999999998) ;
#27926=CIRCLE('',#73694,0.0999999999999998) ;
#27927=CIRCLE('',#73696,0.1) ;
#27928=CIRCLE('',#73698,0.1) ;
#27929=CIRCLE('',#73700,0.1) ;
#27930=CIRCLE('',#73702,0.1) ;
#27931=CIRCLE('',#73704,0.0999999999999998) ;
#27932=CIRCLE('',#73706,0.0999999999999998) ;
#27933=CIRCLE('',#73709,0.100000000000003) ;
#27934=CIRCLE('',#73710,0.100000000000003) ;
#27935=CIRCLE('',#73712,0.1) ;
#27936=CIRCLE('',#73714,0.1) ;
#27937=CIRCLE('',#73716,0.1) ;
#27938=CIRCLE('',#73718,0.0999999999999998) ;
#27939=CIRCLE('',#73720,0.0999999999999998) ;
#27940=CIRCLE('',#73722,0.100000000000003) ;
#27941=CIRCLE('',#73725,0.100000000000003) ;
#27942=CIRCLE('',#73727,0.0999999999999994) ;
#27943=CIRCLE('',#73729,0.0999999999999994) ;
#27944=CIRCLE('',#73731,0.0999999999999994) ;
#27945=CIRCLE('',#73733,0.0999999999999998) ;
#27946=CIRCLE('',#73735,0.1) ;
#27947=CIRCLE('',#73737,0.0999999999999995) ;
#27948=CIRCLE('',#73739,0.1) ;
#27949=CIRCLE('',#73741,0.1) ;
#27950=CIRCLE('',#73743,0.0999999999999994) ;
#27951=CIRCLE('',#73745,0.1) ;
#27952=CIRCLE('',#73747,0.0999999999999998) ;
#27953=CIRCLE('',#73749,0.100000000000003) ;
#27954=CIRCLE('',#73751,0.100000000000003) ;
#27955=CIRCLE('',#73753,0.100000000000003) ;
#27956=CIRCLE('',#73755,0.100000000000003) ;
#27957=CIRCLE('',#73757,0.0999999999999994) ;
#27958=CIRCLE('',#73759,0.1) ;
#27959=CIRCLE('',#73762,0.0999999999999994) ;
#27960=CIRCLE('',#73763,0.0999999999999994) ;
#27961=CIRCLE('',#73765,0.1) ;
#27962=CIRCLE('',#73767,0.1) ;
#27963=CIRCLE('',#73769,0.1) ;
#27964=CIRCLE('',#73771,0.1) ;
#27965=CIRCLE('',#73773,0.0999999999999998) ;
#27966=CIRCLE('',#73775,0.100000000000003) ;
#27967=CIRCLE('',#73778,0.100000000000003) ;
#27968=CIRCLE('',#73780,0.0999999999999994) ;
#27969=CIRCLE('',#73782,0.0999999999999994) ;
#27970=CIRCLE('',#73784,0.0999999999999994) ;
#27971=CIRCLE('',#73786,0.1) ;
#27972=CIRCLE('',#73788,0.1) ;
#27973=CIRCLE('',#73790,0.0999999999999995) ;
#27974=CIRCLE('',#73792,0.1) ;
#27975=CIRCLE('',#73794,0.1) ;
#27976=CIRCLE('',#73796,0.0999999999999994) ;
#27977=CIRCLE('',#73798,0.1) ;
#27978=CIRCLE('',#73800,0.0999999999999994) ;
#27979=CIRCLE('',#73802,0.0999999999999994) ;
#27980=CIRCLE('',#73804,0.0999999999999994) ;
#27981=CIRCLE('',#73806,0.0999999999999994) ;
#27982=CIRCLE('',#73808,0.0999999999999994) ;
#27983=CIRCLE('',#73810,0.0999999999999994) ;
#27984=CIRCLE('',#73812,0.1) ;
#27985=CIRCLE('',#73815,0.0999999999999994) ;
#27986=CIRCLE('',#73816,0.0999999999999994) ;
#27987=CIRCLE('',#73818,0.1) ;
#27988=CIRCLE('',#73820,0.1) ;
#27989=CIRCLE('',#73822,0.1) ;
#27990=CIRCLE('',#73824,0.1) ;
#27991=CIRCLE('',#73826,0.1) ;
#27992=CIRCLE('',#73828,0.0999999999999994) ;
#27993=CIRCLE('',#73831,0.0999999999999994) ;
#27994=CIRCLE('',#73833,0.0999999999999994) ;
#27995=CIRCLE('',#73835,0.0999999999999994) ;
#27996=CIRCLE('',#73837,0.0999999999999994) ;
#27997=CIRCLE('',#73839,0.1) ;
#27998=CIRCLE('',#73841,0.1) ;
#27999=CIRCLE('',#73843,0.0999999999999995) ;
#28000=CIRCLE('',#73845,0.1) ;
#28001=CIRCLE('',#73847,0.1) ;
#28002=CIRCLE('',#73849,0.0999999999999994) ;
#28003=CIRCLE('',#73851,0.1) ;
#28004=CIRCLE('',#73853,0.0999999999999994) ;
#28005=CIRCLE('',#73855,0.0999999999999994) ;
#28006=CIRCLE('',#73857,0.0999999999999994) ;
#28007=CIRCLE('',#73859,0.0999999999999994) ;
#28008=CIRCLE('',#73861,0.0999999999999994) ;
#28009=CIRCLE('',#73863,0.0999999999999994) ;
#28010=CIRCLE('',#73865,0.1) ;
#28011=CIRCLE('',#73868,0.0999999999999994) ;
#28012=CIRCLE('',#73869,0.0999999999999994) ;
#28013=CIRCLE('',#73871,0.1) ;
#28014=CIRCLE('',#73873,0.1) ;
#28015=CIRCLE('',#73875,0.1) ;
#28016=CIRCLE('',#73877,0.1) ;
#28017=CIRCLE('',#73879,0.1) ;
#28018=CIRCLE('',#73881,0.0999999999999994) ;
#28019=CIRCLE('',#73884,0.0999999999999994) ;
#28020=CIRCLE('',#73886,0.0999999999999994) ;
#28021=CIRCLE('',#73888,0.0999999999999994) ;
#28022=CIRCLE('',#73890,0.0999999999999994) ;
#28023=CIRCLE('',#73892,0.1) ;
#28024=CIRCLE('',#73894,0.1) ;
#28025=CIRCLE('',#73896,0.0999999999999995) ;
#28026=CIRCLE('',#73898,0.1) ;
#28027=CIRCLE('',#73900,0.1) ;
#28028=CIRCLE('',#73902,0.0999999999999994) ;
#28029=CIRCLE('',#73904,0.1) ;
#28030=CIRCLE('',#73906,0.0999999999999994) ;
#28031=CIRCLE('',#73908,0.0999999999999994) ;
#28032=CIRCLE('',#73910,0.0999999999999994) ;
#28033=CIRCLE('',#73912,0.0999999999999994) ;
#28034=CIRCLE('',#73914,0.0999999999999994) ;
#28035=CIRCLE('',#73916,0.0999999999999994) ;
#28036=CIRCLE('',#73918,0.1) ;
#28037=CIRCLE('',#73921,0.0999999999999994) ;
#28038=CIRCLE('',#73922,0.0999999999999994) ;
#28039=CIRCLE('',#73924,0.1) ;
#28040=CIRCLE('',#73926,0.1) ;
#28041=CIRCLE('',#73928,0.1) ;
#28042=CIRCLE('',#73930,0.1) ;
#28043=CIRCLE('',#73932,0.1) ;
#28044=CIRCLE('',#73934,0.0999999999999994) ;
#28045=CIRCLE('',#73937,0.0999999999999994) ;
#28046=CIRCLE('',#73939,0.0999999999999994) ;
#28047=CIRCLE('',#73941,0.0999999999999994) ;
#28048=CIRCLE('',#73943,0.0999999999999994) ;
#28049=CIRCLE('',#73945,0.1) ;
#28050=CIRCLE('',#73947,0.1) ;
#28051=CIRCLE('',#73949,0.0999999999999995) ;
#28052=CIRCLE('',#73951,0.1) ;
#28053=CIRCLE('',#73953,0.1) ;
#28054=CIRCLE('',#73955,0.0999999999999994) ;
#28055=CIRCLE('',#73957,0.1) ;
#28056=CIRCLE('',#73959,0.0999999999999994) ;
#28057=CIRCLE('',#73961,0.0999999999999994) ;
#28058=CIRCLE('',#73963,0.0999999999999994) ;
#28059=CIRCLE('',#73965,0.0999999999999994) ;
#28060=CIRCLE('',#73967,0.0999999999999994) ;
#28061=CIRCLE('',#73969,0.0999999999999994) ;
#28062=CIRCLE('',#73971,0.1) ;
#28063=CIRCLE('',#73974,0.0999999999999994) ;
#28064=CIRCLE('',#73975,0.0999999999999994) ;
#28065=CIRCLE('',#73977,0.1) ;
#28066=CIRCLE('',#73979,0.1) ;
#28067=CIRCLE('',#73981,0.1) ;
#28068=CIRCLE('',#73983,0.1) ;
#28069=CIRCLE('',#73985,0.1) ;
#28070=CIRCLE('',#73987,0.0999999999999994) ;
#28071=CIRCLE('',#73990,0.0999999999999994) ;
#28072=CIRCLE('',#73992,0.0999999999999994) ;
#28073=CIRCLE('',#73994,0.0999999999999994) ;
#28074=CIRCLE('',#73996,0.0999999999999994) ;
#28075=CIRCLE('',#73998,0.1) ;
#28076=CIRCLE('',#74000,0.1) ;
#28077=CIRCLE('',#74002,0.1) ;
#28078=CIRCLE('',#74004,0.1) ;
#28079=CIRCLE('',#74006,0.1) ;
#28080=CIRCLE('',#74008,0.0999999999999994) ;
#28081=CIRCLE('',#74010,0.1) ;
#28082=CIRCLE('',#74012,0.0999999999999994) ;
#28083=CIRCLE('',#74014,0.0999999999999994) ;
#28084=CIRCLE('',#74016,0.0999999999999994) ;
#28085=CIRCLE('',#74018,0.0999999999999994) ;
#28086=CIRCLE('',#74020,0.0999999999999994) ;
#28087=CIRCLE('',#74022,0.0999999999999994) ;
#28088=CIRCLE('',#74024,0.1) ;
#28089=CIRCLE('',#74027,0.0999999999999994) ;
#28090=CIRCLE('',#74028,0.0999999999999994) ;
#28091=CIRCLE('',#74030,0.1) ;
#28092=CIRCLE('',#74032,0.1) ;
#28093=CIRCLE('',#74034,0.1) ;
#28094=CIRCLE('',#74036,0.1) ;
#28095=CIRCLE('',#74038,0.1) ;
#28096=CIRCLE('',#74040,0.0999999999999994) ;
#28097=CIRCLE('',#74043,0.0999999999999994) ;
#28098=CIRCLE('',#74045,0.0999999999999994) ;
#28099=CIRCLE('',#74047,0.0999999999999994) ;
#28100=CIRCLE('',#74049,0.0999999999999994) ;
#28101=CIRCLE('',#74051,0.1) ;
#28102=CIRCLE('',#74053,0.1) ;
#28103=CIRCLE('',#74055,0.1) ;
#28104=CIRCLE('',#74057,0.1) ;
#28105=CIRCLE('',#74059,0.1) ;
#28106=CIRCLE('',#74061,0.0999999999999994) ;
#28107=CIRCLE('',#74063,0.1) ;
#28108=CIRCLE('',#74065,0.0999999999999994) ;
#28109=CIRCLE('',#74067,0.0999999999999994) ;
#28110=CIRCLE('',#74069,0.0999999999999994) ;
#28111=CIRCLE('',#74071,0.0999999999999994) ;
#28112=CIRCLE('',#74073,0.0999999999999994) ;
#28113=CIRCLE('',#74075,0.0999999999999994) ;
#28114=CIRCLE('',#74077,0.1) ;
#28115=CIRCLE('',#74080,0.0999999999999994) ;
#28116=CIRCLE('',#74081,0.0999999999999994) ;
#28117=CIRCLE('',#74083,0.1) ;
#28118=CIRCLE('',#74085,0.1) ;
#28119=CIRCLE('',#74087,0.1) ;
#28120=CIRCLE('',#74089,0.1) ;
#28121=CIRCLE('',#74091,0.1) ;
#28122=CIRCLE('',#74093,0.0999999999999994) ;
#28123=CIRCLE('',#74096,0.0999999999999994) ;
#28124=CIRCLE('',#74098,0.0999999999999994) ;
#28125=CIRCLE('',#74100,0.0999999999999994) ;
#28126=CIRCLE('',#74102,0.0999999999999994) ;
#28127=CIRCLE('',#74104,0.1) ;
#28128=CIRCLE('',#74106,0.1) ;
#28129=CIRCLE('',#74108,0.1) ;
#28130=CIRCLE('',#74110,0.1) ;
#28131=CIRCLE('',#74112,0.0999999999999998) ;
#28132=CIRCLE('',#74114,0.0999999999999994) ;
#28133=CIRCLE('',#74116,0.1) ;
#28134=CIRCLE('',#74118,0.0999999999999994) ;
#28135=CIRCLE('',#74120,0.1) ;
#28136=CIRCLE('',#74122,0.1) ;
#28137=CIRCLE('',#74124,0.1) ;
#28138=CIRCLE('',#74126,0.1) ;
#28139=CIRCLE('',#74128,0.0999999999999994) ;
#28140=CIRCLE('',#74130,0.1) ;
#28141=CIRCLE('',#74133,0.1) ;
#28142=CIRCLE('',#74134,0.1) ;
#28143=CIRCLE('',#74136,0.1) ;
#28144=CIRCLE('',#74138,0.1) ;
#28145=CIRCLE('',#74140,0.1) ;
#28146=CIRCLE('',#74142,0.0999999999999998) ;
#28147=CIRCLE('',#74144,0.1) ;
#28148=CIRCLE('',#74146,0.1) ;
#28149=CIRCLE('',#74149,0.1) ;
#28150=CIRCLE('',#74151,0.0999999999999994) ;
#28151=CIRCLE('',#74153,0.0999999999999994) ;
#28152=CIRCLE('',#74155,0.0999999999999994) ;
#28153=CIRCLE('',#74157,0.0999999999999998) ;
#28154=CIRCLE('',#74159,0.1) ;
#28155=CIRCLE('',#74161,0.0999999999999998) ;
#28156=CIRCLE('',#74163,0.1) ;
#28157=CIRCLE('',#74165,0.1) ;
#28158=CIRCLE('',#74167,0.0999999999999994) ;
#28159=CIRCLE('',#74169,0.0999999999999998) ;
#28160=CIRCLE('',#74171,0.0999999999999998) ;
#28161=CIRCLE('',#74173,0.0999999999999998) ;
#28162=CIRCLE('',#74175,0.0999999999999998) ;
#28163=CIRCLE('',#74177,0.0999999999999998) ;
#28164=CIRCLE('',#74179,0.0999999999999998) ;
#28165=CIRCLE('',#74181,0.0999999999999994) ;
#28166=CIRCLE('',#74183,0.1) ;
#28167=CIRCLE('',#74186,0.1) ;
#28168=CIRCLE('',#74187,0.1) ;
#28169=CIRCLE('',#74189,0.1) ;
#28170=CIRCLE('',#74190,0.1) ;
#28171=CIRCLE('',#74192,0.1) ;
#28172=CIRCLE('',#74193,0.1) ;
#28173=CIRCLE('',#74195,0.1) ;
#28174=CIRCLE('',#74196,0.0999999999999998) ;
#28175=CIRCLE('',#74198,0.1) ;
#28176=CIRCLE('',#74200,0.1) ;
#28177=CIRCLE('',#74202,0.1) ;
#28178=CIRCLE('',#74204,0.1) ;
#28179=CIRCLE('',#74206,0.0999999999999998) ;
#28180=CIRCLE('',#74208,0.1) ;
#28181=CIRCLE('',#74210,0.0999999999999994) ;
#28182=CIRCLE('',#74211,0.1) ;
#28183=CIRCLE('',#74214,0.1) ;
#28184=CIRCLE('',#74216,0.1) ;
#28185=CIRCLE('',#74217,0.1) ;
#28186=CIRCLE('',#74219,0.0999999999999994) ;
#28187=CIRCLE('',#74221,0.1) ;
#28188=CIRCLE('',#74223,0.1) ;
#28189=CIRCLE('',#74225,0.1) ;
#28190=CIRCLE('',#74227,0.0999999999999994) ;
#28191=CIRCLE('',#74229,0.1) ;
#28192=CIRCLE('',#74230,0.0999999999999994) ;
#28193=CIRCLE('',#74232,0.1) ;
#28194=CIRCLE('',#74234,0.1) ;
#28195=CIRCLE('',#74236,0.0999999999999998) ;
#28196=CIRCLE('',#74237,0.1) ;
#28197=CIRCLE('',#74239,0.1) ;
#28198=CIRCLE('',#74241,0.1) ;
#28199=CIRCLE('',#74242,0.1) ;
#28200=CIRCLE('',#74244,0.1) ;
#28201=CIRCLE('',#74246,0.1) ;
#28202=CIRCLE('',#74248,0.1) ;
#28203=CIRCLE('',#74250,0.1) ;
#28204=CIRCLE('',#74252,0.1) ;
#28205=CIRCLE('',#74254,0.1) ;
#28206=CIRCLE('',#74256,0.1) ;
#28207=CIRCLE('',#74258,0.0999999999999994) ;
#28208=CIRCLE('',#74259,0.0999999999999994) ;
#28209=CIRCLE('',#74261,0.1) ;
#28210=CIRCLE('',#74263,0.1) ;
#28211=CIRCLE('',#74265,0.1) ;
#28212=CIRCLE('',#74267,0.1) ;
#28213=CIRCLE('',#74268,0.0999999999999994) ;
#28214=CIRCLE('',#74270,0.0999999999999994) ;
#28215=CIRCLE('',#74272,0.0999999999999994) ;
#28216=CIRCLE('',#74274,0.1) ;
#28217=CIRCLE('',#74276,0.0999999999999994) ;
#28218=CIRCLE('',#74279,0.0999999999999994) ;
#28219=CIRCLE('',#74281,0.1) ;
#28220=CIRCLE('',#74283,0.0999999999999994) ;
#28221=CIRCLE('',#74286,0.1) ;
#28222=CIRCLE('',#74287,0.1) ;
#28223=CIRCLE('',#74289,0.0999999999999994) ;
#28224=CIRCLE('',#74291,0.0999999999999994) ;
#28225=CIRCLE('',#74293,0.0999999999999994) ;
#28226=CIRCLE('',#74295,0.0999999999999994) ;
#28227=CIRCLE('',#74297,0.1) ;
#28228=CIRCLE('',#74299,0.0999999999999998) ;
#28229=CIRCLE('',#74301,0.1) ;
#28230=CIRCLE('',#74303,0.1) ;
#28231=CIRCLE('',#74305,0.1) ;
#28232=CIRCLE('',#74307,0.1) ;
#28233=CIRCLE('',#74309,0.1) ;
#28234=CIRCLE('',#74311,0.1) ;
#28235=CIRCLE('',#74313,0.1) ;
#28236=CIRCLE('',#74315,0.1) ;
#28237=CIRCLE('',#74318,0.1) ;
#28238=CIRCLE('',#74320,0.1) ;
#28239=CIRCLE('',#74322,0.1) ;
#28240=CIRCLE('',#74324,0.1) ;
#28241=CIRCLE('',#74326,0.0999999999999998) ;
#28242=CIRCLE('',#74328,0.1) ;
#28243=CIRCLE('',#74330,0.1) ;
#28244=CIRCLE('',#74332,0.1) ;
#28245=CIRCLE('',#74334,0.1) ;
#28246=CIRCLE('',#74336,0.1) ;
#28247=CIRCLE('',#74339,0.0999999999999994) ;
#28248=CIRCLE('',#74340,0.0999999999999994) ;
#28249=CIRCLE('',#74342,0.0999999999999994) ;
#28250=CIRCLE('',#74343,0.1) ;
#28251=CIRCLE('',#74345,0.0999999999999994) ;
#28252=CIRCLE('',#74346,0.1) ;
#28253=CIRCLE('',#74348,0.1) ;
#28254=CIRCLE('',#74349,0.0999999999999998) ;
#28255=CIRCLE('',#74351,0.1) ;
#28256=CIRCLE('',#74353,0.1) ;
#28257=CIRCLE('',#74355,0.0999999999999994) ;
#28258=CIRCLE('',#74357,0.1) ;
#28259=CIRCLE('',#74359,0.0999999999999998) ;
#28260=CIRCLE('',#74361,0.1) ;
#28261=CIRCLE('',#74363,0.0999999999999994) ;
#28262=CIRCLE('',#74364,0.1) ;
#28263=CIRCLE('',#74367,0.1) ;
#28264=CIRCLE('',#74369,0.0999999999999994) ;
#28265=CIRCLE('',#74370,0.0999999999999994) ;
#28266=CIRCLE('',#74372,0.0999999999999994) ;
#28267=CIRCLE('',#74374,0.1) ;
#28268=CIRCLE('',#74376,0.0999999999999994) ;
#28269=CIRCLE('',#74378,0.0999999999999994) ;
#28270=CIRCLE('',#74380,0.0999999999999994) ;
#28271=CIRCLE('',#74382,0.1) ;
#28272=CIRCLE('',#74383,0.0999999999999994) ;
#28273=CIRCLE('',#74385,0.1) ;
#28274=CIRCLE('',#74387,0.0999999999999994) ;
#28275=CIRCLE('',#74389,0.0999999999999998) ;
#28276=CIRCLE('',#74390,0.1) ;
#28277=CIRCLE('',#74392,0.0999999999999994) ;
#28278=CIRCLE('',#74394,0.1) ;
#28279=CIRCLE('',#74395,0.1) ;
#28280=CIRCLE('',#74397,0.1) ;
#28281=CIRCLE('',#74399,0.1) ;
#28282=CIRCLE('',#74401,0.0999999999999994) ;
#28283=CIRCLE('',#74403,0.0999999999999994) ;
#28284=CIRCLE('',#74405,0.1) ;
#28285=CIRCLE('',#74407,0.1) ;
#28286=CIRCLE('',#74409,0.1) ;
#28287=CIRCLE('',#74411,0.0999999999999994) ;
#28288=CIRCLE('',#74412,0.0999999999999994) ;
#28289=CIRCLE('',#74414,0.1) ;
#28290=CIRCLE('',#74416,0.1) ;
#28291=CIRCLE('',#74418,0.1) ;
#28292=CIRCLE('',#74420,0.1) ;
#28293=CIRCLE('',#74421,0.0999999999999994) ;
#28294=CIRCLE('',#74423,0.0999999999999994) ;
#28295=CIRCLE('',#74425,0.0999999999999994) ;
#28296=CIRCLE('',#74427,0.1) ;
#28297=CIRCLE('',#74429,0.0999999999999994) ;
#28298=CIRCLE('',#74432,0.0999999999999994) ;
#28299=CIRCLE('',#74434,0.1) ;
#28300=CIRCLE('',#74436,0.0999999999999994) ;
#28301=CIRCLE('',#74439,0.1) ;
#28302=CIRCLE('',#74440,0.1) ;
#28303=CIRCLE('',#74442,0.0999999999999994) ;
#28304=CIRCLE('',#74444,0.0999999999999994) ;
#28305=CIRCLE('',#74446,0.0999999999999994) ;
#28306=CIRCLE('',#74448,0.0999999999999994) ;
#28307=CIRCLE('',#74450,0.1) ;
#28308=CIRCLE('',#74452,0.0999999999999998) ;
#28309=CIRCLE('',#74454,0.1) ;
#28310=CIRCLE('',#74456,0.1) ;
#28311=CIRCLE('',#74458,0.1) ;
#28312=CIRCLE('',#74460,0.1) ;
#28313=CIRCLE('',#74462,0.1) ;
#28314=CIRCLE('',#74464,0.1) ;
#28315=CIRCLE('',#74466,0.1) ;
#28316=CIRCLE('',#74468,0.1) ;
#28317=CIRCLE('',#74471,0.1) ;
#28318=CIRCLE('',#74473,0.0999999999999994) ;
#28319=CIRCLE('',#74475,0.1) ;
#28320=CIRCLE('',#74477,0.0999999999999994) ;
#28321=CIRCLE('',#74479,0.1) ;
#28322=CIRCLE('',#74481,0.1) ;
#28323=CIRCLE('',#74483,0.1) ;
#28324=CIRCLE('',#74485,0.1) ;
#28325=CIRCLE('',#74487,0.0999999999999994) ;
#28326=CIRCLE('',#74489,0.0999999999999994) ;
#28327=CIRCLE('',#74492,0.0999999999999994) ;
#28328=CIRCLE('',#74493,0.0999999999999994) ;
#28329=CIRCLE('',#74495,0.0999999999999994) ;
#28330=CIRCLE('',#74496,0.1) ;
#28331=CIRCLE('',#74498,0.0999999999999994) ;
#28332=CIRCLE('',#74499,0.1) ;
#28333=CIRCLE('',#74501,0.1) ;
#28334=CIRCLE('',#74502,0.0999999999999998) ;
#28335=CIRCLE('',#74504,0.1) ;
#28336=CIRCLE('',#74506,0.1) ;
#28337=CIRCLE('',#74508,0.0999999999999994) ;
#28338=CIRCLE('',#74510,0.1) ;
#28339=CIRCLE('',#74512,0.0999999999999998) ;
#28340=CIRCLE('',#74514,0.1) ;
#28341=CIRCLE('',#74516,0.0999999999999994) ;
#28342=CIRCLE('',#74517,0.1) ;
#28343=CIRCLE('',#74520,0.1) ;
#28344=CIRCLE('',#74522,0.0999999999999994) ;
#28345=CIRCLE('',#74523,0.0999999999999994) ;
#28346=CIRCLE('',#74525,0.0999999999999994) ;
#28347=CIRCLE('',#74527,0.1) ;
#28348=CIRCLE('',#74529,0.0999999999999994) ;
#28349=CIRCLE('',#74531,0.0999999999999994) ;
#28350=CIRCLE('',#74533,0.0999999999999994) ;
#28351=CIRCLE('',#74535,0.1) ;
#28352=CIRCLE('',#74536,0.0999999999999994) ;
#28353=CIRCLE('',#74538,0.1) ;
#28354=CIRCLE('',#74540,0.0999999999999994) ;
#28355=CIRCLE('',#74542,0.0999999999999998) ;
#28356=CIRCLE('',#74543,0.1) ;
#28357=CIRCLE('',#74545,0.0999999999999994) ;
#28358=CIRCLE('',#74547,0.1) ;
#28359=CIRCLE('',#74548,0.1) ;
#28360=CIRCLE('',#74550,0.1) ;
#28361=CIRCLE('',#74552,0.1) ;
#28362=CIRCLE('',#74554,0.0999999999999994) ;
#28363=CIRCLE('',#74556,0.0999999999999994) ;
#28364=CIRCLE('',#74558,0.1) ;
#28365=CIRCLE('',#74560,0.1) ;
#28366=CIRCLE('',#74562,0.1) ;
#28367=CIRCLE('',#74564,0.0999999999999994) ;
#28368=CIRCLE('',#74565,0.0999999999999994) ;
#28369=CIRCLE('',#74567,0.1) ;
#28370=CIRCLE('',#74569,0.1) ;
#28371=CIRCLE('',#74571,0.1) ;
#28372=CIRCLE('',#74573,0.1) ;
#28373=CIRCLE('',#74574,0.0999999999999994) ;
#28374=CIRCLE('',#74576,0.0999999999999994) ;
#28375=CIRCLE('',#74578,0.0999999999999994) ;
#28376=CIRCLE('',#74580,0.1) ;
#28377=CIRCLE('',#74582,0.0999999999999994) ;
#28378=CIRCLE('',#74585,0.0999999999999994) ;
#28379=CIRCLE('',#74587,0.1) ;
#28380=CIRCLE('',#74589,0.0999999999999994) ;
#28381=CIRCLE('',#74592,0.1) ;
#28382=CIRCLE('',#74593,0.1) ;
#28383=CIRCLE('',#74595,0.0999999999999994) ;
#28384=CIRCLE('',#74597,0.0999999999999994) ;
#28385=CIRCLE('',#74599,0.0999999999999994) ;
#28386=CIRCLE('',#74601,0.0999999999999994) ;
#28387=CIRCLE('',#74603,0.1) ;
#28388=CIRCLE('',#74605,0.1) ;
#28389=CIRCLE('',#74607,0.1) ;
#28390=CIRCLE('',#74609,0.1) ;
#28391=CIRCLE('',#74611,0.1) ;
#28392=CIRCLE('',#74613,0.1) ;
#28393=CIRCLE('',#74615,0.100000000000001) ;
#28394=CIRCLE('',#74617,0.1) ;
#28395=CIRCLE('',#74619,0.1) ;
#28396=CIRCLE('',#74621,0.1) ;
#28397=CIRCLE('',#74624,0.1) ;
#28398=CIRCLE('',#74626,0.0999999999999994) ;
#28399=CIRCLE('',#74628,0.1) ;
#28400=CIRCLE('',#74630,0.0999999999999994) ;
#28401=CIRCLE('',#74632,0.1) ;
#28402=CIRCLE('',#74634,0.1) ;
#28403=CIRCLE('',#74636,0.1) ;
#28404=CIRCLE('',#74638,0.1) ;
#28405=CIRCLE('',#74640,0.0999999999999994) ;
#28406=CIRCLE('',#74642,0.0999999999999994) ;
#28407=CIRCLE('',#74645,0.0999999999999994) ;
#28408=CIRCLE('',#74646,0.0999999999999994) ;
#28409=CIRCLE('',#74648,0.0999999999999994) ;
#28410=CIRCLE('',#74649,0.1) ;
#28411=CIRCLE('',#74651,0.0999999999999994) ;
#28412=CIRCLE('',#74652,0.1) ;
#28413=CIRCLE('',#74654,0.1) ;
#28414=CIRCLE('',#74655,0.0999999999999998) ;
#28415=CIRCLE('',#74657,0.1) ;
#28416=CIRCLE('',#74659,0.1) ;
#28417=CIRCLE('',#74661,0.0999999999999994) ;
#28418=CIRCLE('',#74663,0.1) ;
#28419=CIRCLE('',#74665,0.0999999999999998) ;
#28420=CIRCLE('',#74667,0.1) ;
#28421=CIRCLE('',#74669,0.0999999999999994) ;
#28422=CIRCLE('',#74670,0.1) ;
#28423=CIRCLE('',#74673,0.1) ;
#28424=CIRCLE('',#74675,0.0999999999999994) ;
#28425=CIRCLE('',#74676,0.0999999999999994) ;
#28426=CIRCLE('',#74678,0.0999999999999994) ;
#28427=CIRCLE('',#74680,0.1) ;
#28428=CIRCLE('',#74682,0.0999999999999994) ;
#28429=CIRCLE('',#74684,0.0999999999999994) ;
#28430=CIRCLE('',#74686,0.0999999999999994) ;
#28431=CIRCLE('',#74688,0.1) ;
#28432=CIRCLE('',#74689,0.0999999999999994) ;
#28433=CIRCLE('',#74691,0.1) ;
#28434=CIRCLE('',#74693,0.0999999999999994) ;
#28435=CIRCLE('',#74695,0.0999999999999998) ;
#28436=CIRCLE('',#74696,0.1) ;
#28437=CIRCLE('',#74698,0.0999999999999994) ;
#28438=CIRCLE('',#74700,0.1) ;
#28439=CIRCLE('',#74701,0.1) ;
#28440=CIRCLE('',#74703,0.1) ;
#28441=CIRCLE('',#74705,0.1) ;
#28442=CIRCLE('',#74707,0.0999999999999994) ;
#28443=CIRCLE('',#74709,0.0999999999999994) ;
#28444=CIRCLE('',#74711,0.1) ;
#28445=CIRCLE('',#74713,0.1) ;
#28446=CIRCLE('',#74715,0.1) ;
#28447=CIRCLE('',#74717,0.0999999999999994) ;
#28448=CIRCLE('',#74718,0.0999999999999994) ;
#28449=CIRCLE('',#74720,0.1) ;
#28450=CIRCLE('',#74722,0.1) ;
#28451=CIRCLE('',#74724,0.1) ;
#28452=CIRCLE('',#74726,0.1) ;
#28453=CIRCLE('',#74727,0.0999999999999994) ;
#28454=CIRCLE('',#74729,0.0999999999999994) ;
#28455=CIRCLE('',#74731,0.0999999999999994) ;
#28456=CIRCLE('',#74733,0.1) ;
#28457=CIRCLE('',#74735,0.0999999999999994) ;
#28458=CIRCLE('',#74738,0.0999999999999994) ;
#28459=CIRCLE('',#74740,0.1) ;
#28460=CIRCLE('',#74742,0.0999999999999994) ;
#28461=CIRCLE('',#74745,0.1) ;
#28462=CIRCLE('',#74746,0.1) ;
#28463=CIRCLE('',#74748,0.0999999999999994) ;
#28464=CIRCLE('',#74750,0.0999999999999994) ;
#28465=CIRCLE('',#74752,0.0999999999999994) ;
#28466=CIRCLE('',#74754,0.0999999999999994) ;
#28467=CIRCLE('',#74756,0.1) ;
#28468=CIRCLE('',#74758,0.1) ;
#28469=CIRCLE('',#74760,0.1) ;
#28470=CIRCLE('',#74762,0.1) ;
#28471=CIRCLE('',#74764,0.1) ;
#28472=CIRCLE('',#74766,0.1) ;
#28473=CIRCLE('',#74768,0.0999999999999989) ;
#28474=CIRCLE('',#74770,0.1) ;
#28475=CIRCLE('',#74772,0.1) ;
#28476=CIRCLE('',#74774,0.1) ;
#28477=CIRCLE('',#74777,0.1) ;
#28478=CIRCLE('',#74779,0.0999999999999994) ;
#28479=CIRCLE('',#74781,0.0999999999999995) ;
#28480=CIRCLE('',#74783,0.0999999999999994) ;
#28481=CIRCLE('',#74785,0.1) ;
#28482=CIRCLE('',#74787,0.1) ;
#28483=CIRCLE('',#74789,0.1) ;
#28484=CIRCLE('',#74791,0.1) ;
#28485=CIRCLE('',#74793,0.0999999999999994) ;
#28486=CIRCLE('',#74795,0.0999999999999994) ;
#28487=CIRCLE('',#74798,0.0999999999999994) ;
#28488=CIRCLE('',#74799,0.0999999999999994) ;
#28489=CIRCLE('',#74801,0.0999999999999994) ;
#28490=CIRCLE('',#74802,0.1) ;
#28491=CIRCLE('',#74804,0.0999999999999994) ;
#28492=CIRCLE('',#74805,0.1) ;
#28493=CIRCLE('',#74807,0.1) ;
#28494=CIRCLE('',#74808,0.0999999999999998) ;
#28495=CIRCLE('',#74810,0.1) ;
#28496=CIRCLE('',#74812,0.1) ;
#28497=CIRCLE('',#74814,0.0999999999999994) ;
#28498=CIRCLE('',#74816,0.1) ;
#28499=CIRCLE('',#74818,0.0999999999999998) ;
#28500=CIRCLE('',#74820,0.1) ;
#28501=CIRCLE('',#74822,0.0999999999999994) ;
#28502=CIRCLE('',#74823,0.1) ;
#28503=CIRCLE('',#74826,0.1) ;
#28504=CIRCLE('',#74828,0.0999999999999994) ;
#28505=CIRCLE('',#74829,0.0999999999999994) ;
#28506=CIRCLE('',#74831,0.0999999999999994) ;
#28507=CIRCLE('',#74833,0.1) ;
#28508=CIRCLE('',#74835,0.0999999999999994) ;
#28509=CIRCLE('',#74837,0.0999999999999994) ;
#28510=CIRCLE('',#74839,0.0999999999999994) ;
#28511=CIRCLE('',#74841,0.1) ;
#28512=CIRCLE('',#74842,0.0999999999999994) ;
#28513=CIRCLE('',#74844,0.1) ;
#28514=CIRCLE('',#74846,0.0999999999999994) ;
#28515=CIRCLE('',#74848,0.0999999999999998) ;
#28516=CIRCLE('',#74849,0.1) ;
#28517=CIRCLE('',#74851,0.0999999999999994) ;
#28518=CIRCLE('',#74853,0.1) ;
#28519=CIRCLE('',#74854,0.1) ;
#28520=CIRCLE('',#74856,0.1) ;
#28521=CIRCLE('',#74858,0.1) ;
#28522=CIRCLE('',#74860,0.0999999999999994) ;
#28523=CIRCLE('',#74862,0.0999999999999994) ;
#28524=CIRCLE('',#74864,0.1) ;
#28525=CIRCLE('',#74866,0.1) ;
#28526=CIRCLE('',#74868,0.1) ;
#28527=CIRCLE('',#74870,0.0999999999999994) ;
#28528=CIRCLE('',#74871,0.0999999999999994) ;
#28529=CIRCLE('',#74873,0.1) ;
#28530=CIRCLE('',#74875,0.1) ;
#28531=CIRCLE('',#74877,0.1) ;
#28532=CIRCLE('',#74879,0.1) ;
#28533=CIRCLE('',#74880,0.0999999999999994) ;
#28534=CIRCLE('',#74882,0.0999999999999994) ;
#28535=CIRCLE('',#74884,0.0999999999999994) ;
#28536=CIRCLE('',#74886,0.1) ;
#28537=CIRCLE('',#74888,0.0999999999999994) ;
#28538=CIRCLE('',#74891,0.0999999999999994) ;
#28539=CIRCLE('',#74893,0.1) ;
#28540=CIRCLE('',#74895,0.0999999999999994) ;
#28541=CIRCLE('',#74898,0.1) ;
#28542=CIRCLE('',#74899,0.1) ;
#28543=CIRCLE('',#74901,0.0999999999999994) ;
#28544=CIRCLE('',#74903,0.0999999999999994) ;
#28545=CIRCLE('',#74905,0.0999999999999994) ;
#28546=CIRCLE('',#74907,0.0999999999999994) ;
#28547=CIRCLE('',#74909,0.1) ;
#28548=CIRCLE('',#74911,0.1) ;
#28549=CIRCLE('',#74913,0.1) ;
#28550=CIRCLE('',#74915,0.1) ;
#28551=CIRCLE('',#74917,0.1) ;
#28552=CIRCLE('',#74919,0.1) ;
#28553=CIRCLE('',#74921,0.0999999999999989) ;
#28554=CIRCLE('',#74923,0.1) ;
#28555=CIRCLE('',#74925,0.1) ;
#28556=CIRCLE('',#74927,0.1) ;
#28557=CIRCLE('',#74930,0.1) ;
#28558=CIRCLE('',#74932,0.0999999999999994) ;
#28559=CIRCLE('',#74934,0.0999999999999995) ;
#28560=CIRCLE('',#74936,0.0999999999999994) ;
#28561=CIRCLE('',#74938,0.1) ;
#28562=CIRCLE('',#74940,0.1) ;
#28563=CIRCLE('',#74942,0.1) ;
#28564=CIRCLE('',#74944,0.1) ;
#28565=CIRCLE('',#74946,0.0999999999999994) ;
#28566=CIRCLE('',#74948,0.0999999999999994) ;
#28567=CIRCLE('',#74951,0.0999999999999994) ;
#28568=CIRCLE('',#74952,0.0999999999999994) ;
#28569=CIRCLE('',#74954,0.0999999999999994) ;
#28570=CIRCLE('',#74955,0.1) ;
#28571=CIRCLE('',#74957,0.0999999999999994) ;
#28572=CIRCLE('',#74958,0.1) ;
#28573=CIRCLE('',#74960,0.1) ;
#28574=CIRCLE('',#74961,0.0999999999999998) ;
#28575=CIRCLE('',#74963,0.1) ;
#28576=CIRCLE('',#74965,0.1) ;
#28577=CIRCLE('',#74967,0.0999999999999994) ;
#28578=CIRCLE('',#74969,0.1) ;
#28579=CIRCLE('',#74971,0.0999999999999998) ;
#28580=CIRCLE('',#74973,0.1) ;
#28581=CIRCLE('',#74975,0.0999999999999994) ;
#28582=CIRCLE('',#74976,0.1) ;
#28583=CIRCLE('',#74979,0.1) ;
#28584=CIRCLE('',#74981,0.0999999999999994) ;
#28585=CIRCLE('',#74982,0.0999999999999994) ;
#28586=CIRCLE('',#74984,0.0999999999999994) ;
#28587=CIRCLE('',#74986,0.1) ;
#28588=CIRCLE('',#74988,0.0999999999999994) ;
#28589=CIRCLE('',#74990,0.0999999999999994) ;
#28590=CIRCLE('',#74992,0.0999999999999994) ;
#28591=CIRCLE('',#74994,0.1) ;
#28592=CIRCLE('',#74995,0.0999999999999994) ;
#28593=CIRCLE('',#74997,0.1) ;
#28594=CIRCLE('',#74999,0.0999999999999994) ;
#28595=CIRCLE('',#75001,0.0999999999999998) ;
#28596=CIRCLE('',#75002,0.1) ;
#28597=CIRCLE('',#75004,0.0999999999999994) ;
#28598=CIRCLE('',#75006,0.1) ;
#28599=CIRCLE('',#75007,0.1) ;
#28600=CIRCLE('',#75009,0.1) ;
#28601=CIRCLE('',#75011,0.1) ;
#28602=CIRCLE('',#75013,0.0999999999999994) ;
#28603=CIRCLE('',#75015,0.0999999999999994) ;
#28604=CIRCLE('',#75017,0.1) ;
#28605=CIRCLE('',#75019,0.1) ;
#28606=CIRCLE('',#75021,0.1) ;
#28607=CIRCLE('',#75023,0.0999999999999994) ;
#28608=CIRCLE('',#75024,0.0999999999999994) ;
#28609=CIRCLE('',#75026,0.1) ;
#28610=CIRCLE('',#75028,0.1) ;
#28611=CIRCLE('',#75030,0.1) ;
#28612=CIRCLE('',#75032,0.1) ;
#28613=CIRCLE('',#75033,0.0999999999999994) ;
#28614=CIRCLE('',#75035,0.0999999999999994) ;
#28615=CIRCLE('',#75037,0.0999999999999994) ;
#28616=CIRCLE('',#75039,0.1) ;
#28617=CIRCLE('',#75041,0.0999999999999994) ;
#28618=CIRCLE('',#75044,0.0999999999999994) ;
#28619=CIRCLE('',#75046,0.1) ;
#28620=CIRCLE('',#75048,0.0999999999999994) ;
#28621=CIRCLE('',#75051,0.1) ;
#28622=CIRCLE('',#75052,0.1) ;
#28623=CIRCLE('',#75054,0.0999999999999994) ;
#28624=CIRCLE('',#75056,0.0999999999999994) ;
#28625=CIRCLE('',#75058,0.0999999999999994) ;
#28626=CIRCLE('',#75060,0.0999999999999994) ;
#28627=CIRCLE('',#75062,0.1) ;
#28628=CIRCLE('',#75064,0.1) ;
#28629=CIRCLE('',#75066,0.1) ;
#28630=CIRCLE('',#75068,0.1) ;
#28631=CIRCLE('',#75070,0.1) ;
#28632=CIRCLE('',#75072,0.1) ;
#28633=CIRCLE('',#75074,0.0999999999999989) ;
#28634=CIRCLE('',#75076,0.1) ;
#28635=CIRCLE('',#75078,0.1) ;
#28636=CIRCLE('',#75080,0.1) ;
#28637=CIRCLE('',#75083,0.1) ;
#28638=CIRCLE('',#75085,0.0999999999999994) ;
#28639=CIRCLE('',#75087,0.0999999999999995) ;
#28640=CIRCLE('',#75089,0.0999999999999994) ;
#28641=CIRCLE('',#75091,0.1) ;
#28642=CIRCLE('',#75093,0.1) ;
#28643=CIRCLE('',#75095,0.1) ;
#28644=CIRCLE('',#75097,0.1) ;
#28645=CIRCLE('',#75099,0.0999999999999994) ;
#28646=CIRCLE('',#75101,0.0999999999999994) ;
#28647=CIRCLE('',#75104,0.0999999999999994) ;
#28648=CIRCLE('',#75105,0.0999999999999994) ;
#28649=CIRCLE('',#75107,0.0999999999999994) ;
#28650=CIRCLE('',#75108,0.1) ;
#28651=CIRCLE('',#75110,0.0999999999999994) ;
#28652=CIRCLE('',#75111,0.1) ;
#28653=CIRCLE('',#75113,0.1) ;
#28654=CIRCLE('',#75114,0.0999999999999998) ;
#28655=CIRCLE('',#75116,0.1) ;
#28656=CIRCLE('',#75118,0.1) ;
#28657=CIRCLE('',#75120,0.0999999999999994) ;
#28658=CIRCLE('',#75122,0.1) ;
#28659=CIRCLE('',#75124,0.0999999999999998) ;
#28660=CIRCLE('',#75126,0.1) ;
#28661=CIRCLE('',#75128,0.0999999999999994) ;
#28662=CIRCLE('',#75129,0.1) ;
#28663=CIRCLE('',#75132,0.1) ;
#28664=CIRCLE('',#75134,0.0999999999999994) ;
#28665=CIRCLE('',#75135,0.0999999999999994) ;
#28666=CIRCLE('',#75137,0.0999999999999994) ;
#28667=CIRCLE('',#75139,0.1) ;
#28668=CIRCLE('',#75141,0.0999999999999994) ;
#28669=CIRCLE('',#75143,0.0999999999999994) ;
#28670=CIRCLE('',#75145,0.0999999999999994) ;
#28671=CIRCLE('',#75147,0.1) ;
#28672=CIRCLE('',#75148,0.0999999999999994) ;
#28673=CIRCLE('',#75150,0.1) ;
#28674=CIRCLE('',#75152,0.0999999999999994) ;
#28675=CIRCLE('',#75154,0.0999999999999998) ;
#28676=CIRCLE('',#75155,0.1) ;
#28677=CIRCLE('',#75157,0.0999999999999994) ;
#28678=CIRCLE('',#75159,0.1) ;
#28679=CIRCLE('',#75160,0.1) ;
#28680=CIRCLE('',#75162,0.1) ;
#28681=CIRCLE('',#75164,0.1) ;
#28682=CIRCLE('',#75166,0.0999999999999994) ;
#28683=CIRCLE('',#75168,0.0999999999999994) ;
#28684=CIRCLE('',#75170,0.1) ;
#28685=CIRCLE('',#75172,0.1) ;
#28686=CIRCLE('',#75174,0.1) ;
#28687=CIRCLE('',#75176,0.100000000000003) ;
#28688=CIRCLE('',#75177,0.100000000000003) ;
#28689=CIRCLE('',#75179,0.1) ;
#28690=CIRCLE('',#75181,0.1) ;
#28691=CIRCLE('',#75183,0.1) ;
#28692=CIRCLE('',#75185,0.1) ;
#28693=CIRCLE('',#75186,0.100000000000003) ;
#28694=CIRCLE('',#75188,0.100000000000003) ;
#28695=CIRCLE('',#75190,0.100000000000003) ;
#28696=CIRCLE('',#75192,0.1) ;
#28697=CIRCLE('',#75194,0.100000000000003) ;
#28698=CIRCLE('',#75197,0.100000000000003) ;
#28699=CIRCLE('',#75199,0.1) ;
#28700=CIRCLE('',#75201,0.100000000000003) ;
#28701=CIRCLE('',#75204,0.1) ;
#28702=CIRCLE('',#75205,0.1) ;
#28703=CIRCLE('',#75207,0.0999999999999994) ;
#28704=CIRCLE('',#75209,0.100000000000003) ;
#28705=CIRCLE('',#75211,0.0999999999999994) ;
#28706=CIRCLE('',#75213,0.100000000000003) ;
#28707=CIRCLE('',#75215,0.1) ;
#28708=CIRCLE('',#75217,0.1) ;
#28709=CIRCLE('',#75219,0.1) ;
#28710=CIRCLE('',#75221,0.1) ;
#28711=CIRCLE('',#75223,0.0999999999999999) ;
#28712=CIRCLE('',#75225,0.1) ;
#28713=CIRCLE('',#75227,0.0999999999999992) ;
#28714=CIRCLE('',#75229,0.1) ;
#28715=CIRCLE('',#75231,0.1) ;
#28716=CIRCLE('',#75233,0.1) ;
#28717=CIRCLE('',#75236,0.1) ;
#28718=CIRCLE('',#75238,0.0999999999999994) ;
#28719=CIRCLE('',#75240,0.0999999999999995) ;
#28720=CIRCLE('',#75242,0.0999999999999994) ;
#28721=CIRCLE('',#75244,0.1) ;
#28722=CIRCLE('',#75246,0.1) ;
#28723=CIRCLE('',#75248,0.1) ;
#28724=CIRCLE('',#75250,0.1) ;
#28725=CIRCLE('',#75252,0.0999999999999994) ;
#28726=CIRCLE('',#75254,0.0999999999999994) ;
#28727=CIRCLE('',#75257,0.100000000000003) ;
#28728=CIRCLE('',#75258,0.100000000000003) ;
#28729=CIRCLE('',#75260,0.100000000000003) ;
#28730=CIRCLE('',#75261,0.1) ;
#28731=CIRCLE('',#75263,0.100000000000003) ;
#28732=CIRCLE('',#75264,0.1) ;
#28733=CIRCLE('',#75266,0.1) ;
#28734=CIRCLE('',#75267,0.0999999999999998) ;
#28735=CIRCLE('',#75269,0.1) ;
#28736=CIRCLE('',#75271,0.1) ;
#28737=CIRCLE('',#75273,0.100000000000003) ;
#28738=CIRCLE('',#75275,0.1) ;
#28739=CIRCLE('',#75277,0.0999999999999998) ;
#28740=CIRCLE('',#75279,0.1) ;
#28741=CIRCLE('',#75281,0.100000000000003) ;
#28742=CIRCLE('',#75282,0.1) ;
#28743=CIRCLE('',#75285,0.1) ;
#28744=CIRCLE('',#75287,0.100000000000003) ;
#28745=CIRCLE('',#75288,0.100000000000003) ;
#28746=CIRCLE('',#75290,0.100000000000003) ;
#28747=CIRCLE('',#75292,0.1) ;
#28748=CIRCLE('',#75294,0.100000000000003) ;
#28749=CIRCLE('',#75296,0.100000000000003) ;
#28750=CIRCLE('',#75298,0.100000000000003) ;
#28751=CIRCLE('',#75300,0.1) ;
#28752=CIRCLE('',#75301,0.100000000000003) ;
#28753=CIRCLE('',#75303,0.1) ;
#28754=CIRCLE('',#75305,0.100000000000003) ;
#28755=CIRCLE('',#75307,0.0999999999999998) ;
#28756=CIRCLE('',#75308,0.1) ;
#28757=CIRCLE('',#75310,0.100000000000003) ;
#28758=CIRCLE('',#75312,0.1) ;
#28759=CIRCLE('',#75313,0.1) ;
#28760=CIRCLE('',#75315,0.1) ;
#28761=CIRCLE('',#75317,0.1) ;
#28762=CIRCLE('',#75319,0.100000000000003) ;
#28763=CIRCLE('',#75321,0.100000000000003) ;
#28764=CIRCLE('',#75323,0.1) ;
#28765=CIRCLE('',#75325,0.1) ;
#28766=CIRCLE('',#75327,0.1) ;
#28767=CIRCLE('',#75329,0.100000000000003) ;
#28768=CIRCLE('',#75330,0.100000000000003) ;
#28769=CIRCLE('',#75332,0.1) ;
#28770=CIRCLE('',#75334,0.1) ;
#28771=CIRCLE('',#75336,0.1) ;
#28772=CIRCLE('',#75338,0.1) ;
#28773=CIRCLE('',#75339,0.100000000000003) ;
#28774=CIRCLE('',#75341,0.100000000000003) ;
#28775=CIRCLE('',#75343,0.100000000000003) ;
#28776=CIRCLE('',#75345,0.1) ;
#28777=CIRCLE('',#75347,0.100000000000003) ;
#28778=CIRCLE('',#75350,0.100000000000003) ;
#28779=CIRCLE('',#75352,0.1) ;
#28780=CIRCLE('',#75354,0.100000000000003) ;
#28781=CIRCLE('',#75357,0.1) ;
#28782=CIRCLE('',#75358,0.1) ;
#28783=CIRCLE('',#75360,0.100000000000003) ;
#28784=CIRCLE('',#75362,0.100000000000003) ;
#28785=CIRCLE('',#75364,0.100000000000003) ;
#28786=CIRCLE('',#75366,0.100000000000003) ;
#28787=CIRCLE('',#75368,0.1) ;
#28788=CIRCLE('',#75370,0.1) ;
#28789=CIRCLE('',#75372,0.1) ;
#28790=CIRCLE('',#75374,0.1) ;
#28791=CIRCLE('',#75376,0.0999999999999999) ;
#28792=CIRCLE('',#75378,0.1) ;
#28793=CIRCLE('',#75380,0.0999999999999992) ;
#28794=CIRCLE('',#75382,0.1) ;
#28795=CIRCLE('',#75384,0.1) ;
#28796=CIRCLE('',#75386,0.1) ;
#28797=CIRCLE('',#75389,0.1) ;
#28798=CIRCLE('',#75391,0.100000000000003) ;
#28799=CIRCLE('',#75393,0.0999999999999998) ;
#28800=CIRCLE('',#75395,0.100000000000003) ;
#28801=CIRCLE('',#75397,0.1) ;
#28802=CIRCLE('',#75399,0.1) ;
#28803=CIRCLE('',#75401,0.1) ;
#28804=CIRCLE('',#75403,0.1) ;
#28805=CIRCLE('',#75405,0.100000000000003) ;
#28806=CIRCLE('',#75407,0.100000000000003) ;
#28807=CIRCLE('',#75415,0.3) ;
#28808=CIRCLE('',#75416,0.9) ;
#28809=CIRCLE('',#75418,0.9) ;
#28810=CIRCLE('',#75419,0.3) ;
#28811=CIRCLE('',#75421,1.) ;
#28812=CIRCLE('',#75422,1.) ;
#28813=CIRCLE('',#75424,0.2) ;
#28814=CIRCLE('',#75425,0.2) ;
#28815=CIRCLE('',#75439,0.3) ;
#28816=CIRCLE('',#75440,0.9) ;
#28817=CIRCLE('',#75442,0.9) ;
#28818=CIRCLE('',#75443,0.3) ;
#28819=CIRCLE('',#75445,1.) ;
#28820=CIRCLE('',#75446,1.) ;
#28821=CIRCLE('',#75448,0.2) ;
#28822=CIRCLE('',#75449,0.2) ;
#28823=CIRCLE('',#75463,0.3) ;
#28824=CIRCLE('',#75464,0.9) ;
#28825=CIRCLE('',#75466,0.9) ;
#28826=CIRCLE('',#75467,0.3) ;
#28827=CIRCLE('',#75469,1.) ;
#28828=CIRCLE('',#75470,1.) ;
#28829=CIRCLE('',#75472,0.2) ;
#28830=CIRCLE('',#75473,0.2) ;
#28831=CIRCLE('',#75487,0.3) ;
#28832=CIRCLE('',#75488,0.9) ;
#28833=CIRCLE('',#75490,0.9) ;
#28834=CIRCLE('',#75491,0.3) ;
#28835=CIRCLE('',#75493,1.) ;
#28836=CIRCLE('',#75494,1.) ;
#28837=CIRCLE('',#75496,0.2) ;
#28838=CIRCLE('',#75497,0.2) ;
#28839=CIRCLE('',#75511,0.3) ;
#28840=CIRCLE('',#75512,0.9) ;
#28841=CIRCLE('',#75514,0.9) ;
#28842=CIRCLE('',#75515,0.3) ;
#28843=CIRCLE('',#75517,1.) ;
#28844=CIRCLE('',#75518,1.) ;
#28845=CIRCLE('',#75520,0.2) ;
#28846=CIRCLE('',#75521,0.2) ;
#28847=CIRCLE('',#75535,0.3) ;
#28848=CIRCLE('',#75536,0.9) ;
#28849=CIRCLE('',#75538,0.9) ;
#28850=CIRCLE('',#75539,0.3) ;
#28851=CIRCLE('',#75541,1.) ;
#28852=CIRCLE('',#75542,1.) ;
#28853=CIRCLE('',#75544,0.2) ;
#28854=CIRCLE('',#75545,0.2) ;
#28855=CIRCLE('',#75559,0.3) ;
#28856=CIRCLE('',#75560,0.9) ;
#28857=CIRCLE('',#75562,0.9) ;
#28858=CIRCLE('',#75563,0.3) ;
#28859=CIRCLE('',#75565,1.) ;
#28860=CIRCLE('',#75566,1.) ;
#28861=CIRCLE('',#75568,0.2) ;
#28862=CIRCLE('',#75569,0.2) ;
#28863=CIRCLE('',#75583,0.3) ;
#28864=CIRCLE('',#75584,0.9) ;
#28865=CIRCLE('',#75586,0.9) ;
#28866=CIRCLE('',#75587,0.3) ;
#28867=CIRCLE('',#75589,1.) ;
#28868=CIRCLE('',#75590,1.) ;
#28869=CIRCLE('',#75592,0.2) ;
#28870=CIRCLE('',#75593,0.2) ;
#28871=CIRCLE('',#75607,0.3) ;
#28872=CIRCLE('',#75608,0.9) ;
#28873=CIRCLE('',#75610,0.9) ;
#28874=CIRCLE('',#75611,0.3) ;
#28875=CIRCLE('',#75613,1.) ;
#28876=CIRCLE('',#75614,1.) ;
#28877=CIRCLE('',#75616,0.2) ;
#28878=CIRCLE('',#75617,0.2) ;
#28879=CIRCLE('',#75662,0.1) ;
#28880=CIRCLE('',#75663,0.0999999999999998) ;
#28881=CIRCLE('',#75665,0.1) ;
#28882=CIRCLE('',#75666,0.1) ;
#28883=CIRCLE('',#75668,0.0999999999999998) ;
#28884=CIRCLE('',#75669,0.1) ;
#28885=CIRCLE('',#75671,0.0999999999999999) ;
#28886=CIRCLE('',#75672,0.1) ;
#28887=CIRCLE('',#75674,0.1) ;
#28888=CIRCLE('',#75676,0.0999999999999998) ;
#28889=CIRCLE('',#75678,0.0999999999999998) ;
#28890=CIRCLE('',#75680,0.0999999999999999) ;
#28891=CIRCLE('',#75681,0.1) ;
#28892=CIRCLE('',#75683,0.0999999999999998) ;
#28893=CIRCLE('',#75685,0.1) ;
#28894=CIRCLE('',#75687,0.1) ;
#28895=CIRCLE('',#75689,0.0999999999999999) ;
#28896=CIRCLE('',#75691,0.1) ;
#28897=CIRCLE('',#75692,0.1) ;
#28898=CIRCLE('',#75694,0.1) ;
#28899=CIRCLE('',#75696,0.1) ;
#28900=CIRCLE('',#75697,0.0999999999999998) ;
#28901=CIRCLE('',#75699,0.1) ;
#28902=CIRCLE('',#75700,0.1) ;
#28903=CIRCLE('',#75702,0.0999999999999998) ;
#28904=CIRCLE('',#75703,0.1) ;
#28905=CIRCLE('',#75705,0.1) ;
#28906=CIRCLE('',#75706,0.1) ;
#28907=CIRCLE('',#75708,0.1) ;
#28908=CIRCLE('',#75710,0.1) ;
#28909=CIRCLE('',#75712,0.0999999999999998) ;
#28910=CIRCLE('',#75714,0.1) ;
#28911=CIRCLE('',#75715,0.1) ;
#28912=CIRCLE('',#75717,0.0999999999999998) ;
#28913=CIRCLE('',#75719,0.1) ;
#28914=CIRCLE('',#75721,0.1) ;
#28915=CIRCLE('',#75723,0.1) ;
#28916=CIRCLE('',#75725,0.1) ;
#28917=CIRCLE('',#75726,0.1) ;
#28918=CIRCLE('',#75728,0.1) ;
#28919=CIRCLE('',#75730,0.0999999999999997) ;
#28920=CIRCLE('',#75731,0.0999999999999999) ;
#28921=CIRCLE('',#75733,0.1) ;
#28922=CIRCLE('',#75734,0.1) ;
#28923=CIRCLE('',#75736,0.1) ;
#28924=CIRCLE('',#75737,0.1) ;
#28925=CIRCLE('',#75739,0.1) ;
#28926=CIRCLE('',#75740,0.1) ;
#28927=CIRCLE('',#75742,0.1) ;
#28928=CIRCLE('',#75744,0.1) ;
#28929=CIRCLE('',#75746,0.1) ;
#28930=CIRCLE('',#75748,0.1) ;
#28931=CIRCLE('',#75749,0.1) ;
#28932=CIRCLE('',#75751,0.1) ;
#28933=CIRCLE('',#75753,0.1) ;
#28934=CIRCLE('',#75755,0.1) ;
#28935=CIRCLE('',#75757,0.1) ;
#28936=CIRCLE('',#75759,0.1) ;
#28937=CIRCLE('',#75760,0.1) ;
#28938=CIRCLE('',#75762,0.1) ;
#28939=CIRCLE('',#75764,0.0999999999999999) ;
#28940=CIRCLE('',#75765,0.1) ;
#28941=CIRCLE('',#75767,0.1) ;
#28942=CIRCLE('',#75768,0.1) ;
#28943=CIRCLE('',#75770,0.1) ;
#28944=CIRCLE('',#75771,0.1) ;
#28945=CIRCLE('',#75773,0.1) ;
#28946=CIRCLE('',#75774,0.1) ;
#28947=CIRCLE('',#75776,0.1) ;
#28948=CIRCLE('',#75778,0.1) ;
#28949=CIRCLE('',#75780,0.1) ;
#28950=CIRCLE('',#75782,0.0999999999999999) ;
#28951=CIRCLE('',#75783,0.1) ;
#28952=CIRCLE('',#75785,0.1) ;
#28953=CIRCLE('',#75787,0.1) ;
#28954=CIRCLE('',#75789,0.1) ;
#28955=CIRCLE('',#75791,0.1) ;
#28956=CIRCLE('',#75793,0.1) ;
#28957=CIRCLE('',#75794,0.1) ;
#28958=CIRCLE('',#75796,0.0999999999999997) ;
#28959=CIRCLE('',#75798,0.0999999999999999) ;
#28960=CIRCLE('',#75799,0.1) ;
#28961=CIRCLE('',#75801,0.1) ;
#28962=CIRCLE('',#75802,0.1) ;
#28963=CIRCLE('',#75804,0.0999999999999994) ;
#28964=CIRCLE('',#75805,0.1) ;
#28965=CIRCLE('',#75807,0.1) ;
#28966=CIRCLE('',#75808,0.1) ;
#28967=CIRCLE('',#75810,0.1) ;
#28968=CIRCLE('',#75812,0.0999999999999994) ;
#28969=CIRCLE('',#75814,0.0999999999999994) ;
#28970=CIRCLE('',#75816,0.1) ;
#28971=CIRCLE('',#75817,0.1) ;
#28972=CIRCLE('',#75819,0.0999999999999994) ;
#28973=CIRCLE('',#75821,0.1) ;
#28974=CIRCLE('',#75823,0.1) ;
#28975=CIRCLE('',#75825,0.0999999999999998) ;
#28976=CIRCLE('',#75827,0.1) ;
#28977=CIRCLE('',#75828,0.1) ;
#28978=CIRCLE('',#75830,0.1) ;
#28979=CIRCLE('',#75832,0.1) ;
#28980=CIRCLE('',#75833,0.1) ;
#28981=CIRCLE('',#75835,0.1) ;
#28982=CIRCLE('',#75836,0.1) ;
#28983=CIRCLE('',#75838,0.0999999999999994) ;
#28984=CIRCLE('',#75839,0.1) ;
#28985=CIRCLE('',#75841,0.1) ;
#28986=CIRCLE('',#75842,0.1) ;
#28987=CIRCLE('',#75844,0.1) ;
#28988=CIRCLE('',#75846,0.1) ;
#28989=CIRCLE('',#75848,0.0999999999999994) ;
#28990=CIRCLE('',#75850,0.1) ;
#28991=CIRCLE('',#75851,0.1) ;
#28992=CIRCLE('',#75853,0.0999999999999994) ;
#28993=CIRCLE('',#75855,0.1) ;
#28994=CIRCLE('',#75857,0.1) ;
#28995=CIRCLE('',#75859,0.1) ;
#28996=CIRCLE('',#75861,0.1) ;
#28997=CIRCLE('',#75862,0.1) ;
#28998=CIRCLE('',#75864,0.100000000000001) ;
#28999=CIRCLE('',#75866,0.0999999999999999) ;
#29000=CIRCLE('',#75867,0.0999999999999999) ;
#29001=CIRCLE('',#75869,0.1) ;
#29002=CIRCLE('',#75870,0.1) ;
#29003=CIRCLE('',#75872,0.0999999999999994) ;
#29004=CIRCLE('',#75873,0.1) ;
#29005=CIRCLE('',#75875,0.1) ;
#29006=CIRCLE('',#75876,0.1) ;
#29007=CIRCLE('',#75878,0.1) ;
#29008=CIRCLE('',#75880,0.0999999999999994) ;
#29009=CIRCLE('',#75882,0.0999999999999994) ;
#29010=CIRCLE('',#75884,0.1) ;
#29011=CIRCLE('',#75885,0.1) ;
#29012=CIRCLE('',#75887,0.0999999999999994) ;
#29013=CIRCLE('',#75889,0.1) ;
#29014=CIRCLE('',#75891,0.1) ;
#29015=CIRCLE('',#75893,0.0999999999999999) ;
#29016=CIRCLE('',#75895,0.1) ;
#29017=CIRCLE('',#75896,0.1) ;
#29018=CIRCLE('',#75898,0.0999999999999998) ;
#29019=CIRCLE('',#75900,0.0999999999999999) ;
#29020=CIRCLE('',#75901,0.0999999999999998) ;
#29021=CIRCLE('',#75903,0.1) ;
#29022=CIRCLE('',#75904,0.1) ;
#29023=CIRCLE('',#75906,0.0999999999999994) ;
#29024=CIRCLE('',#75907,0.1) ;
#29025=CIRCLE('',#75909,0.1) ;
#29026=CIRCLE('',#75910,0.1) ;
#29027=CIRCLE('',#75912,0.1) ;
#29028=CIRCLE('',#75914,0.1) ;
#29029=CIRCLE('',#75916,0.0999999999999994) ;
#29030=CIRCLE('',#75918,0.1) ;
#29031=CIRCLE('',#75919,0.1) ;
#29032=CIRCLE('',#75921,0.0999999999999994) ;
#29033=CIRCLE('',#75923,0.1) ;
#29034=CIRCLE('',#75925,0.1) ;
#29035=CIRCLE('',#75927,0.0999999999999995) ;
#29036=CIRCLE('',#75929,0.1) ;
#29037=CIRCLE('',#75930,0.1) ;
#29038=CIRCLE('',#75932,0.1) ;
#29039=CIRCLE('',#75934,0.1) ;
#29040=CIRCLE('',#75935,0.0999999999999999) ;
#29041=CIRCLE('',#75937,0.1) ;
#29042=CIRCLE('',#75938,0.1) ;
#29043=CIRCLE('',#75940,0.0999999999999994) ;
#29044=CIRCLE('',#75941,0.1) ;
#29045=CIRCLE('',#75943,0.099999999999999) ;
#29046=CIRCLE('',#75944,0.1) ;
#29047=CIRCLE('',#75946,0.1) ;
#29048=CIRCLE('',#75948,0.0999999999999994) ;
#29049=CIRCLE('',#75950,0.0999999999999994) ;
#29050=CIRCLE('',#75952,0.0999999999999999) ;
#29051=CIRCLE('',#75953,0.1) ;
#29052=CIRCLE('',#75955,0.0999999999999994) ;
#29053=CIRCLE('',#75957,0.1) ;
#29054=CIRCLE('',#75959,0.099999999999999) ;
#29055=CIRCLE('',#75961,0.1) ;
#29056=CIRCLE('',#75963,0.1) ;
#29057=CIRCLE('',#75964,0.1) ;
#29058=CIRCLE('',#75966,0.0999999999999995) ;
#29059=CIRCLE('',#75968,0.0999999999999991) ;
#29060=CIRCLE('',#75969,0.0999999999999995) ;
#29061=CIRCLE('',#75971,0.1) ;
#29062=CIRCLE('',#75972,0.1) ;
#29063=CIRCLE('',#75974,0.0999999999999994) ;
#29064=CIRCLE('',#75975,0.1) ;
#29065=CIRCLE('',#75977,0.0999999999999989) ;
#29066=CIRCLE('',#75978,0.099999999999999) ;
#29067=CIRCLE('',#75980,0.1) ;
#29068=CIRCLE('',#75982,0.0999999999999994) ;
#29069=CIRCLE('',#75984,0.0999999999999994) ;
#29070=CIRCLE('',#75986,0.1) ;
#29071=CIRCLE('',#75987,0.1) ;
#29072=CIRCLE('',#75989,0.0999999999999994) ;
#29073=CIRCLE('',#75991,0.1) ;
#29074=CIRCLE('',#75993,0.0999999999999989) ;
#29075=CIRCLE('',#75995,0.0999999999999999) ;
#29076=CIRCLE('',#75997,0.1) ;
#29077=CIRCLE('',#75998,0.1) ;
#29078=CIRCLE('',#76000,0.0999999999999989) ;
#29079=CIRCLE('',#76002,0.1) ;
#29080=CIRCLE('',#76003,0.0999999999999999) ;
#29081=CIRCLE('',#76005,0.1) ;
#29082=CIRCLE('',#76006,0.1) ;
#29083=CIRCLE('',#76008,0.0999999999999994) ;
#29084=CIRCLE('',#76009,0.1) ;
#29085=CIRCLE('',#76011,0.099999999999999) ;
#29086=CIRCLE('',#76012,0.1) ;
#29087=CIRCLE('',#76014,0.1) ;
#29088=CIRCLE('',#76016,0.0999999999999994) ;
#29089=CIRCLE('',#76018,0.0999999999999994) ;
#29090=CIRCLE('',#76020,0.0999999999999999) ;
#29091=CIRCLE('',#76021,0.1) ;
#29092=CIRCLE('',#76023,0.0999999999999994) ;
#29093=CIRCLE('',#76025,0.1) ;
#29094=CIRCLE('',#76027,0.099999999999999) ;
#29095=CIRCLE('',#76029,0.1) ;
#29096=CIRCLE('',#76031,0.1) ;
#29097=CIRCLE('',#76032,0.1) ;
#29098=CIRCLE('',#76034,0.0999999999999995) ;
#29099=CIRCLE('',#76036,0.0999999999999991) ;
#29100=CIRCLE('',#76037,0.0999999999999995) ;
#29101=CIRCLE('',#76039,0.1) ;
#29102=CIRCLE('',#76040,0.1) ;
#29103=CIRCLE('',#76042,0.0999999999999994) ;
#29104=CIRCLE('',#76043,0.1) ;
#29105=CIRCLE('',#76045,0.0999999999999989) ;
#29106=CIRCLE('',#76046,0.099999999999999) ;
#29107=CIRCLE('',#76048,0.1) ;
#29108=CIRCLE('',#76050,0.0999999999999994) ;
#29109=CIRCLE('',#76052,0.0999999999999994) ;
#29110=CIRCLE('',#76054,0.1) ;
#29111=CIRCLE('',#76055,0.1) ;
#29112=CIRCLE('',#76057,0.0999999999999994) ;
#29113=CIRCLE('',#76059,0.1) ;
#29114=CIRCLE('',#76061,0.0999999999999989) ;
#29115=CIRCLE('',#76063,0.0999999999999999) ;
#29116=CIRCLE('',#76065,0.1) ;
#29117=CIRCLE('',#76066,0.1) ;
#29118=CIRCLE('',#76068,0.0999999999999989) ;
#29119=CIRCLE('',#76070,0.1) ;
#29120=CIRCLE('',#76071,0.0999999999999999) ;
#29121=CIRCLE('',#76073,0.1) ;
#29122=CIRCLE('',#76074,0.1) ;
#29123=CIRCLE('',#76076,0.0999999999999994) ;
#29124=CIRCLE('',#76077,0.1) ;
#29125=CIRCLE('',#76079,0.099999999999999) ;
#29126=CIRCLE('',#76080,0.1) ;
#29127=CIRCLE('',#76082,0.1) ;
#29128=CIRCLE('',#76084,0.0999999999999994) ;
#29129=CIRCLE('',#76086,0.0999999999999994) ;
#29130=CIRCLE('',#76088,0.0999999999999999) ;
#29131=CIRCLE('',#76089,0.1) ;
#29132=CIRCLE('',#76091,0.0999999999999994) ;
#29133=CIRCLE('',#76093,0.1) ;
#29134=CIRCLE('',#76095,0.099999999999999) ;
#29135=CIRCLE('',#76097,0.1) ;
#29136=CIRCLE('',#76099,0.1) ;
#29137=CIRCLE('',#76100,0.1) ;
#29138=CIRCLE('',#76102,0.0999999999999995) ;
#29139=CIRCLE('',#76104,0.0999999999999991) ;
#29140=CIRCLE('',#76105,0.0999999999999995) ;
#29141=CIRCLE('',#76107,0.1) ;
#29142=CIRCLE('',#76108,0.1) ;
#29143=CIRCLE('',#76110,0.0999999999999994) ;
#29144=CIRCLE('',#76111,0.1) ;
#29145=CIRCLE('',#76113,0.0999999999999989) ;
#29146=CIRCLE('',#76114,0.099999999999999) ;
#29147=CIRCLE('',#76116,0.1) ;
#29148=CIRCLE('',#76118,0.0999999999999994) ;
#29149=CIRCLE('',#76120,0.0999999999999994) ;
#29150=CIRCLE('',#76122,0.1) ;
#29151=CIRCLE('',#76123,0.1) ;
#29152=CIRCLE('',#76125,0.0999999999999994) ;
#29153=CIRCLE('',#76127,0.1) ;
#29154=CIRCLE('',#76129,0.0999999999999989) ;
#29155=CIRCLE('',#76131,0.0999999999999999) ;
#29156=CIRCLE('',#76133,0.1) ;
#29157=CIRCLE('',#76134,0.1) ;
#29158=CIRCLE('',#76136,0.0999999999999989) ;
#29159=CIRCLE('',#76138,0.1) ;
#29160=CIRCLE('',#76139,0.0999999999999999) ;
#29161=CIRCLE('',#76141,0.1) ;
#29162=CIRCLE('',#76142,0.1) ;
#29163=CIRCLE('',#76144,0.0999999999999994) ;
#29164=CIRCLE('',#76145,0.1) ;
#29165=CIRCLE('',#76147,0.099999999999999) ;
#29166=CIRCLE('',#76148,0.1) ;
#29167=CIRCLE('',#76150,0.1) ;
#29168=CIRCLE('',#76152,0.0999999999999994) ;
#29169=CIRCLE('',#76154,0.0999999999999994) ;
#29170=CIRCLE('',#76156,0.0999999999999999) ;
#29171=CIRCLE('',#76157,0.1) ;
#29172=CIRCLE('',#76159,0.0999999999999994) ;
#29173=CIRCLE('',#76161,0.1) ;
#29174=CIRCLE('',#76163,0.099999999999999) ;
#29175=CIRCLE('',#76165,0.1) ;
#29176=CIRCLE('',#76167,0.1) ;
#29177=CIRCLE('',#76168,0.1) ;
#29178=CIRCLE('',#76170,0.0999999999999995) ;
#29179=CIRCLE('',#76172,0.0999999999999991) ;
#29180=CIRCLE('',#76173,0.0999999999999995) ;
#29181=CIRCLE('',#76175,0.1) ;
#29182=CIRCLE('',#76176,0.1) ;
#29183=CIRCLE('',#76178,0.0999999999999994) ;
#29184=CIRCLE('',#76179,0.1) ;
#29185=CIRCLE('',#76181,0.0999999999999989) ;
#29186=CIRCLE('',#76182,0.099999999999999) ;
#29187=CIRCLE('',#76184,0.1) ;
#29188=CIRCLE('',#76186,0.0999999999999994) ;
#29189=CIRCLE('',#76188,0.0999999999999994) ;
#29190=CIRCLE('',#76190,0.1) ;
#29191=CIRCLE('',#76191,0.1) ;
#29192=CIRCLE('',#76193,0.0999999999999994) ;
#29193=CIRCLE('',#76195,0.1) ;
#29194=CIRCLE('',#76197,0.0999999999999989) ;
#29195=CIRCLE('',#76199,0.0999999999999999) ;
#29196=CIRCLE('',#76201,0.1) ;
#29197=CIRCLE('',#76202,0.1) ;
#29198=CIRCLE('',#76204,0.0999999999999989) ;
#29199=CIRCLE('',#76206,0.0999999999999997) ;
#29200=CIRCLE('',#76207,0.0999999999999995) ;
#29201=CIRCLE('',#76209,0.1) ;
#29202=CIRCLE('',#76210,0.1) ;
#29203=CIRCLE('',#76212,0.100000000000003) ;
#29204=CIRCLE('',#76213,0.1) ;
#29205=CIRCLE('',#76215,0.099999999999999) ;
#29206=CIRCLE('',#76216,0.100000000000001) ;
#29207=CIRCLE('',#76218,0.1) ;
#29208=CIRCLE('',#76220,0.100000000000003) ;
#29209=CIRCLE('',#76222,0.100000000000003) ;
#29210=CIRCLE('',#76224,0.0999999999999995) ;
#29211=CIRCLE('',#76225,0.1) ;
#29212=CIRCLE('',#76227,0.100000000000003) ;
#29213=CIRCLE('',#76229,0.1) ;
#29214=CIRCLE('',#76231,0.099999999999999) ;
#29215=CIRCLE('',#76233,0.1) ;
#29216=CIRCLE('',#76235,0.1) ;
#29217=CIRCLE('',#76236,0.1) ;
#29218=CIRCLE('',#76238,0.0999999999999999) ;
#29219=CIRCLE('',#76240,0.1) ;
#29220=CIRCLE('',#76241,0.0999999999999983) ;
#29221=CIRCLE('',#76243,0.1) ;
#29222=CIRCLE('',#76244,0.1) ;
#29223=CIRCLE('',#76246,0.100000000000003) ;
#29224=CIRCLE('',#76247,0.1) ;
#29225=CIRCLE('',#76249,0.0999999999999989) ;
#29226=CIRCLE('',#76250,0.0999999999999998) ;
#29227=CIRCLE('',#76252,0.1) ;
#29228=CIRCLE('',#76254,0.1) ;
#29229=CIRCLE('',#76256,0.100000000000003) ;
#29230=CIRCLE('',#76258,0.0999999999999998) ;
#29231=CIRCLE('',#76259,0.1) ;
#29232=CIRCLE('',#76261,0.100000000000003) ;
#29233=CIRCLE('',#76263,0.1) ;
#29234=CIRCLE('',#76265,0.0999999999999989) ;
#29235=CIRCLE('',#76267,0.1) ;
#29236=CIRCLE('',#76269,0.1) ;
#29237=CIRCLE('',#76270,0.1) ;
#29238=CIRCLE('',#76272,0.100000000000001) ;
#29239=CIRCLE('',#76274,0.1) ;
#29240=CIRCLE('',#76276,0.1) ;
#29241=CIRCLE('',#76278,0.1) ;
#29242=CIRCLE('',#76280,0.1) ;
#29243=CIRCLE('',#76282,0.1) ;
#29244=CIRCLE('',#76284,0.1) ;
#29245=CIRCLE('',#76287,0.0999999999999998) ;
#29246=CIRCLE('',#76289,0.0999999999999998) ;
#29247=CIRCLE('',#76291,0.1) ;
#29248=CIRCLE('',#76293,0.0999999999999998) ;
#29249=CIRCLE('',#76295,0.0999999999999998) ;
#29250=CIRCLE('',#76297,0.0999999999999998) ;
#29251=CIRCLE('',#76300,0.1) ;
#29252=CIRCLE('',#76302,0.1) ;
#29253=CIRCLE('',#76304,0.1) ;
#29254=CIRCLE('',#76306,0.1) ;
#29255=CIRCLE('',#76309,0.0999999999999998) ;
#29256=CIRCLE('',#76311,0.1) ;
#29257=CIRCLE('',#76313,0.0999999999999998) ;
#29258=CIRCLE('',#76315,0.0999999999999998) ;
#29259=CIRCLE('',#76318,0.0999999999999994) ;
#29260=CIRCLE('',#76320,0.0999999999999994) ;
#29261=CIRCLE('',#76322,0.1) ;
#29262=CIRCLE('',#76324,0.0999999999999994) ;
#29263=CIRCLE('',#76326,0.0999999999999994) ;
#29264=CIRCLE('',#76328,0.0999999999999994) ;
#29265=CIRCLE('',#76331,0.1) ;
#29266=CIRCLE('',#76333,0.1) ;
#29267=CIRCLE('',#76335,0.1) ;
#29268=CIRCLE('',#76337,0.1) ;
#29269=CIRCLE('',#76339,0.1) ;
#29270=CIRCLE('',#76341,0.1) ;
#29271=CIRCLE('',#76344,0.0999999999999994) ;
#29272=CIRCLE('',#76346,0.1) ;
#29273=CIRCLE('',#76348,0.0999999999999994) ;
#29274=CIRCLE('',#76350,0.0999999999999994) ;
#29275=CIRCLE('',#76353,0.1) ;
#29276=CIRCLE('',#76355,0.1) ;
#29277=CIRCLE('',#76357,0.1) ;
#29278=CIRCLE('',#76359,0.1) ;
#29279=CIRCLE('',#76362,0.0999999999999994) ;
#29280=CIRCLE('',#76364,0.0999999999999994) ;
#29281=CIRCLE('',#76366,0.1) ;
#29282=CIRCLE('',#76368,0.0999999999999994) ;
#29283=CIRCLE('',#76370,0.0999999999999994) ;
#29284=CIRCLE('',#76372,0.0999999999999994) ;
#29285=CIRCLE('',#76375,0.0999999999999994) ;
#29286=CIRCLE('',#76377,0.0999999999999994) ;
#29287=CIRCLE('',#76379,0.1) ;
#29288=CIRCLE('',#76381,0.0999999999999994) ;
#29289=CIRCLE('',#76383,0.0999999999999994) ;
#29290=CIRCLE('',#76385,0.0999999999999994) ;
#29291=CIRCLE('',#76388,0.0999999999999994) ;
#29292=CIRCLE('',#76390,0.1) ;
#29293=CIRCLE('',#76392,0.0999999999999994) ;
#29294=CIRCLE('',#76394,0.0999999999999994) ;
#29295=CIRCLE('',#76397,0.0999999999999994) ;
#29296=CIRCLE('',#76399,0.1) ;
#29297=CIRCLE('',#76401,0.0999999999999994) ;
#29298=CIRCLE('',#76403,0.0999999999999994) ;
#29299=CIRCLE('',#76406,0.0999999999999994) ;
#29300=CIRCLE('',#76408,0.0999999999999994) ;
#29301=CIRCLE('',#76410,0.0999999999999994) ;
#29302=CIRCLE('',#76412,0.0999999999999994) ;
#29303=CIRCLE('',#76414,0.0999999999999994) ;
#29304=CIRCLE('',#76416,0.0999999999999994) ;
#29305=CIRCLE('',#76419,0.0999999999999994) ;
#29306=CIRCLE('',#76421,0.0999999999999994) ;
#29307=CIRCLE('',#76423,0.1) ;
#29308=CIRCLE('',#76425,0.0999999999999994) ;
#29309=CIRCLE('',#76427,0.0999999999999994) ;
#29310=CIRCLE('',#76429,0.0999999999999994) ;
#29311=CIRCLE('',#76432,0.100000000000001) ;
#29312=CIRCLE('',#76434,0.1) ;
#29313=CIRCLE('',#76436,0.100000000000001) ;
#29314=CIRCLE('',#76438,0.0999999999999994) ;
#29315=CIRCLE('',#76441,0.0999999999999994) ;
#29316=CIRCLE('',#76443,0.1) ;
#29317=CIRCLE('',#76445,0.0999999999999994) ;
#29318=CIRCLE('',#76447,0.0999999999999994) ;
#29319=CIRCLE('',#76450,0.0999999999999994) ;
#29320=CIRCLE('',#76452,0.0999999999999994) ;
#29321=CIRCLE('',#76454,0.1) ;
#29322=CIRCLE('',#76456,0.0999999999999994) ;
#29323=CIRCLE('',#76458,0.0999999999999994) ;
#29324=CIRCLE('',#76460,0.0999999999999994) ;
#29325=CIRCLE('',#76463,0.0999999999999994) ;
#29326=CIRCLE('',#76465,0.0999999999999994) ;
#29327=CIRCLE('',#76467,0.1) ;
#29328=CIRCLE('',#76469,0.0999999999999994) ;
#29329=CIRCLE('',#76471,0.0999999999999994) ;
#29330=CIRCLE('',#76473,0.0999999999999994) ;
#29331=CIRCLE('',#76476,0.0999999999999994) ;
#29332=CIRCLE('',#76478,0.1) ;
#29333=CIRCLE('',#76480,0.0999999999999994) ;
#29334=CIRCLE('',#76482,0.0999999999999994) ;
#29335=CIRCLE('',#76485,0.0999999999999994) ;
#29336=CIRCLE('',#76487,0.1) ;
#29337=CIRCLE('',#76489,0.0999999999999994) ;
#29338=CIRCLE('',#76491,0.0999999999999994) ;
#29339=CIRCLE('',#76494,0.0999999999999994) ;
#29340=CIRCLE('',#76496,0.0999999999999994) ;
#29341=CIRCLE('',#76498,0.1) ;
#29342=CIRCLE('',#76500,0.0999999999999994) ;
#29343=CIRCLE('',#76502,0.0999999999999994) ;
#29344=CIRCLE('',#76504,0.0999999999999994) ;
#29345=CIRCLE('',#76507,0.0999999999999994) ;
#29346=CIRCLE('',#76509,0.0999999999999994) ;
#29347=CIRCLE('',#76511,0.1) ;
#29348=CIRCLE('',#76513,0.0999999999999994) ;
#29349=CIRCLE('',#76515,0.0999999999999994) ;
#29350=CIRCLE('',#76517,0.0999999999999994) ;
#29351=CIRCLE('',#76520,0.0999999999999994) ;
#29352=CIRCLE('',#76522,0.1) ;
#29353=CIRCLE('',#76524,0.0999999999999994) ;
#29354=CIRCLE('',#76526,0.0999999999999994) ;
#29355=CIRCLE('',#76529,0.0999999999999994) ;
#29356=CIRCLE('',#76531,0.1) ;
#29357=CIRCLE('',#76533,0.0999999999999994) ;
#29358=CIRCLE('',#76535,0.0999999999999994) ;
#29359=CIRCLE('',#76538,0.0999999999999994) ;
#29360=CIRCLE('',#76540,0.0999999999999994) ;
#29361=CIRCLE('',#76542,0.1) ;
#29362=CIRCLE('',#76544,0.0999999999999994) ;
#29363=CIRCLE('',#76546,0.0999999999999994) ;
#29364=CIRCLE('',#76548,0.0999999999999994) ;
#29365=CIRCLE('',#76551,0.0999999999999994) ;
#29366=CIRCLE('',#76553,0.0999999999999994) ;
#29367=CIRCLE('',#76555,0.1) ;
#29368=CIRCLE('',#76557,0.0999999999999994) ;
#29369=CIRCLE('',#76559,0.0999999999999994) ;
#29370=CIRCLE('',#76561,0.0999999999999994) ;
#29371=CIRCLE('',#76564,0.0999999999999994) ;
#29372=CIRCLE('',#76566,0.1) ;
#29373=CIRCLE('',#76568,0.0999999999999994) ;
#29374=CIRCLE('',#76570,0.0999999999999994) ;
#29375=CIRCLE('',#76573,0.0999999999999994) ;
#29376=CIRCLE('',#76575,0.1) ;
#29377=CIRCLE('',#76577,0.0999999999999994) ;
#29378=CIRCLE('',#76579,0.0999999999999994) ;
#29379=CIRCLE('',#76582,0.0999999999999994) ;
#29380=CIRCLE('',#76584,0.0999999999999994) ;
#29381=CIRCLE('',#76586,0.1) ;
#29382=CIRCLE('',#76588,0.0999999999999994) ;
#29383=CIRCLE('',#76590,0.0999999999999994) ;
#29384=CIRCLE('',#76592,0.0999999999999994) ;
#29385=CIRCLE('',#76595,0.0999999999999994) ;
#29386=CIRCLE('',#76597,0.0999999999999994) ;
#29387=CIRCLE('',#76599,0.1) ;
#29388=CIRCLE('',#76601,0.0999999999999994) ;
#29389=CIRCLE('',#76603,0.0999999999999994) ;
#29390=CIRCLE('',#76605,0.0999999999999994) ;
#29391=CIRCLE('',#76608,0.0999999999999994) ;
#29392=CIRCLE('',#76610,0.1) ;
#29393=CIRCLE('',#76612,0.0999999999999994) ;
#29394=CIRCLE('',#76614,0.0999999999999994) ;
#29395=CIRCLE('',#76617,0.0999999999999994) ;
#29396=CIRCLE('',#76619,0.1) ;
#29397=CIRCLE('',#76621,0.0999999999999994) ;
#29398=CIRCLE('',#76623,0.0999999999999994) ;
#29399=CIRCLE('',#76626,0.100000000000003) ;
#29400=CIRCLE('',#76628,0.100000000000003) ;
#29401=CIRCLE('',#76630,0.1) ;
#29402=CIRCLE('',#76632,0.100000000000003) ;
#29403=CIRCLE('',#76634,0.100000000000003) ;
#29404=CIRCLE('',#76636,0.100000000000003) ;
#29405=CIRCLE('',#76639,0.100000000000003) ;
#29406=CIRCLE('',#76641,0.100000000000003) ;
#29407=CIRCLE('',#76643,0.1) ;
#29408=CIRCLE('',#76645,0.100000000000003) ;
#29409=CIRCLE('',#76647,0.100000000000003) ;
#29410=CIRCLE('',#76649,0.100000000000003) ;
#29411=CIRCLE('',#76652,0.100000000000003) ;
#29412=CIRCLE('',#76654,0.1) ;
#29413=CIRCLE('',#76656,0.100000000000003) ;
#29414=CIRCLE('',#76658,0.100000000000003) ;
#29415=CIRCLE('',#76661,0.100000000000003) ;
#29416=CIRCLE('',#76663,0.1) ;
#29417=CIRCLE('',#76665,0.100000000000003) ;
#29418=CIRCLE('',#76667,0.100000000000003) ;
#31998=VERTEX_POINT('',#113860) ;
#31999=VERTEX_POINT('',#113862) ;
#32000=VERTEX_POINT('',#113864) ;
#32001=VERTEX_POINT('',#113868) ;
#32002=VERTEX_POINT('',#113870) ;
#32003=VERTEX_POINT('',#113874) ;
#32004=VERTEX_POINT('',#113875) ;
#32005=VERTEX_POINT('',#113877) ;
#32006=VERTEX_POINT('',#113881) ;
#32007=VERTEX_POINT('',#113882) ;
#32008=VERTEX_POINT('',#113884) ;
#32009=VERTEX_POINT('',#113886) ;
#32010=VERTEX_POINT('',#113888) ;
#32011=VERTEX_POINT('',#113890) ;
#32012=VERTEX_POINT('',#113892) ;
#32013=VERTEX_POINT('',#113903) ;
#32014=VERTEX_POINT('',#113905) ;
#32015=VERTEX_POINT('',#113907) ;
#32016=VERTEX_POINT('',#113911) ;
#32017=VERTEX_POINT('',#113913) ;
#32018=VERTEX_POINT('',#113917) ;
#32019=VERTEX_POINT('',#113918) ;
#32020=VERTEX_POINT('',#113920) ;
#32021=VERTEX_POINT('',#113924) ;
#32022=VERTEX_POINT('',#113925) ;
#32023=VERTEX_POINT('',#113927) ;
#32024=VERTEX_POINT('',#113929) ;
#32025=VERTEX_POINT('',#113931) ;
#32026=VERTEX_POINT('',#113933) ;
#32027=VERTEX_POINT('',#113935) ;
#32028=VERTEX_POINT('',#113946) ;
#32029=VERTEX_POINT('',#113948) ;
#32030=VERTEX_POINT('',#113950) ;
#32031=VERTEX_POINT('',#113954) ;
#32032=VERTEX_POINT('',#113956) ;
#32033=VERTEX_POINT('',#113960) ;
#32034=VERTEX_POINT('',#113961) ;
#32035=VERTEX_POINT('',#113963) ;
#32036=VERTEX_POINT('',#113967) ;
#32037=VERTEX_POINT('',#113968) ;
#32038=VERTEX_POINT('',#113970) ;
#32039=VERTEX_POINT('',#113972) ;
#32040=VERTEX_POINT('',#113974) ;
#32041=VERTEX_POINT('',#113976) ;
#32042=VERTEX_POINT('',#113978) ;
#32043=VERTEX_POINT('',#113989) ;
#32044=VERTEX_POINT('',#113991) ;
#32045=VERTEX_POINT('',#113993) ;
#32046=VERTEX_POINT('',#113997) ;
#32047=VERTEX_POINT('',#113999) ;
#32048=VERTEX_POINT('',#114003) ;
#32049=VERTEX_POINT('',#114004) ;
#32050=VERTEX_POINT('',#114006) ;
#32051=VERTEX_POINT('',#114010) ;
#32052=VERTEX_POINT('',#114011) ;
#32053=VERTEX_POINT('',#114013) ;
#32054=VERTEX_POINT('',#114015) ;
#32055=VERTEX_POINT('',#114017) ;
#32056=VERTEX_POINT('',#114019) ;
#32057=VERTEX_POINT('',#114021) ;
#32058=VERTEX_POINT('',#114032) ;
#32059=VERTEX_POINT('',#114034) ;
#32060=VERTEX_POINT('',#114036) ;
#32061=VERTEX_POINT('',#114040) ;
#32062=VERTEX_POINT('',#114042) ;
#32063=VERTEX_POINT('',#114046) ;
#32064=VERTEX_POINT('',#114047) ;
#32065=VERTEX_POINT('',#114049) ;
#32066=VERTEX_POINT('',#114053) ;
#32067=VERTEX_POINT('',#114054) ;
#32068=VERTEX_POINT('',#114056) ;
#32069=VERTEX_POINT('',#114058) ;
#32070=VERTEX_POINT('',#114060) ;
#32071=VERTEX_POINT('',#114062) ;
#32072=VERTEX_POINT('',#114064) ;
#32073=VERTEX_POINT('',#114075) ;
#32074=VERTEX_POINT('',#114077) ;
#32075=VERTEX_POINT('',#114079) ;
#32076=VERTEX_POINT('',#114083) ;
#32077=VERTEX_POINT('',#114085) ;
#32078=VERTEX_POINT('',#114089) ;
#32079=VERTEX_POINT('',#114090) ;
#32080=VERTEX_POINT('',#114092) ;
#32081=VERTEX_POINT('',#114096) ;
#32082=VERTEX_POINT('',#114097) ;
#32083=VERTEX_POINT('',#114099) ;
#32084=VERTEX_POINT('',#114101) ;
#32085=VERTEX_POINT('',#114103) ;
#32086=VERTEX_POINT('',#114105) ;
#32087=VERTEX_POINT('',#114107) ;
#32088=VERTEX_POINT('',#114118) ;
#32089=VERTEX_POINT('',#114120) ;
#32090=VERTEX_POINT('',#114122) ;
#32091=VERTEX_POINT('',#114126) ;
#32092=VERTEX_POINT('',#114128) ;
#32093=VERTEX_POINT('',#114132) ;
#32094=VERTEX_POINT('',#114133) ;
#32095=VERTEX_POINT('',#114135) ;
#32096=VERTEX_POINT('',#114139) ;
#32097=VERTEX_POINT('',#114140) ;
#32098=VERTEX_POINT('',#114142) ;
#32099=VERTEX_POINT('',#114144) ;
#32100=VERTEX_POINT('',#114146) ;
#32101=VERTEX_POINT('',#114148) ;
#32102=VERTEX_POINT('',#114150) ;
#32103=VERTEX_POINT('',#114161) ;
#32104=VERTEX_POINT('',#114163) ;
#32105=VERTEX_POINT('',#114165) ;
#32106=VERTEX_POINT('',#114169) ;
#32107=VERTEX_POINT('',#114171) ;
#32108=VERTEX_POINT('',#114175) ;
#32109=VERTEX_POINT('',#114176) ;
#32110=VERTEX_POINT('',#114178) ;
#32111=VERTEX_POINT('',#114182) ;
#32112=VERTEX_POINT('',#114183) ;
#32113=VERTEX_POINT('',#114185) ;
#32114=VERTEX_POINT('',#114187) ;
#32115=VERTEX_POINT('',#114189) ;
#32116=VERTEX_POINT('',#114191) ;
#32117=VERTEX_POINT('',#114193) ;
#32118=VERTEX_POINT('',#114204) ;
#32119=VERTEX_POINT('',#114206) ;
#32120=VERTEX_POINT('',#114208) ;
#32121=VERTEX_POINT('',#114212) ;
#32122=VERTEX_POINT('',#114213) ;
#32123=VERTEX_POINT('',#114215) ;
#32124=VERTEX_POINT('',#114217) ;
#32125=VERTEX_POINT('',#114221) ;
#32126=VERTEX_POINT('',#114222) ;
#32127=VERTEX_POINT('',#114224) ;
#32128=VERTEX_POINT('',#114226) ;
#32129=VERTEX_POINT('',#114230) ;
#32130=VERTEX_POINT('',#114231) ;
#32131=VERTEX_POINT('',#114233) ;
#32132=VERTEX_POINT('',#114235) ;
#32133=VERTEX_POINT('',#114239) ;
#32134=VERTEX_POINT('',#114240) ;
#32135=VERTEX_POINT('',#114242) ;
#32136=VERTEX_POINT('',#114244) ;
#32137=VERTEX_POINT('',#114248) ;
#32138=VERTEX_POINT('',#114249) ;
#32139=VERTEX_POINT('',#114251) ;
#32140=VERTEX_POINT('',#114253) ;
#32141=VERTEX_POINT('',#114257) ;
#32142=VERTEX_POINT('',#114258) ;
#32143=VERTEX_POINT('',#114260) ;
#32144=VERTEX_POINT('',#114262) ;
#32145=VERTEX_POINT('',#114266) ;
#32146=VERTEX_POINT('',#114267) ;
#32147=VERTEX_POINT('',#114269) ;
#32148=VERTEX_POINT('',#114271) ;
#32149=VERTEX_POINT('',#114275) ;
#32150=VERTEX_POINT('',#114276) ;
#32151=VERTEX_POINT('',#114278) ;
#32152=VERTEX_POINT('',#114280) ;
#32153=VERTEX_POINT('',#114284) ;
#32154=VERTEX_POINT('',#114285) ;
#32155=VERTEX_POINT('',#114287) ;
#32156=VERTEX_POINT('',#114289) ;
#32157=VERTEX_POINT('',#114293) ;
#32158=VERTEX_POINT('',#114295) ;
#32159=VERTEX_POINT('',#114299) ;
#32160=VERTEX_POINT('',#114300) ;
#32161=VERTEX_POINT('',#114302) ;
#32162=VERTEX_POINT('',#114306) ;
#32163=VERTEX_POINT('',#114307) ;
#32164=VERTEX_POINT('',#114309) ;
#32165=VERTEX_POINT('',#114311) ;
#32166=VERTEX_POINT('',#114313) ;
#32167=VERTEX_POINT('',#114315) ;
#32168=VERTEX_POINT('',#114317) ;
#32169=VERTEX_POINT('',#114346) ;
#32170=VERTEX_POINT('',#114347) ;
#32171=VERTEX_POINT('',#114352) ;
#32172=VERTEX_POINT('',#114353) ;
#32173=VERTEX_POINT('',#114358) ;
#32174=VERTEX_POINT('',#114359) ;
#32175=VERTEX_POINT('',#114364) ;
#32176=VERTEX_POINT('',#114365) ;
#32177=VERTEX_POINT('',#114370) ;
#32178=VERTEX_POINT('',#114371) ;
#32179=VERTEX_POINT('',#114376) ;
#32180=VERTEX_POINT('',#114377) ;
#32181=VERTEX_POINT('',#114382) ;
#32182=VERTEX_POINT('',#114383) ;
#32183=VERTEX_POINT('',#114388) ;
#32184=VERTEX_POINT('',#114389) ;
#32185=VERTEX_POINT('',#114394) ;
#32186=VERTEX_POINT('',#114395) ;
#32187=VERTEX_POINT('',#114400) ;
#32188=VERTEX_POINT('',#114402) ;
#32189=VERTEX_POINT('',#114404) ;
#32190=VERTEX_POINT('',#114408) ;
#32191=VERTEX_POINT('',#114409) ;
#32192=VERTEX_POINT('',#114411) ;
#32193=VERTEX_POINT('',#114413) ;
#32194=VERTEX_POINT('',#114417) ;
#32195=VERTEX_POINT('',#114419) ;
#32196=VERTEX_POINT('',#114423) ;
#32197=VERTEX_POINT('',#114424) ;
#32198=VERTEX_POINT('',#114426) ;
#32199=VERTEX_POINT('',#114430) ;
#32200=VERTEX_POINT('',#114431) ;
#32201=VERTEX_POINT('',#114433) ;
#32202=VERTEX_POINT('',#114435) ;
#32203=VERTEX_POINT('',#114437) ;
#32204=VERTEX_POINT('',#114439) ;
#32205=VERTEX_POINT('',#114441) ;
#32206=VERTEX_POINT('',#114454) ;
#32207=VERTEX_POINT('',#114455) ;
#32208=VERTEX_POINT('',#114460) ;
#32209=VERTEX_POINT('',#114461) ;
#32210=VERTEX_POINT('',#114463) ;
#32211=VERTEX_POINT('',#114465) ;
#32212=VERTEX_POINT('',#114468) ;
#32213=VERTEX_POINT('',#114470) ;
#32214=VERTEX_POINT('',#114472) ;
#32215=VERTEX_POINT('',#114474) ;
#32216=VERTEX_POINT('',#114476) ;
#32217=VERTEX_POINT('',#114478) ;
#32218=VERTEX_POINT('',#114482) ;
#32219=VERTEX_POINT('',#114483) ;
#32220=VERTEX_POINT('',#114485) ;
#32221=VERTEX_POINT('',#114487) ;
#32222=VERTEX_POINT('',#114490) ;
#32223=VERTEX_POINT('',#114492) ;
#32224=VERTEX_POINT('',#114494) ;
#32225=VERTEX_POINT('',#114496) ;
#32226=VERTEX_POINT('',#114498) ;
#32227=VERTEX_POINT('',#114500) ;
#32228=VERTEX_POINT('',#114504) ;
#32229=VERTEX_POINT('',#114505) ;
#32230=VERTEX_POINT('',#114507) ;
#32231=VERTEX_POINT('',#114509) ;
#32232=VERTEX_POINT('',#114512) ;
#32233=VERTEX_POINT('',#114514) ;
#32234=VERTEX_POINT('',#114516) ;
#32235=VERTEX_POINT('',#114518) ;
#32236=VERTEX_POINT('',#114520) ;
#32237=VERTEX_POINT('',#114522) ;
#32238=VERTEX_POINT('',#114526) ;
#32239=VERTEX_POINT('',#114527) ;
#32240=VERTEX_POINT('',#114529) ;
#32241=VERTEX_POINT('',#114531) ;
#32242=VERTEX_POINT('',#114534) ;
#32243=VERTEX_POINT('',#114536) ;
#32244=VERTEX_POINT('',#114538) ;
#32245=VERTEX_POINT('',#114540) ;
#32246=VERTEX_POINT('',#114542) ;
#32247=VERTEX_POINT('',#114544) ;
#32248=VERTEX_POINT('',#114548) ;
#32249=VERTEX_POINT('',#114549) ;
#32250=VERTEX_POINT('',#114551) ;
#32251=VERTEX_POINT('',#114553) ;
#32252=VERTEX_POINT('',#114556) ;
#32253=VERTEX_POINT('',#114558) ;
#32254=VERTEX_POINT('',#114560) ;
#32255=VERTEX_POINT('',#114562) ;
#32256=VERTEX_POINT('',#114564) ;
#32257=VERTEX_POINT('',#114566) ;
#32258=VERTEX_POINT('',#114570) ;
#32259=VERTEX_POINT('',#114571) ;
#32260=VERTEX_POINT('',#114573) ;
#32261=VERTEX_POINT('',#114575) ;
#32262=VERTEX_POINT('',#114578) ;
#32263=VERTEX_POINT('',#114580) ;
#32264=VERTEX_POINT('',#114582) ;
#32265=VERTEX_POINT('',#114584) ;
#32266=VERTEX_POINT('',#114586) ;
#32267=VERTEX_POINT('',#114588) ;
#32268=VERTEX_POINT('',#114592) ;
#32269=VERTEX_POINT('',#114593) ;
#32270=VERTEX_POINT('',#114595) ;
#32271=VERTEX_POINT('',#114597) ;
#32272=VERTEX_POINT('',#114600) ;
#32273=VERTEX_POINT('',#114602) ;
#32274=VERTEX_POINT('',#114604) ;
#32275=VERTEX_POINT('',#114606) ;
#32276=VERTEX_POINT('',#114608) ;
#32277=VERTEX_POINT('',#114610) ;
#32278=VERTEX_POINT('',#114614) ;
#32279=VERTEX_POINT('',#114615) ;
#32280=VERTEX_POINT('',#114617) ;
#32281=VERTEX_POINT('',#114619) ;
#32282=VERTEX_POINT('',#114622) ;
#32283=VERTEX_POINT('',#114624) ;
#32284=VERTEX_POINT('',#114626) ;
#32285=VERTEX_POINT('',#114628) ;
#32286=VERTEX_POINT('',#114630) ;
#32287=VERTEX_POINT('',#114632) ;
#32288=VERTEX_POINT('',#114636) ;
#32289=VERTEX_POINT('',#114637) ;
#32290=VERTEX_POINT('',#114639) ;
#32291=VERTEX_POINT('',#114641) ;
#32292=VERTEX_POINT('',#114644) ;
#32293=VERTEX_POINT('',#114646) ;
#32294=VERTEX_POINT('',#114648) ;
#32295=VERTEX_POINT('',#114650) ;
#32296=VERTEX_POINT('',#114652) ;
#32297=VERTEX_POINT('',#114654) ;
#32298=VERTEX_POINT('',#114658) ;
#32299=VERTEX_POINT('',#114659) ;
#32300=VERTEX_POINT('',#114661) ;
#32301=VERTEX_POINT('',#114663) ;
#32302=VERTEX_POINT('',#114665) ;
#32303=VERTEX_POINT('',#114669) ;
#32304=VERTEX_POINT('',#114670) ;
#32305=VERTEX_POINT('',#114672) ;
#32306=VERTEX_POINT('',#114674) ;
#32307=VERTEX_POINT('',#114676) ;
#32308=VERTEX_POINT('',#114680) ;
#32309=VERTEX_POINT('',#114681) ;
#32310=VERTEX_POINT('',#114683) ;
#32311=VERTEX_POINT('',#114685) ;
#32312=VERTEX_POINT('',#114687) ;
#32313=VERTEX_POINT('',#114691) ;
#32314=VERTEX_POINT('',#114692) ;
#32315=VERTEX_POINT('',#114694) ;
#32316=VERTEX_POINT('',#114696) ;
#32317=VERTEX_POINT('',#114698) ;
#32318=VERTEX_POINT('',#114702) ;
#32319=VERTEX_POINT('',#114703) ;
#32320=VERTEX_POINT('',#114705) ;
#32321=VERTEX_POINT('',#114707) ;
#32322=VERTEX_POINT('',#114709) ;
#32323=VERTEX_POINT('',#114713) ;
#32324=VERTEX_POINT('',#114714) ;
#32325=VERTEX_POINT('',#114716) ;
#32326=VERTEX_POINT('',#114718) ;
#32327=VERTEX_POINT('',#114720) ;
#32328=VERTEX_POINT('',#114724) ;
#32329=VERTEX_POINT('',#114725) ;
#32330=VERTEX_POINT('',#114727) ;
#32331=VERTEX_POINT('',#114729) ;
#32332=VERTEX_POINT('',#114731) ;
#32333=VERTEX_POINT('',#114735) ;
#32334=VERTEX_POINT('',#114736) ;
#32335=VERTEX_POINT('',#114738) ;
#32336=VERTEX_POINT('',#114740) ;
#32337=VERTEX_POINT('',#114742) ;
#32338=VERTEX_POINT('',#114746) ;
#32339=VERTEX_POINT('',#114747) ;
#32340=VERTEX_POINT('',#114749) ;
#32341=VERTEX_POINT('',#114751) ;
#32342=VERTEX_POINT('',#114753) ;
#32343=VERTEX_POINT('',#114757) ;
#32344=VERTEX_POINT('',#114758) ;
#32345=VERTEX_POINT('',#114760) ;
#32346=VERTEX_POINT('',#114762) ;
#32347=VERTEX_POINT('',#114764) ;
#32348=VERTEX_POINT('',#114768) ;
#32349=VERTEX_POINT('',#114769) ;
#32350=VERTEX_POINT('',#114771) ;
#32351=VERTEX_POINT('',#114773) ;
#32352=VERTEX_POINT('',#114775) ;
#32353=VERTEX_POINT('',#114779) ;
#32354=VERTEX_POINT('',#114780) ;
#32355=VERTEX_POINT('',#114782) ;
#32356=VERTEX_POINT('',#114784) ;
#32357=VERTEX_POINT('',#114786) ;
#32358=VERTEX_POINT('',#114790) ;
#32359=VERTEX_POINT('',#114791) ;
#32360=VERTEX_POINT('',#114793) ;
#32361=VERTEX_POINT('',#114795) ;
#32362=VERTEX_POINT('',#114797) ;
#32363=VERTEX_POINT('',#114801) ;
#32364=VERTEX_POINT('',#114802) ;
#32365=VERTEX_POINT('',#114804) ;
#32366=VERTEX_POINT('',#114806) ;
#32367=VERTEX_POINT('',#114808) ;
#32368=VERTEX_POINT('',#114812) ;
#32369=VERTEX_POINT('',#114813) ;
#32370=VERTEX_POINT('',#114815) ;
#32371=VERTEX_POINT('',#114817) ;
#32372=VERTEX_POINT('',#114819) ;
#32373=VERTEX_POINT('',#114823) ;
#32374=VERTEX_POINT('',#114824) ;
#32375=VERTEX_POINT('',#114826) ;
#32376=VERTEX_POINT('',#114828) ;
#32377=VERTEX_POINT('',#114830) ;
#32378=VERTEX_POINT('',#114834) ;
#32379=VERTEX_POINT('',#114835) ;
#32380=VERTEX_POINT('',#114837) ;
#32381=VERTEX_POINT('',#114839) ;
#32382=VERTEX_POINT('',#114841) ;
#32383=VERTEX_POINT('',#114845) ;
#32384=VERTEX_POINT('',#114846) ;
#32385=VERTEX_POINT('',#114848) ;
#32386=VERTEX_POINT('',#114850) ;
#32387=VERTEX_POINT('',#114852) ;
#32388=VERTEX_POINT('',#114856) ;
#32389=VERTEX_POINT('',#114857) ;
#32390=VERTEX_POINT('',#114859) ;
#32391=VERTEX_POINT('',#114861) ;
#32392=VERTEX_POINT('',#114865) ;
#32393=VERTEX_POINT('',#114866) ;
#32394=VERTEX_POINT('',#114868) ;
#32395=VERTEX_POINT('',#114870) ;
#32396=VERTEX_POINT('',#114874) ;
#32397=VERTEX_POINT('',#114875) ;
#32398=VERTEX_POINT('',#114877) ;
#32399=VERTEX_POINT('',#114879) ;
#32400=VERTEX_POINT('',#114883) ;
#32401=VERTEX_POINT('',#114884) ;
#32402=VERTEX_POINT('',#114886) ;
#32403=VERTEX_POINT('',#114888) ;
#32404=VERTEX_POINT('',#114892) ;
#32405=VERTEX_POINT('',#114893) ;
#32406=VERTEX_POINT('',#114895) ;
#32407=VERTEX_POINT('',#114897) ;
#32408=VERTEX_POINT('',#114901) ;
#32409=VERTEX_POINT('',#114902) ;
#32410=VERTEX_POINT('',#114904) ;
#32411=VERTEX_POINT('',#114906) ;
#32412=VERTEX_POINT('',#114910) ;
#32413=VERTEX_POINT('',#114911) ;
#32414=VERTEX_POINT('',#114913) ;
#32415=VERTEX_POINT('',#114915) ;
#32416=VERTEX_POINT('',#114919) ;
#32417=VERTEX_POINT('',#114920) ;
#32418=VERTEX_POINT('',#114922) ;
#32419=VERTEX_POINT('',#114924) ;
#32420=VERTEX_POINT('',#114928) ;
#32421=VERTEX_POINT('',#114929) ;
#32422=VERTEX_POINT('',#114931) ;
#32423=VERTEX_POINT('',#114933) ;
#32424=VERTEX_POINT('',#114937) ;
#32425=VERTEX_POINT('',#114938) ;
#32426=VERTEX_POINT('',#114940) ;
#32427=VERTEX_POINT('',#114942) ;
#32428=VERTEX_POINT('',#114945) ;
#32429=VERTEX_POINT('',#114947) ;
#32430=VERTEX_POINT('',#114949) ;
#32431=VERTEX_POINT('',#114951) ;
#32432=VERTEX_POINT('',#114953) ;
#32433=VERTEX_POINT('',#114955) ;
#32434=VERTEX_POINT('',#114959) ;
#32435=VERTEX_POINT('',#114960) ;
#32436=VERTEX_POINT('',#114962) ;
#32437=VERTEX_POINT('',#114964) ;
#32438=VERTEX_POINT('',#114966) ;
#32439=VERTEX_POINT('',#114970) ;
#32440=VERTEX_POINT('',#114971) ;
#32441=VERTEX_POINT('',#114973) ;
#32442=VERTEX_POINT('',#114975) ;
#32443=VERTEX_POINT('',#114977) ;
#32444=VERTEX_POINT('',#114981) ;
#32445=VERTEX_POINT('',#114982) ;
#32446=VERTEX_POINT('',#114984) ;
#32447=VERTEX_POINT('',#114986) ;
#32448=VERTEX_POINT('',#114990) ;
#32449=VERTEX_POINT('',#114991) ;
#32450=VERTEX_POINT('',#114993) ;
#32451=VERTEX_POINT('',#114995) ;
#32452=VERTEX_POINT('',#114999) ;
#32453=VERTEX_POINT('',#115000) ;
#32454=VERTEX_POINT('',#115002) ;
#32455=VERTEX_POINT('',#115004) ;
#32456=VERTEX_POINT('',#115008) ;
#32457=VERTEX_POINT('',#115010) ;
#32458=VERTEX_POINT('',#115012) ;
#32459=VERTEX_POINT('',#115014) ;
#32460=VERTEX_POINT('',#115017) ;
#32461=VERTEX_POINT('',#115019) ;
#32462=VERTEX_POINT('',#115021) ;
#32463=VERTEX_POINT('',#115023) ;
#32464=VERTEX_POINT('',#115026) ;
#32465=VERTEX_POINT('',#115028) ;
#32466=VERTEX_POINT('',#115030) ;
#32467=VERTEX_POINT('',#115032) ;
#32468=VERTEX_POINT('',#115035) ;
#32469=VERTEX_POINT('',#115037) ;
#32470=VERTEX_POINT('',#115039) ;
#32471=VERTEX_POINT('',#115041) ;
#32472=VERTEX_POINT('',#115044) ;
#32473=VERTEX_POINT('',#115046) ;
#32474=VERTEX_POINT('',#115048) ;
#32475=VERTEX_POINT('',#115050) ;
#32476=VERTEX_POINT('',#115053) ;
#32477=VERTEX_POINT('',#115055) ;
#32478=VERTEX_POINT('',#115057) ;
#32479=VERTEX_POINT('',#115059) ;
#32480=VERTEX_POINT('',#115062) ;
#32481=VERTEX_POINT('',#115064) ;
#32482=VERTEX_POINT('',#115066) ;
#32483=VERTEX_POINT('',#115068) ;
#32484=VERTEX_POINT('',#115071) ;
#32485=VERTEX_POINT('',#115073) ;
#32486=VERTEX_POINT('',#115075) ;
#32487=VERTEX_POINT('',#115077) ;
#32488=VERTEX_POINT('',#115080) ;
#32489=VERTEX_POINT('',#115082) ;
#32490=VERTEX_POINT('',#115084) ;
#32491=VERTEX_POINT('',#115086) ;
#32492=VERTEX_POINT('',#115089) ;
#32493=VERTEX_POINT('',#115091) ;
#32494=VERTEX_POINT('',#115095) ;
#32495=VERTEX_POINT('',#115097) ;
#32496=VERTEX_POINT('',#115101) ;
#32497=VERTEX_POINT('',#115102) ;
#32498=VERTEX_POINT('',#115105) ;
#32499=VERTEX_POINT('',#115107) ;
#32500=VERTEX_POINT('',#115109) ;
#32501=VERTEX_POINT('',#115111) ;
#32502=VERTEX_POINT('',#115114) ;
#32503=VERTEX_POINT('',#115116) ;
#32504=VERTEX_POINT('',#115118) ;
#32505=VERTEX_POINT('',#115120) ;
#32506=VERTEX_POINT('',#115123) ;
#32507=VERTEX_POINT('',#115125) ;
#32508=VERTEX_POINT('',#115127) ;
#32509=VERTEX_POINT('',#115129) ;
#32510=VERTEX_POINT('',#115132) ;
#32511=VERTEX_POINT('',#115134) ;
#32512=VERTEX_POINT('',#115136) ;
#32513=VERTEX_POINT('',#115138) ;
#32514=VERTEX_POINT('',#115141) ;
#32515=VERTEX_POINT('',#115143) ;
#32516=VERTEX_POINT('',#115145) ;
#32517=VERTEX_POINT('',#115147) ;
#32518=VERTEX_POINT('',#115150) ;
#32519=VERTEX_POINT('',#115152) ;
#32520=VERTEX_POINT('',#115154) ;
#32521=VERTEX_POINT('',#115156) ;
#32522=VERTEX_POINT('',#115159) ;
#32523=VERTEX_POINT('',#115161) ;
#32524=VERTEX_POINT('',#115163) ;
#32525=VERTEX_POINT('',#115165) ;
#32526=VERTEX_POINT('',#115168) ;
#32527=VERTEX_POINT('',#115170) ;
#32528=VERTEX_POINT('',#115172) ;
#32529=VERTEX_POINT('',#115174) ;
#32530=VERTEX_POINT('',#115177) ;
#32531=VERTEX_POINT('',#115179) ;
#32532=VERTEX_POINT('',#115181) ;
#32533=VERTEX_POINT('',#115183) ;
#32534=VERTEX_POINT('',#115186) ;
#32535=VERTEX_POINT('',#115188) ;
#32536=VERTEX_POINT('',#115191) ;
#32537=VERTEX_POINT('',#115193) ;
#32538=VERTEX_POINT('',#115197) ;
#32539=VERTEX_POINT('',#115198) ;
#32540=VERTEX_POINT('',#115203) ;
#32541=VERTEX_POINT('',#115204) ;
#32542=VERTEX_POINT('',#115209) ;
#32543=VERTEX_POINT('',#115210) ;
#32544=VERTEX_POINT('',#115215) ;
#32545=VERTEX_POINT('',#115216) ;
#32546=VERTEX_POINT('',#115221) ;
#32547=VERTEX_POINT('',#115222) ;
#32548=VERTEX_POINT('',#115227) ;
#32549=VERTEX_POINT('',#115228) ;
#32550=VERTEX_POINT('',#115233) ;
#32551=VERTEX_POINT('',#115234) ;
#32552=VERTEX_POINT('',#115239) ;
#32553=VERTEX_POINT('',#115240) ;
#32554=VERTEX_POINT('',#115245) ;
#32555=VERTEX_POINT('',#115246) ;
#32556=VERTEX_POINT('',#115251) ;
#32557=VERTEX_POINT('',#115252) ;
#32558=VERTEX_POINT('',#115257) ;
#32559=VERTEX_POINT('',#115258) ;
#32560=VERTEX_POINT('',#115265) ;
#32561=VERTEX_POINT('',#115266) ;
#32562=VERTEX_POINT('',#115268) ;
#32563=VERTEX_POINT('',#115270) ;
#32564=VERTEX_POINT('',#115272) ;
#32565=VERTEX_POINT('',#115274) ;
#32566=VERTEX_POINT('',#115276) ;
#32567=VERTEX_POINT('',#115278) ;
#32568=VERTEX_POINT('',#115281) ;
#32569=VERTEX_POINT('',#115283) ;
#32570=VERTEX_POINT('',#115285) ;
#32571=VERTEX_POINT('',#115287) ;
#32572=VERTEX_POINT('',#115289) ;
#32573=VERTEX_POINT('',#115291) ;
#32574=VERTEX_POINT('',#115293) ;
#32575=VERTEX_POINT('',#115295) ;
#32576=VERTEX_POINT('',#115297) ;
#32577=VERTEX_POINT('',#115299) ;
#32578=VERTEX_POINT('',#115301) ;
#32579=VERTEX_POINT('',#115303) ;
#32580=VERTEX_POINT('',#115305) ;
#32581=VERTEX_POINT('',#115307) ;
#32582=VERTEX_POINT('',#115310) ;
#32583=VERTEX_POINT('',#115311) ;
#32584=VERTEX_POINT('',#115313) ;
#32585=VERTEX_POINT('',#115315) ;
#32586=VERTEX_POINT('',#115317) ;
#32587=VERTEX_POINT('',#115319) ;
#32588=VERTEX_POINT('',#115321) ;
#32589=VERTEX_POINT('',#115323) ;
#32590=VERTEX_POINT('',#115326) ;
#32591=VERTEX_POINT('',#115328) ;
#32592=VERTEX_POINT('',#115330) ;
#32593=VERTEX_POINT('',#115332) ;
#32594=VERTEX_POINT('',#115334) ;
#32595=VERTEX_POINT('',#115336) ;
#32596=VERTEX_POINT('',#115338) ;
#32597=VERTEX_POINT('',#115340) ;
#32598=VERTEX_POINT('',#115342) ;
#32599=VERTEX_POINT('',#115344) ;
#32600=VERTEX_POINT('',#115346) ;
#32601=VERTEX_POINT('',#115348) ;
#32602=VERTEX_POINT('',#115350) ;
#32603=VERTEX_POINT('',#115352) ;
#32604=VERTEX_POINT('',#115355) ;
#32605=VERTEX_POINT('',#115356) ;
#32606=VERTEX_POINT('',#115358) ;
#32607=VERTEX_POINT('',#115360) ;
#32608=VERTEX_POINT('',#115362) ;
#32609=VERTEX_POINT('',#115364) ;
#32610=VERTEX_POINT('',#115366) ;
#32611=VERTEX_POINT('',#115368) ;
#32612=VERTEX_POINT('',#115371) ;
#32613=VERTEX_POINT('',#115373) ;
#32614=VERTEX_POINT('',#115375) ;
#32615=VERTEX_POINT('',#115377) ;
#32616=VERTEX_POINT('',#115379) ;
#32617=VERTEX_POINT('',#115381) ;
#32618=VERTEX_POINT('',#115383) ;
#32619=VERTEX_POINT('',#115385) ;
#32620=VERTEX_POINT('',#115387) ;
#32621=VERTEX_POINT('',#115389) ;
#32622=VERTEX_POINT('',#115391) ;
#32623=VERTEX_POINT('',#115393) ;
#32624=VERTEX_POINT('',#115395) ;
#32625=VERTEX_POINT('',#115397) ;
#32626=VERTEX_POINT('',#115400) ;
#32627=VERTEX_POINT('',#115401) ;
#32628=VERTEX_POINT('',#115403) ;
#32629=VERTEX_POINT('',#115405) ;
#32630=VERTEX_POINT('',#115407) ;
#32631=VERTEX_POINT('',#115409) ;
#32632=VERTEX_POINT('',#115411) ;
#32633=VERTEX_POINT('',#115413) ;
#32634=VERTEX_POINT('',#115416) ;
#32635=VERTEX_POINT('',#115418) ;
#32636=VERTEX_POINT('',#115420) ;
#32637=VERTEX_POINT('',#115422) ;
#32638=VERTEX_POINT('',#115424) ;
#32639=VERTEX_POINT('',#115426) ;
#32640=VERTEX_POINT('',#115428) ;
#32641=VERTEX_POINT('',#115430) ;
#32642=VERTEX_POINT('',#115432) ;
#32643=VERTEX_POINT('',#115434) ;
#32644=VERTEX_POINT('',#115436) ;
#32645=VERTEX_POINT('',#115438) ;
#32646=VERTEX_POINT('',#115440) ;
#32647=VERTEX_POINT('',#115442) ;
#32648=VERTEX_POINT('',#115445) ;
#32649=VERTEX_POINT('',#115446) ;
#32650=VERTEX_POINT('',#115448) ;
#32651=VERTEX_POINT('',#115450) ;
#32652=VERTEX_POINT('',#115452) ;
#32653=VERTEX_POINT('',#115454) ;
#32654=VERTEX_POINT('',#115456) ;
#32655=VERTEX_POINT('',#115458) ;
#32656=VERTEX_POINT('',#115461) ;
#32657=VERTEX_POINT('',#115463) ;
#32658=VERTEX_POINT('',#115465) ;
#32659=VERTEX_POINT('',#115467) ;
#32660=VERTEX_POINT('',#115469) ;
#32661=VERTEX_POINT('',#115471) ;
#32662=VERTEX_POINT('',#115473) ;
#32663=VERTEX_POINT('',#115475) ;
#32664=VERTEX_POINT('',#115477) ;
#32665=VERTEX_POINT('',#115479) ;
#32666=VERTEX_POINT('',#115481) ;
#32667=VERTEX_POINT('',#115483) ;
#32668=VERTEX_POINT('',#115485) ;
#32669=VERTEX_POINT('',#115487) ;
#32670=VERTEX_POINT('',#115490) ;
#32671=VERTEX_POINT('',#115491) ;
#32672=VERTEX_POINT('',#115493) ;
#32673=VERTEX_POINT('',#115495) ;
#32674=VERTEX_POINT('',#115497) ;
#32675=VERTEX_POINT('',#115499) ;
#32676=VERTEX_POINT('',#115501) ;
#32677=VERTEX_POINT('',#115503) ;
#32678=VERTEX_POINT('',#115506) ;
#32679=VERTEX_POINT('',#115508) ;
#32680=VERTEX_POINT('',#115510) ;
#32681=VERTEX_POINT('',#115512) ;
#32682=VERTEX_POINT('',#115514) ;
#32683=VERTEX_POINT('',#115516) ;
#32684=VERTEX_POINT('',#115518) ;
#32685=VERTEX_POINT('',#115520) ;
#32686=VERTEX_POINT('',#115522) ;
#32687=VERTEX_POINT('',#115524) ;
#32688=VERTEX_POINT('',#115526) ;
#32689=VERTEX_POINT('',#115528) ;
#32690=VERTEX_POINT('',#115530) ;
#32691=VERTEX_POINT('',#115532) ;
#32692=VERTEX_POINT('',#115535) ;
#32693=VERTEX_POINT('',#115536) ;
#32694=VERTEX_POINT('',#115538) ;
#32695=VERTEX_POINT('',#115540) ;
#32696=VERTEX_POINT('',#115542) ;
#32697=VERTEX_POINT('',#115544) ;
#32698=VERTEX_POINT('',#115546) ;
#32699=VERTEX_POINT('',#115548) ;
#32700=VERTEX_POINT('',#115551) ;
#32701=VERTEX_POINT('',#115553) ;
#32702=VERTEX_POINT('',#115555) ;
#32703=VERTEX_POINT('',#115557) ;
#32704=VERTEX_POINT('',#115559) ;
#32705=VERTEX_POINT('',#115561) ;
#32706=VERTEX_POINT('',#115563) ;
#32707=VERTEX_POINT('',#115565) ;
#32708=VERTEX_POINT('',#115567) ;
#32709=VERTEX_POINT('',#115569) ;
#32710=VERTEX_POINT('',#115571) ;
#32711=VERTEX_POINT('',#115573) ;
#32712=VERTEX_POINT('',#115575) ;
#32713=VERTEX_POINT('',#115577) ;
#32714=VERTEX_POINT('',#115580) ;
#32715=VERTEX_POINT('',#115581) ;
#32716=VERTEX_POINT('',#115583) ;
#32717=VERTEX_POINT('',#115585) ;
#32718=VERTEX_POINT('',#115587) ;
#32719=VERTEX_POINT('',#115589) ;
#32720=VERTEX_POINT('',#115591) ;
#32721=VERTEX_POINT('',#115593) ;
#32722=VERTEX_POINT('',#115596) ;
#32723=VERTEX_POINT('',#115598) ;
#32724=VERTEX_POINT('',#115600) ;
#32725=VERTEX_POINT('',#115602) ;
#32726=VERTEX_POINT('',#115604) ;
#32727=VERTEX_POINT('',#115606) ;
#32728=VERTEX_POINT('',#115608) ;
#32729=VERTEX_POINT('',#115610) ;
#32730=VERTEX_POINT('',#115612) ;
#32731=VERTEX_POINT('',#115614) ;
#32732=VERTEX_POINT('',#115616) ;
#32733=VERTEX_POINT('',#115618) ;
#32734=VERTEX_POINT('',#115620) ;
#32735=VERTEX_POINT('',#115622) ;
#32736=VERTEX_POINT('',#115625) ;
#32737=VERTEX_POINT('',#115626) ;
#32738=VERTEX_POINT('',#115628) ;
#32739=VERTEX_POINT('',#115630) ;
#32740=VERTEX_POINT('',#115632) ;
#32741=VERTEX_POINT('',#115634) ;
#32742=VERTEX_POINT('',#115636) ;
#32743=VERTEX_POINT('',#115638) ;
#32744=VERTEX_POINT('',#115641) ;
#32745=VERTEX_POINT('',#115643) ;
#32746=VERTEX_POINT('',#115645) ;
#32747=VERTEX_POINT('',#115647) ;
#32748=VERTEX_POINT('',#115649) ;
#32749=VERTEX_POINT('',#115651) ;
#32750=VERTEX_POINT('',#115653) ;
#32751=VERTEX_POINT('',#115655) ;
#32752=VERTEX_POINT('',#115657) ;
#32753=VERTEX_POINT('',#115659) ;
#32754=VERTEX_POINT('',#115661) ;
#32755=VERTEX_POINT('',#115663) ;
#32756=VERTEX_POINT('',#115665) ;
#32757=VERTEX_POINT('',#115667) ;
#32758=VERTEX_POINT('',#115670) ;
#32759=VERTEX_POINT('',#115671) ;
#32760=VERTEX_POINT('',#115673) ;
#32761=VERTEX_POINT('',#115675) ;
#32762=VERTEX_POINT('',#115677) ;
#32763=VERTEX_POINT('',#115679) ;
#32764=VERTEX_POINT('',#115681) ;
#32765=VERTEX_POINT('',#115683) ;
#32766=VERTEX_POINT('',#115686) ;
#32767=VERTEX_POINT('',#115688) ;
#32768=VERTEX_POINT('',#115690) ;
#32769=VERTEX_POINT('',#115692) ;
#32770=VERTEX_POINT('',#115694) ;
#32771=VERTEX_POINT('',#115696) ;
#32772=VERTEX_POINT('',#115698) ;
#32773=VERTEX_POINT('',#115700) ;
#32774=VERTEX_POINT('',#115702) ;
#32775=VERTEX_POINT('',#115704) ;
#32776=VERTEX_POINT('',#115706) ;
#32777=VERTEX_POINT('',#115708) ;
#32778=VERTEX_POINT('',#115710) ;
#32779=VERTEX_POINT('',#115712) ;
#32780=VERTEX_POINT('',#115716) ;
#32781=VERTEX_POINT('',#115717) ;
#32782=VERTEX_POINT('',#115719) ;
#32783=VERTEX_POINT('',#115721) ;
#32784=VERTEX_POINT('',#115723) ;
#32785=VERTEX_POINT('',#115725) ;
#32786=VERTEX_POINT('',#115727) ;
#32787=VERTEX_POINT('',#115729) ;
#32788=VERTEX_POINT('',#115731) ;
#32789=VERTEX_POINT('',#115733) ;
#32790=VERTEX_POINT('',#115737) ;
#32791=VERTEX_POINT('',#115738) ;
#32792=VERTEX_POINT('',#115740) ;
#32793=VERTEX_POINT('',#115742) ;
#32794=VERTEX_POINT('',#115744) ;
#32795=VERTEX_POINT('',#115746) ;
#32796=VERTEX_POINT('',#115748) ;
#32797=VERTEX_POINT('',#115750) ;
#32798=VERTEX_POINT('',#115752) ;
#32799=VERTEX_POINT('',#115754) ;
#32800=VERTEX_POINT('',#115758) ;
#32801=VERTEX_POINT('',#115759) ;
#32802=VERTEX_POINT('',#115761) ;
#32803=VERTEX_POINT('',#115763) ;
#32804=VERTEX_POINT('',#115765) ;
#32805=VERTEX_POINT('',#115767) ;
#32806=VERTEX_POINT('',#115769) ;
#32807=VERTEX_POINT('',#115771) ;
#32808=VERTEX_POINT('',#115773) ;
#32809=VERTEX_POINT('',#115775) ;
#32810=VERTEX_POINT('',#115779) ;
#32811=VERTEX_POINT('',#115780) ;
#32812=VERTEX_POINT('',#115782) ;
#32813=VERTEX_POINT('',#115784) ;
#32814=VERTEX_POINT('',#115788) ;
#32815=VERTEX_POINT('',#115790) ;
#32816=VERTEX_POINT('',#115794) ;
#32817=VERTEX_POINT('',#115795) ;
#32818=VERTEX_POINT('',#115797) ;
#32819=VERTEX_POINT('',#115799) ;
#32820=VERTEX_POINT('',#115803) ;
#32821=VERTEX_POINT('',#115804) ;
#32822=VERTEX_POINT('',#115806) ;
#32823=VERTEX_POINT('',#115808) ;
#32824=VERTEX_POINT('',#115812) ;
#32825=VERTEX_POINT('',#115813) ;
#32826=VERTEX_POINT('',#115815) ;
#32827=VERTEX_POINT('',#115817) ;
#32828=VERTEX_POINT('',#115821) ;
#32829=VERTEX_POINT('',#115822) ;
#32830=VERTEX_POINT('',#115824) ;
#32831=VERTEX_POINT('',#115826) ;
#32832=VERTEX_POINT('',#115830) ;
#32833=VERTEX_POINT('',#115832) ;
#32834=VERTEX_POINT('',#115836) ;
#32835=VERTEX_POINT('',#115838) ;
#32836=VERTEX_POINT('',#115842) ;
#32837=VERTEX_POINT('',#115844) ;
#32838=VERTEX_POINT('',#115848) ;
#32839=VERTEX_POINT('',#115850) ;
#32840=VERTEX_POINT('',#115855) ;
#32841=VERTEX_POINT('',#115859) ;
#32842=VERTEX_POINT('',#115866) ;
#32843=VERTEX_POINT('',#115868) ;
#32844=VERTEX_POINT('',#115872) ;
#32845=VERTEX_POINT('',#115874) ;
#32846=VERTEX_POINT('',#115878) ;
#32847=VERTEX_POINT('',#115880) ;
#32848=VERTEX_POINT('',#115884) ;
#32849=VERTEX_POINT('',#115886) ;
#32850=VERTEX_POINT('',#115890) ;
#32851=VERTEX_POINT('',#115892) ;
#32852=VERTEX_POINT('',#115896) ;
#32853=VERTEX_POINT('',#115898) ;
#32854=VERTEX_POINT('',#115902) ;
#32855=VERTEX_POINT('',#115904) ;
#32856=VERTEX_POINT('',#115908) ;
#32857=VERTEX_POINT('',#115910) ;
#32858=VERTEX_POINT('',#115914) ;
#32859=VERTEX_POINT('',#115916) ;
#32860=VERTEX_POINT('',#115920) ;
#32861=VERTEX_POINT('',#115922) ;
#32862=VERTEX_POINT('',#115926) ;
#32863=VERTEX_POINT('',#115928) ;
#32864=VERTEX_POINT('',#115932) ;
#32865=VERTEX_POINT('',#115934) ;
#32866=VERTEX_POINT('',#115938) ;
#32867=VERTEX_POINT('',#115940) ;
#32868=VERTEX_POINT('',#115944) ;
#32869=VERTEX_POINT('',#115946) ;
#32870=VERTEX_POINT('',#115950) ;
#32871=VERTEX_POINT('',#115952) ;
#32872=VERTEX_POINT('',#115956) ;
#32873=VERTEX_POINT('',#115958) ;
#32874=VERTEX_POINT('',#115962) ;
#32875=VERTEX_POINT('',#115964) ;
#32876=VERTEX_POINT('',#115968) ;
#32877=VERTEX_POINT('',#115970) ;
#32878=VERTEX_POINT('',#115977) ;
#32879=VERTEX_POINT('',#115978) ;
#32880=VERTEX_POINT('',#115980) ;
#32881=VERTEX_POINT('',#115982) ;
#32882=VERTEX_POINT('',#115984) ;
#32883=VERTEX_POINT('',#115986) ;
#32884=VERTEX_POINT('',#115988) ;
#32885=VERTEX_POINT('',#115990) ;
#32886=VERTEX_POINT('',#115992) ;
#32887=VERTEX_POINT('',#115994) ;
#32888=VERTEX_POINT('',#115996) ;
#32889=VERTEX_POINT('',#115998) ;
#32890=VERTEX_POINT('',#116000) ;
#32891=VERTEX_POINT('',#116002) ;
#32892=VERTEX_POINT('',#116004) ;
#32893=VERTEX_POINT('',#116006) ;
#32894=VERTEX_POINT('',#116009) ;
#32895=VERTEX_POINT('',#116013) ;
#32896=VERTEX_POINT('',#116014) ;
#32897=VERTEX_POINT('',#116016) ;
#32898=VERTEX_POINT('',#116018) ;
#32899=VERTEX_POINT('',#116020) ;
#32900=VERTEX_POINT('',#116022) ;
#32901=VERTEX_POINT('',#116024) ;
#32902=VERTEX_POINT('',#116026) ;
#32903=VERTEX_POINT('',#116036) ;
#32904=VERTEX_POINT('',#116046) ;
#32905=VERTEX_POINT('',#116057) ;
#32906=VERTEX_POINT('',#116089) ;
#32907=VERTEX_POINT('',#116136) ;
#32908=VERTEX_POINT('',#116154) ;
#32909=VERTEX_POINT('',#116168) ;
#32910=VERTEX_POINT('',#116183) ;
#32911=VERTEX_POINT('',#116374) ;
#32912=VERTEX_POINT('',#116375) ;
#32913=VERTEX_POINT('',#116377) ;
#32914=VERTEX_POINT('',#116379) ;
#32915=VERTEX_POINT('',#116383) ;
#32916=VERTEX_POINT('',#116384) ;
#32917=VERTEX_POINT('',#116386) ;
#32918=VERTEX_POINT('',#116388) ;
#32919=VERTEX_POINT('',#116392) ;
#32920=VERTEX_POINT('',#116393) ;
#32921=VERTEX_POINT('',#116395) ;
#32922=VERTEX_POINT('',#116397) ;
#32923=VERTEX_POINT('',#116401) ;
#32924=VERTEX_POINT('',#116402) ;
#32925=VERTEX_POINT('',#116404) ;
#32926=VERTEX_POINT('',#116406) ;
#32927=VERTEX_POINT('',#116410) ;
#32928=VERTEX_POINT('',#116411) ;
#32929=VERTEX_POINT('',#116413) ;
#32930=VERTEX_POINT('',#116415) ;
#32931=VERTEX_POINT('',#116419) ;
#32932=VERTEX_POINT('',#116420) ;
#32933=VERTEX_POINT('',#116423) ;
#32934=VERTEX_POINT('',#116425) ;
#32935=VERTEX_POINT('',#116429) ;
#32936=VERTEX_POINT('',#116430) ;
#32937=VERTEX_POINT('',#116433) ;
#32938=VERTEX_POINT('',#116435) ;
#32939=VERTEX_POINT('',#116445) ;
#32940=VERTEX_POINT('',#116446) ;
#32941=VERTEX_POINT('',#116448) ;
#32942=VERTEX_POINT('',#116450) ;
#32943=VERTEX_POINT('',#116454) ;
#32944=VERTEX_POINT('',#116455) ;
#32945=VERTEX_POINT('',#116460) ;
#32946=VERTEX_POINT('',#116462) ;
#32947=VERTEX_POINT('',#116466) ;
#32948=VERTEX_POINT('',#116467) ;
#32949=VERTEX_POINT('',#116469) ;
#32950=VERTEX_POINT('',#116471) ;
#32951=VERTEX_POINT('',#116475) ;
#32952=VERTEX_POINT('',#116476) ;
#32953=VERTEX_POINT('',#116478) ;
#32954=VERTEX_POINT('',#116480) ;
#32955=VERTEX_POINT('',#116484) ;
#32956=VERTEX_POINT('',#116485) ;
#32957=VERTEX_POINT('',#116490) ;
#32958=VERTEX_POINT('',#116492) ;
#32959=VERTEX_POINT('',#116496) ;
#32960=VERTEX_POINT('',#116497) ;
#32961=VERTEX_POINT('',#116499) ;
#32962=VERTEX_POINT('',#116501) ;
#32963=VERTEX_POINT('',#116505) ;
#32964=VERTEX_POINT('',#116506) ;
#32965=VERTEX_POINT('',#116508) ;
#32966=VERTEX_POINT('',#116510) ;
#32967=VERTEX_POINT('',#116514) ;
#32968=VERTEX_POINT('',#116515) ;
#32969=VERTEX_POINT('',#116517) ;
#32970=VERTEX_POINT('',#116519) ;
#32971=VERTEX_POINT('',#116523) ;
#32972=VERTEX_POINT('',#116524) ;
#32973=VERTEX_POINT('',#116526) ;
#32974=VERTEX_POINT('',#116528) ;
#32975=VERTEX_POINT('',#116644) ;
#32976=VERTEX_POINT('',#116645) ;
#32977=VERTEX_POINT('',#116647) ;
#32978=VERTEX_POINT('',#116649) ;
#32979=VERTEX_POINT('',#116651) ;
#32980=VERTEX_POINT('',#116653) ;
#32981=VERTEX_POINT('',#116655) ;
#32982=VERTEX_POINT('',#116657) ;
#32983=VERTEX_POINT('',#116659) ;
#32984=VERTEX_POINT('',#116661) ;
#32985=VERTEX_POINT('',#116665) ;
#32986=VERTEX_POINT('',#116666) ;
#32987=VERTEX_POINT('',#116668) ;
#32988=VERTEX_POINT('',#116670) ;
#32989=VERTEX_POINT('',#116672) ;
#32990=VERTEX_POINT('',#116674) ;
#32991=VERTEX_POINT('',#116676) ;
#32992=VERTEX_POINT('',#116678) ;
#32993=VERTEX_POINT('',#116680) ;
#32994=VERTEX_POINT('',#116682) ;
#32995=VERTEX_POINT('',#116686) ;
#32996=VERTEX_POINT('',#116687) ;
#32997=VERTEX_POINT('',#116689) ;
#32998=VERTEX_POINT('',#116691) ;
#32999=VERTEX_POINT('',#116693) ;
#33000=VERTEX_POINT('',#116695) ;
#33001=VERTEX_POINT('',#116697) ;
#33002=VERTEX_POINT('',#116699) ;
#33003=VERTEX_POINT('',#116701) ;
#33004=VERTEX_POINT('',#116703) ;
#33005=VERTEX_POINT('',#116707) ;
#33006=VERTEX_POINT('',#116708) ;
#33007=VERTEX_POINT('',#116710) ;
#33008=VERTEX_POINT('',#116712) ;
#33009=VERTEX_POINT('',#116714) ;
#33010=VERTEX_POINT('',#116716) ;
#33011=VERTEX_POINT('',#116718) ;
#33012=VERTEX_POINT('',#116720) ;
#33013=VERTEX_POINT('',#116722) ;
#33014=VERTEX_POINT('',#116724) ;
#33015=VERTEX_POINT('',#116728) ;
#33016=VERTEX_POINT('',#116729) ;
#33017=VERTEX_POINT('',#116731) ;
#33018=VERTEX_POINT('',#116733) ;
#33019=VERTEX_POINT('',#116735) ;
#33020=VERTEX_POINT('',#116737) ;
#33021=VERTEX_POINT('',#116739) ;
#33022=VERTEX_POINT('',#116741) ;
#33023=VERTEX_POINT('',#116743) ;
#33024=VERTEX_POINT('',#116745) ;
#33025=VERTEX_POINT('',#116749) ;
#33026=VERTEX_POINT('',#116750) ;
#33027=VERTEX_POINT('',#116752) ;
#33028=VERTEX_POINT('',#116754) ;
#33029=VERTEX_POINT('',#116756) ;
#33030=VERTEX_POINT('',#116758) ;
#33031=VERTEX_POINT('',#116760) ;
#33032=VERTEX_POINT('',#116762) ;
#33033=VERTEX_POINT('',#116764) ;
#33034=VERTEX_POINT('',#116766) ;
#33035=VERTEX_POINT('',#116770) ;
#33036=VERTEX_POINT('',#116771) ;
#33037=VERTEX_POINT('',#116773) ;
#33038=VERTEX_POINT('',#116775) ;
#33039=VERTEX_POINT('',#116777) ;
#33040=VERTEX_POINT('',#116779) ;
#33041=VERTEX_POINT('',#116781) ;
#33042=VERTEX_POINT('',#116783) ;
#33043=VERTEX_POINT('',#116785) ;
#33044=VERTEX_POINT('',#116787) ;
#33045=VERTEX_POINT('',#116791) ;
#33046=VERTEX_POINT('',#116792) ;
#33047=VERTEX_POINT('',#116794) ;
#33048=VERTEX_POINT('',#116796) ;
#33049=VERTEX_POINT('',#116798) ;
#33050=VERTEX_POINT('',#116800) ;
#33051=VERTEX_POINT('',#116802) ;
#33052=VERTEX_POINT('',#116804) ;
#33053=VERTEX_POINT('',#116806) ;
#33054=VERTEX_POINT('',#116808) ;
#33055=VERTEX_POINT('',#116812) ;
#33056=VERTEX_POINT('',#116813) ;
#33057=VERTEX_POINT('',#116815) ;
#33058=VERTEX_POINT('',#116817) ;
#33059=VERTEX_POINT('',#116819) ;
#33060=VERTEX_POINT('',#116821) ;
#33061=VERTEX_POINT('',#116823) ;
#33062=VERTEX_POINT('',#116825) ;
#33063=VERTEX_POINT('',#116827) ;
#33064=VERTEX_POINT('',#116829) ;
#33065=VERTEX_POINT('',#116833) ;
#33066=VERTEX_POINT('',#116834) ;
#33067=VERTEX_POINT('',#116836) ;
#33068=VERTEX_POINT('',#116838) ;
#33069=VERTEX_POINT('',#116842) ;
#33070=VERTEX_POINT('',#116844) ;
#33071=VERTEX_POINT('',#116848) ;
#33072=VERTEX_POINT('',#116849) ;
#33073=VERTEX_POINT('',#116851) ;
#33074=VERTEX_POINT('',#116853) ;
#33075=VERTEX_POINT('',#116857) ;
#33076=VERTEX_POINT('',#116858) ;
#33077=VERTEX_POINT('',#116860) ;
#33078=VERTEX_POINT('',#116862) ;
#33079=VERTEX_POINT('',#116866) ;
#33080=VERTEX_POINT('',#116867) ;
#33081=VERTEX_POINT('',#116869) ;
#33082=VERTEX_POINT('',#116871) ;
#33083=VERTEX_POINT('',#116875) ;
#33084=VERTEX_POINT('',#116876) ;
#33085=VERTEX_POINT('',#116878) ;
#33086=VERTEX_POINT('',#116880) ;
#33087=VERTEX_POINT('',#116884) ;
#33088=VERTEX_POINT('',#116886) ;
#33089=VERTEX_POINT('',#116890) ;
#33090=VERTEX_POINT('',#116891) ;
#33091=VERTEX_POINT('',#116893) ;
#33092=VERTEX_POINT('',#116895) ;
#33093=VERTEX_POINT('',#116899) ;
#33094=VERTEX_POINT('',#116900) ;
#33095=VERTEX_POINT('',#116902) ;
#33096=VERTEX_POINT('',#116904) ;
#33097=VERTEX_POINT('',#116908) ;
#33098=VERTEX_POINT('',#116909) ;
#33099=VERTEX_POINT('',#116911) ;
#33100=VERTEX_POINT('',#116913) ;
#33101=VERTEX_POINT('',#116917) ;
#33102=VERTEX_POINT('',#116918) ;
#33103=VERTEX_POINT('',#116920) ;
#33104=VERTEX_POINT('',#116922) ;
#33105=VERTEX_POINT('',#116926) ;
#33106=VERTEX_POINT('',#116928) ;
#33107=VERTEX_POINT('',#116932) ;
#33108=VERTEX_POINT('',#116933) ;
#33109=VERTEX_POINT('',#116935) ;
#33110=VERTEX_POINT('',#116937) ;
#33111=VERTEX_POINT('',#116941) ;
#33112=VERTEX_POINT('',#116942) ;
#33113=VERTEX_POINT('',#116944) ;
#33114=VERTEX_POINT('',#116946) ;
#33115=VERTEX_POINT('',#116950) ;
#33116=VERTEX_POINT('',#116951) ;
#33117=VERTEX_POINT('',#116953) ;
#33118=VERTEX_POINT('',#116955) ;
#33119=VERTEX_POINT('',#116959) ;
#33120=VERTEX_POINT('',#116960) ;
#33121=VERTEX_POINT('',#116962) ;
#33122=VERTEX_POINT('',#116964) ;
#33123=VERTEX_POINT('',#116968) ;
#33124=VERTEX_POINT('',#116970) ;
#33125=VERTEX_POINT('',#116974) ;
#33126=VERTEX_POINT('',#116975) ;
#33127=VERTEX_POINT('',#116977) ;
#33128=VERTEX_POINT('',#116979) ;
#33129=VERTEX_POINT('',#116983) ;
#33130=VERTEX_POINT('',#116984) ;
#33131=VERTEX_POINT('',#116986) ;
#33132=VERTEX_POINT('',#116988) ;
#33133=VERTEX_POINT('',#116992) ;
#33134=VERTEX_POINT('',#116993) ;
#33135=VERTEX_POINT('',#116995) ;
#33136=VERTEX_POINT('',#116997) ;
#33137=VERTEX_POINT('',#117001) ;
#33138=VERTEX_POINT('',#117002) ;
#33139=VERTEX_POINT('',#117004) ;
#33140=VERTEX_POINT('',#117006) ;
#33141=VERTEX_POINT('',#117010) ;
#33142=VERTEX_POINT('',#117012) ;
#33143=VERTEX_POINT('',#117016) ;
#33144=VERTEX_POINT('',#117017) ;
#33145=VERTEX_POINT('',#117019) ;
#33146=VERTEX_POINT('',#117021) ;
#33147=VERTEX_POINT('',#117025) ;
#33148=VERTEX_POINT('',#117026) ;
#33149=VERTEX_POINT('',#117028) ;
#33150=VERTEX_POINT('',#117030) ;
#33151=VERTEX_POINT('',#117034) ;
#33152=VERTEX_POINT('',#117035) ;
#33153=VERTEX_POINT('',#117037) ;
#33154=VERTEX_POINT('',#117039) ;
#33155=VERTEX_POINT('',#117043) ;
#33156=VERTEX_POINT('',#117044) ;
#33157=VERTEX_POINT('',#117046) ;
#33158=VERTEX_POINT('',#117048) ;
#33159=VERTEX_POINT('',#117052) ;
#33160=VERTEX_POINT('',#117054) ;
#33161=VERTEX_POINT('',#117058) ;
#33162=VERTEX_POINT('',#117059) ;
#33163=VERTEX_POINT('',#117061) ;
#33164=VERTEX_POINT('',#117063) ;
#33165=VERTEX_POINT('',#117067) ;
#33166=VERTEX_POINT('',#117068) ;
#33167=VERTEX_POINT('',#117070) ;
#33168=VERTEX_POINT('',#117072) ;
#33169=VERTEX_POINT('',#117076) ;
#33170=VERTEX_POINT('',#117077) ;
#33171=VERTEX_POINT('',#117079) ;
#33172=VERTEX_POINT('',#117081) ;
#33173=VERTEX_POINT('',#117085) ;
#33174=VERTEX_POINT('',#117086) ;
#33175=VERTEX_POINT('',#117088) ;
#33176=VERTEX_POINT('',#117090) ;
#33177=VERTEX_POINT('',#117094) ;
#33178=VERTEX_POINT('',#117096) ;
#33179=VERTEX_POINT('',#117100) ;
#33180=VERTEX_POINT('',#117101) ;
#33181=VERTEX_POINT('',#117103) ;
#33182=VERTEX_POINT('',#117105) ;
#33183=VERTEX_POINT('',#117109) ;
#33184=VERTEX_POINT('',#117110) ;
#33185=VERTEX_POINT('',#117112) ;
#33186=VERTEX_POINT('',#117114) ;
#33187=VERTEX_POINT('',#117118) ;
#33188=VERTEX_POINT('',#117119) ;
#33189=VERTEX_POINT('',#117121) ;
#33190=VERTEX_POINT('',#117123) ;
#33191=VERTEX_POINT('',#117127) ;
#33192=VERTEX_POINT('',#117128) ;
#33193=VERTEX_POINT('',#117130) ;
#33194=VERTEX_POINT('',#117132) ;
#33195=VERTEX_POINT('',#117136) ;
#33196=VERTEX_POINT('',#117138) ;
#33197=VERTEX_POINT('',#117142) ;
#33198=VERTEX_POINT('',#117143) ;
#33199=VERTEX_POINT('',#117145) ;
#33200=VERTEX_POINT('',#117147) ;
#33201=VERTEX_POINT('',#117151) ;
#33202=VERTEX_POINT('',#117152) ;
#33203=VERTEX_POINT('',#117154) ;
#33204=VERTEX_POINT('',#117156) ;
#33205=VERTEX_POINT('',#117160) ;
#33206=VERTEX_POINT('',#117161) ;
#33207=VERTEX_POINT('',#117163) ;
#33208=VERTEX_POINT('',#117165) ;
#33209=VERTEX_POINT('',#117169) ;
#33210=VERTEX_POINT('',#117170) ;
#33211=VERTEX_POINT('',#117172) ;
#33212=VERTEX_POINT('',#117174) ;
#33213=VERTEX_POINT('',#117178) ;
#33214=VERTEX_POINT('',#117180) ;
#33215=VERTEX_POINT('',#117184) ;
#33216=VERTEX_POINT('',#117185) ;
#33217=VERTEX_POINT('',#117187) ;
#33218=VERTEX_POINT('',#117189) ;
#33219=VERTEX_POINT('',#117193) ;
#33220=VERTEX_POINT('',#117194) ;
#33221=VERTEX_POINT('',#117196) ;
#33222=VERTEX_POINT('',#117198) ;
#33223=VERTEX_POINT('',#117202) ;
#33224=VERTEX_POINT('',#117203) ;
#33225=VERTEX_POINT('',#117205) ;
#33226=VERTEX_POINT('',#117207) ;
#33227=VERTEX_POINT('',#117211) ;
#33228=VERTEX_POINT('',#117212) ;
#33229=VERTEX_POINT('',#117214) ;
#33230=VERTEX_POINT('',#117216) ;
#33231=VERTEX_POINT('',#117220) ;
#33232=VERTEX_POINT('',#117222) ;
#33233=VERTEX_POINT('',#117226) ;
#33234=VERTEX_POINT('',#117228) ;
#33235=VERTEX_POINT('',#117232) ;
#33236=VERTEX_POINT('',#117234) ;
#33237=VERTEX_POINT('',#117238) ;
#33238=VERTEX_POINT('',#117240) ;
#33239=VERTEX_POINT('',#117245) ;
#33240=VERTEX_POINT('',#117249) ;
#33241=VERTEX_POINT('',#117256) ;
#33242=VERTEX_POINT('',#117258) ;
#33243=VERTEX_POINT('',#117262) ;
#33244=VERTEX_POINT('',#117264) ;
#33245=VERTEX_POINT('',#117268) ;
#33246=VERTEX_POINT('',#117270) ;
#33247=VERTEX_POINT('',#117274) ;
#33248=VERTEX_POINT('',#117276) ;
#33249=VERTEX_POINT('',#117280) ;
#33250=VERTEX_POINT('',#117282) ;
#33251=VERTEX_POINT('',#117286) ;
#33252=VERTEX_POINT('',#117288) ;
#33253=VERTEX_POINT('',#117292) ;
#33254=VERTEX_POINT('',#117294) ;
#33255=VERTEX_POINT('',#117298) ;
#33256=VERTEX_POINT('',#117300) ;
#33257=VERTEX_POINT('',#117304) ;
#33258=VERTEX_POINT('',#117306) ;
#33259=VERTEX_POINT('',#117310) ;
#33260=VERTEX_POINT('',#117312) ;
#33261=VERTEX_POINT('',#117316) ;
#33262=VERTEX_POINT('',#117318) ;
#33263=VERTEX_POINT('',#117322) ;
#33264=VERTEX_POINT('',#117324) ;
#33265=VERTEX_POINT('',#117328) ;
#33266=VERTEX_POINT('',#117330) ;
#33267=VERTEX_POINT('',#117334) ;
#33268=VERTEX_POINT('',#117336) ;
#33269=VERTEX_POINT('',#117340) ;
#33270=VERTEX_POINT('',#117342) ;
#33271=VERTEX_POINT('',#117346) ;
#33272=VERTEX_POINT('',#117348) ;
#33273=VERTEX_POINT('',#117352) ;
#33274=VERTEX_POINT('',#117354) ;
#33275=VERTEX_POINT('',#117358) ;
#33276=VERTEX_POINT('',#117360) ;
#33277=VERTEX_POINT('',#117367) ;
#33278=VERTEX_POINT('',#117368) ;
#33279=VERTEX_POINT('',#117370) ;
#33280=VERTEX_POINT('',#117372) ;
#33281=VERTEX_POINT('',#117374) ;
#33282=VERTEX_POINT('',#117376) ;
#33283=VERTEX_POINT('',#117378) ;
#33284=VERTEX_POINT('',#117380) ;
#33285=VERTEX_POINT('',#117382) ;
#33286=VERTEX_POINT('',#117384) ;
#33287=VERTEX_POINT('',#117386) ;
#33288=VERTEX_POINT('',#117388) ;
#33289=VERTEX_POINT('',#117390) ;
#33290=VERTEX_POINT('',#117392) ;
#33291=VERTEX_POINT('',#117394) ;
#33292=VERTEX_POINT('',#117396) ;
#33293=VERTEX_POINT('',#117399) ;
#33294=VERTEX_POINT('',#117403) ;
#33295=VERTEX_POINT('',#117404) ;
#33296=VERTEX_POINT('',#117406) ;
#33297=VERTEX_POINT('',#117408) ;
#33298=VERTEX_POINT('',#117412) ;
#33299=VERTEX_POINT('',#117414) ;
#33300=VERTEX_POINT('',#117418) ;
#33301=VERTEX_POINT('',#117420) ;
#33302=VERTEX_POINT('',#117424) ;
#33303=VERTEX_POINT('',#117426) ;
#33304=VERTEX_POINT('',#117430) ;
#33305=VERTEX_POINT('',#117432) ;
#33306=VERTEX_POINT('',#117437) ;
#33307=VERTEX_POINT('',#117441) ;
#33308=VERTEX_POINT('',#117448) ;
#33309=VERTEX_POINT('',#117450) ;
#33310=VERTEX_POINT('',#117454) ;
#33311=VERTEX_POINT('',#117456) ;
#33312=VERTEX_POINT('',#117460) ;
#33313=VERTEX_POINT('',#117462) ;
#33314=VERTEX_POINT('',#117466) ;
#33315=VERTEX_POINT('',#117468) ;
#33316=VERTEX_POINT('',#117472) ;
#33317=VERTEX_POINT('',#117474) ;
#33318=VERTEX_POINT('',#117478) ;
#33319=VERTEX_POINT('',#117480) ;
#33320=VERTEX_POINT('',#117484) ;
#33321=VERTEX_POINT('',#117486) ;
#33322=VERTEX_POINT('',#117490) ;
#33323=VERTEX_POINT('',#117492) ;
#33324=VERTEX_POINT('',#117496) ;
#33325=VERTEX_POINT('',#117498) ;
#33326=VERTEX_POINT('',#117502) ;
#33327=VERTEX_POINT('',#117504) ;
#33328=VERTEX_POINT('',#117508) ;
#33329=VERTEX_POINT('',#117510) ;
#33330=VERTEX_POINT('',#117514) ;
#33331=VERTEX_POINT('',#117516) ;
#33332=VERTEX_POINT('',#117520) ;
#33333=VERTEX_POINT('',#117522) ;
#33334=VERTEX_POINT('',#117526) ;
#33335=VERTEX_POINT('',#117528) ;
#33336=VERTEX_POINT('',#117532) ;
#33337=VERTEX_POINT('',#117534) ;
#33338=VERTEX_POINT('',#117538) ;
#33339=VERTEX_POINT('',#117540) ;
#33340=VERTEX_POINT('',#117544) ;
#33341=VERTEX_POINT('',#117546) ;
#33342=VERTEX_POINT('',#117550) ;
#33343=VERTEX_POINT('',#117552) ;
#33344=VERTEX_POINT('',#117559) ;
#33345=VERTEX_POINT('',#117560) ;
#33346=VERTEX_POINT('',#117562) ;
#33347=VERTEX_POINT('',#117564) ;
#33348=VERTEX_POINT('',#117566) ;
#33349=VERTEX_POINT('',#117568) ;
#33350=VERTEX_POINT('',#117570) ;
#33351=VERTEX_POINT('',#117572) ;
#33352=VERTEX_POINT('',#117574) ;
#33353=VERTEX_POINT('',#117576) ;
#33354=VERTEX_POINT('',#117578) ;
#33355=VERTEX_POINT('',#117580) ;
#33356=VERTEX_POINT('',#117582) ;
#33357=VERTEX_POINT('',#117584) ;
#33358=VERTEX_POINT('',#117586) ;
#33359=VERTEX_POINT('',#117588) ;
#33360=VERTEX_POINT('',#117591) ;
#33361=VERTEX_POINT('',#117595) ;
#33362=VERTEX_POINT('',#117596) ;
#33363=VERTEX_POINT('',#117598) ;
#33364=VERTEX_POINT('',#117600) ;
#33365=VERTEX_POINT('',#117604) ;
#33366=VERTEX_POINT('',#117606) ;
#33367=VERTEX_POINT('',#117610) ;
#33368=VERTEX_POINT('',#117612) ;
#33369=VERTEX_POINT('',#117616) ;
#33370=VERTEX_POINT('',#117618) ;
#33371=VERTEX_POINT('',#117622) ;
#33372=VERTEX_POINT('',#117624) ;
#33373=VERTEX_POINT('',#117629) ;
#33374=VERTEX_POINT('',#117633) ;
#33375=VERTEX_POINT('',#117640) ;
#33376=VERTEX_POINT('',#117642) ;
#33377=VERTEX_POINT('',#117646) ;
#33378=VERTEX_POINT('',#117648) ;
#33379=VERTEX_POINT('',#117652) ;
#33380=VERTEX_POINT('',#117654) ;
#33381=VERTEX_POINT('',#117658) ;
#33382=VERTEX_POINT('',#117660) ;
#33383=VERTEX_POINT('',#117664) ;
#33384=VERTEX_POINT('',#117666) ;
#33385=VERTEX_POINT('',#117670) ;
#33386=VERTEX_POINT('',#117672) ;
#33387=VERTEX_POINT('',#117676) ;
#33388=VERTEX_POINT('',#117678) ;
#33389=VERTEX_POINT('',#117682) ;
#33390=VERTEX_POINT('',#117684) ;
#33391=VERTEX_POINT('',#117688) ;
#33392=VERTEX_POINT('',#117690) ;
#33393=VERTEX_POINT('',#117694) ;
#33394=VERTEX_POINT('',#117696) ;
#33395=VERTEX_POINT('',#117700) ;
#33396=VERTEX_POINT('',#117702) ;
#33397=VERTEX_POINT('',#117706) ;
#33398=VERTEX_POINT('',#117708) ;
#33399=VERTEX_POINT('',#117712) ;
#33400=VERTEX_POINT('',#117714) ;
#33401=VERTEX_POINT('',#117718) ;
#33402=VERTEX_POINT('',#117720) ;
#33403=VERTEX_POINT('',#117724) ;
#33404=VERTEX_POINT('',#117726) ;
#33405=VERTEX_POINT('',#117730) ;
#33406=VERTEX_POINT('',#117732) ;
#33407=VERTEX_POINT('',#117736) ;
#33408=VERTEX_POINT('',#117738) ;
#33409=VERTEX_POINT('',#117742) ;
#33410=VERTEX_POINT('',#117744) ;
#33411=VERTEX_POINT('',#117751) ;
#33412=VERTEX_POINT('',#117752) ;
#33413=VERTEX_POINT('',#117754) ;
#33414=VERTEX_POINT('',#117756) ;
#33415=VERTEX_POINT('',#117758) ;
#33416=VERTEX_POINT('',#117760) ;
#33417=VERTEX_POINT('',#117762) ;
#33418=VERTEX_POINT('',#117764) ;
#33419=VERTEX_POINT('',#117766) ;
#33420=VERTEX_POINT('',#117768) ;
#33421=VERTEX_POINT('',#117770) ;
#33422=VERTEX_POINT('',#117772) ;
#33423=VERTEX_POINT('',#117774) ;
#33424=VERTEX_POINT('',#117776) ;
#33425=VERTEX_POINT('',#117778) ;
#33426=VERTEX_POINT('',#117780) ;
#33427=VERTEX_POINT('',#117783) ;
#33428=VERTEX_POINT('',#117787) ;
#33429=VERTEX_POINT('',#117788) ;
#33430=VERTEX_POINT('',#117790) ;
#33431=VERTEX_POINT('',#117792) ;
#33432=VERTEX_POINT('',#117796) ;
#33433=VERTEX_POINT('',#117798) ;
#33434=VERTEX_POINT('',#117802) ;
#33435=VERTEX_POINT('',#117804) ;
#33436=VERTEX_POINT('',#117808) ;
#33437=VERTEX_POINT('',#117810) ;
#33438=VERTEX_POINT('',#117814) ;
#33439=VERTEX_POINT('',#117816) ;
#33440=VERTEX_POINT('',#117821) ;
#33441=VERTEX_POINT('',#117825) ;
#33442=VERTEX_POINT('',#117832) ;
#33443=VERTEX_POINT('',#117834) ;
#33444=VERTEX_POINT('',#117838) ;
#33445=VERTEX_POINT('',#117840) ;
#33446=VERTEX_POINT('',#117844) ;
#33447=VERTEX_POINT('',#117846) ;
#33448=VERTEX_POINT('',#117850) ;
#33449=VERTEX_POINT('',#117852) ;
#33450=VERTEX_POINT('',#117856) ;
#33451=VERTEX_POINT('',#117858) ;
#33452=VERTEX_POINT('',#117862) ;
#33453=VERTEX_POINT('',#117864) ;
#33454=VERTEX_POINT('',#117868) ;
#33455=VERTEX_POINT('',#117870) ;
#33456=VERTEX_POINT('',#117874) ;
#33457=VERTEX_POINT('',#117876) ;
#33458=VERTEX_POINT('',#117880) ;
#33459=VERTEX_POINT('',#117882) ;
#33460=VERTEX_POINT('',#117886) ;
#33461=VERTEX_POINT('',#117888) ;
#33462=VERTEX_POINT('',#117892) ;
#33463=VERTEX_POINT('',#117894) ;
#33464=VERTEX_POINT('',#117898) ;
#33465=VERTEX_POINT('',#117900) ;
#33466=VERTEX_POINT('',#117904) ;
#33467=VERTEX_POINT('',#117906) ;
#33468=VERTEX_POINT('',#117910) ;
#33469=VERTEX_POINT('',#117912) ;
#33470=VERTEX_POINT('',#117916) ;
#33471=VERTEX_POINT('',#117918) ;
#33472=VERTEX_POINT('',#117922) ;
#33473=VERTEX_POINT('',#117924) ;
#33474=VERTEX_POINT('',#117928) ;
#33475=VERTEX_POINT('',#117930) ;
#33476=VERTEX_POINT('',#117934) ;
#33477=VERTEX_POINT('',#117936) ;
#33478=VERTEX_POINT('',#117943) ;
#33479=VERTEX_POINT('',#117944) ;
#33480=VERTEX_POINT('',#117946) ;
#33481=VERTEX_POINT('',#117948) ;
#33482=VERTEX_POINT('',#117950) ;
#33483=VERTEX_POINT('',#117952) ;
#33484=VERTEX_POINT('',#117954) ;
#33485=VERTEX_POINT('',#117956) ;
#33486=VERTEX_POINT('',#117958) ;
#33487=VERTEX_POINT('',#117960) ;
#33488=VERTEX_POINT('',#117962) ;
#33489=VERTEX_POINT('',#117964) ;
#33490=VERTEX_POINT('',#117966) ;
#33491=VERTEX_POINT('',#117968) ;
#33492=VERTEX_POINT('',#117970) ;
#33493=VERTEX_POINT('',#117972) ;
#33494=VERTEX_POINT('',#117975) ;
#33495=VERTEX_POINT('',#117979) ;
#33496=VERTEX_POINT('',#117980) ;
#33497=VERTEX_POINT('',#117982) ;
#33498=VERTEX_POINT('',#117984) ;
#33499=VERTEX_POINT('',#117988) ;
#33500=VERTEX_POINT('',#117990) ;
#33501=VERTEX_POINT('',#117994) ;
#33502=VERTEX_POINT('',#117996) ;
#33503=VERTEX_POINT('',#118000) ;
#33504=VERTEX_POINT('',#118002) ;
#33505=VERTEX_POINT('',#118006) ;
#33506=VERTEX_POINT('',#118008) ;
#33507=VERTEX_POINT('',#118013) ;
#33508=VERTEX_POINT('',#118017) ;
#33509=VERTEX_POINT('',#118024) ;
#33510=VERTEX_POINT('',#118026) ;
#33511=VERTEX_POINT('',#118030) ;
#33512=VERTEX_POINT('',#118032) ;
#33513=VERTEX_POINT('',#118036) ;
#33514=VERTEX_POINT('',#118038) ;
#33515=VERTEX_POINT('',#118042) ;
#33516=VERTEX_POINT('',#118044) ;
#33517=VERTEX_POINT('',#118048) ;
#33518=VERTEX_POINT('',#118050) ;
#33519=VERTEX_POINT('',#118054) ;
#33520=VERTEX_POINT('',#118056) ;
#33521=VERTEX_POINT('',#118060) ;
#33522=VERTEX_POINT('',#118062) ;
#33523=VERTEX_POINT('',#118066) ;
#33524=VERTEX_POINT('',#118068) ;
#33525=VERTEX_POINT('',#118072) ;
#33526=VERTEX_POINT('',#118074) ;
#33527=VERTEX_POINT('',#118078) ;
#33528=VERTEX_POINT('',#118080) ;
#33529=VERTEX_POINT('',#118084) ;
#33530=VERTEX_POINT('',#118086) ;
#33531=VERTEX_POINT('',#118090) ;
#33532=VERTEX_POINT('',#118092) ;
#33533=VERTEX_POINT('',#118096) ;
#33534=VERTEX_POINT('',#118098) ;
#33535=VERTEX_POINT('',#118102) ;
#33536=VERTEX_POINT('',#118104) ;
#33537=VERTEX_POINT('',#118108) ;
#33538=VERTEX_POINT('',#118110) ;
#33539=VERTEX_POINT('',#118114) ;
#33540=VERTEX_POINT('',#118116) ;
#33541=VERTEX_POINT('',#118120) ;
#33542=VERTEX_POINT('',#118122) ;
#33543=VERTEX_POINT('',#118126) ;
#33544=VERTEX_POINT('',#118128) ;
#33545=VERTEX_POINT('',#118135) ;
#33546=VERTEX_POINT('',#118136) ;
#33547=VERTEX_POINT('',#118138) ;
#33548=VERTEX_POINT('',#118140) ;
#33549=VERTEX_POINT('',#118142) ;
#33550=VERTEX_POINT('',#118144) ;
#33551=VERTEX_POINT('',#118146) ;
#33552=VERTEX_POINT('',#118148) ;
#33553=VERTEX_POINT('',#118150) ;
#33554=VERTEX_POINT('',#118152) ;
#33555=VERTEX_POINT('',#118154) ;
#33556=VERTEX_POINT('',#118156) ;
#33557=VERTEX_POINT('',#118158) ;
#33558=VERTEX_POINT('',#118160) ;
#33559=VERTEX_POINT('',#118162) ;
#33560=VERTEX_POINT('',#118164) ;
#33561=VERTEX_POINT('',#118167) ;
#33562=VERTEX_POINT('',#118171) ;
#33563=VERTEX_POINT('',#118172) ;
#33564=VERTEX_POINT('',#118174) ;
#33565=VERTEX_POINT('',#118176) ;
#33566=VERTEX_POINT('',#118180) ;
#33567=VERTEX_POINT('',#118182) ;
#33568=VERTEX_POINT('',#118186) ;
#33569=VERTEX_POINT('',#118188) ;
#33570=VERTEX_POINT('',#118192) ;
#33571=VERTEX_POINT('',#118194) ;
#33572=VERTEX_POINT('',#118198) ;
#33573=VERTEX_POINT('',#118200) ;
#33574=VERTEX_POINT('',#118205) ;
#33575=VERTEX_POINT('',#118209) ;
#33576=VERTEX_POINT('',#118216) ;
#33577=VERTEX_POINT('',#118218) ;
#33578=VERTEX_POINT('',#118222) ;
#33579=VERTEX_POINT('',#118224) ;
#33580=VERTEX_POINT('',#118228) ;
#33581=VERTEX_POINT('',#118230) ;
#33582=VERTEX_POINT('',#118234) ;
#33583=VERTEX_POINT('',#118236) ;
#33584=VERTEX_POINT('',#118240) ;
#33585=VERTEX_POINT('',#118242) ;
#33586=VERTEX_POINT('',#118246) ;
#33587=VERTEX_POINT('',#118248) ;
#33588=VERTEX_POINT('',#118252) ;
#33589=VERTEX_POINT('',#118254) ;
#33590=VERTEX_POINT('',#118258) ;
#33591=VERTEX_POINT('',#118260) ;
#33592=VERTEX_POINT('',#118264) ;
#33593=VERTEX_POINT('',#118266) ;
#33594=VERTEX_POINT('',#118270) ;
#33595=VERTEX_POINT('',#118272) ;
#33596=VERTEX_POINT('',#118276) ;
#33597=VERTEX_POINT('',#118278) ;
#33598=VERTEX_POINT('',#118282) ;
#33599=VERTEX_POINT('',#118284) ;
#33600=VERTEX_POINT('',#118288) ;
#33601=VERTEX_POINT('',#118290) ;
#33602=VERTEX_POINT('',#118294) ;
#33603=VERTEX_POINT('',#118296) ;
#33604=VERTEX_POINT('',#118300) ;
#33605=VERTEX_POINT('',#118302) ;
#33606=VERTEX_POINT('',#118306) ;
#33607=VERTEX_POINT('',#118308) ;
#33608=VERTEX_POINT('',#118312) ;
#33609=VERTEX_POINT('',#118314) ;
#33610=VERTEX_POINT('',#118318) ;
#33611=VERTEX_POINT('',#118320) ;
#33612=VERTEX_POINT('',#118327) ;
#33613=VERTEX_POINT('',#118328) ;
#33614=VERTEX_POINT('',#118330) ;
#33615=VERTEX_POINT('',#118332) ;
#33616=VERTEX_POINT('',#118334) ;
#33617=VERTEX_POINT('',#118336) ;
#33618=VERTEX_POINT('',#118338) ;
#33619=VERTEX_POINT('',#118340) ;
#33620=VERTEX_POINT('',#118342) ;
#33621=VERTEX_POINT('',#118344) ;
#33622=VERTEX_POINT('',#118346) ;
#33623=VERTEX_POINT('',#118348) ;
#33624=VERTEX_POINT('',#118350) ;
#33625=VERTEX_POINT('',#118352) ;
#33626=VERTEX_POINT('',#118354) ;
#33627=VERTEX_POINT('',#118356) ;
#33628=VERTEX_POINT('',#118359) ;
#33629=VERTEX_POINT('',#118363) ;
#33630=VERTEX_POINT('',#118364) ;
#33631=VERTEX_POINT('',#118366) ;
#33632=VERTEX_POINT('',#118368) ;
#33633=VERTEX_POINT('',#118372) ;
#33634=VERTEX_POINT('',#118374) ;
#33635=VERTEX_POINT('',#118378) ;
#33636=VERTEX_POINT('',#118380) ;
#33637=VERTEX_POINT('',#118384) ;
#33638=VERTEX_POINT('',#118386) ;
#33639=VERTEX_POINT('',#118390) ;
#33640=VERTEX_POINT('',#118392) ;
#33641=VERTEX_POINT('',#118397) ;
#33642=VERTEX_POINT('',#118401) ;
#33643=VERTEX_POINT('',#118408) ;
#33644=VERTEX_POINT('',#118410) ;
#33645=VERTEX_POINT('',#118414) ;
#33646=VERTEX_POINT('',#118416) ;
#33647=VERTEX_POINT('',#118420) ;
#33648=VERTEX_POINT('',#118422) ;
#33649=VERTEX_POINT('',#118426) ;
#33650=VERTEX_POINT('',#118428) ;
#33651=VERTEX_POINT('',#118432) ;
#33652=VERTEX_POINT('',#118434) ;
#33653=VERTEX_POINT('',#118438) ;
#33654=VERTEX_POINT('',#118440) ;
#33655=VERTEX_POINT('',#118444) ;
#33656=VERTEX_POINT('',#118446) ;
#33657=VERTEX_POINT('',#118450) ;
#33658=VERTEX_POINT('',#118452) ;
#33659=VERTEX_POINT('',#118456) ;
#33660=VERTEX_POINT('',#118458) ;
#33661=VERTEX_POINT('',#118462) ;
#33662=VERTEX_POINT('',#118464) ;
#33663=VERTEX_POINT('',#118468) ;
#33664=VERTEX_POINT('',#118470) ;
#33665=VERTEX_POINT('',#118474) ;
#33666=VERTEX_POINT('',#118476) ;
#33667=VERTEX_POINT('',#118480) ;
#33668=VERTEX_POINT('',#118482) ;
#33669=VERTEX_POINT('',#118486) ;
#33670=VERTEX_POINT('',#118488) ;
#33671=VERTEX_POINT('',#118492) ;
#33672=VERTEX_POINT('',#118494) ;
#33673=VERTEX_POINT('',#118498) ;
#33674=VERTEX_POINT('',#118500) ;
#33675=VERTEX_POINT('',#118504) ;
#33676=VERTEX_POINT('',#118506) ;
#33677=VERTEX_POINT('',#118510) ;
#33678=VERTEX_POINT('',#118512) ;
#33679=VERTEX_POINT('',#118519) ;
#33680=VERTEX_POINT('',#118520) ;
#33681=VERTEX_POINT('',#118522) ;
#33682=VERTEX_POINT('',#118524) ;
#33683=VERTEX_POINT('',#118526) ;
#33684=VERTEX_POINT('',#118528) ;
#33685=VERTEX_POINT('',#118530) ;
#33686=VERTEX_POINT('',#118532) ;
#33687=VERTEX_POINT('',#118534) ;
#33688=VERTEX_POINT('',#118536) ;
#33689=VERTEX_POINT('',#118538) ;
#33690=VERTEX_POINT('',#118540) ;
#33691=VERTEX_POINT('',#118542) ;
#33692=VERTEX_POINT('',#118544) ;
#33693=VERTEX_POINT('',#118546) ;
#33694=VERTEX_POINT('',#118548) ;
#33695=VERTEX_POINT('',#118551) ;
#33696=VERTEX_POINT('',#118555) ;
#33697=VERTEX_POINT('',#118556) ;
#33698=VERTEX_POINT('',#118558) ;
#33699=VERTEX_POINT('',#118560) ;
#33700=VERTEX_POINT('',#118564) ;
#33701=VERTEX_POINT('',#118566) ;
#33702=VERTEX_POINT('',#118570) ;
#33703=VERTEX_POINT('',#118572) ;
#33704=VERTEX_POINT('',#118576) ;
#33705=VERTEX_POINT('',#118578) ;
#33706=VERTEX_POINT('',#118582) ;
#33707=VERTEX_POINT('',#118584) ;
#33708=VERTEX_POINT('',#118589) ;
#33709=VERTEX_POINT('',#118593) ;
#33710=VERTEX_POINT('',#118600) ;
#33711=VERTEX_POINT('',#118602) ;
#33712=VERTEX_POINT('',#118606) ;
#33713=VERTEX_POINT('',#118608) ;
#33714=VERTEX_POINT('',#118612) ;
#33715=VERTEX_POINT('',#118614) ;
#33716=VERTEX_POINT('',#118618) ;
#33717=VERTEX_POINT('',#118620) ;
#33718=VERTEX_POINT('',#118624) ;
#33719=VERTEX_POINT('',#118626) ;
#33720=VERTEX_POINT('',#118630) ;
#33721=VERTEX_POINT('',#118632) ;
#33722=VERTEX_POINT('',#118636) ;
#33723=VERTEX_POINT('',#118638) ;
#33724=VERTEX_POINT('',#118642) ;
#33725=VERTEX_POINT('',#118644) ;
#33726=VERTEX_POINT('',#118648) ;
#33727=VERTEX_POINT('',#118650) ;
#33728=VERTEX_POINT('',#118654) ;
#33729=VERTEX_POINT('',#118656) ;
#33730=VERTEX_POINT('',#118660) ;
#33731=VERTEX_POINT('',#118662) ;
#33732=VERTEX_POINT('',#118666) ;
#33733=VERTEX_POINT('',#118668) ;
#33734=VERTEX_POINT('',#118672) ;
#33735=VERTEX_POINT('',#118674) ;
#33736=VERTEX_POINT('',#118678) ;
#33737=VERTEX_POINT('',#118680) ;
#33738=VERTEX_POINT('',#118684) ;
#33739=VERTEX_POINT('',#118686) ;
#33740=VERTEX_POINT('',#118690) ;
#33741=VERTEX_POINT('',#118692) ;
#33742=VERTEX_POINT('',#118696) ;
#33743=VERTEX_POINT('',#118698) ;
#33744=VERTEX_POINT('',#118702) ;
#33745=VERTEX_POINT('',#118704) ;
#33746=VERTEX_POINT('',#118711) ;
#33747=VERTEX_POINT('',#118712) ;
#33748=VERTEX_POINT('',#118714) ;
#33749=VERTEX_POINT('',#118716) ;
#33750=VERTEX_POINT('',#118718) ;
#33751=VERTEX_POINT('',#118720) ;
#33752=VERTEX_POINT('',#118722) ;
#33753=VERTEX_POINT('',#118724) ;
#33754=VERTEX_POINT('',#118726) ;
#33755=VERTEX_POINT('',#118728) ;
#33756=VERTEX_POINT('',#118730) ;
#33757=VERTEX_POINT('',#118732) ;
#33758=VERTEX_POINT('',#118734) ;
#33759=VERTEX_POINT('',#118736) ;
#33760=VERTEX_POINT('',#118738) ;
#33761=VERTEX_POINT('',#118740) ;
#33762=VERTEX_POINT('',#118743) ;
#33763=VERTEX_POINT('',#118747) ;
#33764=VERTEX_POINT('',#118748) ;
#33765=VERTEX_POINT('',#118750) ;
#33766=VERTEX_POINT('',#118752) ;
#33767=VERTEX_POINT('',#118756) ;
#33768=VERTEX_POINT('',#118758) ;
#33769=VERTEX_POINT('',#118762) ;
#33770=VERTEX_POINT('',#118764) ;
#33771=VERTEX_POINT('',#118768) ;
#33772=VERTEX_POINT('',#118770) ;
#33773=VERTEX_POINT('',#118774) ;
#33774=VERTEX_POINT('',#118776) ;
#33775=VERTEX_POINT('',#118781) ;
#33776=VERTEX_POINT('',#118785) ;
#33777=VERTEX_POINT('',#118792) ;
#33778=VERTEX_POINT('',#118794) ;
#33779=VERTEX_POINT('',#118798) ;
#33780=VERTEX_POINT('',#118800) ;
#33781=VERTEX_POINT('',#118804) ;
#33782=VERTEX_POINT('',#118806) ;
#33783=VERTEX_POINT('',#118810) ;
#33784=VERTEX_POINT('',#118812) ;
#33785=VERTEX_POINT('',#118816) ;
#33786=VERTEX_POINT('',#118818) ;
#33787=VERTEX_POINT('',#118822) ;
#33788=VERTEX_POINT('',#118824) ;
#33789=VERTEX_POINT('',#118828) ;
#33790=VERTEX_POINT('',#118830) ;
#33791=VERTEX_POINT('',#118834) ;
#33792=VERTEX_POINT('',#118836) ;
#33793=VERTEX_POINT('',#118840) ;
#33794=VERTEX_POINT('',#118842) ;
#33795=VERTEX_POINT('',#118846) ;
#33796=VERTEX_POINT('',#118848) ;
#33797=VERTEX_POINT('',#118852) ;
#33798=VERTEX_POINT('',#118854) ;
#33799=VERTEX_POINT('',#118858) ;
#33800=VERTEX_POINT('',#118860) ;
#33801=VERTEX_POINT('',#118864) ;
#33802=VERTEX_POINT('',#118866) ;
#33803=VERTEX_POINT('',#118870) ;
#33804=VERTEX_POINT('',#118872) ;
#33805=VERTEX_POINT('',#118876) ;
#33806=VERTEX_POINT('',#118878) ;
#33807=VERTEX_POINT('',#118882) ;
#33808=VERTEX_POINT('',#118884) ;
#33809=VERTEX_POINT('',#118888) ;
#33810=VERTEX_POINT('',#118890) ;
#33811=VERTEX_POINT('',#118894) ;
#33812=VERTEX_POINT('',#118896) ;
#33813=VERTEX_POINT('',#118903) ;
#33814=VERTEX_POINT('',#118904) ;
#33815=VERTEX_POINT('',#118906) ;
#33816=VERTEX_POINT('',#118908) ;
#33817=VERTEX_POINT('',#118910) ;
#33818=VERTEX_POINT('',#118912) ;
#33819=VERTEX_POINT('',#118914) ;
#33820=VERTEX_POINT('',#118916) ;
#33821=VERTEX_POINT('',#118918) ;
#33822=VERTEX_POINT('',#118920) ;
#33823=VERTEX_POINT('',#118922) ;
#33824=VERTEX_POINT('',#118924) ;
#33825=VERTEX_POINT('',#118926) ;
#33826=VERTEX_POINT('',#118928) ;
#33827=VERTEX_POINT('',#118930) ;
#33828=VERTEX_POINT('',#118932) ;
#33829=VERTEX_POINT('',#118935) ;
#33830=VERTEX_POINT('',#118939) ;
#33831=VERTEX_POINT('',#118940) ;
#33832=VERTEX_POINT('',#118942) ;
#33833=VERTEX_POINT('',#118944) ;
#33834=VERTEX_POINT('',#118946) ;
#33835=VERTEX_POINT('',#118948) ;
#33836=VERTEX_POINT('',#118950) ;
#33837=VERTEX_POINT('',#118952) ;
#33838=VERTEX_POINT('',#118956) ;
#33839=VERTEX_POINT('',#118957) ;
#33840=VERTEX_POINT('',#118959) ;
#33841=VERTEX_POINT('',#118961) ;
#33842=VERTEX_POINT('',#118963) ;
#33843=VERTEX_POINT('',#118965) ;
#33844=VERTEX_POINT('',#118967) ;
#33845=VERTEX_POINT('',#118969) ;
#33846=VERTEX_POINT('',#118973) ;
#33847=VERTEX_POINT('',#118974) ;
#33848=VERTEX_POINT('',#118976) ;
#33849=VERTEX_POINT('',#118978) ;
#33850=VERTEX_POINT('',#118980) ;
#33851=VERTEX_POINT('',#118982) ;
#33852=VERTEX_POINT('',#118984) ;
#33853=VERTEX_POINT('',#118986) ;
#33854=VERTEX_POINT('',#118990) ;
#33855=VERTEX_POINT('',#118991) ;
#33856=VERTEX_POINT('',#118993) ;
#33857=VERTEX_POINT('',#118995) ;
#33858=VERTEX_POINT('',#118997) ;
#33859=VERTEX_POINT('',#118999) ;
#33860=VERTEX_POINT('',#119001) ;
#33861=VERTEX_POINT('',#119003) ;
#33862=VERTEX_POINT('',#119007) ;
#33863=VERTEX_POINT('',#119008) ;
#33864=VERTEX_POINT('',#119010) ;
#33865=VERTEX_POINT('',#119012) ;
#33866=VERTEX_POINT('',#119014) ;
#33867=VERTEX_POINT('',#119016) ;
#33868=VERTEX_POINT('',#119018) ;
#33869=VERTEX_POINT('',#119020) ;
#33870=VERTEX_POINT('',#119024) ;
#33871=VERTEX_POINT('',#119025) ;
#33872=VERTEX_POINT('',#119027) ;
#33873=VERTEX_POINT('',#119029) ;
#33874=VERTEX_POINT('',#119031) ;
#33875=VERTEX_POINT('',#119033) ;
#33876=VERTEX_POINT('',#119035) ;
#33877=VERTEX_POINT('',#119037) ;
#33878=VERTEX_POINT('',#119041) ;
#33879=VERTEX_POINT('',#119042) ;
#33880=VERTEX_POINT('',#119044) ;
#33881=VERTEX_POINT('',#119046) ;
#33882=VERTEX_POINT('',#119048) ;
#33883=VERTEX_POINT('',#119050) ;
#33884=VERTEX_POINT('',#119052) ;
#33885=VERTEX_POINT('',#119054) ;
#33886=VERTEX_POINT('',#119058) ;
#33887=VERTEX_POINT('',#119059) ;
#33888=VERTEX_POINT('',#119061) ;
#33889=VERTEX_POINT('',#119063) ;
#33890=VERTEX_POINT('',#119065) ;
#33891=VERTEX_POINT('',#119067) ;
#33892=VERTEX_POINT('',#119069) ;
#33893=VERTEX_POINT('',#119071) ;
#33894=VERTEX_POINT('',#119075) ;
#33895=VERTEX_POINT('',#119076) ;
#33896=VERTEX_POINT('',#119078) ;
#33897=VERTEX_POINT('',#119080) ;
#33898=VERTEX_POINT('',#119082) ;
#33899=VERTEX_POINT('',#119084) ;
#33900=VERTEX_POINT('',#119086) ;
#33901=VERTEX_POINT('',#119088) ;
#33902=VERTEX_POINT('',#119098) ;
#33903=VERTEX_POINT('',#119108) ;
#33904=VERTEX_POINT('',#119119) ;
#33905=VERTEX_POINT('',#119151) ;
#33906=VERTEX_POINT('',#119198) ;
#33907=VERTEX_POINT('',#119216) ;
#33908=VERTEX_POINT('',#119230) ;
#33909=VERTEX_POINT('',#119245) ;
#33910=VERTEX_POINT('',#119802) ;
#33911=VERTEX_POINT('',#119812) ;
#33912=VERTEX_POINT('',#119823) ;
#33913=VERTEX_POINT('',#119855) ;
#33914=VERTEX_POINT('',#119902) ;
#33915=VERTEX_POINT('',#119920) ;
#33916=VERTEX_POINT('',#119934) ;
#33917=VERTEX_POINT('',#119949) ;
#33918=VERTEX_POINT('',#120029) ;
#33919=VERTEX_POINT('',#120039) ;
#33920=VERTEX_POINT('',#120050) ;
#33921=VERTEX_POINT('',#120082) ;
#33922=VERTEX_POINT('',#120129) ;
#33923=VERTEX_POINT('',#120147) ;
#33924=VERTEX_POINT('',#120161) ;
#33925=VERTEX_POINT('',#120176) ;
#33926=VERTEX_POINT('',#120256) ;
#33927=VERTEX_POINT('',#120266) ;
#33928=VERTEX_POINT('',#120277) ;
#33929=VERTEX_POINT('',#120309) ;
#33930=VERTEX_POINT('',#120356) ;
#33931=VERTEX_POINT('',#120374) ;
#33932=VERTEX_POINT('',#120388) ;
#33933=VERTEX_POINT('',#120403) ;
#33934=VERTEX_POINT('',#120483) ;
#33935=VERTEX_POINT('',#120493) ;
#33936=VERTEX_POINT('',#120504) ;
#33937=VERTEX_POINT('',#120536) ;
#33938=VERTEX_POINT('',#120583) ;
#33939=VERTEX_POINT('',#120601) ;
#33940=VERTEX_POINT('',#120615) ;
#33941=VERTEX_POINT('',#120630) ;
#33942=VERTEX_POINT('',#120710) ;
#33943=VERTEX_POINT('',#120720) ;
#33944=VERTEX_POINT('',#120731) ;
#33945=VERTEX_POINT('',#120763) ;
#33946=VERTEX_POINT('',#120810) ;
#33947=VERTEX_POINT('',#120828) ;
#33948=VERTEX_POINT('',#120842) ;
#33949=VERTEX_POINT('',#120857) ;
#33950=VERTEX_POINT('',#120937) ;
#33951=VERTEX_POINT('',#120947) ;
#33952=VERTEX_POINT('',#120958) ;
#33953=VERTEX_POINT('',#120990) ;
#33954=VERTEX_POINT('',#121037) ;
#33955=VERTEX_POINT('',#121055) ;
#33956=VERTEX_POINT('',#121069) ;
#33957=VERTEX_POINT('',#121084) ;
#33958=VERTEX_POINT('',#121164) ;
#33959=VERTEX_POINT('',#121174) ;
#33960=VERTEX_POINT('',#121185) ;
#33961=VERTEX_POINT('',#121217) ;
#33962=VERTEX_POINT('',#121264) ;
#33963=VERTEX_POINT('',#121282) ;
#33964=VERTEX_POINT('',#121296) ;
#33965=VERTEX_POINT('',#121311) ;
#33966=VERTEX_POINT('',#121391) ;
#33967=VERTEX_POINT('',#121401) ;
#33968=VERTEX_POINT('',#121412) ;
#33969=VERTEX_POINT('',#121444) ;
#33970=VERTEX_POINT('',#121491) ;
#33971=VERTEX_POINT('',#121509) ;
#33972=VERTEX_POINT('',#121523) ;
#33973=VERTEX_POINT('',#121538) ;
#33974=VERTEX_POINT('',#121612) ;
#33975=VERTEX_POINT('',#121613) ;
#33976=VERTEX_POINT('',#121615) ;
#33977=VERTEX_POINT('',#121617) ;
#33978=VERTEX_POINT('',#121621) ;
#33979=VERTEX_POINT('',#121622) ;
#33980=VERTEX_POINT('',#121624) ;
#33981=VERTEX_POINT('',#121626) ;
#33982=VERTEX_POINT('',#121630) ;
#33983=VERTEX_POINT('',#121631) ;
#33984=VERTEX_POINT('',#121633) ;
#33985=VERTEX_POINT('',#121635) ;
#33986=VERTEX_POINT('',#121639) ;
#33987=VERTEX_POINT('',#121640) ;
#33988=VERTEX_POINT('',#121642) ;
#33989=VERTEX_POINT('',#121644) ;
#33990=VERTEX_POINT('',#121648) ;
#33991=VERTEX_POINT('',#121649) ;
#33992=VERTEX_POINT('',#121651) ;
#33993=VERTEX_POINT('',#121653) ;
#33994=VERTEX_POINT('',#121657) ;
#33995=VERTEX_POINT('',#121658) ;
#33996=VERTEX_POINT('',#121661) ;
#33997=VERTEX_POINT('',#121663) ;
#33998=VERTEX_POINT('',#121667) ;
#33999=VERTEX_POINT('',#121668) ;
#34000=VERTEX_POINT('',#121671) ;
#34001=VERTEX_POINT('',#121673) ;
#34002=VERTEX_POINT('',#121683) ;
#34003=VERTEX_POINT('',#121684) ;
#34004=VERTEX_POINT('',#121686) ;
#34005=VERTEX_POINT('',#121688) ;
#34006=VERTEX_POINT('',#121692) ;
#34007=VERTEX_POINT('',#121693) ;
#34008=VERTEX_POINT('',#121698) ;
#34009=VERTEX_POINT('',#121700) ;
#34010=VERTEX_POINT('',#121704) ;
#34011=VERTEX_POINT('',#121705) ;
#34012=VERTEX_POINT('',#121707) ;
#34013=VERTEX_POINT('',#121709) ;
#34014=VERTEX_POINT('',#121713) ;
#34015=VERTEX_POINT('',#121714) ;
#34016=VERTEX_POINT('',#121716) ;
#34017=VERTEX_POINT('',#121718) ;
#34018=VERTEX_POINT('',#121722) ;
#34019=VERTEX_POINT('',#121723) ;
#34020=VERTEX_POINT('',#121728) ;
#34021=VERTEX_POINT('',#121730) ;
#34022=VERTEX_POINT('',#121734) ;
#34023=VERTEX_POINT('',#121735) ;
#34024=VERTEX_POINT('',#121737) ;
#34025=VERTEX_POINT('',#121739) ;
#34026=VERTEX_POINT('',#121743) ;
#34027=VERTEX_POINT('',#121744) ;
#34028=VERTEX_POINT('',#121746) ;
#34029=VERTEX_POINT('',#121748) ;
#34030=VERTEX_POINT('',#121752) ;
#34031=VERTEX_POINT('',#121753) ;
#34032=VERTEX_POINT('',#121755) ;
#34033=VERTEX_POINT('',#121757) ;
#34034=VERTEX_POINT('',#121761) ;
#34035=VERTEX_POINT('',#121762) ;
#34036=VERTEX_POINT('',#121764) ;
#34037=VERTEX_POINT('',#121766) ;
#34038=VERTEX_POINT('',#121770) ;
#34039=VERTEX_POINT('',#121771) ;
#34040=VERTEX_POINT('',#121773) ;
#34041=VERTEX_POINT('',#121775) ;
#34042=VERTEX_POINT('',#121779) ;
#34043=VERTEX_POINT('',#121780) ;
#34044=VERTEX_POINT('',#121783) ;
#34045=VERTEX_POINT('',#121785) ;
#34046=VERTEX_POINT('',#121789) ;
#34047=VERTEX_POINT('',#121790) ;
#34048=VERTEX_POINT('',#121793) ;
#34049=VERTEX_POINT('',#121795) ;
#34050=VERTEX_POINT('',#121805) ;
#34051=VERTEX_POINT('',#121806) ;
#34052=VERTEX_POINT('',#121808) ;
#34053=VERTEX_POINT('',#121810) ;
#34054=VERTEX_POINT('',#121814) ;
#34055=VERTEX_POINT('',#121815) ;
#34056=VERTEX_POINT('',#121820) ;
#34057=VERTEX_POINT('',#121822) ;
#34058=VERTEX_POINT('',#121826) ;
#34059=VERTEX_POINT('',#121827) ;
#34060=VERTEX_POINT('',#121829) ;
#34061=VERTEX_POINT('',#121831) ;
#34062=VERTEX_POINT('',#121835) ;
#34063=VERTEX_POINT('',#121836) ;
#34064=VERTEX_POINT('',#121838) ;
#34065=VERTEX_POINT('',#121840) ;
#34066=VERTEX_POINT('',#121844) ;
#34067=VERTEX_POINT('',#121845) ;
#34068=VERTEX_POINT('',#121850) ;
#34069=VERTEX_POINT('',#121852) ;
#34070=VERTEX_POINT('',#121856) ;
#34071=VERTEX_POINT('',#121857) ;
#34072=VERTEX_POINT('',#121859) ;
#34073=VERTEX_POINT('',#121861) ;
#34074=VERTEX_POINT('',#121865) ;
#34075=VERTEX_POINT('',#121866) ;
#34076=VERTEX_POINT('',#121868) ;
#34077=VERTEX_POINT('',#121870) ;
#34078=VERTEX_POINT('',#121874) ;
#34079=VERTEX_POINT('',#121875) ;
#34080=VERTEX_POINT('',#121877) ;
#34081=VERTEX_POINT('',#121879) ;
#34082=VERTEX_POINT('',#121883) ;
#34083=VERTEX_POINT('',#121884) ;
#34084=VERTEX_POINT('',#121886) ;
#34085=VERTEX_POINT('',#121888) ;
#34086=VERTEX_POINT('',#121892) ;
#34087=VERTEX_POINT('',#121893) ;
#34088=VERTEX_POINT('',#121895) ;
#34089=VERTEX_POINT('',#121897) ;
#34090=VERTEX_POINT('',#121901) ;
#34091=VERTEX_POINT('',#121902) ;
#34092=VERTEX_POINT('',#121905) ;
#34093=VERTEX_POINT('',#121907) ;
#34094=VERTEX_POINT('',#121911) ;
#34095=VERTEX_POINT('',#121912) ;
#34096=VERTEX_POINT('',#121915) ;
#34097=VERTEX_POINT('',#121917) ;
#34098=VERTEX_POINT('',#121927) ;
#34099=VERTEX_POINT('',#121928) ;
#34100=VERTEX_POINT('',#121930) ;
#34101=VERTEX_POINT('',#121932) ;
#34102=VERTEX_POINT('',#121936) ;
#34103=VERTEX_POINT('',#121937) ;
#34104=VERTEX_POINT('',#121942) ;
#34105=VERTEX_POINT('',#121944) ;
#34106=VERTEX_POINT('',#121948) ;
#34107=VERTEX_POINT('',#121949) ;
#34108=VERTEX_POINT('',#121951) ;
#34109=VERTEX_POINT('',#121953) ;
#34110=VERTEX_POINT('',#121957) ;
#34111=VERTEX_POINT('',#121958) ;
#34112=VERTEX_POINT('',#121960) ;
#34113=VERTEX_POINT('',#121962) ;
#34114=VERTEX_POINT('',#121966) ;
#34115=VERTEX_POINT('',#121967) ;
#34116=VERTEX_POINT('',#121972) ;
#34117=VERTEX_POINT('',#121974) ;
#34118=VERTEX_POINT('',#121978) ;
#34119=VERTEX_POINT('',#121979) ;
#34120=VERTEX_POINT('',#121981) ;
#34121=VERTEX_POINT('',#121983) ;
#34122=VERTEX_POINT('',#121987) ;
#34123=VERTEX_POINT('',#121988) ;
#34124=VERTEX_POINT('',#121990) ;
#34125=VERTEX_POINT('',#121992) ;
#34126=VERTEX_POINT('',#121996) ;
#34127=VERTEX_POINT('',#121997) ;
#34128=VERTEX_POINT('',#121999) ;
#34129=VERTEX_POINT('',#122001) ;
#34130=VERTEX_POINT('',#122005) ;
#34131=VERTEX_POINT('',#122006) ;
#34132=VERTEX_POINT('',#122008) ;
#34133=VERTEX_POINT('',#122010) ;
#34134=VERTEX_POINT('',#122014) ;
#34135=VERTEX_POINT('',#122015) ;
#34136=VERTEX_POINT('',#122017) ;
#34137=VERTEX_POINT('',#122019) ;
#34138=VERTEX_POINT('',#122023) ;
#34139=VERTEX_POINT('',#122024) ;
#34140=VERTEX_POINT('',#122027) ;
#34141=VERTEX_POINT('',#122029) ;
#34142=VERTEX_POINT('',#122033) ;
#34143=VERTEX_POINT('',#122034) ;
#34144=VERTEX_POINT('',#122037) ;
#34145=VERTEX_POINT('',#122039) ;
#34146=VERTEX_POINT('',#122049) ;
#34147=VERTEX_POINT('',#122050) ;
#34148=VERTEX_POINT('',#122052) ;
#34149=VERTEX_POINT('',#122054) ;
#34150=VERTEX_POINT('',#122058) ;
#34151=VERTEX_POINT('',#122059) ;
#34152=VERTEX_POINT('',#122064) ;
#34153=VERTEX_POINT('',#122066) ;
#34154=VERTEX_POINT('',#122070) ;
#34155=VERTEX_POINT('',#122071) ;
#34156=VERTEX_POINT('',#122073) ;
#34157=VERTEX_POINT('',#122075) ;
#34158=VERTEX_POINT('',#122079) ;
#34159=VERTEX_POINT('',#122080) ;
#34160=VERTEX_POINT('',#122082) ;
#34161=VERTEX_POINT('',#122084) ;
#34162=VERTEX_POINT('',#122088) ;
#34163=VERTEX_POINT('',#122089) ;
#34164=VERTEX_POINT('',#122094) ;
#34165=VERTEX_POINT('',#122096) ;
#34166=VERTEX_POINT('',#122100) ;
#34167=VERTEX_POINT('',#122101) ;
#34168=VERTEX_POINT('',#122103) ;
#34169=VERTEX_POINT('',#122105) ;
#34170=VERTEX_POINT('',#122109) ;
#34171=VERTEX_POINT('',#122110) ;
#34172=VERTEX_POINT('',#122112) ;
#34173=VERTEX_POINT('',#122114) ;
#34174=VERTEX_POINT('',#122118) ;
#34175=VERTEX_POINT('',#122119) ;
#34176=VERTEX_POINT('',#122121) ;
#34177=VERTEX_POINT('',#122123) ;
#34178=VERTEX_POINT('',#122127) ;
#34179=VERTEX_POINT('',#122128) ;
#34180=VERTEX_POINT('',#122130) ;
#34181=VERTEX_POINT('',#122132) ;
#34182=VERTEX_POINT('',#122136) ;
#34183=VERTEX_POINT('',#122137) ;
#34184=VERTEX_POINT('',#122139) ;
#34185=VERTEX_POINT('',#122141) ;
#34186=VERTEX_POINT('',#122145) ;
#34187=VERTEX_POINT('',#122146) ;
#34188=VERTEX_POINT('',#122149) ;
#34189=VERTEX_POINT('',#122151) ;
#34190=VERTEX_POINT('',#122155) ;
#34191=VERTEX_POINT('',#122156) ;
#34192=VERTEX_POINT('',#122159) ;
#34193=VERTEX_POINT('',#122161) ;
#34194=VERTEX_POINT('',#122171) ;
#34195=VERTEX_POINT('',#122172) ;
#34196=VERTEX_POINT('',#122174) ;
#34197=VERTEX_POINT('',#122176) ;
#34198=VERTEX_POINT('',#122180) ;
#34199=VERTEX_POINT('',#122181) ;
#34200=VERTEX_POINT('',#122186) ;
#34201=VERTEX_POINT('',#122188) ;
#34202=VERTEX_POINT('',#122192) ;
#34203=VERTEX_POINT('',#122193) ;
#34204=VERTEX_POINT('',#122195) ;
#34205=VERTEX_POINT('',#122197) ;
#34206=VERTEX_POINT('',#122201) ;
#34207=VERTEX_POINT('',#122202) ;
#34208=VERTEX_POINT('',#122204) ;
#34209=VERTEX_POINT('',#122206) ;
#34210=VERTEX_POINT('',#122210) ;
#34211=VERTEX_POINT('',#122211) ;
#34212=VERTEX_POINT('',#122216) ;
#34213=VERTEX_POINT('',#122218) ;
#34214=VERTEX_POINT('',#122222) ;
#34215=VERTEX_POINT('',#122223) ;
#34216=VERTEX_POINT('',#122225) ;
#34217=VERTEX_POINT('',#122227) ;
#34218=VERTEX_POINT('',#122231) ;
#34219=VERTEX_POINT('',#122232) ;
#34220=VERTEX_POINT('',#122234) ;
#34221=VERTEX_POINT('',#122236) ;
#34222=VERTEX_POINT('',#122240) ;
#34223=VERTEX_POINT('',#122241) ;
#34224=VERTEX_POINT('',#122243) ;
#34225=VERTEX_POINT('',#122245) ;
#34226=VERTEX_POINT('',#122249) ;
#34227=VERTEX_POINT('',#122250) ;
#34228=VERTEX_POINT('',#122252) ;
#34229=VERTEX_POINT('',#122254) ;
#34230=VERTEX_POINT('',#122258) ;
#34231=VERTEX_POINT('',#122259) ;
#34232=VERTEX_POINT('',#122261) ;
#34233=VERTEX_POINT('',#122263) ;
#34234=VERTEX_POINT('',#122267) ;
#34235=VERTEX_POINT('',#122268) ;
#34236=VERTEX_POINT('',#122271) ;
#34237=VERTEX_POINT('',#122273) ;
#34238=VERTEX_POINT('',#122277) ;
#34239=VERTEX_POINT('',#122278) ;
#34240=VERTEX_POINT('',#122281) ;
#34241=VERTEX_POINT('',#122283) ;
#34242=VERTEX_POINT('',#122293) ;
#34243=VERTEX_POINT('',#122294) ;
#34244=VERTEX_POINT('',#122296) ;
#34245=VERTEX_POINT('',#122298) ;
#34246=VERTEX_POINT('',#122302) ;
#34247=VERTEX_POINT('',#122303) ;
#34248=VERTEX_POINT('',#122308) ;
#34249=VERTEX_POINT('',#122310) ;
#34250=VERTEX_POINT('',#122314) ;
#34251=VERTEX_POINT('',#122315) ;
#34252=VERTEX_POINT('',#122317) ;
#34253=VERTEX_POINT('',#122319) ;
#34254=VERTEX_POINT('',#122323) ;
#34255=VERTEX_POINT('',#122324) ;
#34256=VERTEX_POINT('',#122326) ;
#34257=VERTEX_POINT('',#122328) ;
#34258=VERTEX_POINT('',#122332) ;
#34259=VERTEX_POINT('',#122333) ;
#34260=VERTEX_POINT('',#122338) ;
#34261=VERTEX_POINT('',#122340) ;
#34262=VERTEX_POINT('',#122344) ;
#34263=VERTEX_POINT('',#122345) ;
#34264=VERTEX_POINT('',#122347) ;
#34265=VERTEX_POINT('',#122349) ;
#34266=VERTEX_POINT('',#122353) ;
#34267=VERTEX_POINT('',#122354) ;
#34268=VERTEX_POINT('',#122356) ;
#34269=VERTEX_POINT('',#122358) ;
#34270=VERTEX_POINT('',#122362) ;
#34271=VERTEX_POINT('',#122363) ;
#34272=VERTEX_POINT('',#122365) ;
#34273=VERTEX_POINT('',#122367) ;
#34274=VERTEX_POINT('',#122371) ;
#34275=VERTEX_POINT('',#122372) ;
#34276=VERTEX_POINT('',#122374) ;
#34277=VERTEX_POINT('',#122376) ;
#34278=VERTEX_POINT('',#122380) ;
#34279=VERTEX_POINT('',#122381) ;
#34280=VERTEX_POINT('',#122383) ;
#34281=VERTEX_POINT('',#122385) ;
#34282=VERTEX_POINT('',#122389) ;
#34283=VERTEX_POINT('',#122390) ;
#34284=VERTEX_POINT('',#122393) ;
#34285=VERTEX_POINT('',#122395) ;
#34286=VERTEX_POINT('',#122399) ;
#34287=VERTEX_POINT('',#122400) ;
#34288=VERTEX_POINT('',#122403) ;
#34289=VERTEX_POINT('',#122405) ;
#34290=VERTEX_POINT('',#122415) ;
#34291=VERTEX_POINT('',#122416) ;
#34292=VERTEX_POINT('',#122418) ;
#34293=VERTEX_POINT('',#122420) ;
#34294=VERTEX_POINT('',#122424) ;
#34295=VERTEX_POINT('',#122425) ;
#34296=VERTEX_POINT('',#122430) ;
#34297=VERTEX_POINT('',#122432) ;
#34298=VERTEX_POINT('',#122436) ;
#34299=VERTEX_POINT('',#122437) ;
#34300=VERTEX_POINT('',#122439) ;
#34301=VERTEX_POINT('',#122441) ;
#34302=VERTEX_POINT('',#122445) ;
#34303=VERTEX_POINT('',#122446) ;
#34304=VERTEX_POINT('',#122448) ;
#34305=VERTEX_POINT('',#122450) ;
#34306=VERTEX_POINT('',#122454) ;
#34307=VERTEX_POINT('',#122455) ;
#34308=VERTEX_POINT('',#122460) ;
#34309=VERTEX_POINT('',#122462) ;
#34310=VERTEX_POINT('',#122466) ;
#34311=VERTEX_POINT('',#122467) ;
#34312=VERTEX_POINT('',#122469) ;
#34313=VERTEX_POINT('',#122471) ;
#34314=VERTEX_POINT('',#122475) ;
#34315=VERTEX_POINT('',#122476) ;
#34316=VERTEX_POINT('',#122478) ;
#34317=VERTEX_POINT('',#122480) ;
#34318=VERTEX_POINT('',#122484) ;
#34319=VERTEX_POINT('',#122485) ;
#34320=VERTEX_POINT('',#122487) ;
#34321=VERTEX_POINT('',#122489) ;
#34322=VERTEX_POINT('',#122493) ;
#34323=VERTEX_POINT('',#122494) ;
#34324=VERTEX_POINT('',#122496) ;
#34325=VERTEX_POINT('',#122498) ;
#34326=VERTEX_POINT('',#122502) ;
#34327=VERTEX_POINT('',#122503) ;
#34328=VERTEX_POINT('',#122505) ;
#34329=VERTEX_POINT('',#122507) ;
#34330=VERTEX_POINT('',#122511) ;
#34331=VERTEX_POINT('',#122512) ;
#34332=VERTEX_POINT('',#122515) ;
#34333=VERTEX_POINT('',#122517) ;
#34334=VERTEX_POINT('',#122521) ;
#34335=VERTEX_POINT('',#122522) ;
#34336=VERTEX_POINT('',#122525) ;
#34337=VERTEX_POINT('',#122527) ;
#34338=VERTEX_POINT('',#122537) ;
#34339=VERTEX_POINT('',#122538) ;
#34340=VERTEX_POINT('',#122540) ;
#34341=VERTEX_POINT('',#122542) ;
#34342=VERTEX_POINT('',#122546) ;
#34343=VERTEX_POINT('',#122547) ;
#34344=VERTEX_POINT('',#122552) ;
#34345=VERTEX_POINT('',#122554) ;
#34346=VERTEX_POINT('',#122558) ;
#34347=VERTEX_POINT('',#122559) ;
#34348=VERTEX_POINT('',#122561) ;
#34349=VERTEX_POINT('',#122563) ;
#34350=VERTEX_POINT('',#122567) ;
#34351=VERTEX_POINT('',#122568) ;
#34352=VERTEX_POINT('',#122570) ;
#34353=VERTEX_POINT('',#122572) ;
#34354=VERTEX_POINT('',#122576) ;
#34355=VERTEX_POINT('',#122577) ;
#34356=VERTEX_POINT('',#122582) ;
#34357=VERTEX_POINT('',#122584) ;
#34358=VERTEX_POINT('',#122588) ;
#34359=VERTEX_POINT('',#122589) ;
#34360=VERTEX_POINT('',#122591) ;
#34361=VERTEX_POINT('',#122593) ;
#34362=VERTEX_POINT('',#122597) ;
#34363=VERTEX_POINT('',#122598) ;
#34364=VERTEX_POINT('',#122600) ;
#34365=VERTEX_POINT('',#122602) ;
#34366=VERTEX_POINT('',#122606) ;
#34367=VERTEX_POINT('',#122607) ;
#34368=VERTEX_POINT('',#122609) ;
#34369=VERTEX_POINT('',#122611) ;
#34370=VERTEX_POINT('',#122615) ;
#34371=VERTEX_POINT('',#122616) ;
#34372=VERTEX_POINT('',#122618) ;
#34373=VERTEX_POINT('',#122620) ;
#34374=VERTEX_POINT('',#122624) ;
#34375=VERTEX_POINT('',#122625) ;
#34376=VERTEX_POINT('',#122627) ;
#34377=VERTEX_POINT('',#122629) ;
#34378=VERTEX_POINT('',#122633) ;
#34379=VERTEX_POINT('',#122634) ;
#34380=VERTEX_POINT('',#122637) ;
#34381=VERTEX_POINT('',#122639) ;
#34382=VERTEX_POINT('',#122643) ;
#34383=VERTEX_POINT('',#122644) ;
#34384=VERTEX_POINT('',#122647) ;
#34385=VERTEX_POINT('',#122649) ;
#34386=VERTEX_POINT('',#122659) ;
#34387=VERTEX_POINT('',#122660) ;
#34388=VERTEX_POINT('',#122662) ;
#34389=VERTEX_POINT('',#122664) ;
#34390=VERTEX_POINT('',#122668) ;
#34391=VERTEX_POINT('',#122669) ;
#34392=VERTEX_POINT('',#122674) ;
#34393=VERTEX_POINT('',#122676) ;
#34394=VERTEX_POINT('',#122680) ;
#34395=VERTEX_POINT('',#122681) ;
#34396=VERTEX_POINT('',#122683) ;
#34397=VERTEX_POINT('',#122685) ;
#34398=VERTEX_POINT('',#122689) ;
#34399=VERTEX_POINT('',#122690) ;
#34400=VERTEX_POINT('',#122692) ;
#34401=VERTEX_POINT('',#122694) ;
#34402=VERTEX_POINT('',#122698) ;
#34403=VERTEX_POINT('',#122699) ;
#34404=VERTEX_POINT('',#122704) ;
#34405=VERTEX_POINT('',#122706) ;
#34406=VERTEX_POINT('',#122710) ;
#34407=VERTEX_POINT('',#122711) ;
#34408=VERTEX_POINT('',#122713) ;
#34409=VERTEX_POINT('',#122715) ;
#34410=VERTEX_POINT('',#122719) ;
#34411=VERTEX_POINT('',#122720) ;
#34412=VERTEX_POINT('',#122722) ;
#34413=VERTEX_POINT('',#122724) ;
#34414=VERTEX_POINT('',#122728) ;
#34415=VERTEX_POINT('',#122729) ;
#34416=VERTEX_POINT('',#122731) ;
#34417=VERTEX_POINT('',#122733) ;
#34418=VERTEX_POINT('',#122737) ;
#34419=VERTEX_POINT('',#122738) ;
#34420=VERTEX_POINT('',#122740) ;
#34421=VERTEX_POINT('',#122742) ;
#34422=VERTEX_POINT('',#122746) ;
#34423=VERTEX_POINT('',#122747) ;
#34424=VERTEX_POINT('',#122749) ;
#34425=VERTEX_POINT('',#122751) ;
#34426=VERTEX_POINT('',#122755) ;
#34427=VERTEX_POINT('',#122756) ;
#34428=VERTEX_POINT('',#122758) ;
#34429=VERTEX_POINT('',#122760) ;
#34430=VERTEX_POINT('',#122764) ;
#34431=VERTEX_POINT('',#122765) ;
#34432=VERTEX_POINT('',#122767) ;
#34433=VERTEX_POINT('',#122769) ;
#34434=VERTEX_POINT('',#122773) ;
#34435=VERTEX_POINT('',#122774) ;
#34436=VERTEX_POINT('',#122776) ;
#34437=VERTEX_POINT('',#122778) ;
#34438=VERTEX_POINT('',#122782) ;
#34439=VERTEX_POINT('',#122783) ;
#34440=VERTEX_POINT('',#122785) ;
#34441=VERTEX_POINT('',#122787) ;
#34442=VERTEX_POINT('',#122791) ;
#34443=VERTEX_POINT('',#122792) ;
#34444=VERTEX_POINT('',#122794) ;
#34445=VERTEX_POINT('',#122796) ;
#34446=VERTEX_POINT('',#122800) ;
#34447=VERTEX_POINT('',#122801) ;
#34448=VERTEX_POINT('',#122803) ;
#34449=VERTEX_POINT('',#122805) ;
#34450=VERTEX_POINT('',#122809) ;
#34451=VERTEX_POINT('',#122810) ;
#34452=VERTEX_POINT('',#122812) ;
#34453=VERTEX_POINT('',#122814) ;
#34454=VERTEX_POINT('',#122818) ;
#34455=VERTEX_POINT('',#122819) ;
#34456=VERTEX_POINT('',#122821) ;
#34457=VERTEX_POINT('',#122823) ;
#34458=VERTEX_POINT('',#122827) ;
#34459=VERTEX_POINT('',#122828) ;
#34460=VERTEX_POINT('',#122830) ;
#34461=VERTEX_POINT('',#122832) ;
#34462=VERTEX_POINT('',#122836) ;
#34463=VERTEX_POINT('',#122837) ;
#34464=VERTEX_POINT('',#122839) ;
#34465=VERTEX_POINT('',#122841) ;
#34466=VERTEX_POINT('',#122845) ;
#34467=VERTEX_POINT('',#122846) ;
#34468=VERTEX_POINT('',#122848) ;
#34469=VERTEX_POINT('',#122850) ;
#34470=VERTEX_POINT('',#122854) ;
#34471=VERTEX_POINT('',#122855) ;
#34472=VERTEX_POINT('',#122857) ;
#34473=VERTEX_POINT('',#122859) ;
#34474=VERTEX_POINT('',#122863) ;
#34475=VERTEX_POINT('',#122864) ;
#34476=VERTEX_POINT('',#122866) ;
#34477=VERTEX_POINT('',#122868) ;
#34478=VERTEX_POINT('',#122872) ;
#34479=VERTEX_POINT('',#122873) ;
#34480=VERTEX_POINT('',#122875) ;
#34481=VERTEX_POINT('',#122877) ;
#34482=VERTEX_POINT('',#122881) ;
#34483=VERTEX_POINT('',#122882) ;
#34484=VERTEX_POINT('',#122884) ;
#34485=VERTEX_POINT('',#122886) ;
#34486=VERTEX_POINT('',#122890) ;
#34487=VERTEX_POINT('',#122891) ;
#34488=VERTEX_POINT('',#122893) ;
#34489=VERTEX_POINT('',#122895) ;
#34490=VERTEX_POINT('',#122899) ;
#34491=VERTEX_POINT('',#122900) ;
#34492=VERTEX_POINT('',#122902) ;
#34493=VERTEX_POINT('',#122904) ;
#34494=VERTEX_POINT('',#122908) ;
#34495=VERTEX_POINT('',#122909) ;
#34496=VERTEX_POINT('',#122911) ;
#34497=VERTEX_POINT('',#122913) ;
#34498=VERTEX_POINT('',#122917) ;
#34499=VERTEX_POINT('',#122918) ;
#34500=VERTEX_POINT('',#122920) ;
#34501=VERTEX_POINT('',#122922) ;
#34502=VERTEX_POINT('',#122926) ;
#34503=VERTEX_POINT('',#122927) ;
#34504=VERTEX_POINT('',#122929) ;
#34505=VERTEX_POINT('',#122931) ;
#34506=VERTEX_POINT('',#122935) ;
#34507=VERTEX_POINT('',#122936) ;
#34508=VERTEX_POINT('',#122938) ;
#34509=VERTEX_POINT('',#122940) ;
#34510=VERTEX_POINT('',#122944) ;
#34511=VERTEX_POINT('',#122945) ;
#34512=VERTEX_POINT('',#122947) ;
#34513=VERTEX_POINT('',#122949) ;
#34514=VERTEX_POINT('',#122953) ;
#34515=VERTEX_POINT('',#122954) ;
#34516=VERTEX_POINT('',#122956) ;
#34517=VERTEX_POINT('',#122958) ;
#34518=VERTEX_POINT('',#122962) ;
#34519=VERTEX_POINT('',#122963) ;
#34520=VERTEX_POINT('',#122965) ;
#34521=VERTEX_POINT('',#122967) ;
#34522=VERTEX_POINT('',#122971) ;
#34523=VERTEX_POINT('',#122972) ;
#34524=VERTEX_POINT('',#122974) ;
#34525=VERTEX_POINT('',#122976) ;
#34526=VERTEX_POINT('',#122980) ;
#34527=VERTEX_POINT('',#122981) ;
#34528=VERTEX_POINT('',#122983) ;
#34529=VERTEX_POINT('',#122985) ;
#34530=VERTEX_POINT('',#122989) ;
#34531=VERTEX_POINT('',#122990) ;
#34532=VERTEX_POINT('',#122992) ;
#34533=VERTEX_POINT('',#122994) ;
#34534=VERTEX_POINT('',#122998) ;
#34535=VERTEX_POINT('',#122999) ;
#34536=VERTEX_POINT('',#123001) ;
#34537=VERTEX_POINT('',#123003) ;
#34538=VERTEX_POINT('',#123007) ;
#34539=VERTEX_POINT('',#123008) ;
#34540=VERTEX_POINT('',#123010) ;
#34541=VERTEX_POINT('',#123012) ;
#34542=VERTEX_POINT('',#123016) ;
#34543=VERTEX_POINT('',#123017) ;
#34544=VERTEX_POINT('',#123019) ;
#34545=VERTEX_POINT('',#123021) ;
#34546=VERTEX_POINT('',#123025) ;
#34547=VERTEX_POINT('',#123026) ;
#34548=VERTEX_POINT('',#123028) ;
#34549=VERTEX_POINT('',#123030) ;
#39088=EDGE_CURVE('',#31998,#31998,#26857,.T.) ;
#39089=EDGE_CURVE('',#31998,#31999,#26858,.T.) ;
#39090=EDGE_CURVE('',#32000,#31999,#26859,.T.) ;
#39091=EDGE_CURVE('',#31999,#32000,#26860,.T.) ;
#39092=EDGE_CURVE('',#32001,#32001,#26861,.T.) ;
#39093=EDGE_CURVE('',#32001,#32002,#26862,.T.) ;
#39094=EDGE_CURVE('',#32002,#32002,#26863,.T.) ;
#39095=EDGE_CURVE('',#32003,#32004,#26864,.T.) ;
#39096=EDGE_CURVE('',#32005,#32003,#26865,.T.) ;
#39097=EDGE_CURVE('',#32005,#32004,#26866,.T.) ;
#39098=EDGE_CURVE('',#32006,#32007,#4973,.T.) ;
#39099=EDGE_CURVE('',#32006,#32008,#26867,.T.) ;
#39100=EDGE_CURVE('',#32009,#32008,#9806,.T.) ;
#39101=EDGE_CURVE('',#32010,#32009,#26868,.T.) ;
#39102=EDGE_CURVE('',#32011,#32010,#9807,.T.) ;
#39103=EDGE_CURVE('',#32012,#32011,#9808,.T.) ;
#39104=EDGE_CURVE('',#32012,#32007,#290,.T.) ;
#39105=EDGE_CURVE('',#32013,#32013,#26869,.T.) ;
#39106=EDGE_CURVE('',#32013,#32014,#26870,.T.) ;
#39107=EDGE_CURVE('',#32015,#32014,#26871,.T.) ;
#39108=EDGE_CURVE('',#32014,#32015,#26872,.T.) ;
#39109=EDGE_CURVE('',#32016,#32016,#26873,.T.) ;
#39110=EDGE_CURVE('',#32016,#32017,#26874,.T.) ;
#39111=EDGE_CURVE('',#32017,#32017,#26875,.T.) ;
#39112=EDGE_CURVE('',#32018,#32019,#26876,.T.) ;
#39113=EDGE_CURVE('',#32020,#32018,#26877,.T.) ;
#39114=EDGE_CURVE('',#32020,#32019,#26878,.T.) ;
#39115=EDGE_CURVE('',#32021,#32022,#4974,.T.) ;
#39116=EDGE_CURVE('',#32021,#32023,#26879,.T.) ;
#39117=EDGE_CURVE('',#32024,#32023,#9809,.T.) ;
#39118=EDGE_CURVE('',#32025,#32024,#26880,.T.) ;
#39119=EDGE_CURVE('',#32026,#32025,#9810,.T.) ;
#39120=EDGE_CURVE('',#32027,#32026,#9811,.T.) ;
#39121=EDGE_CURVE('',#32027,#32022,#291,.T.) ;
#39122=EDGE_CURVE('',#32028,#32028,#26881,.T.) ;
#39123=EDGE_CURVE('',#32028,#32029,#26882,.T.) ;
#39124=EDGE_CURVE('',#32030,#32029,#26883,.T.) ;
#39125=EDGE_CURVE('',#32029,#32030,#26884,.T.) ;
#39126=EDGE_CURVE('',#32031,#32031,#26885,.T.) ;
#39127=EDGE_CURVE('',#32031,#32032,#26886,.T.) ;
#39128=EDGE_CURVE('',#32032,#32032,#26887,.T.) ;
#39129=EDGE_CURVE('',#32033,#32034,#26888,.T.) ;
#39130=EDGE_CURVE('',#32035,#32033,#26889,.T.) ;
#39131=EDGE_CURVE('',#32035,#32034,#26890,.T.) ;
#39132=EDGE_CURVE('',#32036,#32037,#4975,.T.) ;
#39133=EDGE_CURVE('',#32036,#32038,#26891,.T.) ;
#39134=EDGE_CURVE('',#32039,#32038,#9812,.T.) ;
#39135=EDGE_CURVE('',#32040,#32039,#26892,.T.) ;
#39136=EDGE_CURVE('',#32041,#32040,#9813,.T.) ;
#39137=EDGE_CURVE('',#32042,#32041,#9814,.T.) ;
#39138=EDGE_CURVE('',#32042,#32037,#292,.T.) ;
#39139=EDGE_CURVE('',#32043,#32043,#26893,.T.) ;
#39140=EDGE_CURVE('',#32043,#32044,#26894,.T.) ;
#39141=EDGE_CURVE('',#32045,#32044,#26895,.T.) ;
#39142=EDGE_CURVE('',#32044,#32045,#26896,.T.) ;
#39143=EDGE_CURVE('',#32046,#32046,#26897,.T.) ;
#39144=EDGE_CURVE('',#32046,#32047,#26898,.T.) ;
#39145=EDGE_CURVE('',#32047,#32047,#26899,.T.) ;
#39146=EDGE_CURVE('',#32048,#32049,#26900,.T.) ;
#39147=EDGE_CURVE('',#32050,#32048,#26901,.T.) ;
#39148=EDGE_CURVE('',#32050,#32049,#26902,.T.) ;
#39149=EDGE_CURVE('',#32051,#32052,#4976,.T.) ;
#39150=EDGE_CURVE('',#32051,#32053,#26903,.T.) ;
#39151=EDGE_CURVE('',#32054,#32053,#9815,.T.) ;
#39152=EDGE_CURVE('',#32055,#32054,#26904,.T.) ;
#39153=EDGE_CURVE('',#32056,#32055,#9816,.T.) ;
#39154=EDGE_CURVE('',#32057,#32056,#9817,.T.) ;
#39155=EDGE_CURVE('',#32057,#32052,#293,.T.) ;
#39156=EDGE_CURVE('',#32058,#32058,#26905,.T.) ;
#39157=EDGE_CURVE('',#32058,#32059,#26906,.T.) ;
#39158=EDGE_CURVE('',#32060,#32059,#26907,.T.) ;
#39159=EDGE_CURVE('',#32059,#32060,#26908,.T.) ;
#39160=EDGE_CURVE('',#32061,#32061,#26909,.T.) ;
#39161=EDGE_CURVE('',#32061,#32062,#26910,.T.) ;
#39162=EDGE_CURVE('',#32062,#32062,#26911,.T.) ;
#39163=EDGE_CURVE('',#32063,#32064,#26912,.T.) ;
#39164=EDGE_CURVE('',#32065,#32063,#26913,.T.) ;
#39165=EDGE_CURVE('',#32065,#32064,#26914,.T.) ;
#39166=EDGE_CURVE('',#32066,#32067,#4977,.T.) ;
#39167=EDGE_CURVE('',#32066,#32068,#26915,.T.) ;
#39168=EDGE_CURVE('',#32069,#32068,#9818,.T.) ;
#39169=EDGE_CURVE('',#32070,#32069,#26916,.T.) ;
#39170=EDGE_CURVE('',#32071,#32070,#9819,.T.) ;
#39171=EDGE_CURVE('',#32072,#32071,#9820,.T.) ;
#39172=EDGE_CURVE('',#32072,#32067,#294,.T.) ;
#39173=EDGE_CURVE('',#32073,#32073,#26917,.T.) ;
#39174=EDGE_CURVE('',#32073,#32074,#26918,.T.) ;
#39175=EDGE_CURVE('',#32075,#32074,#26919,.T.) ;
#39176=EDGE_CURVE('',#32074,#32075,#26920,.T.) ;
#39177=EDGE_CURVE('',#32076,#32076,#26921,.T.) ;
#39178=EDGE_CURVE('',#32076,#32077,#26922,.T.) ;
#39179=EDGE_CURVE('',#32077,#32077,#26923,.T.) ;
#39180=EDGE_CURVE('',#32078,#32079,#26924,.T.) ;
#39181=EDGE_CURVE('',#32080,#32078,#26925,.T.) ;
#39182=EDGE_CURVE('',#32080,#32079,#26926,.T.) ;
#39183=EDGE_CURVE('',#32081,#32082,#4978,.T.) ;
#39184=EDGE_CURVE('',#32081,#32083,#26927,.T.) ;
#39185=EDGE_CURVE('',#32084,#32083,#9821,.T.) ;
#39186=EDGE_CURVE('',#32085,#32084,#26928,.T.) ;
#39187=EDGE_CURVE('',#32086,#32085,#9822,.T.) ;
#39188=EDGE_CURVE('',#32087,#32086,#9823,.T.) ;
#39189=EDGE_CURVE('',#32087,#32082,#295,.T.) ;
#39190=EDGE_CURVE('',#32088,#32088,#26929,.T.) ;
#39191=EDGE_CURVE('',#32088,#32089,#26930,.T.) ;
#39192=EDGE_CURVE('',#32090,#32089,#26931,.T.) ;
#39193=EDGE_CURVE('',#32089,#32090,#26932,.T.) ;
#39194=EDGE_CURVE('',#32091,#32091,#26933,.T.) ;
#39195=EDGE_CURVE('',#32091,#32092,#26934,.T.) ;
#39196=EDGE_CURVE('',#32092,#32092,#26935,.T.) ;
#39197=EDGE_CURVE('',#32093,#32094,#26936,.T.) ;
#39198=EDGE_CURVE('',#32095,#32093,#26937,.T.) ;
#39199=EDGE_CURVE('',#32095,#32094,#26938,.T.) ;
#39200=EDGE_CURVE('',#32096,#32097,#4979,.T.) ;
#39201=EDGE_CURVE('',#32096,#32098,#26939,.T.) ;
#39202=EDGE_CURVE('',#32099,#32098,#9824,.T.) ;
#39203=EDGE_CURVE('',#32100,#32099,#26940,.T.) ;
#39204=EDGE_CURVE('',#32101,#32100,#9825,.T.) ;
#39205=EDGE_CURVE('',#32102,#32101,#9826,.T.) ;
#39206=EDGE_CURVE('',#32102,#32097,#296,.T.) ;
#39207=EDGE_CURVE('',#32103,#32103,#26941,.T.) ;
#39208=EDGE_CURVE('',#32103,#32104,#26942,.T.) ;
#39209=EDGE_CURVE('',#32105,#32104,#26943,.T.) ;
#39210=EDGE_CURVE('',#32104,#32105,#26944,.T.) ;
#39211=EDGE_CURVE('',#32106,#32106,#26945,.T.) ;
#39212=EDGE_CURVE('',#32106,#32107,#26946,.T.) ;
#39213=EDGE_CURVE('',#32107,#32107,#26947,.T.) ;
#39214=EDGE_CURVE('',#32108,#32109,#26948,.T.) ;
#39215=EDGE_CURVE('',#32110,#32108,#26949,.T.) ;
#39216=EDGE_CURVE('',#32110,#32109,#26950,.T.) ;
#39217=EDGE_CURVE('',#32111,#32112,#4980,.T.) ;
#39218=EDGE_CURVE('',#32111,#32113,#26951,.T.) ;
#39219=EDGE_CURVE('',#32114,#32113,#9827,.T.) ;
#39220=EDGE_CURVE('',#32115,#32114,#26952,.T.) ;
#39221=EDGE_CURVE('',#32116,#32115,#9828,.T.) ;
#39222=EDGE_CURVE('',#32117,#32116,#9829,.T.) ;
#39223=EDGE_CURVE('',#32117,#32112,#297,.T.) ;
#39224=EDGE_CURVE('',#32118,#32118,#26953,.T.) ;
#39225=EDGE_CURVE('',#32118,#32119,#26954,.T.) ;
#39226=EDGE_CURVE('',#32120,#32119,#26955,.T.) ;
#39227=EDGE_CURVE('',#32119,#32120,#26956,.T.) ;
#39228=EDGE_CURVE('',#32121,#32122,#26957,.T.) ;
#39229=EDGE_CURVE('',#32123,#32121,#26958,.T.) ;
#39230=EDGE_CURVE('',#32124,#32123,#26959,.T.) ;
#39231=EDGE_CURVE('',#32124,#32122,#26960,.T.) ;
#39232=EDGE_CURVE('',#32125,#32126,#26961,.T.) ;
#39233=EDGE_CURVE('',#32127,#32125,#26962,.T.) ;
#39234=EDGE_CURVE('',#32128,#32127,#26963,.T.) ;
#39235=EDGE_CURVE('',#32128,#32126,#26964,.T.) ;
#39236=EDGE_CURVE('',#32129,#32130,#26965,.T.) ;
#39237=EDGE_CURVE('',#32131,#32129,#26966,.T.) ;
#39238=EDGE_CURVE('',#32132,#32131,#26967,.T.) ;
#39239=EDGE_CURVE('',#32132,#32130,#26968,.T.) ;
#39240=EDGE_CURVE('',#32133,#32134,#26969,.T.) ;
#39241=EDGE_CURVE('',#32135,#32133,#26970,.T.) ;
#39242=EDGE_CURVE('',#32136,#32135,#26971,.T.) ;
#39243=EDGE_CURVE('',#32136,#32134,#26972,.T.) ;
#39244=EDGE_CURVE('',#32137,#32138,#26973,.T.) ;
#39245=EDGE_CURVE('',#32139,#32137,#26974,.T.) ;
#39246=EDGE_CURVE('',#32140,#32139,#26975,.T.) ;
#39247=EDGE_CURVE('',#32140,#32138,#26976,.T.) ;
#39248=EDGE_CURVE('',#32141,#32142,#26977,.T.) ;
#39249=EDGE_CURVE('',#32143,#32141,#26978,.T.) ;
#39250=EDGE_CURVE('',#32144,#32143,#26979,.T.) ;
#39251=EDGE_CURVE('',#32144,#32142,#26980,.T.) ;
#39252=EDGE_CURVE('',#32145,#32146,#26981,.T.) ;
#39253=EDGE_CURVE('',#32147,#32145,#26982,.T.) ;
#39254=EDGE_CURVE('',#32148,#32147,#26983,.T.) ;
#39255=EDGE_CURVE('',#32148,#32146,#26984,.T.) ;
#39256=EDGE_CURVE('',#32149,#32150,#26985,.T.) ;
#39257=EDGE_CURVE('',#32151,#32149,#26986,.T.) ;
#39258=EDGE_CURVE('',#32152,#32151,#26987,.T.) ;
#39259=EDGE_CURVE('',#32152,#32150,#26988,.T.) ;
#39260=EDGE_CURVE('',#32153,#32154,#26989,.T.) ;
#39261=EDGE_CURVE('',#32155,#32153,#26990,.T.) ;
#39262=EDGE_CURVE('',#32156,#32155,#26991,.T.) ;
#39263=EDGE_CURVE('',#32156,#32154,#26992,.T.) ;
#39264=EDGE_CURVE('',#32157,#32157,#26993,.T.) ;
#39265=EDGE_CURVE('',#32157,#32158,#26994,.T.) ;
#39266=EDGE_CURVE('',#32158,#32158,#26995,.T.) ;
#39267=EDGE_CURVE('',#32159,#32160,#26996,.T.) ;
#39268=EDGE_CURVE('',#32161,#32159,#26997,.T.) ;
#39269=EDGE_CURVE('',#32161,#32160,#26998,.T.) ;
#39270=EDGE_CURVE('',#32162,#32163,#4981,.T.) ;
#39271=EDGE_CURVE('',#32162,#32164,#26999,.T.) ;
#39272=EDGE_CURVE('',#32165,#32164,#9830,.T.) ;
#39273=EDGE_CURVE('',#32166,#32165,#27000,.T.) ;
#39274=EDGE_CURVE('',#32167,#32166,#9831,.T.) ;
#39275=EDGE_CURVE('',#32168,#32167,#9832,.T.) ;
#39276=EDGE_CURVE('',#32168,#32163,#298,.T.) ;
#39277=EDGE_CURVE('',#32002,#32000,#9833,.T.) ;
#39278=EDGE_CURVE('',#32017,#32015,#9834,.T.) ;
#39279=EDGE_CURVE('',#32032,#32030,#9835,.T.) ;
#39280=EDGE_CURVE('',#32047,#32045,#9836,.T.) ;
#39281=EDGE_CURVE('',#32062,#32060,#9837,.T.) ;
#39282=EDGE_CURVE('',#32077,#32075,#9838,.T.) ;
#39283=EDGE_CURVE('',#32092,#32090,#9839,.T.) ;
#39284=EDGE_CURVE('',#32107,#32105,#9840,.T.) ;
#39285=EDGE_CURVE('',#32158,#32120,#9841,.T.) ;
#39286=EDGE_CURVE('',#32169,#32170,#27001,.T.) ;
#39287=EDGE_CURVE('',#32170,#32124,#9842,.T.) ;
#39288=EDGE_CURVE('',#32169,#32123,#9843,.T.) ;
#39289=EDGE_CURVE('',#32171,#32172,#27002,.T.) ;
#39290=EDGE_CURVE('',#32172,#32128,#9844,.T.) ;
#39291=EDGE_CURVE('',#32171,#32127,#9845,.T.) ;
#39292=EDGE_CURVE('',#32173,#32174,#27003,.T.) ;
#39293=EDGE_CURVE('',#32174,#32132,#9846,.T.) ;
#39294=EDGE_CURVE('',#32173,#32131,#9847,.T.) ;
#39295=EDGE_CURVE('',#32175,#32176,#27004,.T.) ;
#39296=EDGE_CURVE('',#32176,#32136,#9848,.T.) ;
#39297=EDGE_CURVE('',#32175,#32135,#9849,.T.) ;
#39298=EDGE_CURVE('',#32177,#32178,#27005,.T.) ;
#39299=EDGE_CURVE('',#32178,#32140,#9850,.T.) ;
#39300=EDGE_CURVE('',#32177,#32139,#9851,.T.) ;
#39301=EDGE_CURVE('',#32179,#32180,#27006,.T.) ;
#39302=EDGE_CURVE('',#32180,#32144,#9852,.T.) ;
#39303=EDGE_CURVE('',#32179,#32143,#9853,.T.) ;
#39304=EDGE_CURVE('',#32181,#32182,#27007,.T.) ;
#39305=EDGE_CURVE('',#32182,#32148,#9854,.T.) ;
#39306=EDGE_CURVE('',#32181,#32147,#9855,.T.) ;
#39307=EDGE_CURVE('',#32183,#32184,#27008,.T.) ;
#39308=EDGE_CURVE('',#32184,#32152,#9856,.T.) ;
#39309=EDGE_CURVE('',#32183,#32151,#9857,.T.) ;
#39310=EDGE_CURVE('',#32185,#32186,#27009,.T.) ;
#39311=EDGE_CURVE('',#32186,#32156,#9858,.T.) ;
#39312=EDGE_CURVE('',#32185,#32155,#9859,.T.) ;
#39313=EDGE_CURVE('',#32187,#32187,#27010,.T.) ;
#39314=EDGE_CURVE('',#32187,#32188,#27011,.T.) ;
#39315=EDGE_CURVE('',#32189,#32188,#27012,.T.) ;
#39316=EDGE_CURVE('',#32188,#32189,#27013,.T.) ;
#39317=EDGE_CURVE('',#32190,#32191,#27014,.T.) ;
#39318=EDGE_CURVE('',#32192,#32190,#27015,.T.) ;
#39319=EDGE_CURVE('',#32193,#32192,#27016,.T.) ;
#39320=EDGE_CURVE('',#32193,#32191,#27017,.T.) ;
#39321=EDGE_CURVE('',#32194,#32194,#27018,.T.) ;
#39322=EDGE_CURVE('',#32194,#32195,#27019,.T.) ;
#39323=EDGE_CURVE('',#32195,#32195,#27020,.T.) ;
#39324=EDGE_CURVE('',#32196,#32197,#27021,.T.) ;
#39325=EDGE_CURVE('',#32198,#32196,#27022,.T.) ;
#39326=EDGE_CURVE('',#32198,#32197,#27023,.T.) ;
#39327=EDGE_CURVE('',#32199,#32200,#4982,.T.) ;
#39328=EDGE_CURVE('',#32199,#32201,#27024,.T.) ;
#39329=EDGE_CURVE('',#32202,#32201,#9860,.T.) ;
#39330=EDGE_CURVE('',#32203,#32202,#27025,.T.) ;
#39331=EDGE_CURVE('',#32204,#32203,#9861,.T.) ;
#39332=EDGE_CURVE('',#32205,#32204,#9862,.T.) ;
#39333=EDGE_CURVE('',#32205,#32200,#299,.T.) ;
#39334=EDGE_CURVE('',#32195,#32189,#9863,.T.) ;
#39335=EDGE_CURVE('',#32206,#32207,#27026,.T.) ;
#39336=EDGE_CURVE('',#32207,#32193,#9864,.T.) ;
#39337=EDGE_CURVE('',#32206,#32192,#9865,.T.) ;
#39338=EDGE_CURVE('',#32208,#32209,#9866,.T.) ;
#39339=EDGE_CURVE('',#32209,#32210,#27027,.T.) ;
#39340=EDGE_CURVE('',#32210,#32211,#9867,.T.) ;
#39341=EDGE_CURVE('',#32211,#32011,#27028,.T.) ;
#39342=EDGE_CURVE('',#32212,#32010,#27029,.T.) ;
#39343=EDGE_CURVE('',#32212,#32213,#9868,.T.) ;
#39344=EDGE_CURVE('',#32213,#32214,#9869,.T.) ;
#39345=EDGE_CURVE('',#32214,#32215,#9870,.T.) ;
#39346=EDGE_CURVE('',#32215,#32216,#9871,.T.) ;
#39347=EDGE_CURVE('',#32216,#32217,#9872,.T.) ;
#39348=EDGE_CURVE('',#32208,#32217,#27030,.T.) ;
#39349=EDGE_CURVE('',#32218,#32219,#9873,.T.) ;
#39350=EDGE_CURVE('',#32219,#32220,#27031,.T.) ;
#39351=EDGE_CURVE('',#32220,#32221,#9874,.T.) ;
#39352=EDGE_CURVE('',#32221,#32026,#27032,.T.) ;
#39353=EDGE_CURVE('',#32222,#32025,#27033,.T.) ;
#39354=EDGE_CURVE('',#32222,#32223,#9875,.T.) ;
#39355=EDGE_CURVE('',#32223,#32224,#9876,.T.) ;
#39356=EDGE_CURVE('',#32224,#32225,#9877,.T.) ;
#39357=EDGE_CURVE('',#32225,#32226,#9878,.T.) ;
#39358=EDGE_CURVE('',#32226,#32227,#9879,.T.) ;
#39359=EDGE_CURVE('',#32218,#32227,#27034,.T.) ;
#39360=EDGE_CURVE('',#32228,#32229,#9880,.T.) ;
#39361=EDGE_CURVE('',#32229,#32230,#27035,.T.) ;
#39362=EDGE_CURVE('',#32230,#32231,#9881,.T.) ;
#39363=EDGE_CURVE('',#32231,#32041,#27036,.T.) ;
#39364=EDGE_CURVE('',#32232,#32040,#27037,.T.) ;
#39365=EDGE_CURVE('',#32232,#32233,#9882,.T.) ;
#39366=EDGE_CURVE('',#32233,#32234,#9883,.T.) ;
#39367=EDGE_CURVE('',#32234,#32235,#9884,.T.) ;
#39368=EDGE_CURVE('',#32235,#32236,#9885,.T.) ;
#39369=EDGE_CURVE('',#32236,#32237,#9886,.T.) ;
#39370=EDGE_CURVE('',#32228,#32237,#27038,.T.) ;
#39371=EDGE_CURVE('',#32238,#32239,#9887,.T.) ;
#39372=EDGE_CURVE('',#32239,#32240,#27039,.T.) ;
#39373=EDGE_CURVE('',#32240,#32241,#9888,.T.) ;
#39374=EDGE_CURVE('',#32241,#32056,#27040,.T.) ;
#39375=EDGE_CURVE('',#32242,#32055,#27041,.T.) ;
#39376=EDGE_CURVE('',#32242,#32243,#9889,.T.) ;
#39377=EDGE_CURVE('',#32243,#32244,#9890,.T.) ;
#39378=EDGE_CURVE('',#32244,#32245,#9891,.T.) ;
#39379=EDGE_CURVE('',#32245,#32246,#9892,.T.) ;
#39380=EDGE_CURVE('',#32246,#32247,#9893,.T.) ;
#39381=EDGE_CURVE('',#32238,#32247,#27042,.T.) ;
#39382=EDGE_CURVE('',#32248,#32249,#9894,.T.) ;
#39383=EDGE_CURVE('',#32249,#32250,#27043,.T.) ;
#39384=EDGE_CURVE('',#32250,#32251,#9895,.T.) ;
#39385=EDGE_CURVE('',#32251,#32071,#27044,.T.) ;
#39386=EDGE_CURVE('',#32252,#32070,#27045,.T.) ;
#39387=EDGE_CURVE('',#32252,#32253,#9896,.T.) ;
#39388=EDGE_CURVE('',#32253,#32254,#9897,.T.) ;
#39389=EDGE_CURVE('',#32254,#32255,#9898,.T.) ;
#39390=EDGE_CURVE('',#32255,#32256,#9899,.T.) ;
#39391=EDGE_CURVE('',#32256,#32257,#9900,.T.) ;
#39392=EDGE_CURVE('',#32248,#32257,#27046,.T.) ;
#39393=EDGE_CURVE('',#32258,#32259,#9901,.T.) ;
#39394=EDGE_CURVE('',#32259,#32260,#27047,.T.) ;
#39395=EDGE_CURVE('',#32260,#32261,#9902,.T.) ;
#39396=EDGE_CURVE('',#32261,#32086,#27048,.T.) ;
#39397=EDGE_CURVE('',#32262,#32085,#27049,.T.) ;
#39398=EDGE_CURVE('',#32262,#32263,#9903,.T.) ;
#39399=EDGE_CURVE('',#32263,#32264,#9904,.T.) ;
#39400=EDGE_CURVE('',#32264,#32265,#9905,.T.) ;
#39401=EDGE_CURVE('',#32265,#32266,#9906,.T.) ;
#39402=EDGE_CURVE('',#32266,#32267,#9907,.T.) ;
#39403=EDGE_CURVE('',#32258,#32267,#27050,.T.) ;
#39404=EDGE_CURVE('',#32268,#32269,#9908,.T.) ;
#39405=EDGE_CURVE('',#32269,#32270,#27051,.T.) ;
#39406=EDGE_CURVE('',#32270,#32271,#9909,.T.) ;
#39407=EDGE_CURVE('',#32271,#32101,#27052,.T.) ;
#39408=EDGE_CURVE('',#32272,#32100,#27053,.T.) ;
#39409=EDGE_CURVE('',#32272,#32273,#9910,.T.) ;
#39410=EDGE_CURVE('',#32273,#32274,#9911,.T.) ;
#39411=EDGE_CURVE('',#32274,#32275,#9912,.T.) ;
#39412=EDGE_CURVE('',#32275,#32276,#9913,.T.) ;
#39413=EDGE_CURVE('',#32276,#32277,#9914,.T.) ;
#39414=EDGE_CURVE('',#32268,#32277,#27054,.T.) ;
#39415=EDGE_CURVE('',#32278,#32279,#9915,.T.) ;
#39416=EDGE_CURVE('',#32279,#32280,#27055,.T.) ;
#39417=EDGE_CURVE('',#32280,#32281,#9916,.T.) ;
#39418=EDGE_CURVE('',#32281,#32116,#27056,.T.) ;
#39419=EDGE_CURVE('',#32282,#32115,#27057,.T.) ;
#39420=EDGE_CURVE('',#32282,#32283,#9917,.T.) ;
#39421=EDGE_CURVE('',#32283,#32284,#9918,.T.) ;
#39422=EDGE_CURVE('',#32284,#32285,#9919,.T.) ;
#39423=EDGE_CURVE('',#32285,#32286,#9920,.T.) ;
#39424=EDGE_CURVE('',#32286,#32287,#9921,.T.) ;
#39425=EDGE_CURVE('',#32278,#32287,#27058,.T.) ;
#39426=EDGE_CURVE('',#32288,#32289,#9922,.T.) ;
#39427=EDGE_CURVE('',#32289,#32290,#27059,.T.) ;
#39428=EDGE_CURVE('',#32290,#32291,#9923,.T.) ;
#39429=EDGE_CURVE('',#32291,#32167,#27060,.T.) ;
#39430=EDGE_CURVE('',#32292,#32166,#27061,.T.) ;
#39431=EDGE_CURVE('',#32292,#32293,#9924,.T.) ;
#39432=EDGE_CURVE('',#32293,#32294,#9925,.T.) ;
#39433=EDGE_CURVE('',#32294,#32295,#9926,.T.) ;
#39434=EDGE_CURVE('',#32295,#32296,#9927,.T.) ;
#39435=EDGE_CURVE('',#32296,#32297,#9928,.T.) ;
#39436=EDGE_CURVE('',#32288,#32297,#27062,.T.) ;
#39437=EDGE_CURVE('',#32298,#32299,#27063,.T.) ;
#39438=EDGE_CURVE('',#32298,#32300,#9929,.T.) ;
#39439=EDGE_CURVE('',#32300,#32301,#9930,.T.) ;
#39440=EDGE_CURVE('',#32301,#32302,#9931,.T.) ;
#39441=EDGE_CURVE('',#32302,#32299,#9932,.T.) ;
#39442=EDGE_CURVE('',#32303,#32304,#27064,.T.) ;
#39443=EDGE_CURVE('',#32303,#32305,#9933,.T.) ;
#39444=EDGE_CURVE('',#32305,#32306,#9934,.T.) ;
#39445=EDGE_CURVE('',#32306,#32307,#9935,.T.) ;
#39446=EDGE_CURVE('',#32307,#32304,#9936,.T.) ;
#39447=EDGE_CURVE('',#32308,#32309,#27065,.T.) ;
#39448=EDGE_CURVE('',#32308,#32310,#9937,.T.) ;
#39449=EDGE_CURVE('',#32310,#32311,#9938,.T.) ;
#39450=EDGE_CURVE('',#32311,#32312,#9939,.T.) ;
#39451=EDGE_CURVE('',#32312,#32309,#9940,.T.) ;
#39452=EDGE_CURVE('',#32313,#32314,#27066,.T.) ;
#39453=EDGE_CURVE('',#32313,#32315,#9941,.T.) ;
#39454=EDGE_CURVE('',#32315,#32316,#9942,.T.) ;
#39455=EDGE_CURVE('',#32316,#32317,#9943,.T.) ;
#39456=EDGE_CURVE('',#32317,#32314,#9944,.T.) ;
#39457=EDGE_CURVE('',#32318,#32319,#27067,.T.) ;
#39458=EDGE_CURVE('',#32318,#32320,#9945,.T.) ;
#39459=EDGE_CURVE('',#32320,#32321,#9946,.T.) ;
#39460=EDGE_CURVE('',#32321,#32322,#9947,.T.) ;
#39461=EDGE_CURVE('',#32322,#32319,#9948,.T.) ;
#39462=EDGE_CURVE('',#32323,#32324,#27068,.T.) ;
#39463=EDGE_CURVE('',#32323,#32325,#9949,.T.) ;
#39464=EDGE_CURVE('',#32325,#32326,#9950,.T.) ;
#39465=EDGE_CURVE('',#32326,#32327,#9951,.T.) ;
#39466=EDGE_CURVE('',#32327,#32324,#9952,.T.) ;
#39467=EDGE_CURVE('',#32328,#32329,#27069,.T.) ;
#39468=EDGE_CURVE('',#32328,#32330,#9953,.T.) ;
#39469=EDGE_CURVE('',#32330,#32331,#9954,.T.) ;
#39470=EDGE_CURVE('',#32331,#32332,#9955,.T.) ;
#39471=EDGE_CURVE('',#32332,#32329,#9956,.T.) ;
#39472=EDGE_CURVE('',#32333,#32334,#27070,.T.) ;
#39473=EDGE_CURVE('',#32333,#32335,#9957,.T.) ;
#39474=EDGE_CURVE('',#32335,#32336,#9958,.T.) ;
#39475=EDGE_CURVE('',#32336,#32337,#9959,.T.) ;
#39476=EDGE_CURVE('',#32337,#32334,#9960,.T.) ;
#39477=EDGE_CURVE('',#32338,#32339,#27071,.T.) ;
#39478=EDGE_CURVE('',#32338,#32340,#9961,.T.) ;
#39479=EDGE_CURVE('',#32340,#32341,#9962,.T.) ;
#39480=EDGE_CURVE('',#32341,#32342,#9963,.T.) ;
#39481=EDGE_CURVE('',#32342,#32339,#9964,.T.) ;
#39482=EDGE_CURVE('',#32343,#32344,#27072,.T.) ;
#39483=EDGE_CURVE('',#32343,#32345,#9965,.T.) ;
#39484=EDGE_CURVE('',#32345,#32346,#9966,.T.) ;
#39485=EDGE_CURVE('',#32346,#32347,#9967,.T.) ;
#39486=EDGE_CURVE('',#32347,#32344,#9968,.T.) ;
#39487=EDGE_CURVE('',#32348,#32349,#27073,.T.) ;
#39488=EDGE_CURVE('',#32348,#32350,#9969,.T.) ;
#39489=EDGE_CURVE('',#32350,#32351,#9970,.T.) ;
#39490=EDGE_CURVE('',#32351,#32352,#9971,.T.) ;
#39491=EDGE_CURVE('',#32352,#32349,#9972,.T.) ;
#39492=EDGE_CURVE('',#32353,#32354,#27074,.T.) ;
#39493=EDGE_CURVE('',#32353,#32355,#9973,.T.) ;
#39494=EDGE_CURVE('',#32355,#32356,#9974,.T.) ;
#39495=EDGE_CURVE('',#32356,#32357,#9975,.T.) ;
#39496=EDGE_CURVE('',#32357,#32354,#9976,.T.) ;
#39497=EDGE_CURVE('',#32358,#32359,#27075,.T.) ;
#39498=EDGE_CURVE('',#32358,#32360,#9977,.T.) ;
#39499=EDGE_CURVE('',#32360,#32361,#9978,.T.) ;
#39500=EDGE_CURVE('',#32361,#32362,#9979,.T.) ;
#39501=EDGE_CURVE('',#32362,#32359,#9980,.T.) ;
#39502=EDGE_CURVE('',#32363,#32364,#27076,.T.) ;
#39503=EDGE_CURVE('',#32363,#32365,#9981,.T.) ;
#39504=EDGE_CURVE('',#32365,#32366,#9982,.T.) ;
#39505=EDGE_CURVE('',#32366,#32367,#9983,.T.) ;
#39506=EDGE_CURVE('',#32367,#32364,#9984,.T.) ;
#39507=EDGE_CURVE('',#32368,#32369,#27077,.T.) ;
#39508=EDGE_CURVE('',#32368,#32370,#9985,.T.) ;
#39509=EDGE_CURVE('',#32370,#32371,#9986,.T.) ;
#39510=EDGE_CURVE('',#32371,#32372,#9987,.T.) ;
#39511=EDGE_CURVE('',#32372,#32369,#9988,.T.) ;
#39512=EDGE_CURVE('',#32373,#32374,#27078,.T.) ;
#39513=EDGE_CURVE('',#32373,#32375,#9989,.T.) ;
#39514=EDGE_CURVE('',#32375,#32376,#9990,.T.) ;
#39515=EDGE_CURVE('',#32376,#32377,#9991,.T.) ;
#39516=EDGE_CURVE('',#32377,#32374,#9992,.T.) ;
#39517=EDGE_CURVE('',#32378,#32379,#27079,.T.) ;
#39518=EDGE_CURVE('',#32378,#32380,#9993,.T.) ;
#39519=EDGE_CURVE('',#32380,#32381,#9994,.T.) ;
#39520=EDGE_CURVE('',#32381,#32382,#9995,.T.) ;
#39521=EDGE_CURVE('',#32382,#32379,#9996,.T.) ;
#39522=EDGE_CURVE('',#32383,#32384,#27080,.T.) ;
#39523=EDGE_CURVE('',#32383,#32385,#9997,.T.) ;
#39524=EDGE_CURVE('',#32385,#32386,#9998,.T.) ;
#39525=EDGE_CURVE('',#32386,#32387,#9999,.T.) ;
#39526=EDGE_CURVE('',#32387,#32384,#10000,.T.) ;
#39527=EDGE_CURVE('',#32388,#32389,#10001,.T.) ;
#39528=EDGE_CURVE('',#32388,#32390,#27081,.T.) ;
#39529=EDGE_CURVE('',#32390,#32391,#10002,.T.) ;
#39530=EDGE_CURVE('',#32391,#32389,#27082,.T.) ;
#39531=EDGE_CURVE('',#32392,#32393,#10003,.T.) ;
#39532=EDGE_CURVE('',#32392,#32394,#27083,.T.) ;
#39533=EDGE_CURVE('',#32394,#32395,#10004,.T.) ;
#39534=EDGE_CURVE('',#32395,#32393,#27084,.T.) ;
#39535=EDGE_CURVE('',#32396,#32397,#10005,.T.) ;
#39536=EDGE_CURVE('',#32396,#32398,#27085,.T.) ;
#39537=EDGE_CURVE('',#32398,#32399,#10006,.T.) ;
#39538=EDGE_CURVE('',#32399,#32397,#27086,.T.) ;
#39539=EDGE_CURVE('',#32400,#32401,#10007,.T.) ;
#39540=EDGE_CURVE('',#32400,#32402,#27087,.T.) ;
#39541=EDGE_CURVE('',#32402,#32403,#10008,.T.) ;
#39542=EDGE_CURVE('',#32403,#32401,#27088,.T.) ;
#39543=EDGE_CURVE('',#32404,#32405,#10009,.T.) ;
#39544=EDGE_CURVE('',#32404,#32406,#27089,.T.) ;
#39545=EDGE_CURVE('',#32406,#32407,#10010,.T.) ;
#39546=EDGE_CURVE('',#32407,#32405,#27090,.T.) ;
#39547=EDGE_CURVE('',#32408,#32409,#10011,.T.) ;
#39548=EDGE_CURVE('',#32408,#32410,#27091,.T.) ;
#39549=EDGE_CURVE('',#32410,#32411,#10012,.T.) ;
#39550=EDGE_CURVE('',#32411,#32409,#27092,.T.) ;
#39551=EDGE_CURVE('',#32412,#32413,#10013,.T.) ;
#39552=EDGE_CURVE('',#32412,#32414,#27093,.T.) ;
#39553=EDGE_CURVE('',#32414,#32415,#10014,.T.) ;
#39554=EDGE_CURVE('',#32415,#32413,#27094,.T.) ;
#39555=EDGE_CURVE('',#32416,#32417,#10015,.T.) ;
#39556=EDGE_CURVE('',#32416,#32418,#27095,.T.) ;
#39557=EDGE_CURVE('',#32418,#32419,#10016,.T.) ;
#39558=EDGE_CURVE('',#32419,#32417,#27096,.T.) ;
#39559=EDGE_CURVE('',#32420,#32421,#10017,.T.) ;
#39560=EDGE_CURVE('',#32420,#32422,#27097,.T.) ;
#39561=EDGE_CURVE('',#32422,#32423,#10018,.T.) ;
#39562=EDGE_CURVE('',#32423,#32421,#27098,.T.) ;
#39563=EDGE_CURVE('',#32424,#32425,#10019,.T.) ;
#39564=EDGE_CURVE('',#32425,#32426,#27099,.T.) ;
#39565=EDGE_CURVE('',#32426,#32427,#10020,.T.) ;
#39566=EDGE_CURVE('',#32427,#32204,#27100,.T.) ;
#39567=EDGE_CURVE('',#32428,#32203,#27101,.T.) ;
#39568=EDGE_CURVE('',#32428,#32429,#10021,.T.) ;
#39569=EDGE_CURVE('',#32429,#32430,#10022,.T.) ;
#39570=EDGE_CURVE('',#32430,#32431,#10023,.T.) ;
#39571=EDGE_CURVE('',#32431,#32432,#10024,.T.) ;
#39572=EDGE_CURVE('',#32432,#32433,#10025,.T.) ;
#39573=EDGE_CURVE('',#32424,#32433,#27102,.T.) ;
#39574=EDGE_CURVE('',#32434,#32435,#27103,.T.) ;
#39575=EDGE_CURVE('',#32434,#32436,#10026,.T.) ;
#39576=EDGE_CURVE('',#32436,#32437,#10027,.T.) ;
#39577=EDGE_CURVE('',#32437,#32438,#10028,.T.) ;
#39578=EDGE_CURVE('',#32438,#32435,#10029,.T.) ;
#39579=EDGE_CURVE('',#32439,#32440,#27104,.T.) ;
#39580=EDGE_CURVE('',#32439,#32441,#10030,.T.) ;
#39581=EDGE_CURVE('',#32441,#32442,#10031,.T.) ;
#39582=EDGE_CURVE('',#32442,#32443,#10032,.T.) ;
#39583=EDGE_CURVE('',#32443,#32440,#10033,.T.) ;
#39584=EDGE_CURVE('',#32444,#32445,#10034,.T.) ;
#39585=EDGE_CURVE('',#32444,#32446,#27105,.T.) ;
#39586=EDGE_CURVE('',#32446,#32447,#10035,.T.) ;
#39587=EDGE_CURVE('',#32447,#32445,#27106,.T.) ;
#39588=EDGE_CURVE('',#32448,#32449,#10036,.T.) ;
#39589=EDGE_CURVE('',#32448,#32450,#27107,.T.) ;
#39590=EDGE_CURVE('',#32450,#32451,#10037,.T.) ;
#39591=EDGE_CURVE('',#32451,#32449,#27108,.T.) ;
#39592=EDGE_CURVE('',#32452,#32453,#27109,.T.) ;
#39593=EDGE_CURVE('',#32452,#32454,#10038,.T.) ;
#39594=EDGE_CURVE('',#32455,#32454,#10039,.T.) ;
#39595=EDGE_CURVE('',#32455,#32448,#10040,.T.) ;
#39596=EDGE_CURVE('',#32449,#32447,#10041,.T.) ;
#39597=EDGE_CURVE('',#32446,#32456,#10042,.T.) ;
#39598=EDGE_CURVE('',#32457,#32456,#27110,.T.) ;
#39599=EDGE_CURVE('',#32457,#32458,#10043,.T.) ;
#39600=EDGE_CURVE('',#32459,#32458,#27111,.T.) ;
#39601=EDGE_CURVE('',#32459,#32391,#10044,.T.) ;
#39602=EDGE_CURVE('',#32390,#32460,#10045,.T.) ;
#39603=EDGE_CURVE('',#32461,#32460,#27112,.T.) ;
#39604=EDGE_CURVE('',#32461,#32462,#10046,.T.) ;
#39605=EDGE_CURVE('',#32463,#32462,#27113,.T.) ;
#39606=EDGE_CURVE('',#32463,#32395,#10047,.T.) ;
#39607=EDGE_CURVE('',#32394,#32464,#10048,.T.) ;
#39608=EDGE_CURVE('',#32465,#32464,#27114,.T.) ;
#39609=EDGE_CURVE('',#32465,#32466,#10049,.T.) ;
#39610=EDGE_CURVE('',#32467,#32466,#27115,.T.) ;
#39611=EDGE_CURVE('',#32467,#32399,#10050,.T.) ;
#39612=EDGE_CURVE('',#32398,#32468,#10051,.T.) ;
#39613=EDGE_CURVE('',#32469,#32468,#27116,.T.) ;
#39614=EDGE_CURVE('',#32469,#32470,#10052,.T.) ;
#39615=EDGE_CURVE('',#32471,#32470,#27117,.T.) ;
#39616=EDGE_CURVE('',#32471,#32403,#10053,.T.) ;
#39617=EDGE_CURVE('',#32402,#32472,#10054,.T.) ;
#39618=EDGE_CURVE('',#32473,#32472,#27118,.T.) ;
#39619=EDGE_CURVE('',#32473,#32474,#10055,.T.) ;
#39620=EDGE_CURVE('',#32475,#32474,#27119,.T.) ;
#39621=EDGE_CURVE('',#32475,#32407,#10056,.T.) ;
#39622=EDGE_CURVE('',#32406,#32476,#10057,.T.) ;
#39623=EDGE_CURVE('',#32477,#32476,#27120,.T.) ;
#39624=EDGE_CURVE('',#32477,#32478,#10058,.T.) ;
#39625=EDGE_CURVE('',#32479,#32478,#27121,.T.) ;
#39626=EDGE_CURVE('',#32479,#32411,#10059,.T.) ;
#39627=EDGE_CURVE('',#32410,#32480,#10060,.T.) ;
#39628=EDGE_CURVE('',#32481,#32480,#27122,.T.) ;
#39629=EDGE_CURVE('',#32481,#32482,#10061,.T.) ;
#39630=EDGE_CURVE('',#32483,#32482,#27123,.T.) ;
#39631=EDGE_CURVE('',#32483,#32415,#10062,.T.) ;
#39632=EDGE_CURVE('',#32414,#32484,#10063,.T.) ;
#39633=EDGE_CURVE('',#32485,#32484,#27124,.T.) ;
#39634=EDGE_CURVE('',#32485,#32486,#10064,.T.) ;
#39635=EDGE_CURVE('',#32487,#32486,#27125,.T.) ;
#39636=EDGE_CURVE('',#32487,#32419,#10065,.T.) ;
#39637=EDGE_CURVE('',#32418,#32488,#10066,.T.) ;
#39638=EDGE_CURVE('',#32489,#32488,#27126,.T.) ;
#39639=EDGE_CURVE('',#32489,#32490,#10067,.T.) ;
#39640=EDGE_CURVE('',#32491,#32490,#27127,.T.) ;
#39641=EDGE_CURVE('',#32491,#32423,#10068,.T.) ;
#39642=EDGE_CURVE('',#32422,#32492,#10069,.T.) ;
#39643=EDGE_CURVE('',#32493,#32492,#27128,.T.) ;
#39644=EDGE_CURVE('',#32493,#32453,#10070,.T.) ;
#39645=EDGE_CURVE('',#32454,#32494,#27129,.T.) ;
#39646=EDGE_CURVE('',#32495,#32494,#10071,.T.) ;
#39647=EDGE_CURVE('',#32495,#32455,#27130,.T.) ;
#39648=EDGE_CURVE('',#32496,#32497,#27131,.T.) ;
#39649=EDGE_CURVE('',#32496,#32420,#10072,.T.) ;
#39650=EDGE_CURVE('',#32421,#32498,#10073,.T.) ;
#39651=EDGE_CURVE('',#32499,#32498,#27132,.T.) ;
#39652=EDGE_CURVE('',#32499,#32500,#10074,.T.) ;
#39653=EDGE_CURVE('',#32501,#32500,#27133,.T.) ;
#39654=EDGE_CURVE('',#32501,#32416,#10075,.T.) ;
#39655=EDGE_CURVE('',#32417,#32502,#10076,.T.) ;
#39656=EDGE_CURVE('',#32503,#32502,#27134,.T.) ;
#39657=EDGE_CURVE('',#32503,#32504,#10077,.T.) ;
#39658=EDGE_CURVE('',#32505,#32504,#27135,.T.) ;
#39659=EDGE_CURVE('',#32505,#32412,#10078,.T.) ;
#39660=EDGE_CURVE('',#32413,#32506,#10079,.T.) ;
#39661=EDGE_CURVE('',#32507,#32506,#27136,.T.) ;
#39662=EDGE_CURVE('',#32507,#32508,#10080,.T.) ;
#39663=EDGE_CURVE('',#32509,#32508,#27137,.T.) ;
#39664=EDGE_CURVE('',#32509,#32408,#10081,.T.) ;
#39665=EDGE_CURVE('',#32409,#32510,#10082,.T.) ;
#39666=EDGE_CURVE('',#32511,#32510,#27138,.T.) ;
#39667=EDGE_CURVE('',#32511,#32512,#10083,.T.) ;
#39668=EDGE_CURVE('',#32513,#32512,#27139,.T.) ;
#39669=EDGE_CURVE('',#32513,#32404,#10084,.T.) ;
#39670=EDGE_CURVE('',#32405,#32514,#10085,.T.) ;
#39671=EDGE_CURVE('',#32515,#32514,#27140,.T.) ;
#39672=EDGE_CURVE('',#32515,#32516,#10086,.T.) ;
#39673=EDGE_CURVE('',#32517,#32516,#27141,.T.) ;
#39674=EDGE_CURVE('',#32517,#32400,#10087,.T.) ;
#39675=EDGE_CURVE('',#32401,#32518,#10088,.T.) ;
#39676=EDGE_CURVE('',#32519,#32518,#27142,.T.) ;
#39677=EDGE_CURVE('',#32519,#32520,#10089,.T.) ;
#39678=EDGE_CURVE('',#32521,#32520,#27143,.T.) ;
#39679=EDGE_CURVE('',#32521,#32396,#10090,.T.) ;
#39680=EDGE_CURVE('',#32397,#32522,#10091,.T.) ;
#39681=EDGE_CURVE('',#32523,#32522,#27144,.T.) ;
#39682=EDGE_CURVE('',#32523,#32524,#10092,.T.) ;
#39683=EDGE_CURVE('',#32525,#32524,#27145,.T.) ;
#39684=EDGE_CURVE('',#32525,#32392,#10093,.T.) ;
#39685=EDGE_CURVE('',#32393,#32526,#10094,.T.) ;
#39686=EDGE_CURVE('',#32527,#32526,#27146,.T.) ;
#39687=EDGE_CURVE('',#32527,#32528,#10095,.T.) ;
#39688=EDGE_CURVE('',#32529,#32528,#27147,.T.) ;
#39689=EDGE_CURVE('',#32529,#32388,#10096,.T.) ;
#39690=EDGE_CURVE('',#32389,#32530,#10097,.T.) ;
#39691=EDGE_CURVE('',#32531,#32530,#27148,.T.) ;
#39692=EDGE_CURVE('',#32531,#32532,#10098,.T.) ;
#39693=EDGE_CURVE('',#32533,#32532,#27149,.T.) ;
#39694=EDGE_CURVE('',#32533,#32444,#10099,.T.) ;
#39695=EDGE_CURVE('',#32445,#32534,#10100,.T.) ;
#39696=EDGE_CURVE('',#32535,#32534,#10101,.T.) ;
#39697=EDGE_CURVE('',#32535,#32495,#10102,.T.) ;
#39698=EDGE_CURVE('',#32494,#32536,#10103,.T.) ;
#39699=EDGE_CURVE('',#32537,#32536,#27150,.T.) ;
#39700=EDGE_CURVE('',#32537,#32497,#10104,.T.) ;
#39701=EDGE_CURVE('',#32538,#32539,#10105,.T.) ;
#39702=EDGE_CURVE('',#32538,#32535,#27151,.T.) ;
#39703=EDGE_CURVE('',#32534,#32539,#27152,.T.) ;
#39704=EDGE_CURVE('',#32540,#32541,#10106,.T.) ;
#39705=EDGE_CURVE('',#32540,#32538,#10107,.T.) ;
#39706=EDGE_CURVE('',#32539,#32541,#10108,.T.) ;
#39707=EDGE_CURVE('',#32542,#32543,#10109,.T.) ;
#39708=EDGE_CURVE('',#32542,#32540,#27153,.T.) ;
#39709=EDGE_CURVE('',#32541,#32543,#27154,.T.) ;
#39710=EDGE_CURVE('',#32544,#32545,#10110,.T.) ;
#39711=EDGE_CURVE('',#32544,#32542,#10111,.T.) ;
#39712=EDGE_CURVE('',#32543,#32545,#10112,.T.) ;
#39713=EDGE_CURVE('',#32546,#32547,#10113,.T.) ;
#39714=EDGE_CURVE('',#32546,#32544,#27155,.T.) ;
#39715=EDGE_CURVE('',#32545,#32547,#27156,.T.) ;
#39716=EDGE_CURVE('',#32548,#32549,#10114,.T.) ;
#39717=EDGE_CURVE('',#32548,#32546,#10115,.T.) ;
#39718=EDGE_CURVE('',#32547,#32549,#10116,.T.) ;
#39719=EDGE_CURVE('',#32550,#32551,#10117,.T.) ;
#39720=EDGE_CURVE('',#32550,#32548,#27157,.T.) ;
#39721=EDGE_CURVE('',#32549,#32551,#27158,.T.) ;
#39722=EDGE_CURVE('',#32552,#32553,#10118,.T.) ;
#39723=EDGE_CURVE('',#32552,#32550,#10119,.T.) ;
#39724=EDGE_CURVE('',#32551,#32553,#10120,.T.) ;
#39725=EDGE_CURVE('',#32554,#32555,#10121,.T.) ;
#39726=EDGE_CURVE('',#32554,#32552,#27159,.T.) ;
#39727=EDGE_CURVE('',#32553,#32555,#27160,.T.) ;
#39728=EDGE_CURVE('',#32556,#32557,#10122,.T.) ;
#39729=EDGE_CURVE('',#32556,#32554,#10123,.T.) ;
#39730=EDGE_CURVE('',#32555,#32557,#10124,.T.) ;
#39731=EDGE_CURVE('',#32558,#32559,#10125,.T.) ;
#39732=EDGE_CURVE('',#32558,#32556,#27161,.T.) ;
#39733=EDGE_CURVE('',#32557,#32559,#27162,.T.) ;
#39734=EDGE_CURVE('',#32450,#32558,#10126,.T.) ;
#39735=EDGE_CURVE('',#32559,#32451,#10127,.T.) ;
#39736=EDGE_CURVE('',#32560,#32561,#27163,.T.) ;
#39737=EDGE_CURVE('',#32561,#32562,#10128,.T.) ;
#39738=EDGE_CURVE('',#32562,#32563,#10129,.T.) ;
#39739=EDGE_CURVE('',#32563,#32564,#10130,.T.) ;
#39740=EDGE_CURVE('',#32564,#32565,#27164,.T.) ;
#39741=EDGE_CURVE('',#32565,#32566,#10131,.T.) ;
#39742=EDGE_CURVE('',#32566,#32567,#27165,.T.) ;
#39743=EDGE_CURVE('',#32567,#32153,#10132,.T.) ;
#39744=EDGE_CURVE('',#32154,#32568,#10133,.T.) ;
#39745=EDGE_CURVE('',#32568,#32569,#27166,.T.) ;
#39746=EDGE_CURVE('',#32569,#32570,#10134,.T.) ;
#39747=EDGE_CURVE('',#32570,#32571,#10135,.T.) ;
#39748=EDGE_CURVE('',#32571,#32572,#10136,.T.) ;
#39749=EDGE_CURVE('',#32572,#32573,#27167,.T.) ;
#39750=EDGE_CURVE('',#32573,#32574,#10137,.T.) ;
#39751=EDGE_CURVE('',#32574,#32575,#27168,.T.) ;
#39752=EDGE_CURVE('',#32575,#32576,#10138,.T.) ;
#39753=EDGE_CURVE('',#32576,#32577,#27169,.T.) ;
#39754=EDGE_CURVE('',#32577,#32578,#27170,.T.) ;
#39755=EDGE_CURVE('',#32578,#32579,#27171,.T.) ;
#39756=EDGE_CURVE('',#32579,#32580,#10139,.T.) ;
#39757=EDGE_CURVE('',#32580,#32581,#27172,.T.) ;
#39758=EDGE_CURVE('',#32581,#32560,#10140,.T.) ;
#39759=EDGE_CURVE('',#32582,#32583,#27173,.T.) ;
#39760=EDGE_CURVE('',#32583,#32584,#10141,.T.) ;
#39761=EDGE_CURVE('',#32584,#32585,#10142,.T.) ;
#39762=EDGE_CURVE('',#32585,#32586,#10143,.T.) ;
#39763=EDGE_CURVE('',#32586,#32587,#27174,.T.) ;
#39764=EDGE_CURVE('',#32587,#32588,#10144,.T.) ;
#39765=EDGE_CURVE('',#32588,#32589,#27175,.T.) ;
#39766=EDGE_CURVE('',#32589,#32149,#10145,.T.) ;
#39767=EDGE_CURVE('',#32150,#32590,#10146,.T.) ;
#39768=EDGE_CURVE('',#32590,#32591,#27176,.T.) ;
#39769=EDGE_CURVE('',#32591,#32592,#10147,.T.) ;
#39770=EDGE_CURVE('',#32592,#32593,#10148,.T.) ;
#39771=EDGE_CURVE('',#32593,#32594,#10149,.T.) ;
#39772=EDGE_CURVE('',#32594,#32595,#27177,.T.) ;
#39773=EDGE_CURVE('',#32595,#32596,#10150,.T.) ;
#39774=EDGE_CURVE('',#32596,#32597,#27178,.T.) ;
#39775=EDGE_CURVE('',#32597,#32598,#10151,.T.) ;
#39776=EDGE_CURVE('',#32598,#32599,#27179,.T.) ;
#39777=EDGE_CURVE('',#32599,#32600,#27180,.T.) ;
#39778=EDGE_CURVE('',#32600,#32601,#27181,.T.) ;
#39779=EDGE_CURVE('',#32601,#32602,#10152,.T.) ;
#39780=EDGE_CURVE('',#32602,#32603,#27182,.T.) ;
#39781=EDGE_CURVE('',#32603,#32582,#10153,.T.) ;
#39782=EDGE_CURVE('',#32604,#32605,#27183,.T.) ;
#39783=EDGE_CURVE('',#32605,#32606,#10154,.T.) ;
#39784=EDGE_CURVE('',#32606,#32607,#10155,.T.) ;
#39785=EDGE_CURVE('',#32607,#32608,#10156,.T.) ;
#39786=EDGE_CURVE('',#32608,#32609,#27184,.T.) ;
#39787=EDGE_CURVE('',#32609,#32610,#10157,.T.) ;
#39788=EDGE_CURVE('',#32610,#32611,#27185,.T.) ;
#39789=EDGE_CURVE('',#32611,#32145,#10158,.T.) ;
#39790=EDGE_CURVE('',#32146,#32612,#10159,.T.) ;
#39791=EDGE_CURVE('',#32612,#32613,#27186,.T.) ;
#39792=EDGE_CURVE('',#32613,#32614,#10160,.T.) ;
#39793=EDGE_CURVE('',#32614,#32615,#10161,.T.) ;
#39794=EDGE_CURVE('',#32615,#32616,#10162,.T.) ;
#39795=EDGE_CURVE('',#32616,#32617,#27187,.T.) ;
#39796=EDGE_CURVE('',#32617,#32618,#10163,.T.) ;
#39797=EDGE_CURVE('',#32618,#32619,#27188,.T.) ;
#39798=EDGE_CURVE('',#32619,#32620,#10164,.T.) ;
#39799=EDGE_CURVE('',#32620,#32621,#27189,.T.) ;
#39800=EDGE_CURVE('',#32621,#32622,#27190,.T.) ;
#39801=EDGE_CURVE('',#32622,#32623,#27191,.T.) ;
#39802=EDGE_CURVE('',#32623,#32624,#10165,.T.) ;
#39803=EDGE_CURVE('',#32624,#32625,#27192,.T.) ;
#39804=EDGE_CURVE('',#32625,#32604,#10166,.T.) ;
#39805=EDGE_CURVE('',#32626,#32627,#27193,.T.) ;
#39806=EDGE_CURVE('',#32627,#32628,#10167,.T.) ;
#39807=EDGE_CURVE('',#32628,#32629,#10168,.T.) ;
#39808=EDGE_CURVE('',#32629,#32630,#10169,.T.) ;
#39809=EDGE_CURVE('',#32630,#32631,#27194,.T.) ;
#39810=EDGE_CURVE('',#32631,#32632,#10170,.T.) ;
#39811=EDGE_CURVE('',#32632,#32633,#27195,.T.) ;
#39812=EDGE_CURVE('',#32633,#32141,#10171,.T.) ;
#39813=EDGE_CURVE('',#32142,#32634,#10172,.T.) ;
#39814=EDGE_CURVE('',#32634,#32635,#27196,.T.) ;
#39815=EDGE_CURVE('',#32635,#32636,#10173,.T.) ;
#39816=EDGE_CURVE('',#32636,#32637,#10174,.T.) ;
#39817=EDGE_CURVE('',#32637,#32638,#10175,.T.) ;
#39818=EDGE_CURVE('',#32638,#32639,#27197,.T.) ;
#39819=EDGE_CURVE('',#32639,#32640,#10176,.T.) ;
#39820=EDGE_CURVE('',#32640,#32641,#27198,.T.) ;
#39821=EDGE_CURVE('',#32641,#32642,#10177,.T.) ;
#39822=EDGE_CURVE('',#32642,#32643,#27199,.T.) ;
#39823=EDGE_CURVE('',#32643,#32644,#27200,.T.) ;
#39824=EDGE_CURVE('',#32644,#32645,#27201,.T.) ;
#39825=EDGE_CURVE('',#32645,#32646,#10178,.T.) ;
#39826=EDGE_CURVE('',#32646,#32647,#27202,.T.) ;
#39827=EDGE_CURVE('',#32647,#32626,#10179,.T.) ;
#39828=EDGE_CURVE('',#32648,#32649,#27203,.T.) ;
#39829=EDGE_CURVE('',#32649,#32650,#10180,.T.) ;
#39830=EDGE_CURVE('',#32650,#32651,#10181,.T.) ;
#39831=EDGE_CURVE('',#32651,#32652,#10182,.T.) ;
#39832=EDGE_CURVE('',#32652,#32653,#27204,.T.) ;
#39833=EDGE_CURVE('',#32653,#32654,#10183,.T.) ;
#39834=EDGE_CURVE('',#32654,#32655,#27205,.T.) ;
#39835=EDGE_CURVE('',#32655,#32137,#10184,.T.) ;
#39836=EDGE_CURVE('',#32138,#32656,#10185,.T.) ;
#39837=EDGE_CURVE('',#32656,#32657,#27206,.T.) ;
#39838=EDGE_CURVE('',#32657,#32658,#10186,.T.) ;
#39839=EDGE_CURVE('',#32658,#32659,#10187,.T.) ;
#39840=EDGE_CURVE('',#32659,#32660,#10188,.T.) ;
#39841=EDGE_CURVE('',#32660,#32661,#27207,.T.) ;
#39842=EDGE_CURVE('',#32661,#32662,#10189,.T.) ;
#39843=EDGE_CURVE('',#32662,#32663,#27208,.T.) ;
#39844=EDGE_CURVE('',#32663,#32664,#10190,.T.) ;
#39845=EDGE_CURVE('',#32664,#32665,#27209,.T.) ;
#39846=EDGE_CURVE('',#32665,#32666,#27210,.T.) ;
#39847=EDGE_CURVE('',#32666,#32667,#27211,.T.) ;
#39848=EDGE_CURVE('',#32667,#32668,#10191,.T.) ;
#39849=EDGE_CURVE('',#32668,#32669,#27212,.T.) ;
#39850=EDGE_CURVE('',#32669,#32648,#10192,.T.) ;
#39851=EDGE_CURVE('',#32670,#32671,#27213,.T.) ;
#39852=EDGE_CURVE('',#32671,#32672,#10193,.T.) ;
#39853=EDGE_CURVE('',#32672,#32673,#10194,.T.) ;
#39854=EDGE_CURVE('',#32673,#32674,#10195,.T.) ;
#39855=EDGE_CURVE('',#32674,#32675,#27214,.T.) ;
#39856=EDGE_CURVE('',#32675,#32676,#10196,.T.) ;
#39857=EDGE_CURVE('',#32676,#32677,#27215,.T.) ;
#39858=EDGE_CURVE('',#32677,#32133,#10197,.T.) ;
#39859=EDGE_CURVE('',#32134,#32678,#10198,.T.) ;
#39860=EDGE_CURVE('',#32678,#32679,#27216,.T.) ;
#39861=EDGE_CURVE('',#32679,#32680,#10199,.T.) ;
#39862=EDGE_CURVE('',#32680,#32681,#10200,.T.) ;
#39863=EDGE_CURVE('',#32681,#32682,#10201,.T.) ;
#39864=EDGE_CURVE('',#32682,#32683,#27217,.T.) ;
#39865=EDGE_CURVE('',#32683,#32684,#10202,.T.) ;
#39866=EDGE_CURVE('',#32684,#32685,#27218,.T.) ;
#39867=EDGE_CURVE('',#32685,#32686,#10203,.T.) ;
#39868=EDGE_CURVE('',#32686,#32687,#27219,.T.) ;
#39869=EDGE_CURVE('',#32687,#32688,#27220,.T.) ;
#39870=EDGE_CURVE('',#32688,#32689,#27221,.T.) ;
#39871=EDGE_CURVE('',#32689,#32690,#10204,.T.) ;
#39872=EDGE_CURVE('',#32690,#32691,#27222,.T.) ;
#39873=EDGE_CURVE('',#32691,#32670,#10205,.T.) ;
#39874=EDGE_CURVE('',#32692,#32693,#27223,.T.) ;
#39875=EDGE_CURVE('',#32693,#32694,#10206,.T.) ;
#39876=EDGE_CURVE('',#32694,#32695,#10207,.T.) ;
#39877=EDGE_CURVE('',#32695,#32696,#10208,.T.) ;
#39878=EDGE_CURVE('',#32696,#32697,#27224,.T.) ;
#39879=EDGE_CURVE('',#32697,#32698,#10209,.T.) ;
#39880=EDGE_CURVE('',#32698,#32699,#27225,.T.) ;
#39881=EDGE_CURVE('',#32699,#32129,#10210,.T.) ;
#39882=EDGE_CURVE('',#32130,#32700,#10211,.T.) ;
#39883=EDGE_CURVE('',#32700,#32701,#27226,.T.) ;
#39884=EDGE_CURVE('',#32701,#32702,#10212,.T.) ;
#39885=EDGE_CURVE('',#32702,#32703,#10213,.T.) ;
#39886=EDGE_CURVE('',#32703,#32704,#10214,.T.) ;
#39887=EDGE_CURVE('',#32704,#32705,#27227,.T.) ;
#39888=EDGE_CURVE('',#32705,#32706,#10215,.T.) ;
#39889=EDGE_CURVE('',#32706,#32707,#27228,.T.) ;
#39890=EDGE_CURVE('',#32707,#32708,#10216,.T.) ;
#39891=EDGE_CURVE('',#32708,#32709,#27229,.T.) ;
#39892=EDGE_CURVE('',#32709,#32710,#27230,.T.) ;
#39893=EDGE_CURVE('',#32710,#32711,#27231,.T.) ;
#39894=EDGE_CURVE('',#32711,#32712,#10217,.T.) ;
#39895=EDGE_CURVE('',#32712,#32713,#27232,.T.) ;
#39896=EDGE_CURVE('',#32713,#32692,#10218,.T.) ;
#39897=EDGE_CURVE('',#32714,#32715,#27233,.T.) ;
#39898=EDGE_CURVE('',#32715,#32716,#10219,.T.) ;
#39899=EDGE_CURVE('',#32716,#32717,#10220,.T.) ;
#39900=EDGE_CURVE('',#32717,#32718,#10221,.T.) ;
#39901=EDGE_CURVE('',#32718,#32719,#27234,.T.) ;
#39902=EDGE_CURVE('',#32719,#32720,#10222,.T.) ;
#39903=EDGE_CURVE('',#32720,#32721,#27235,.T.) ;
#39904=EDGE_CURVE('',#32721,#32125,#10223,.T.) ;
#39905=EDGE_CURVE('',#32126,#32722,#10224,.T.) ;
#39906=EDGE_CURVE('',#32722,#32723,#27236,.T.) ;
#39907=EDGE_CURVE('',#32723,#32724,#10225,.T.) ;
#39908=EDGE_CURVE('',#32724,#32725,#10226,.T.) ;
#39909=EDGE_CURVE('',#32725,#32726,#10227,.T.) ;
#39910=EDGE_CURVE('',#32726,#32727,#27237,.T.) ;
#39911=EDGE_CURVE('',#32727,#32728,#10228,.T.) ;
#39912=EDGE_CURVE('',#32728,#32729,#27238,.T.) ;
#39913=EDGE_CURVE('',#32729,#32730,#10229,.T.) ;
#39914=EDGE_CURVE('',#32730,#32731,#27239,.T.) ;
#39915=EDGE_CURVE('',#32731,#32732,#27240,.T.) ;
#39916=EDGE_CURVE('',#32732,#32733,#27241,.T.) ;
#39917=EDGE_CURVE('',#32733,#32734,#10230,.T.) ;
#39918=EDGE_CURVE('',#32734,#32735,#27242,.T.) ;
#39919=EDGE_CURVE('',#32735,#32714,#10231,.T.) ;
#39920=EDGE_CURVE('',#32736,#32737,#27243,.T.) ;
#39921=EDGE_CURVE('',#32737,#32738,#10232,.T.) ;
#39922=EDGE_CURVE('',#32738,#32739,#10233,.T.) ;
#39923=EDGE_CURVE('',#32739,#32740,#10234,.T.) ;
#39924=EDGE_CURVE('',#32740,#32741,#27244,.T.) ;
#39925=EDGE_CURVE('',#32741,#32742,#10235,.T.) ;
#39926=EDGE_CURVE('',#32742,#32743,#27245,.T.) ;
#39927=EDGE_CURVE('',#32743,#32121,#10236,.T.) ;
#39928=EDGE_CURVE('',#32122,#32744,#10237,.T.) ;
#39929=EDGE_CURVE('',#32744,#32745,#27246,.T.) ;
#39930=EDGE_CURVE('',#32745,#32746,#10238,.T.) ;
#39931=EDGE_CURVE('',#32746,#32747,#10239,.T.) ;
#39932=EDGE_CURVE('',#32747,#32748,#10240,.T.) ;
#39933=EDGE_CURVE('',#32748,#32749,#27247,.T.) ;
#39934=EDGE_CURVE('',#32749,#32750,#10241,.T.) ;
#39935=EDGE_CURVE('',#32750,#32751,#27248,.T.) ;
#39936=EDGE_CURVE('',#32751,#32752,#10242,.T.) ;
#39937=EDGE_CURVE('',#32752,#32753,#27249,.T.) ;
#39938=EDGE_CURVE('',#32753,#32754,#27250,.T.) ;
#39939=EDGE_CURVE('',#32754,#32755,#27251,.T.) ;
#39940=EDGE_CURVE('',#32755,#32756,#10243,.T.) ;
#39941=EDGE_CURVE('',#32756,#32757,#27252,.T.) ;
#39942=EDGE_CURVE('',#32757,#32736,#10244,.T.) ;
#39943=EDGE_CURVE('',#32758,#32759,#27253,.T.) ;
#39944=EDGE_CURVE('',#32759,#32760,#10245,.T.) ;
#39945=EDGE_CURVE('',#32760,#32761,#10246,.T.) ;
#39946=EDGE_CURVE('',#32761,#32762,#10247,.T.) ;
#39947=EDGE_CURVE('',#32762,#32763,#27254,.T.) ;
#39948=EDGE_CURVE('',#32763,#32764,#10248,.T.) ;
#39949=EDGE_CURVE('',#32764,#32765,#27255,.T.) ;
#39950=EDGE_CURVE('',#32765,#32190,#10249,.T.) ;
#39951=EDGE_CURVE('',#32191,#32766,#10250,.T.) ;
#39952=EDGE_CURVE('',#32766,#32767,#27256,.T.) ;
#39953=EDGE_CURVE('',#32767,#32768,#10251,.T.) ;
#39954=EDGE_CURVE('',#32768,#32769,#10252,.T.) ;
#39955=EDGE_CURVE('',#32769,#32770,#10253,.T.) ;
#39956=EDGE_CURVE('',#32770,#32771,#27257,.T.) ;
#39957=EDGE_CURVE('',#32771,#32772,#10254,.T.) ;
#39958=EDGE_CURVE('',#32772,#32773,#27258,.T.) ;
#39959=EDGE_CURVE('',#32773,#32774,#10255,.T.) ;
#39960=EDGE_CURVE('',#32774,#32775,#27259,.T.) ;
#39961=EDGE_CURVE('',#32775,#32776,#27260,.T.) ;
#39962=EDGE_CURVE('',#32776,#32777,#27261,.T.) ;
#39963=EDGE_CURVE('',#32777,#32778,#10256,.T.) ;
#39964=EDGE_CURVE('',#32778,#32779,#27262,.T.) ;
#39965=EDGE_CURVE('',#32779,#32758,#10257,.T.) ;
#39966=EDGE_CURVE('',#32780,#32781,#10258,.T.) ;
#39967=EDGE_CURVE('',#32781,#32782,#10259,.T.) ;
#39968=EDGE_CURVE('',#32782,#32783,#10260,.T.) ;
#39969=EDGE_CURVE('',#32783,#32784,#10261,.T.) ;
#39970=EDGE_CURVE('',#32784,#32785,#27263,.T.) ;
#39971=EDGE_CURVE('',#32785,#32786,#10262,.T.) ;
#39972=EDGE_CURVE('',#32786,#32787,#10263,.T.) ;
#39973=EDGE_CURVE('',#32787,#32788,#10264,.T.) ;
#39974=EDGE_CURVE('',#32788,#32789,#27264,.T.) ;
#39975=EDGE_CURVE('',#32789,#32780,#10265,.T.) ;
#39976=EDGE_CURVE('',#32790,#32791,#10266,.T.) ;
#39977=EDGE_CURVE('',#32791,#32792,#10267,.T.) ;
#39978=EDGE_CURVE('',#32792,#32793,#10268,.T.) ;
#39979=EDGE_CURVE('',#32793,#32794,#10269,.T.) ;
#39980=EDGE_CURVE('',#32794,#32795,#27265,.T.) ;
#39981=EDGE_CURVE('',#32795,#32796,#10270,.T.) ;
#39982=EDGE_CURVE('',#32796,#32797,#10271,.T.) ;
#39983=EDGE_CURVE('',#32797,#32798,#10272,.T.) ;
#39984=EDGE_CURVE('',#32798,#32799,#27266,.T.) ;
#39985=EDGE_CURVE('',#32799,#32790,#10273,.T.) ;
#39986=EDGE_CURVE('',#32800,#32801,#10274,.T.) ;
#39987=EDGE_CURVE('',#32801,#32802,#10275,.T.) ;
#39988=EDGE_CURVE('',#32802,#32803,#10276,.T.) ;
#39989=EDGE_CURVE('',#32803,#32804,#10277,.T.) ;
#39990=EDGE_CURVE('',#32804,#32805,#10278,.T.) ;
#39991=EDGE_CURVE('',#32805,#32806,#10279,.T.) ;
#39992=EDGE_CURVE('',#32807,#32806,#27267,.T.) ;
#39993=EDGE_CURVE('',#32807,#32808,#10280,.T.) ;
#39994=EDGE_CURVE('',#32809,#32808,#27268,.T.) ;
#39995=EDGE_CURVE('',#32809,#32800,#10281,.T.) ;
#39996=EDGE_CURVE('',#32810,#32811,#10282,.T.) ;
#39997=EDGE_CURVE('',#32811,#32812,#10283,.T.) ;
#39998=EDGE_CURVE('',#32812,#32813,#10284,.T.) ;
#39999=EDGE_CURVE('',#32813,#32810,#10285,.T.) ;
#40000=EDGE_CURVE('',#32201,#32814,#10286,.T.) ;
#40001=EDGE_CURVE('',#32814,#32815,#10287,.T.) ;
#40002=EDGE_CURVE('',#32815,#32202,#10288,.T.) ;
#40003=EDGE_CURVE('',#32816,#32817,#10289,.T.) ;
#40004=EDGE_CURVE('',#32817,#32818,#10290,.T.) ;
#40005=EDGE_CURVE('',#32818,#32819,#10291,.T.) ;
#40006=EDGE_CURVE('',#32819,#32816,#10292,.T.) ;
#40007=EDGE_CURVE('',#32820,#32821,#10293,.T.) ;
#40008=EDGE_CURVE('',#32821,#32822,#10294,.T.) ;
#40009=EDGE_CURVE('',#32822,#32823,#10295,.T.) ;
#40010=EDGE_CURVE('',#32823,#32820,#10296,.T.) ;
#40011=EDGE_CURVE('',#32824,#32825,#10297,.T.) ;
#40012=EDGE_CURVE('',#32825,#32826,#10298,.T.) ;
#40013=EDGE_CURVE('',#32826,#32827,#10299,.T.) ;
#40014=EDGE_CURVE('',#32827,#32824,#10300,.T.) ;
#40015=EDGE_CURVE('',#32828,#32829,#10301,.T.) ;
#40016=EDGE_CURVE('',#32828,#32830,#27269,.T.) ;
#40017=EDGE_CURVE('',#32830,#32831,#10302,.T.) ;
#40018=EDGE_CURVE('',#32831,#32829,#27270,.T.) ;
#40019=EDGE_CURVE('',#32830,#32832,#10303,.T.) ;
#40020=EDGE_CURVE('',#32832,#32833,#10304,.T.) ;
#40021=EDGE_CURVE('',#32833,#32831,#10305,.T.) ;
#40022=EDGE_CURVE('',#32832,#32834,#27271,.T.) ;
#40023=EDGE_CURVE('',#32834,#32835,#10306,.T.) ;
#40024=EDGE_CURVE('',#32835,#32833,#27272,.T.) ;
#40025=EDGE_CURVE('',#32834,#32836,#10307,.T.) ;
#40026=EDGE_CURVE('',#32836,#32837,#10308,.T.) ;
#40027=EDGE_CURVE('',#32837,#32835,#10309,.T.) ;
#40028=EDGE_CURVE('',#32836,#32838,#27273,.T.) ;
#40029=EDGE_CURVE('',#32838,#32839,#10310,.T.) ;
#40030=EDGE_CURVE('',#32839,#32837,#27274,.T.) ;
#40031=EDGE_CURVE('',#32838,#32196,#10311,.T.) ;
#40032=EDGE_CURVE('',#32196,#32840,#10312,.T.) ;
#40033=EDGE_CURVE('',#32840,#32839,#10313,.T.) ;
#40034=EDGE_CURVE('',#32197,#32841,#10314,.T.) ;
#40035=EDGE_CURVE('',#32841,#32840,#27275,.T.) ;
#40036=EDGE_CURVE('',#32197,#32206,#10315,.T.) ;
#40037=EDGE_CURVE('',#32192,#32841,#10316,.T.) ;
#40038=EDGE_CURVE('',#32207,#32842,#10317,.T.) ;
#40039=EDGE_CURVE('',#32842,#32843,#10318,.T.) ;
#40040=EDGE_CURVE('',#32843,#32193,#10319,.T.) ;
#40041=EDGE_CURVE('',#32842,#32844,#27276,.T.) ;
#40042=EDGE_CURVE('',#32844,#32845,#10320,.T.) ;
#40043=EDGE_CURVE('',#32845,#32843,#27277,.T.) ;
#40044=EDGE_CURVE('',#32844,#32846,#10321,.T.) ;
#40045=EDGE_CURVE('',#32846,#32847,#10322,.T.) ;
#40046=EDGE_CURVE('',#32847,#32845,#10323,.T.) ;
#40047=EDGE_CURVE('',#32846,#32848,#27278,.T.) ;
#40048=EDGE_CURVE('',#32848,#32849,#10324,.T.) ;
#40049=EDGE_CURVE('',#32849,#32847,#27279,.T.) ;
#40050=EDGE_CURVE('',#32848,#32850,#10325,.T.) ;
#40051=EDGE_CURVE('',#32850,#32851,#10326,.T.) ;
#40052=EDGE_CURVE('',#32851,#32849,#10327,.T.) ;
#40053=EDGE_CURVE('',#32850,#32852,#27280,.T.) ;
#40054=EDGE_CURVE('',#32852,#32853,#10328,.T.) ;
#40055=EDGE_CURVE('',#32853,#32851,#27281,.T.) ;
#40056=EDGE_CURVE('',#32852,#32854,#10329,.T.) ;
#40057=EDGE_CURVE('',#32854,#32855,#10330,.T.) ;
#40058=EDGE_CURVE('',#32855,#32853,#10331,.T.) ;
#40059=EDGE_CURVE('',#32854,#32856,#27282,.T.) ;
#40060=EDGE_CURVE('',#32856,#32857,#10332,.T.) ;
#40061=EDGE_CURVE('',#32857,#32855,#27283,.T.) ;
#40062=EDGE_CURVE('',#32856,#32858,#10333,.T.) ;
#40063=EDGE_CURVE('',#32858,#32859,#10334,.T.) ;
#40064=EDGE_CURVE('',#32859,#32857,#10335,.T.) ;
#40065=EDGE_CURVE('',#32858,#32860,#27284,.T.) ;
#40066=EDGE_CURVE('',#32860,#32861,#10336,.T.) ;
#40067=EDGE_CURVE('',#32861,#32859,#27285,.T.) ;
#40068=EDGE_CURVE('',#32860,#32862,#10337,.T.) ;
#40069=EDGE_CURVE('',#32862,#32863,#10338,.T.) ;
#40070=EDGE_CURVE('',#32863,#32861,#10339,.T.) ;
#40071=EDGE_CURVE('',#32862,#32864,#27286,.T.) ;
#40072=EDGE_CURVE('',#32864,#32865,#10340,.T.) ;
#40073=EDGE_CURVE('',#32865,#32863,#27287,.T.) ;
#40074=EDGE_CURVE('',#32864,#32866,#27288,.T.) ;
#40075=EDGE_CURVE('',#32866,#32867,#10341,.T.) ;
#40076=EDGE_CURVE('',#32867,#32865,#27289,.T.) ;
#40077=EDGE_CURVE('',#32866,#32868,#27290,.T.) ;
#40078=EDGE_CURVE('',#32868,#32869,#10342,.T.) ;
#40079=EDGE_CURVE('',#32869,#32867,#27291,.T.) ;
#40080=EDGE_CURVE('',#32868,#32870,#10343,.T.) ;
#40081=EDGE_CURVE('',#32870,#32871,#10344,.T.) ;
#40082=EDGE_CURVE('',#32871,#32869,#10345,.T.) ;
#40083=EDGE_CURVE('',#32870,#32872,#27292,.T.) ;
#40084=EDGE_CURVE('',#32872,#32873,#10346,.T.) ;
#40085=EDGE_CURVE('',#32873,#32871,#27293,.T.) ;
#40086=EDGE_CURVE('',#32872,#32874,#10347,.T.) ;
#40087=EDGE_CURVE('',#32874,#32875,#10348,.T.) ;
#40088=EDGE_CURVE('',#32875,#32873,#10349,.T.) ;
#40089=EDGE_CURVE('',#32874,#32876,#27294,.T.) ;
#40090=EDGE_CURVE('',#32876,#32877,#10350,.T.) ;
#40091=EDGE_CURVE('',#32877,#32875,#27295,.T.) ;
#40092=EDGE_CURVE('',#32876,#32828,#10351,.T.) ;
#40093=EDGE_CURVE('',#32829,#32877,#10352,.T.) ;
#40094=EDGE_CURVE('',#32878,#32879,#27296,.T.) ;
#40095=EDGE_CURVE('',#32879,#32880,#10353,.T.) ;
#40096=EDGE_CURVE('',#32880,#32881,#27297,.T.) ;
#40097=EDGE_CURVE('',#32881,#32882,#10354,.T.) ;
#40098=EDGE_CURVE('',#32882,#32883,#10355,.T.) ;
#40099=EDGE_CURVE('',#32883,#32884,#10356,.T.) ;
#40100=EDGE_CURVE('',#32884,#32885,#27298,.T.) ;
#40101=EDGE_CURVE('',#32885,#32886,#10357,.T.) ;
#40102=EDGE_CURVE('',#32886,#32887,#10358,.T.) ;
#40103=EDGE_CURVE('',#32887,#32888,#10359,.T.) ;
#40104=EDGE_CURVE('',#32888,#32889,#27299,.T.) ;
#40105=EDGE_CURVE('',#32889,#32890,#10360,.T.) ;
#40106=EDGE_CURVE('',#32890,#32891,#27300,.T.) ;
#40107=EDGE_CURVE('',#32891,#32892,#10361,.T.) ;
#40108=EDGE_CURVE('',#32892,#32893,#10362,.T.) ;
#40109=EDGE_CURVE('',#32893,#32198,#10363,.T.) ;
#40110=EDGE_CURVE('',#32198,#32894,#10364,.T.) ;
#40111=EDGE_CURVE('',#32894,#32878,#10365,.T.) ;
#40112=EDGE_CURVE('',#32895,#32896,#10366,.T.) ;
#40113=EDGE_CURVE('',#32895,#32897,#27301,.T.) ;
#40114=EDGE_CURVE('',#32897,#32898,#10367,.T.) ;
#40115=EDGE_CURVE('',#32898,#32899,#27302,.T.) ;
#40116=EDGE_CURVE('',#32899,#32900,#10368,.T.) ;
#40117=EDGE_CURVE('',#32900,#32901,#27303,.T.) ;
#40118=EDGE_CURVE('',#32901,#32902,#10369,.T.) ;
#40119=EDGE_CURVE('',#32902,#32896,#27304,.T.) ;
#40120=EDGE_CURVE('',#32822,#32809,#27305,.T.) ;
#40121=EDGE_CURVE('',#32800,#32821,#27306,.T.) ;
#40122=EDGE_CURVE('',#32823,#32816,#27307,.T.) ;
#40123=EDGE_CURVE('',#32817,#32822,#27308,.T.) ;
#40124=EDGE_CURVE('',#32823,#32903,#27309,.T.) ;
#40125=EDGE_CURVE('',#32903,#32816,#27310,.T.) ;
#40126=EDGE_CURVE('',#32800,#32826,#27311,.T.) ;
#40127=EDGE_CURVE('',#32826,#32821,#27312,.T.) ;
#40128=EDGE_CURVE('',#32817,#32808,#27313,.T.) ;
#40129=EDGE_CURVE('',#32199,#32819,#27314,.T.) ;
#40130=EDGE_CURVE('',#32200,#32904,#300,.T.) ;
#40131=EDGE_CURVE('',#32903,#32904,#10370,.T.) ;
#40132=EDGE_CURVE('',#32905,#32903,#301,.T.) ;
#40133=EDGE_CURVE('',#32905,#32906,#302,.T.) ;
#40134=EDGE_CURVE('',#32425,#32906,#10371,.T.) ;
#40135=EDGE_CURVE('',#32820,#32424,#27315,.T.) ;
#40136=EDGE_CURVE('',#32827,#32820,#27316,.T.) ;
#40137=EDGE_CURVE('',#32801,#32825,#27317,.T.) ;
#40138=EDGE_CURVE('',#32818,#32807,#27318,.T.) ;
#40139=EDGE_CURVE('',#32819,#32201,#27319,.T.) ;
#40140=EDGE_CURVE('',#32814,#32818,#27320,.T.) ;
#40141=EDGE_CURVE('',#32827,#32433,#27321,.T.) ;
#40142=EDGE_CURVE('',#32801,#32440,#27322,.T.) ;
#40143=EDGE_CURVE('',#32439,#32825,#27323,.T.) ;
#40144=EDGE_CURVE('',#32814,#32806,#27324,.T.) ;
#40145=EDGE_CURVE('',#32824,#32432,#27325,.T.) ;
#40146=EDGE_CURVE('',#32441,#32824,#27326,.T.) ;
#40147=EDGE_CURVE('',#32907,#32440,#10372,.T.) ;
#40148=EDGE_CURVE('',#32802,#32907,#27327,.T.) ;
#40149=EDGE_CURVE('',#32815,#32805,#27328,.T.) ;
#40150=EDGE_CURVE('',#32202,#32810,#27329,.T.) ;
#40151=EDGE_CURVE('',#32811,#32815,#27330,.T.) ;
#40152=EDGE_CURVE('',#32428,#32810,#27331,.T.) ;
#40153=EDGE_CURVE('',#32441,#32432,#27332,.T.) ;
#40154=EDGE_CURVE('',#32446,#32443,#27333,.T.) ;
#40155=EDGE_CURVE('',#32443,#32444,#27334,.T.) ;
#40156=EDGE_CURVE('',#32907,#32533,#27335,.T.) ;
#40157=EDGE_CURVE('',#32908,#32907,#27336,.T.) ;
#40158=EDGE_CURVE('',#32802,#32908,#27337,.T.) ;
#40159=EDGE_CURVE('',#32811,#32805,#27338,.T.) ;
#40160=EDGE_CURVE('',#32429,#32813,#27339,.T.) ;
#40161=EDGE_CURVE('',#32442,#32431,#27340,.T.) ;
#40162=EDGE_CURVE('',#32456,#32442,#27341,.T.) ;
#40163=EDGE_CURVE('',#32908,#32532,#27342,.T.) ;
#40164=EDGE_CURVE('',#32909,#32908,#10373,.T.) ;
#40165=EDGE_CURVE('',#32803,#32909,#27343,.T.) ;
#40166=EDGE_CURVE('',#32812,#32804,#27344,.T.) ;
#40167=EDGE_CURVE('',#32813,#32438,#27345,.T.) ;
#40168=EDGE_CURVE('',#32435,#32812,#27346,.T.) ;
#40169=EDGE_CURVE('',#32429,#32438,#27347,.T.) ;
#40170=EDGE_CURVE('',#32457,#32431,#27348,.T.) ;
#40171=EDGE_CURVE('',#32909,#32531,#27349,.T.) ;
#40172=EDGE_CURVE('',#32910,#32909,#27350,.T.) ;
#40173=EDGE_CURVE('',#32803,#32910,#27351,.T.) ;
#40174=EDGE_CURVE('',#32434,#32804,#27352,.T.) ;
#40175=EDGE_CURVE('',#32430,#32437,#27353,.T.) ;
#40176=EDGE_CURVE('',#32458,#32430,#27354,.T.) ;
#40177=EDGE_CURVE('',#32910,#32530,#27355,.T.) ;
#40178=EDGE_CURVE('',#32434,#32910,#10374,.T.) ;
#40179=EDGE_CURVE('',#32459,#32437,#27356,.T.) ;
#40180=EDGE_CURVE('',#32436,#32389,#27357,.T.) ;
#40181=EDGE_CURVE('',#32391,#32436,#27358,.T.) ;
#40182=EDGE_CURVE('',#32786,#32546,#27359,.T.) ;
#40183=EDGE_CURVE('',#32544,#32786,#27360,.T.) ;
#40184=EDGE_CURVE('',#32542,#32785,#27361,.T.) ;
#40185=EDGE_CURVE('',#32787,#32548,#27362,.T.) ;
#40186=EDGE_CURVE('',#32540,#32784,#27363,.T.) ;
#40187=EDGE_CURVE('',#32787,#32550,#27364,.T.) ;
#40188=EDGE_CURVE('',#32538,#32783,#27365,.T.) ;
#40189=EDGE_CURVE('',#32788,#32552,#27366,.T.) ;
#40190=EDGE_CURVE('',#32535,#32783,#27367,.T.) ;
#40191=EDGE_CURVE('',#32789,#32554,#27368,.T.) ;
#40192=EDGE_CURVE('',#32495,#32782,#27369,.T.) ;
#40193=EDGE_CURVE('',#32780,#32556,#27370,.T.) ;
#40194=EDGE_CURVE('',#32455,#32782,#27371,.T.) ;
#40195=EDGE_CURVE('',#32780,#32558,#27372,.T.) ;
#40196=EDGE_CURVE('',#32448,#32781,#27373,.T.) ;
#40197=EDGE_CURVE('',#32781,#32450,#27374,.T.) ;
#40198=EDGE_CURVE('',#32547,#32797,#27375,.T.) ;
#40199=EDGE_CURVE('',#32797,#32545,#27376,.T.) ;
#40200=EDGE_CURVE('',#32798,#32543,#27377,.T.) ;
#40201=EDGE_CURVE('',#32549,#32796,#27378,.T.) ;
#40202=EDGE_CURVE('',#32799,#32541,#27379,.T.) ;
#40203=EDGE_CURVE('',#32551,#32796,#27380,.T.) ;
#40204=EDGE_CURVE('',#32790,#32539,#27381,.T.) ;
#40205=EDGE_CURVE('',#32553,#32795,#27382,.T.) ;
#40206=EDGE_CURVE('',#32790,#32534,#27383,.T.) ;
#40207=EDGE_CURVE('',#32555,#32794,#27384,.T.) ;
#40208=EDGE_CURVE('',#32791,#32445,#27385,.T.) ;
#40209=EDGE_CURVE('',#32557,#32793,#27386,.T.) ;
#40210=EDGE_CURVE('',#32791,#32447,#27387,.T.) ;
#40211=EDGE_CURVE('',#32559,#32793,#27388,.T.) ;
#40212=EDGE_CURVE('',#32792,#32449,#27389,.T.) ;
#40213=EDGE_CURVE('',#32451,#32792,#27390,.T.) ;
#40214=EDGE_CURVE('',#32854,#32887,#27391,.T.) ;
#40215=EDGE_CURVE('',#32888,#32852,#27392,.T.) ;
#40216=EDGE_CURVE('',#32889,#32850,#27393,.T.) ;
#40217=EDGE_CURVE('',#32856,#32887,#27394,.T.) ;
#40218=EDGE_CURVE('',#32890,#32848,#27395,.T.) ;
#40219=EDGE_CURVE('',#32858,#32886,#27396,.T.) ;
#40220=EDGE_CURVE('',#32891,#32846,#27397,.T.) ;
#40221=EDGE_CURVE('',#32860,#32886,#27398,.T.) ;
#40222=EDGE_CURVE('',#32892,#32844,#27399,.T.) ;
#40223=EDGE_CURVE('',#32862,#32885,#27400,.T.) ;
#40224=EDGE_CURVE('',#32892,#32842,#27401,.T.) ;
#40225=EDGE_CURVE('',#32864,#32885,#27402,.T.) ;
#40226=EDGE_CURVE('',#32893,#32207,#27403,.T.) ;
#40227=EDGE_CURVE('',#32866,#32884,#27404,.T.) ;
#40228=EDGE_CURVE('',#32893,#32206,#27405,.T.) ;
#40229=EDGE_CURVE('',#32868,#32884,#27406,.T.) ;
#40230=EDGE_CURVE('',#32870,#32883,#27407,.T.) ;
#40231=EDGE_CURVE('',#32872,#32883,#27408,.T.) ;
#40232=EDGE_CURVE('',#32894,#32838,#27409,.T.) ;
#40233=EDGE_CURVE('',#32874,#32882,#27410,.T.) ;
#40234=EDGE_CURVE('',#32894,#32836,#27411,.T.) ;
#40235=EDGE_CURVE('',#32876,#32882,#27412,.T.) ;
#40236=EDGE_CURVE('',#32878,#32834,#27413,.T.) ;
#40237=EDGE_CURVE('',#32828,#32881,#27414,.T.) ;
#40238=EDGE_CURVE('',#32879,#32832,#27415,.T.) ;
#40239=EDGE_CURVE('',#32830,#32880,#27416,.T.) ;
#40240=EDGE_CURVE('',#32849,#32768,#27417,.T.) ;
#40241=EDGE_CURVE('',#32769,#32851,#27418,.T.) ;
#40242=EDGE_CURVE('',#32847,#32768,#27419,.T.) ;
#40243=EDGE_CURVE('',#32769,#32853,#27420,.T.) ;
#40244=EDGE_CURVE('',#32845,#32767,#27421,.T.) ;
#40245=EDGE_CURVE('',#32770,#32855,#27422,.T.) ;
#40246=EDGE_CURVE('',#32843,#32766,#27423,.T.) ;
#40247=EDGE_CURVE('',#32771,#32857,#27424,.T.) ;
#40248=EDGE_CURVE('',#32772,#32859,#27425,.T.) ;
#40249=EDGE_CURVE('',#32773,#32861,#27426,.T.) ;
#40250=EDGE_CURVE('',#32841,#32765,#27427,.T.) ;
#40251=EDGE_CURVE('',#32774,#32863,#27428,.T.) ;
#40252=EDGE_CURVE('',#32840,#32764,#27429,.T.) ;
#40253=EDGE_CURVE('',#32775,#32865,#27430,.T.) ;
#40254=EDGE_CURVE('',#32839,#32763,#27431,.T.) ;
#40255=EDGE_CURVE('',#32776,#32867,#27432,.T.) ;
#40256=EDGE_CURVE('',#32837,#32762,#27433,.T.) ;
#40257=EDGE_CURVE('',#32777,#32869,#27434,.T.) ;
#40258=EDGE_CURVE('',#32835,#32761,#27435,.T.) ;
#40259=EDGE_CURVE('',#32778,#32871,#27436,.T.) ;
#40260=EDGE_CURVE('',#32833,#32761,#27437,.T.) ;
#40261=EDGE_CURVE('',#32779,#32873,#27438,.T.) ;
#40262=EDGE_CURVE('',#32831,#32760,#27439,.T.) ;
#40263=EDGE_CURVE('',#32758,#32875,#27440,.T.) ;
#40264=EDGE_CURVE('',#32829,#32760,#27441,.T.) ;
#40265=EDGE_CURVE('',#32759,#32877,#27442,.T.) ;
#40266=EDGE_CURVE('',#32911,#32912,#10375,.T.) ;
#40267=EDGE_CURVE('',#32912,#32913,#10376,.T.) ;
#40268=EDGE_CURVE('',#32913,#32914,#10377,.T.) ;
#40269=EDGE_CURVE('',#32914,#32911,#10378,.T.) ;
#40270=EDGE_CURVE('',#32915,#32916,#10379,.T.) ;
#40271=EDGE_CURVE('',#32916,#32917,#10380,.T.) ;
#40272=EDGE_CURVE('',#32917,#32918,#10381,.T.) ;
#40273=EDGE_CURVE('',#32918,#32915,#10382,.T.) ;
#40274=EDGE_CURVE('',#32919,#32920,#10383,.T.) ;
#40275=EDGE_CURVE('',#32920,#32921,#10384,.T.) ;
#40276=EDGE_CURVE('',#32921,#32922,#10385,.T.) ;
#40277=EDGE_CURVE('',#32922,#32919,#10386,.T.) ;
#40278=EDGE_CURVE('',#32923,#32924,#10387,.T.) ;
#40279=EDGE_CURVE('',#32924,#32925,#10388,.T.) ;
#40280=EDGE_CURVE('',#32925,#32926,#10389,.T.) ;
#40281=EDGE_CURVE('',#32926,#32923,#10390,.T.) ;
#40282=EDGE_CURVE('',#32927,#32928,#10391,.T.) ;
#40283=EDGE_CURVE('',#32928,#32929,#10392,.T.) ;
#40284=EDGE_CURVE('',#32930,#32929,#10393,.T.) ;
#40285=EDGE_CURVE('',#32930,#32927,#10394,.T.) ;
#40286=EDGE_CURVE('',#32931,#32932,#10395,.T.) ;
#40287=EDGE_CURVE('',#32932,#32425,#27443,.T.) ;
#40288=EDGE_CURVE('',#32906,#32933,#27444,.T.) ;
#40289=EDGE_CURVE('',#32933,#32934,#10396,.T.) ;
#40290=EDGE_CURVE('',#32934,#32931,#10397,.T.) ;
#40291=EDGE_CURVE('',#32935,#32936,#10398,.T.) ;
#40292=EDGE_CURVE('',#32936,#32205,#27445,.T.) ;
#40293=EDGE_CURVE('',#32204,#32937,#27446,.T.) ;
#40294=EDGE_CURVE('',#32937,#32938,#10399,.T.) ;
#40295=EDGE_CURVE('',#32938,#32935,#10400,.T.) ;
#40296=EDGE_CURVE('',#32904,#32912,#27447,.T.) ;
#40297=EDGE_CURVE('',#32911,#32905,#27448,.T.) ;
#40298=EDGE_CURVE('',#32929,#32427,#27449,.T.) ;
#40299=EDGE_CURVE('',#32426,#32930,#27450,.T.) ;
#40300=EDGE_CURVE('',#32939,#32940,#10401,.T.) ;
#40301=EDGE_CURVE('',#32940,#32941,#10402,.T.) ;
#40302=EDGE_CURVE('',#32941,#32942,#10403,.T.) ;
#40303=EDGE_CURVE('',#32942,#32939,#10404,.T.) ;
#40304=EDGE_CURVE('',#32943,#32944,#10405,.T.) ;
#40305=EDGE_CURVE('',#32944,#32898,#10406,.T.) ;
#40306=EDGE_CURVE('',#32897,#32943,#10407,.T.) ;
#40307=EDGE_CURVE('',#32901,#32945,#10408,.T.) ;
#40308=EDGE_CURVE('',#32945,#32946,#10409,.T.) ;
#40309=EDGE_CURVE('',#32946,#32902,#10410,.T.) ;
#40310=EDGE_CURVE('',#32947,#32948,#10411,.T.) ;
#40311=EDGE_CURVE('',#32948,#32949,#10412,.T.) ;
#40312=EDGE_CURVE('',#32949,#32950,#10413,.T.) ;
#40313=EDGE_CURVE('',#32950,#32947,#10414,.T.) ;
#40314=EDGE_CURVE('',#32951,#32952,#10415,.T.) ;
#40315=EDGE_CURVE('',#32952,#32953,#10416,.T.) ;
#40316=EDGE_CURVE('',#32953,#32954,#10417,.T.) ;
#40317=EDGE_CURVE('',#32954,#32951,#10418,.T.) ;
#40318=EDGE_CURVE('',#32955,#32956,#10419,.T.) ;
#40319=EDGE_CURVE('',#32956,#32895,#10420,.T.) ;
#40320=EDGE_CURVE('',#32896,#32955,#10421,.T.) ;
#40321=EDGE_CURVE('',#32899,#32957,#10422,.T.) ;
#40322=EDGE_CURVE('',#32957,#32958,#10423,.T.) ;
#40323=EDGE_CURVE('',#32958,#32900,#10424,.T.) ;
#40324=EDGE_CURVE('',#32959,#32960,#10425,.T.) ;
#40325=EDGE_CURVE('',#32960,#32961,#10426,.T.) ;
#40326=EDGE_CURVE('',#32961,#32962,#10427,.T.) ;
#40327=EDGE_CURVE('',#32962,#32959,#10428,.T.) ;
#40328=EDGE_CURVE('',#32963,#32964,#10429,.T.) ;
#40329=EDGE_CURVE('',#32964,#32965,#10430,.T.) ;
#40330=EDGE_CURVE('',#32965,#32966,#10431,.T.) ;
#40331=EDGE_CURVE('',#32966,#32963,#10432,.T.) ;
#40332=EDGE_CURVE('',#32967,#32968,#10433,.T.) ;
#40333=EDGE_CURVE('',#32968,#32969,#10434,.T.) ;
#40334=EDGE_CURVE('',#32969,#32970,#10435,.T.) ;
#40335=EDGE_CURVE('',#32970,#32967,#10436,.T.) ;
#40336=EDGE_CURVE('',#32971,#32972,#10437,.T.) ;
#40337=EDGE_CURVE('',#32972,#32973,#10438,.T.) ;
#40338=EDGE_CURVE('',#32973,#32974,#10439,.T.) ;
#40339=EDGE_CURVE('',#32974,#32971,#10440,.T.) ;
#40340=EDGE_CURVE('',#32961,#32923,#27451,.T.) ;
#40341=EDGE_CURVE('',#32962,#32926,#27452,.T.) ;
#40342=EDGE_CURVE('',#32923,#32928,#27453,.T.) ;
#40343=EDGE_CURVE('',#32927,#32924,#27454,.T.) ;
#40344=EDGE_CURVE('',#32962,#32919,#27455,.T.) ;
#40345=EDGE_CURVE('',#32919,#32926,#27456,.T.) ;
#40346=EDGE_CURVE('',#32924,#32964,#27457,.T.) ;
#40347=EDGE_CURVE('',#32925,#32963,#27458,.T.) ;
#40348=EDGE_CURVE('',#32920,#32925,#27459,.T.) ;
#40349=EDGE_CURVE('',#32959,#32922,#27460,.T.) ;
#40350=EDGE_CURVE('',#32920,#32963,#27461,.T.) ;
#40351=EDGE_CURVE('',#32959,#32915,#27462,.T.) ;
#40352=EDGE_CURVE('',#32915,#32922,#27463,.T.) ;
#40353=EDGE_CURVE('',#32921,#32966,#27464,.T.) ;
#40354=EDGE_CURVE('',#32916,#32921,#27465,.T.) ;
#40355=EDGE_CURVE('',#32918,#32960,#27466,.T.) ;
#40356=EDGE_CURVE('',#32916,#32966,#27467,.T.) ;
#40357=EDGE_CURVE('',#32913,#32918,#27468,.T.) ;
#40358=EDGE_CURVE('',#32917,#32914,#27469,.T.) ;
#40359=EDGE_CURVE('',#32965,#32917,#27470,.T.) ;
#40360=EDGE_CURVE('',#32969,#32939,#27471,.T.) ;
#40361=EDGE_CURVE('',#32970,#32942,#27472,.T.) ;
#40362=EDGE_CURVE('',#32939,#32944,#27473,.T.) ;
#40363=EDGE_CURVE('',#32943,#32940,#27474,.T.) ;
#40364=EDGE_CURVE('',#32970,#32953,#27475,.T.) ;
#40365=EDGE_CURVE('',#32953,#32942,#27476,.T.) ;
#40366=EDGE_CURVE('',#32940,#32972,#27477,.T.) ;
#40367=EDGE_CURVE('',#32941,#32971,#27478,.T.) ;
#40368=EDGE_CURVE('',#32954,#32941,#27479,.T.) ;
#40369=EDGE_CURVE('',#32967,#32952,#27480,.T.) ;
#40370=EDGE_CURVE('',#32954,#32971,#27481,.T.) ;
#40371=EDGE_CURVE('',#32967,#32947,#27482,.T.) ;
#40372=EDGE_CURVE('',#32947,#32952,#27483,.T.) ;
#40373=EDGE_CURVE('',#32951,#32974,#27484,.T.) ;
#40374=EDGE_CURVE('',#32948,#32951,#27485,.T.) ;
#40375=EDGE_CURVE('',#32950,#32968,#27486,.T.) ;
#40376=EDGE_CURVE('',#32948,#32974,#27487,.T.) ;
#40377=EDGE_CURVE('',#32945,#32950,#27488,.T.) ;
#40378=EDGE_CURVE('',#32949,#32946,#27489,.T.) ;
#40379=EDGE_CURVE('',#32973,#32949,#27490,.T.) ;
#40380=EDGE_CURVE('',#32937,#32929,#27491,.T.) ;
#40381=EDGE_CURVE('',#32938,#32928,#27492,.T.) ;
#40382=EDGE_CURVE('',#32938,#32961,#27493,.T.) ;
#40383=EDGE_CURVE('',#32935,#32960,#27494,.T.) ;
#40384=EDGE_CURVE('',#32935,#32913,#27495,.T.) ;
#40385=EDGE_CURVE('',#32936,#32912,#27496,.T.) ;
#40386=EDGE_CURVE('',#32933,#32911,#27497,.T.) ;
#40387=EDGE_CURVE('',#32934,#32914,#27498,.T.) ;
#40388=EDGE_CURVE('',#32934,#32965,#27499,.T.) ;
#40389=EDGE_CURVE('',#32931,#32964,#27500,.T.) ;
#40390=EDGE_CURVE('',#32931,#32927,#27501,.T.) ;
#40391=EDGE_CURVE('',#32932,#32930,#27502,.T.) ;
#40392=EDGE_CURVE('',#32957,#32944,#27503,.T.) ;
#40393=EDGE_CURVE('',#32957,#32969,#27504,.T.) ;
#40394=EDGE_CURVE('',#32958,#32968,#27505,.T.) ;
#40395=EDGE_CURVE('',#32958,#32945,#27506,.T.) ;
#40396=EDGE_CURVE('',#32943,#32956,#27507,.T.) ;
#40397=EDGE_CURVE('',#32972,#32956,#27508,.T.) ;
#40398=EDGE_CURVE('',#32973,#32955,#27509,.T.) ;
#40399=EDGE_CURVE('',#32955,#32946,#27510,.T.) ;
#40400=EDGE_CURVE('',#32975,#32976,#10441,.T.) ;
#40401=EDGE_CURVE('',#32976,#32977,#10442,.T.) ;
#40402=EDGE_CURVE('',#32977,#32978,#10443,.T.) ;
#40403=EDGE_CURVE('',#32978,#32979,#10444,.T.) ;
#40404=EDGE_CURVE('',#32979,#32980,#10445,.T.) ;
#40405=EDGE_CURVE('',#32980,#32981,#10446,.T.) ;
#40406=EDGE_CURVE('',#32982,#32981,#27511,.T.) ;
#40407=EDGE_CURVE('',#32982,#32983,#10447,.T.) ;
#40408=EDGE_CURVE('',#32984,#32983,#27512,.T.) ;
#40409=EDGE_CURVE('',#32984,#32975,#10448,.T.) ;
#40410=EDGE_CURVE('',#32985,#32986,#10449,.T.) ;
#40411=EDGE_CURVE('',#32986,#32987,#10450,.T.) ;
#40412=EDGE_CURVE('',#32987,#32988,#10451,.T.) ;
#40413=EDGE_CURVE('',#32988,#32989,#10452,.T.) ;
#40414=EDGE_CURVE('',#32989,#32990,#10453,.T.) ;
#40415=EDGE_CURVE('',#32990,#32991,#10454,.T.) ;
#40416=EDGE_CURVE('',#32992,#32991,#27513,.T.) ;
#40417=EDGE_CURVE('',#32992,#32993,#10455,.T.) ;
#40418=EDGE_CURVE('',#32994,#32993,#27514,.T.) ;
#40419=EDGE_CURVE('',#32994,#32985,#10456,.T.) ;
#40420=EDGE_CURVE('',#32995,#32996,#10457,.T.) ;
#40421=EDGE_CURVE('',#32996,#32997,#10458,.T.) ;
#40422=EDGE_CURVE('',#32997,#32998,#10459,.T.) ;
#40423=EDGE_CURVE('',#32998,#32999,#10460,.T.) ;
#40424=EDGE_CURVE('',#32999,#33000,#10461,.T.) ;
#40425=EDGE_CURVE('',#33000,#33001,#10462,.T.) ;
#40426=EDGE_CURVE('',#33002,#33001,#27515,.T.) ;
#40427=EDGE_CURVE('',#33002,#33003,#10463,.T.) ;
#40428=EDGE_CURVE('',#33004,#33003,#27516,.T.) ;
#40429=EDGE_CURVE('',#33004,#32995,#10464,.T.) ;
#40430=EDGE_CURVE('',#33005,#33006,#10465,.T.) ;
#40431=EDGE_CURVE('',#33006,#33007,#10466,.T.) ;
#40432=EDGE_CURVE('',#33007,#33008,#10467,.T.) ;
#40433=EDGE_CURVE('',#33008,#33009,#10468,.T.) ;
#40434=EDGE_CURVE('',#33009,#33010,#10469,.T.) ;
#40435=EDGE_CURVE('',#33010,#33011,#10470,.T.) ;
#40436=EDGE_CURVE('',#33012,#33011,#27517,.T.) ;
#40437=EDGE_CURVE('',#33012,#33013,#10471,.T.) ;
#40438=EDGE_CURVE('',#33014,#33013,#27518,.T.) ;
#40439=EDGE_CURVE('',#33014,#33005,#10472,.T.) ;
#40440=EDGE_CURVE('',#33015,#33016,#10473,.T.) ;
#40441=EDGE_CURVE('',#33016,#33017,#10474,.T.) ;
#40442=EDGE_CURVE('',#33017,#33018,#10475,.T.) ;
#40443=EDGE_CURVE('',#33018,#33019,#10476,.T.) ;
#40444=EDGE_CURVE('',#33019,#33020,#10477,.T.) ;
#40445=EDGE_CURVE('',#33020,#33021,#10478,.T.) ;
#40446=EDGE_CURVE('',#33022,#33021,#27519,.T.) ;
#40447=EDGE_CURVE('',#33022,#33023,#10479,.T.) ;
#40448=EDGE_CURVE('',#33024,#33023,#27520,.T.) ;
#40449=EDGE_CURVE('',#33024,#33015,#10480,.T.) ;
#40450=EDGE_CURVE('',#33025,#33026,#10481,.T.) ;
#40451=EDGE_CURVE('',#33026,#33027,#10482,.T.) ;
#40452=EDGE_CURVE('',#33027,#33028,#10483,.T.) ;
#40453=EDGE_CURVE('',#33028,#33029,#10484,.T.) ;
#40454=EDGE_CURVE('',#33029,#33030,#10485,.T.) ;
#40455=EDGE_CURVE('',#33030,#33031,#10486,.T.) ;
#40456=EDGE_CURVE('',#33032,#33031,#27521,.T.) ;
#40457=EDGE_CURVE('',#33032,#33033,#10487,.T.) ;
#40458=EDGE_CURVE('',#33034,#33033,#27522,.T.) ;
#40459=EDGE_CURVE('',#33034,#33025,#10488,.T.) ;
#40460=EDGE_CURVE('',#33035,#33036,#10489,.T.) ;
#40461=EDGE_CURVE('',#33036,#33037,#10490,.T.) ;
#40462=EDGE_CURVE('',#33037,#33038,#10491,.T.) ;
#40463=EDGE_CURVE('',#33038,#33039,#10492,.T.) ;
#40464=EDGE_CURVE('',#33039,#33040,#10493,.T.) ;
#40465=EDGE_CURVE('',#33040,#33041,#10494,.T.) ;
#40466=EDGE_CURVE('',#33042,#33041,#27523,.T.) ;
#40467=EDGE_CURVE('',#33042,#33043,#10495,.T.) ;
#40468=EDGE_CURVE('',#33044,#33043,#27524,.T.) ;
#40469=EDGE_CURVE('',#33044,#33035,#10496,.T.) ;
#40470=EDGE_CURVE('',#33045,#33046,#10497,.T.) ;
#40471=EDGE_CURVE('',#33046,#33047,#10498,.T.) ;
#40472=EDGE_CURVE('',#33047,#33048,#10499,.T.) ;
#40473=EDGE_CURVE('',#33048,#33049,#10500,.T.) ;
#40474=EDGE_CURVE('',#33049,#33050,#10501,.T.) ;
#40475=EDGE_CURVE('',#33050,#33051,#10502,.T.) ;
#40476=EDGE_CURVE('',#33052,#33051,#27525,.T.) ;
#40477=EDGE_CURVE('',#33052,#33053,#10503,.T.) ;
#40478=EDGE_CURVE('',#33054,#33053,#27526,.T.) ;
#40479=EDGE_CURVE('',#33054,#33045,#10504,.T.) ;
#40480=EDGE_CURVE('',#33055,#33056,#10505,.T.) ;
#40481=EDGE_CURVE('',#33056,#33057,#10506,.T.) ;
#40482=EDGE_CURVE('',#33057,#33058,#10507,.T.) ;
#40483=EDGE_CURVE('',#33058,#33059,#10508,.T.) ;
#40484=EDGE_CURVE('',#33059,#33060,#10509,.T.) ;
#40485=EDGE_CURVE('',#33060,#33061,#10510,.T.) ;
#40486=EDGE_CURVE('',#33062,#33061,#27527,.T.) ;
#40487=EDGE_CURVE('',#33062,#33063,#10511,.T.) ;
#40488=EDGE_CURVE('',#33064,#33063,#27528,.T.) ;
#40489=EDGE_CURVE('',#33064,#33055,#10512,.T.) ;
#40490=EDGE_CURVE('',#33065,#33066,#10513,.T.) ;
#40491=EDGE_CURVE('',#33066,#33067,#10514,.T.) ;
#40492=EDGE_CURVE('',#33067,#33068,#10515,.T.) ;
#40493=EDGE_CURVE('',#33068,#33065,#10516,.T.) ;
#40494=EDGE_CURVE('',#32164,#33069,#10517,.T.) ;
#40495=EDGE_CURVE('',#33069,#33070,#10518,.T.) ;
#40496=EDGE_CURVE('',#33070,#32165,#10519,.T.) ;
#40497=EDGE_CURVE('',#33071,#33072,#10520,.T.) ;
#40498=EDGE_CURVE('',#33072,#33073,#10521,.T.) ;
#40499=EDGE_CURVE('',#33073,#33074,#10522,.T.) ;
#40500=EDGE_CURVE('',#33074,#33071,#10523,.T.) ;
#40501=EDGE_CURVE('',#33075,#33076,#10524,.T.) ;
#40502=EDGE_CURVE('',#33076,#33077,#10525,.T.) ;
#40503=EDGE_CURVE('',#33077,#33078,#10526,.T.) ;
#40504=EDGE_CURVE('',#33078,#33075,#10527,.T.) ;
#40505=EDGE_CURVE('',#33079,#33080,#10528,.T.) ;
#40506=EDGE_CURVE('',#33080,#33081,#10529,.T.) ;
#40507=EDGE_CURVE('',#33081,#33082,#10530,.T.) ;
#40508=EDGE_CURVE('',#33082,#33079,#10531,.T.) ;
#40509=EDGE_CURVE('',#33083,#33084,#10532,.T.) ;
#40510=EDGE_CURVE('',#33084,#33085,#10533,.T.) ;
#40511=EDGE_CURVE('',#33085,#33086,#10534,.T.) ;
#40512=EDGE_CURVE('',#33086,#33083,#10535,.T.) ;
#40513=EDGE_CURVE('',#32113,#33087,#10536,.T.) ;
#40514=EDGE_CURVE('',#33087,#33088,#10537,.T.) ;
#40515=EDGE_CURVE('',#33088,#32114,#10538,.T.) ;
#40516=EDGE_CURVE('',#33089,#33090,#10539,.T.) ;
#40517=EDGE_CURVE('',#33090,#33091,#10540,.T.) ;
#40518=EDGE_CURVE('',#33091,#33092,#10541,.T.) ;
#40519=EDGE_CURVE('',#33092,#33089,#10542,.T.) ;
#40520=EDGE_CURVE('',#33093,#33094,#10543,.T.) ;
#40521=EDGE_CURVE('',#33094,#33095,#10544,.T.) ;
#40522=EDGE_CURVE('',#33095,#33096,#10545,.T.) ;
#40523=EDGE_CURVE('',#33096,#33093,#10546,.T.) ;
#40524=EDGE_CURVE('',#33097,#33098,#10547,.T.) ;
#40525=EDGE_CURVE('',#33098,#33099,#10548,.T.) ;
#40526=EDGE_CURVE('',#33099,#33100,#10549,.T.) ;
#40527=EDGE_CURVE('',#33100,#33097,#10550,.T.) ;
#40528=EDGE_CURVE('',#33101,#33102,#10551,.T.) ;
#40529=EDGE_CURVE('',#33102,#33103,#10552,.T.) ;
#40530=EDGE_CURVE('',#33103,#33104,#10553,.T.) ;
#40531=EDGE_CURVE('',#33104,#33101,#10554,.T.) ;
#40532=EDGE_CURVE('',#32098,#33105,#10555,.T.) ;
#40533=EDGE_CURVE('',#33105,#33106,#10556,.T.) ;
#40534=EDGE_CURVE('',#33106,#32099,#10557,.T.) ;
#40535=EDGE_CURVE('',#33107,#33108,#10558,.T.) ;
#40536=EDGE_CURVE('',#33108,#33109,#10559,.T.) ;
#40537=EDGE_CURVE('',#33109,#33110,#10560,.T.) ;
#40538=EDGE_CURVE('',#33110,#33107,#10561,.T.) ;
#40539=EDGE_CURVE('',#33111,#33112,#10562,.T.) ;
#40540=EDGE_CURVE('',#33112,#33113,#10563,.T.) ;
#40541=EDGE_CURVE('',#33113,#33114,#10564,.T.) ;
#40542=EDGE_CURVE('',#33114,#33111,#10565,.T.) ;
#40543=EDGE_CURVE('',#33115,#33116,#10566,.T.) ;
#40544=EDGE_CURVE('',#33116,#33117,#10567,.T.) ;
#40545=EDGE_CURVE('',#33117,#33118,#10568,.T.) ;
#40546=EDGE_CURVE('',#33118,#33115,#10569,.T.) ;
#40547=EDGE_CURVE('',#33119,#33120,#10570,.T.) ;
#40548=EDGE_CURVE('',#33120,#33121,#10571,.T.) ;
#40549=EDGE_CURVE('',#33121,#33122,#10572,.T.) ;
#40550=EDGE_CURVE('',#33122,#33119,#10573,.T.) ;
#40551=EDGE_CURVE('',#32083,#33123,#10574,.T.) ;
#40552=EDGE_CURVE('',#33123,#33124,#10575,.T.) ;
#40553=EDGE_CURVE('',#33124,#32084,#10576,.T.) ;
#40554=EDGE_CURVE('',#33125,#33126,#10577,.T.) ;
#40555=EDGE_CURVE('',#33126,#33127,#10578,.T.) ;
#40556=EDGE_CURVE('',#33127,#33128,#10579,.T.) ;
#40557=EDGE_CURVE('',#33128,#33125,#10580,.T.) ;
#40558=EDGE_CURVE('',#33129,#33130,#10581,.T.) ;
#40559=EDGE_CURVE('',#33130,#33131,#10582,.T.) ;
#40560=EDGE_CURVE('',#33131,#33132,#10583,.T.) ;
#40561=EDGE_CURVE('',#33132,#33129,#10584,.T.) ;
#40562=EDGE_CURVE('',#33133,#33134,#10585,.T.) ;
#40563=EDGE_CURVE('',#33134,#33135,#10586,.T.) ;
#40564=EDGE_CURVE('',#33135,#33136,#10587,.T.) ;
#40565=EDGE_CURVE('',#33136,#33133,#10588,.T.) ;
#40566=EDGE_CURVE('',#33137,#33138,#10589,.T.) ;
#40567=EDGE_CURVE('',#33138,#33139,#10590,.T.) ;
#40568=EDGE_CURVE('',#33139,#33140,#10591,.T.) ;
#40569=EDGE_CURVE('',#33140,#33137,#10592,.T.) ;
#40570=EDGE_CURVE('',#32068,#33141,#10593,.T.) ;
#40571=EDGE_CURVE('',#33141,#33142,#10594,.T.) ;
#40572=EDGE_CURVE('',#33142,#32069,#10595,.T.) ;
#40573=EDGE_CURVE('',#33143,#33144,#10596,.T.) ;
#40574=EDGE_CURVE('',#33144,#33145,#10597,.T.) ;
#40575=EDGE_CURVE('',#33145,#33146,#10598,.T.) ;
#40576=EDGE_CURVE('',#33146,#33143,#10599,.T.) ;
#40577=EDGE_CURVE('',#33147,#33148,#10600,.T.) ;
#40578=EDGE_CURVE('',#33148,#33149,#10601,.T.) ;
#40579=EDGE_CURVE('',#33149,#33150,#10602,.T.) ;
#40580=EDGE_CURVE('',#33150,#33147,#10603,.T.) ;
#40581=EDGE_CURVE('',#33151,#33152,#10604,.T.) ;
#40582=EDGE_CURVE('',#33152,#33153,#10605,.T.) ;
#40583=EDGE_CURVE('',#33153,#33154,#10606,.T.) ;
#40584=EDGE_CURVE('',#33154,#33151,#10607,.T.) ;
#40585=EDGE_CURVE('',#33155,#33156,#10608,.T.) ;
#40586=EDGE_CURVE('',#33156,#33157,#10609,.T.) ;
#40587=EDGE_CURVE('',#33157,#33158,#10610,.T.) ;
#40588=EDGE_CURVE('',#33158,#33155,#10611,.T.) ;
#40589=EDGE_CURVE('',#32053,#33159,#10612,.T.) ;
#40590=EDGE_CURVE('',#33159,#33160,#10613,.T.) ;
#40591=EDGE_CURVE('',#33160,#32054,#10614,.T.) ;
#40592=EDGE_CURVE('',#33161,#33162,#10615,.T.) ;
#40593=EDGE_CURVE('',#33162,#33163,#10616,.T.) ;
#40594=EDGE_CURVE('',#33163,#33164,#10617,.T.) ;
#40595=EDGE_CURVE('',#33164,#33161,#10618,.T.) ;
#40596=EDGE_CURVE('',#33165,#33166,#10619,.T.) ;
#40597=EDGE_CURVE('',#33166,#33167,#10620,.T.) ;
#40598=EDGE_CURVE('',#33167,#33168,#10621,.T.) ;
#40599=EDGE_CURVE('',#33168,#33165,#10622,.T.) ;
#40600=EDGE_CURVE('',#33169,#33170,#10623,.T.) ;
#40601=EDGE_CURVE('',#33170,#33171,#10624,.T.) ;
#40602=EDGE_CURVE('',#33171,#33172,#10625,.T.) ;
#40603=EDGE_CURVE('',#33172,#33169,#10626,.T.) ;
#40604=EDGE_CURVE('',#33173,#33174,#10627,.T.) ;
#40605=EDGE_CURVE('',#33174,#33175,#10628,.T.) ;
#40606=EDGE_CURVE('',#33175,#33176,#10629,.T.) ;
#40607=EDGE_CURVE('',#33176,#33173,#10630,.T.) ;
#40608=EDGE_CURVE('',#32038,#33177,#10631,.T.) ;
#40609=EDGE_CURVE('',#33177,#33178,#10632,.T.) ;
#40610=EDGE_CURVE('',#33178,#32039,#10633,.T.) ;
#40611=EDGE_CURVE('',#33179,#33180,#10634,.T.) ;
#40612=EDGE_CURVE('',#33180,#33181,#10635,.T.) ;
#40613=EDGE_CURVE('',#33181,#33182,#10636,.T.) ;
#40614=EDGE_CURVE('',#33182,#33179,#10637,.T.) ;
#40615=EDGE_CURVE('',#33183,#33184,#10638,.T.) ;
#40616=EDGE_CURVE('',#33184,#33185,#10639,.T.) ;
#40617=EDGE_CURVE('',#33185,#33186,#10640,.T.) ;
#40618=EDGE_CURVE('',#33186,#33183,#10641,.T.) ;
#40619=EDGE_CURVE('',#33187,#33188,#10642,.T.) ;
#40620=EDGE_CURVE('',#33188,#33189,#10643,.T.) ;
#40621=EDGE_CURVE('',#33189,#33190,#10644,.T.) ;
#40622=EDGE_CURVE('',#33190,#33187,#10645,.T.) ;
#40623=EDGE_CURVE('',#33191,#33192,#10646,.T.) ;
#40624=EDGE_CURVE('',#33192,#33193,#10647,.T.) ;
#40625=EDGE_CURVE('',#33193,#33194,#10648,.T.) ;
#40626=EDGE_CURVE('',#33194,#33191,#10649,.T.) ;
#40627=EDGE_CURVE('',#32023,#33195,#10650,.T.) ;
#40628=EDGE_CURVE('',#33195,#33196,#10651,.T.) ;
#40629=EDGE_CURVE('',#33196,#32024,#10652,.T.) ;
#40630=EDGE_CURVE('',#33197,#33198,#10653,.T.) ;
#40631=EDGE_CURVE('',#33198,#33199,#10654,.T.) ;
#40632=EDGE_CURVE('',#33199,#33200,#10655,.T.) ;
#40633=EDGE_CURVE('',#33200,#33197,#10656,.T.) ;
#40634=EDGE_CURVE('',#33201,#33202,#10657,.T.) ;
#40635=EDGE_CURVE('',#33202,#33203,#10658,.T.) ;
#40636=EDGE_CURVE('',#33203,#33204,#10659,.T.) ;
#40637=EDGE_CURVE('',#33204,#33201,#10660,.T.) ;
#40638=EDGE_CURVE('',#33205,#33206,#10661,.T.) ;
#40639=EDGE_CURVE('',#33206,#33207,#10662,.T.) ;
#40640=EDGE_CURVE('',#33207,#33208,#10663,.T.) ;
#40641=EDGE_CURVE('',#33208,#33205,#10664,.T.) ;
#40642=EDGE_CURVE('',#33209,#33210,#10665,.T.) ;
#40643=EDGE_CURVE('',#33210,#33211,#10666,.T.) ;
#40644=EDGE_CURVE('',#33211,#33212,#10667,.T.) ;
#40645=EDGE_CURVE('',#33212,#33209,#10668,.T.) ;
#40646=EDGE_CURVE('',#32008,#33213,#10669,.T.) ;
#40647=EDGE_CURVE('',#33213,#33214,#10670,.T.) ;
#40648=EDGE_CURVE('',#33214,#32009,#10671,.T.) ;
#40649=EDGE_CURVE('',#33215,#33216,#10672,.T.) ;
#40650=EDGE_CURVE('',#33216,#33217,#10673,.T.) ;
#40651=EDGE_CURVE('',#33217,#33218,#10674,.T.) ;
#40652=EDGE_CURVE('',#33218,#33215,#10675,.T.) ;
#40653=EDGE_CURVE('',#33219,#33220,#10676,.T.) ;
#40654=EDGE_CURVE('',#33220,#33221,#10677,.T.) ;
#40655=EDGE_CURVE('',#33221,#33222,#10678,.T.) ;
#40656=EDGE_CURVE('',#33222,#33219,#10679,.T.) ;
#40657=EDGE_CURVE('',#33223,#33224,#10680,.T.) ;
#40658=EDGE_CURVE('',#33224,#33225,#10681,.T.) ;
#40659=EDGE_CURVE('',#33225,#33226,#10682,.T.) ;
#40660=EDGE_CURVE('',#33226,#33223,#10683,.T.) ;
#40661=EDGE_CURVE('',#33227,#33228,#10684,.T.) ;
#40662=EDGE_CURVE('',#33227,#33229,#27529,.T.) ;
#40663=EDGE_CURVE('',#33229,#33230,#10685,.T.) ;
#40664=EDGE_CURVE('',#33230,#33228,#27530,.T.) ;
#40665=EDGE_CURVE('',#33229,#33231,#10686,.T.) ;
#40666=EDGE_CURVE('',#33231,#33232,#10687,.T.) ;
#40667=EDGE_CURVE('',#33232,#33230,#10688,.T.) ;
#40668=EDGE_CURVE('',#33231,#33233,#27531,.T.) ;
#40669=EDGE_CURVE('',#33233,#33234,#10689,.T.) ;
#40670=EDGE_CURVE('',#33234,#33232,#27532,.T.) ;
#40671=EDGE_CURVE('',#33233,#33235,#10690,.T.) ;
#40672=EDGE_CURVE('',#33235,#33236,#10691,.T.) ;
#40673=EDGE_CURVE('',#33236,#33234,#10692,.T.) ;
#40674=EDGE_CURVE('',#33235,#33237,#27533,.T.) ;
#40675=EDGE_CURVE('',#33237,#33238,#10693,.T.) ;
#40676=EDGE_CURVE('',#33238,#33236,#27534,.T.) ;
#40677=EDGE_CURVE('',#33237,#32003,#10694,.T.) ;
#40678=EDGE_CURVE('',#32003,#33239,#10695,.T.) ;
#40679=EDGE_CURVE('',#33239,#33238,#10696,.T.) ;
#40680=EDGE_CURVE('',#32004,#33240,#10697,.T.) ;
#40681=EDGE_CURVE('',#33240,#33239,#27535,.T.) ;
#40682=EDGE_CURVE('',#32004,#32185,#10698,.T.) ;
#40683=EDGE_CURVE('',#32155,#33240,#10699,.T.) ;
#40684=EDGE_CURVE('',#32186,#33241,#10700,.T.) ;
#40685=EDGE_CURVE('',#33241,#33242,#10701,.T.) ;
#40686=EDGE_CURVE('',#33242,#32156,#10702,.T.) ;
#40687=EDGE_CURVE('',#33241,#33243,#27536,.T.) ;
#40688=EDGE_CURVE('',#33243,#33244,#10703,.T.) ;
#40689=EDGE_CURVE('',#33244,#33242,#27537,.T.) ;
#40690=EDGE_CURVE('',#33243,#33245,#10704,.T.) ;
#40691=EDGE_CURVE('',#33245,#33246,#10705,.T.) ;
#40692=EDGE_CURVE('',#33246,#33244,#10706,.T.) ;
#40693=EDGE_CURVE('',#33245,#33247,#27538,.T.) ;
#40694=EDGE_CURVE('',#33247,#33248,#10707,.T.) ;
#40695=EDGE_CURVE('',#33248,#33246,#27539,.T.) ;
#40696=EDGE_CURVE('',#33247,#33249,#10708,.T.) ;
#40697=EDGE_CURVE('',#33249,#33250,#10709,.T.) ;
#40698=EDGE_CURVE('',#33250,#33248,#10710,.T.) ;
#40699=EDGE_CURVE('',#33249,#33251,#27540,.T.) ;
#40700=EDGE_CURVE('',#33251,#33252,#10711,.T.) ;
#40701=EDGE_CURVE('',#33252,#33250,#27541,.T.) ;
#40702=EDGE_CURVE('',#33251,#33253,#10712,.T.) ;
#40703=EDGE_CURVE('',#33253,#33254,#10713,.T.) ;
#40704=EDGE_CURVE('',#33254,#33252,#10714,.T.) ;
#40705=EDGE_CURVE('',#33253,#33255,#27542,.T.) ;
#40706=EDGE_CURVE('',#33255,#33256,#10715,.T.) ;
#40707=EDGE_CURVE('',#33256,#33254,#27543,.T.) ;
#40708=EDGE_CURVE('',#33255,#33257,#10716,.T.) ;
#40709=EDGE_CURVE('',#33257,#33258,#10717,.T.) ;
#40710=EDGE_CURVE('',#33258,#33256,#10718,.T.) ;
#40711=EDGE_CURVE('',#33257,#33259,#27544,.T.) ;
#40712=EDGE_CURVE('',#33259,#33260,#10719,.T.) ;
#40713=EDGE_CURVE('',#33260,#33258,#27545,.T.) ;
#40714=EDGE_CURVE('',#33259,#33261,#10720,.T.) ;
#40715=EDGE_CURVE('',#33261,#33262,#10721,.T.) ;
#40716=EDGE_CURVE('',#33262,#33260,#10722,.T.) ;
#40717=EDGE_CURVE('',#33261,#33263,#27546,.T.) ;
#40718=EDGE_CURVE('',#33263,#33264,#10723,.T.) ;
#40719=EDGE_CURVE('',#33264,#33262,#27547,.T.) ;
#40720=EDGE_CURVE('',#33263,#33265,#27548,.T.) ;
#40721=EDGE_CURVE('',#33265,#33266,#10724,.T.) ;
#40722=EDGE_CURVE('',#33266,#33264,#27549,.T.) ;
#40723=EDGE_CURVE('',#33265,#33267,#27550,.T.) ;
#40724=EDGE_CURVE('',#33267,#33268,#10725,.T.) ;
#40725=EDGE_CURVE('',#33268,#33266,#27551,.T.) ;
#40726=EDGE_CURVE('',#33267,#33269,#10726,.T.) ;
#40727=EDGE_CURVE('',#33269,#33270,#10727,.T.) ;
#40728=EDGE_CURVE('',#33270,#33268,#10728,.T.) ;
#40729=EDGE_CURVE('',#33269,#33271,#27552,.T.) ;
#40730=EDGE_CURVE('',#33271,#33272,#10729,.T.) ;
#40731=EDGE_CURVE('',#33272,#33270,#27553,.T.) ;
#40732=EDGE_CURVE('',#33271,#33273,#10730,.T.) ;
#40733=EDGE_CURVE('',#33273,#33274,#10731,.T.) ;
#40734=EDGE_CURVE('',#33274,#33272,#10732,.T.) ;
#40735=EDGE_CURVE('',#33273,#33275,#27554,.T.) ;
#40736=EDGE_CURVE('',#33275,#33276,#10733,.T.) ;
#40737=EDGE_CURVE('',#33276,#33274,#27555,.T.) ;
#40738=EDGE_CURVE('',#33275,#33227,#10734,.T.) ;
#40739=EDGE_CURVE('',#33228,#33276,#10735,.T.) ;
#40740=EDGE_CURVE('',#33277,#33278,#27556,.T.) ;
#40741=EDGE_CURVE('',#33278,#33279,#10736,.T.) ;
#40742=EDGE_CURVE('',#33279,#33280,#27557,.T.) ;
#40743=EDGE_CURVE('',#33280,#33281,#10737,.T.) ;
#40744=EDGE_CURVE('',#33281,#33282,#10738,.T.) ;
#40745=EDGE_CURVE('',#33282,#33283,#10739,.T.) ;
#40746=EDGE_CURVE('',#33283,#33284,#27558,.T.) ;
#40747=EDGE_CURVE('',#33284,#33285,#10740,.T.) ;
#40748=EDGE_CURVE('',#33285,#33286,#10741,.T.) ;
#40749=EDGE_CURVE('',#33286,#33287,#10742,.T.) ;
#40750=EDGE_CURVE('',#33287,#33288,#27559,.T.) ;
#40751=EDGE_CURVE('',#33288,#33289,#10743,.T.) ;
#40752=EDGE_CURVE('',#33289,#33290,#27560,.T.) ;
#40753=EDGE_CURVE('',#33290,#33291,#10744,.T.) ;
#40754=EDGE_CURVE('',#33291,#33292,#10745,.T.) ;
#40755=EDGE_CURVE('',#33292,#32005,#10746,.T.) ;
#40756=EDGE_CURVE('',#32005,#33293,#10747,.T.) ;
#40757=EDGE_CURVE('',#33293,#33277,#10748,.T.) ;
#40758=EDGE_CURVE('',#33294,#33295,#10749,.T.) ;
#40759=EDGE_CURVE('',#33294,#33296,#27561,.T.) ;
#40760=EDGE_CURVE('',#33296,#33297,#10750,.T.) ;
#40761=EDGE_CURVE('',#33297,#33295,#27562,.T.) ;
#40762=EDGE_CURVE('',#33296,#33298,#10751,.T.) ;
#40763=EDGE_CURVE('',#33298,#33299,#10752,.T.) ;
#40764=EDGE_CURVE('',#33299,#33297,#10753,.T.) ;
#40765=EDGE_CURVE('',#33298,#33300,#27563,.T.) ;
#40766=EDGE_CURVE('',#33300,#33301,#10754,.T.) ;
#40767=EDGE_CURVE('',#33301,#33299,#27564,.T.) ;
#40768=EDGE_CURVE('',#33300,#33302,#10755,.T.) ;
#40769=EDGE_CURVE('',#33302,#33303,#10756,.T.) ;
#40770=EDGE_CURVE('',#33303,#33301,#10757,.T.) ;
#40771=EDGE_CURVE('',#33302,#33304,#27565,.T.) ;
#40772=EDGE_CURVE('',#33304,#33305,#10758,.T.) ;
#40773=EDGE_CURVE('',#33305,#33303,#27566,.T.) ;
#40774=EDGE_CURVE('',#33304,#32018,#10759,.T.) ;
#40775=EDGE_CURVE('',#32018,#33306,#10760,.T.) ;
#40776=EDGE_CURVE('',#33306,#33305,#10761,.T.) ;
#40777=EDGE_CURVE('',#32019,#33307,#10762,.T.) ;
#40778=EDGE_CURVE('',#33307,#33306,#27567,.T.) ;
#40779=EDGE_CURVE('',#32019,#32183,#10763,.T.) ;
#40780=EDGE_CURVE('',#32151,#33307,#10764,.T.) ;
#40781=EDGE_CURVE('',#32184,#33308,#10765,.T.) ;
#40782=EDGE_CURVE('',#33308,#33309,#10766,.T.) ;
#40783=EDGE_CURVE('',#33309,#32152,#10767,.T.) ;
#40784=EDGE_CURVE('',#33308,#33310,#27568,.T.) ;
#40785=EDGE_CURVE('',#33310,#33311,#10768,.T.) ;
#40786=EDGE_CURVE('',#33311,#33309,#27569,.T.) ;
#40787=EDGE_CURVE('',#33310,#33312,#10769,.T.) ;
#40788=EDGE_CURVE('',#33312,#33313,#10770,.T.) ;
#40789=EDGE_CURVE('',#33313,#33311,#10771,.T.) ;
#40790=EDGE_CURVE('',#33312,#33314,#27570,.T.) ;
#40791=EDGE_CURVE('',#33314,#33315,#10772,.T.) ;
#40792=EDGE_CURVE('',#33315,#33313,#27571,.T.) ;
#40793=EDGE_CURVE('',#33314,#33316,#10773,.T.) ;
#40794=EDGE_CURVE('',#33316,#33317,#10774,.T.) ;
#40795=EDGE_CURVE('',#33317,#33315,#10775,.T.) ;
#40796=EDGE_CURVE('',#33316,#33318,#27572,.T.) ;
#40797=EDGE_CURVE('',#33318,#33319,#10776,.T.) ;
#40798=EDGE_CURVE('',#33319,#33317,#27573,.T.) ;
#40799=EDGE_CURVE('',#33318,#33320,#10777,.T.) ;
#40800=EDGE_CURVE('',#33320,#33321,#10778,.T.) ;
#40801=EDGE_CURVE('',#33321,#33319,#10779,.T.) ;
#40802=EDGE_CURVE('',#33320,#33322,#27574,.T.) ;
#40803=EDGE_CURVE('',#33322,#33323,#10780,.T.) ;
#40804=EDGE_CURVE('',#33323,#33321,#27575,.T.) ;
#40805=EDGE_CURVE('',#33322,#33324,#10781,.T.) ;
#40806=EDGE_CURVE('',#33324,#33325,#10782,.T.) ;
#40807=EDGE_CURVE('',#33325,#33323,#10783,.T.) ;
#40808=EDGE_CURVE('',#33324,#33326,#27576,.T.) ;
#40809=EDGE_CURVE('',#33326,#33327,#10784,.T.) ;
#40810=EDGE_CURVE('',#33327,#33325,#27577,.T.) ;
#40811=EDGE_CURVE('',#33326,#33328,#10785,.T.) ;
#40812=EDGE_CURVE('',#33328,#33329,#10786,.T.) ;
#40813=EDGE_CURVE('',#33329,#33327,#10787,.T.) ;
#40814=EDGE_CURVE('',#33328,#33330,#27578,.T.) ;
#40815=EDGE_CURVE('',#33330,#33331,#10788,.T.) ;
#40816=EDGE_CURVE('',#33331,#33329,#27579,.T.) ;
#40817=EDGE_CURVE('',#33330,#33332,#27580,.T.) ;
#40818=EDGE_CURVE('',#33332,#33333,#10789,.T.) ;
#40819=EDGE_CURVE('',#33333,#33331,#27581,.T.) ;
#40820=EDGE_CURVE('',#33332,#33334,#27582,.T.) ;
#40821=EDGE_CURVE('',#33334,#33335,#10790,.T.) ;
#40822=EDGE_CURVE('',#33335,#33333,#27583,.T.) ;
#40823=EDGE_CURVE('',#33334,#33336,#10791,.T.) ;
#40824=EDGE_CURVE('',#33336,#33337,#10792,.T.) ;
#40825=EDGE_CURVE('',#33337,#33335,#10793,.T.) ;
#40826=EDGE_CURVE('',#33336,#33338,#27584,.T.) ;
#40827=EDGE_CURVE('',#33338,#33339,#10794,.T.) ;
#40828=EDGE_CURVE('',#33339,#33337,#27585,.T.) ;
#40829=EDGE_CURVE('',#33338,#33340,#10795,.T.) ;
#40830=EDGE_CURVE('',#33340,#33341,#10796,.T.) ;
#40831=EDGE_CURVE('',#33341,#33339,#10797,.T.) ;
#40832=EDGE_CURVE('',#33340,#33342,#27586,.T.) ;
#40833=EDGE_CURVE('',#33342,#33343,#10798,.T.) ;
#40834=EDGE_CURVE('',#33343,#33341,#27587,.T.) ;
#40835=EDGE_CURVE('',#33342,#33294,#10799,.T.) ;
#40836=EDGE_CURVE('',#33295,#33343,#10800,.T.) ;
#40837=EDGE_CURVE('',#33344,#33345,#27588,.T.) ;
#40838=EDGE_CURVE('',#33345,#33346,#10801,.T.) ;
#40839=EDGE_CURVE('',#33346,#33347,#27589,.T.) ;
#40840=EDGE_CURVE('',#33347,#33348,#10802,.T.) ;
#40841=EDGE_CURVE('',#33348,#33349,#10803,.T.) ;
#40842=EDGE_CURVE('',#33349,#33350,#10804,.T.) ;
#40843=EDGE_CURVE('',#33350,#33351,#27590,.T.) ;
#40844=EDGE_CURVE('',#33351,#33352,#10805,.T.) ;
#40845=EDGE_CURVE('',#33352,#33353,#10806,.T.) ;
#40846=EDGE_CURVE('',#33353,#33354,#10807,.T.) ;
#40847=EDGE_CURVE('',#33354,#33355,#27591,.T.) ;
#40848=EDGE_CURVE('',#33355,#33356,#10808,.T.) ;
#40849=EDGE_CURVE('',#33356,#33357,#27592,.T.) ;
#40850=EDGE_CURVE('',#33357,#33358,#10809,.T.) ;
#40851=EDGE_CURVE('',#33358,#33359,#10810,.T.) ;
#40852=EDGE_CURVE('',#33359,#32020,#10811,.T.) ;
#40853=EDGE_CURVE('',#32020,#33360,#10812,.T.) ;
#40854=EDGE_CURVE('',#33360,#33344,#10813,.T.) ;
#40855=EDGE_CURVE('',#33361,#33362,#10814,.T.) ;
#40856=EDGE_CURVE('',#33361,#33363,#27593,.T.) ;
#40857=EDGE_CURVE('',#33363,#33364,#10815,.T.) ;
#40858=EDGE_CURVE('',#33364,#33362,#27594,.T.) ;
#40859=EDGE_CURVE('',#33363,#33365,#10816,.T.) ;
#40860=EDGE_CURVE('',#33365,#33366,#10817,.T.) ;
#40861=EDGE_CURVE('',#33366,#33364,#10818,.T.) ;
#40862=EDGE_CURVE('',#33365,#33367,#27595,.T.) ;
#40863=EDGE_CURVE('',#33367,#33368,#10819,.T.) ;
#40864=EDGE_CURVE('',#33368,#33366,#27596,.T.) ;
#40865=EDGE_CURVE('',#33367,#33369,#10820,.T.) ;
#40866=EDGE_CURVE('',#33369,#33370,#10821,.T.) ;
#40867=EDGE_CURVE('',#33370,#33368,#10822,.T.) ;
#40868=EDGE_CURVE('',#33369,#33371,#27597,.T.) ;
#40869=EDGE_CURVE('',#33371,#33372,#10823,.T.) ;
#40870=EDGE_CURVE('',#33372,#33370,#27598,.T.) ;
#40871=EDGE_CURVE('',#33371,#32033,#10824,.T.) ;
#40872=EDGE_CURVE('',#32033,#33373,#10825,.T.) ;
#40873=EDGE_CURVE('',#33373,#33372,#10826,.T.) ;
#40874=EDGE_CURVE('',#32034,#33374,#10827,.T.) ;
#40875=EDGE_CURVE('',#33374,#33373,#27599,.T.) ;
#40876=EDGE_CURVE('',#32034,#32181,#10828,.T.) ;
#40877=EDGE_CURVE('',#32147,#33374,#10829,.T.) ;
#40878=EDGE_CURVE('',#32182,#33375,#10830,.T.) ;
#40879=EDGE_CURVE('',#33375,#33376,#10831,.T.) ;
#40880=EDGE_CURVE('',#33376,#32148,#10832,.T.) ;
#40881=EDGE_CURVE('',#33375,#33377,#27600,.T.) ;
#40882=EDGE_CURVE('',#33377,#33378,#10833,.T.) ;
#40883=EDGE_CURVE('',#33378,#33376,#27601,.T.) ;
#40884=EDGE_CURVE('',#33377,#33379,#10834,.T.) ;
#40885=EDGE_CURVE('',#33379,#33380,#10835,.T.) ;
#40886=EDGE_CURVE('',#33380,#33378,#10836,.T.) ;
#40887=EDGE_CURVE('',#33379,#33381,#27602,.T.) ;
#40888=EDGE_CURVE('',#33381,#33382,#10837,.T.) ;
#40889=EDGE_CURVE('',#33382,#33380,#27603,.T.) ;
#40890=EDGE_CURVE('',#33381,#33383,#10838,.T.) ;
#40891=EDGE_CURVE('',#33383,#33384,#10839,.T.) ;
#40892=EDGE_CURVE('',#33384,#33382,#10840,.T.) ;
#40893=EDGE_CURVE('',#33383,#33385,#27604,.T.) ;
#40894=EDGE_CURVE('',#33385,#33386,#10841,.T.) ;
#40895=EDGE_CURVE('',#33386,#33384,#27605,.T.) ;
#40896=EDGE_CURVE('',#33385,#33387,#10842,.T.) ;
#40897=EDGE_CURVE('',#33387,#33388,#10843,.T.) ;
#40898=EDGE_CURVE('',#33388,#33386,#10844,.T.) ;
#40899=EDGE_CURVE('',#33387,#33389,#27606,.T.) ;
#40900=EDGE_CURVE('',#33389,#33390,#10845,.T.) ;
#40901=EDGE_CURVE('',#33390,#33388,#27607,.T.) ;
#40902=EDGE_CURVE('',#33389,#33391,#10846,.T.) ;
#40903=EDGE_CURVE('',#33391,#33392,#10847,.T.) ;
#40904=EDGE_CURVE('',#33392,#33390,#10848,.T.) ;
#40905=EDGE_CURVE('',#33391,#33393,#27608,.T.) ;
#40906=EDGE_CURVE('',#33393,#33394,#10849,.T.) ;
#40907=EDGE_CURVE('',#33394,#33392,#27609,.T.) ;
#40908=EDGE_CURVE('',#33393,#33395,#10850,.T.) ;
#40909=EDGE_CURVE('',#33395,#33396,#10851,.T.) ;
#40910=EDGE_CURVE('',#33396,#33394,#10852,.T.) ;
#40911=EDGE_CURVE('',#33395,#33397,#27610,.T.) ;
#40912=EDGE_CURVE('',#33397,#33398,#10853,.T.) ;
#40913=EDGE_CURVE('',#33398,#33396,#27611,.T.) ;
#40914=EDGE_CURVE('',#33397,#33399,#27612,.T.) ;
#40915=EDGE_CURVE('',#33399,#33400,#10854,.T.) ;
#40916=EDGE_CURVE('',#33400,#33398,#27613,.T.) ;
#40917=EDGE_CURVE('',#33399,#33401,#27614,.T.) ;
#40918=EDGE_CURVE('',#33401,#33402,#10855,.T.) ;
#40919=EDGE_CURVE('',#33402,#33400,#27615,.T.) ;
#40920=EDGE_CURVE('',#33401,#33403,#10856,.T.) ;
#40921=EDGE_CURVE('',#33403,#33404,#10857,.T.) ;
#40922=EDGE_CURVE('',#33404,#33402,#10858,.T.) ;
#40923=EDGE_CURVE('',#33403,#33405,#27616,.T.) ;
#40924=EDGE_CURVE('',#33405,#33406,#10859,.T.) ;
#40925=EDGE_CURVE('',#33406,#33404,#27617,.T.) ;
#40926=EDGE_CURVE('',#33405,#33407,#10860,.T.) ;
#40927=EDGE_CURVE('',#33407,#33408,#10861,.T.) ;
#40928=EDGE_CURVE('',#33408,#33406,#10862,.T.) ;
#40929=EDGE_CURVE('',#33407,#33409,#27618,.T.) ;
#40930=EDGE_CURVE('',#33409,#33410,#10863,.T.) ;
#40931=EDGE_CURVE('',#33410,#33408,#27619,.T.) ;
#40932=EDGE_CURVE('',#33409,#33361,#10864,.T.) ;
#40933=EDGE_CURVE('',#33362,#33410,#10865,.T.) ;
#40934=EDGE_CURVE('',#33411,#33412,#27620,.T.) ;
#40935=EDGE_CURVE('',#33412,#33413,#10866,.T.) ;
#40936=EDGE_CURVE('',#33413,#33414,#27621,.T.) ;
#40937=EDGE_CURVE('',#33414,#33415,#10867,.T.) ;
#40938=EDGE_CURVE('',#33415,#33416,#10868,.T.) ;
#40939=EDGE_CURVE('',#33416,#33417,#10869,.T.) ;
#40940=EDGE_CURVE('',#33417,#33418,#27622,.T.) ;
#40941=EDGE_CURVE('',#33418,#33419,#10870,.T.) ;
#40942=EDGE_CURVE('',#33419,#33420,#10871,.T.) ;
#40943=EDGE_CURVE('',#33420,#33421,#10872,.T.) ;
#40944=EDGE_CURVE('',#33421,#33422,#27623,.T.) ;
#40945=EDGE_CURVE('',#33422,#33423,#10873,.T.) ;
#40946=EDGE_CURVE('',#33423,#33424,#27624,.T.) ;
#40947=EDGE_CURVE('',#33424,#33425,#10874,.T.) ;
#40948=EDGE_CURVE('',#33425,#33426,#10875,.T.) ;
#40949=EDGE_CURVE('',#33426,#32035,#10876,.T.) ;
#40950=EDGE_CURVE('',#32035,#33427,#10877,.T.) ;
#40951=EDGE_CURVE('',#33427,#33411,#10878,.T.) ;
#40952=EDGE_CURVE('',#33428,#33429,#10879,.T.) ;
#40953=EDGE_CURVE('',#33428,#33430,#27625,.T.) ;
#40954=EDGE_CURVE('',#33430,#33431,#10880,.T.) ;
#40955=EDGE_CURVE('',#33431,#33429,#27626,.T.) ;
#40956=EDGE_CURVE('',#33430,#33432,#10881,.T.) ;
#40957=EDGE_CURVE('',#33432,#33433,#10882,.T.) ;
#40958=EDGE_CURVE('',#33433,#33431,#10883,.T.) ;
#40959=EDGE_CURVE('',#33432,#33434,#27627,.T.) ;
#40960=EDGE_CURVE('',#33434,#33435,#10884,.T.) ;
#40961=EDGE_CURVE('',#33435,#33433,#27628,.T.) ;
#40962=EDGE_CURVE('',#33434,#33436,#10885,.T.) ;
#40963=EDGE_CURVE('',#33436,#33437,#10886,.T.) ;
#40964=EDGE_CURVE('',#33437,#33435,#10887,.T.) ;
#40965=EDGE_CURVE('',#33436,#33438,#27629,.T.) ;
#40966=EDGE_CURVE('',#33438,#33439,#10888,.T.) ;
#40967=EDGE_CURVE('',#33439,#33437,#27630,.T.) ;
#40968=EDGE_CURVE('',#33438,#32048,#10889,.T.) ;
#40969=EDGE_CURVE('',#32048,#33440,#10890,.T.) ;
#40970=EDGE_CURVE('',#33440,#33439,#10891,.T.) ;
#40971=EDGE_CURVE('',#32049,#33441,#10892,.T.) ;
#40972=EDGE_CURVE('',#33441,#33440,#27631,.T.) ;
#40973=EDGE_CURVE('',#32049,#32179,#10893,.T.) ;
#40974=EDGE_CURVE('',#32143,#33441,#10894,.T.) ;
#40975=EDGE_CURVE('',#32180,#33442,#10895,.T.) ;
#40976=EDGE_CURVE('',#33442,#33443,#10896,.T.) ;
#40977=EDGE_CURVE('',#33443,#32144,#10897,.T.) ;
#40978=EDGE_CURVE('',#33442,#33444,#27632,.T.) ;
#40979=EDGE_CURVE('',#33444,#33445,#10898,.T.) ;
#40980=EDGE_CURVE('',#33445,#33443,#27633,.T.) ;
#40981=EDGE_CURVE('',#33444,#33446,#10899,.T.) ;
#40982=EDGE_CURVE('',#33446,#33447,#10900,.T.) ;
#40983=EDGE_CURVE('',#33447,#33445,#10901,.T.) ;
#40984=EDGE_CURVE('',#33446,#33448,#27634,.T.) ;
#40985=EDGE_CURVE('',#33448,#33449,#10902,.T.) ;
#40986=EDGE_CURVE('',#33449,#33447,#27635,.T.) ;
#40987=EDGE_CURVE('',#33448,#33450,#10903,.T.) ;
#40988=EDGE_CURVE('',#33450,#33451,#10904,.T.) ;
#40989=EDGE_CURVE('',#33451,#33449,#10905,.T.) ;
#40990=EDGE_CURVE('',#33450,#33452,#27636,.T.) ;
#40991=EDGE_CURVE('',#33452,#33453,#10906,.T.) ;
#40992=EDGE_CURVE('',#33453,#33451,#27637,.T.) ;
#40993=EDGE_CURVE('',#33452,#33454,#10907,.T.) ;
#40994=EDGE_CURVE('',#33454,#33455,#10908,.T.) ;
#40995=EDGE_CURVE('',#33455,#33453,#10909,.T.) ;
#40996=EDGE_CURVE('',#33454,#33456,#27638,.T.) ;
#40997=EDGE_CURVE('',#33456,#33457,#10910,.T.) ;
#40998=EDGE_CURVE('',#33457,#33455,#27639,.T.) ;
#40999=EDGE_CURVE('',#33456,#33458,#10911,.T.) ;
#41000=EDGE_CURVE('',#33458,#33459,#10912,.T.) ;
#41001=EDGE_CURVE('',#33459,#33457,#10913,.T.) ;
#41002=EDGE_CURVE('',#33458,#33460,#27640,.T.) ;
#41003=EDGE_CURVE('',#33460,#33461,#10914,.T.) ;
#41004=EDGE_CURVE('',#33461,#33459,#27641,.T.) ;
#41005=EDGE_CURVE('',#33460,#33462,#10915,.T.) ;
#41006=EDGE_CURVE('',#33462,#33463,#10916,.T.) ;
#41007=EDGE_CURVE('',#33463,#33461,#10917,.T.) ;
#41008=EDGE_CURVE('',#33462,#33464,#27642,.T.) ;
#41009=EDGE_CURVE('',#33464,#33465,#10918,.T.) ;
#41010=EDGE_CURVE('',#33465,#33463,#27643,.T.) ;
#41011=EDGE_CURVE('',#33464,#33466,#27644,.T.) ;
#41012=EDGE_CURVE('',#33466,#33467,#10919,.T.) ;
#41013=EDGE_CURVE('',#33467,#33465,#27645,.T.) ;
#41014=EDGE_CURVE('',#33466,#33468,#27646,.T.) ;
#41015=EDGE_CURVE('',#33468,#33469,#10920,.T.) ;
#41016=EDGE_CURVE('',#33469,#33467,#27647,.T.) ;
#41017=EDGE_CURVE('',#33468,#33470,#10921,.T.) ;
#41018=EDGE_CURVE('',#33470,#33471,#10922,.T.) ;
#41019=EDGE_CURVE('',#33471,#33469,#10923,.T.) ;
#41020=EDGE_CURVE('',#33470,#33472,#27648,.T.) ;
#41021=EDGE_CURVE('',#33472,#33473,#10924,.T.) ;
#41022=EDGE_CURVE('',#33473,#33471,#27649,.T.) ;
#41023=EDGE_CURVE('',#33472,#33474,#10925,.T.) ;
#41024=EDGE_CURVE('',#33474,#33475,#10926,.T.) ;
#41025=EDGE_CURVE('',#33475,#33473,#10927,.T.) ;
#41026=EDGE_CURVE('',#33474,#33476,#27650,.T.) ;
#41027=EDGE_CURVE('',#33476,#33477,#10928,.T.) ;
#41028=EDGE_CURVE('',#33477,#33475,#27651,.T.) ;
#41029=EDGE_CURVE('',#33476,#33428,#10929,.T.) ;
#41030=EDGE_CURVE('',#33429,#33477,#10930,.T.) ;
#41031=EDGE_CURVE('',#33478,#33479,#27652,.T.) ;
#41032=EDGE_CURVE('',#33479,#33480,#10931,.T.) ;
#41033=EDGE_CURVE('',#33480,#33481,#27653,.T.) ;
#41034=EDGE_CURVE('',#33481,#33482,#10932,.T.) ;
#41035=EDGE_CURVE('',#33482,#33483,#10933,.T.) ;
#41036=EDGE_CURVE('',#33483,#33484,#10934,.T.) ;
#41037=EDGE_CURVE('',#33484,#33485,#27654,.T.) ;
#41038=EDGE_CURVE('',#33485,#33486,#10935,.T.) ;
#41039=EDGE_CURVE('',#33486,#33487,#10936,.T.) ;
#41040=EDGE_CURVE('',#33487,#33488,#10937,.T.) ;
#41041=EDGE_CURVE('',#33488,#33489,#27655,.T.) ;
#41042=EDGE_CURVE('',#33489,#33490,#10938,.T.) ;
#41043=EDGE_CURVE('',#33490,#33491,#27656,.T.) ;
#41044=EDGE_CURVE('',#33491,#33492,#10939,.T.) ;
#41045=EDGE_CURVE('',#33492,#33493,#10940,.T.) ;
#41046=EDGE_CURVE('',#33493,#32050,#10941,.T.) ;
#41047=EDGE_CURVE('',#32050,#33494,#10942,.T.) ;
#41048=EDGE_CURVE('',#33494,#33478,#10943,.T.) ;
#41049=EDGE_CURVE('',#33495,#33496,#10944,.T.) ;
#41050=EDGE_CURVE('',#33495,#33497,#27657,.T.) ;
#41051=EDGE_CURVE('',#33497,#33498,#10945,.T.) ;
#41052=EDGE_CURVE('',#33498,#33496,#27658,.T.) ;
#41053=EDGE_CURVE('',#33497,#33499,#10946,.T.) ;
#41054=EDGE_CURVE('',#33499,#33500,#10947,.T.) ;
#41055=EDGE_CURVE('',#33500,#33498,#10948,.T.) ;
#41056=EDGE_CURVE('',#33499,#33501,#27659,.T.) ;
#41057=EDGE_CURVE('',#33501,#33502,#10949,.T.) ;
#41058=EDGE_CURVE('',#33502,#33500,#27660,.T.) ;
#41059=EDGE_CURVE('',#33501,#33503,#10950,.T.) ;
#41060=EDGE_CURVE('',#33503,#33504,#10951,.T.) ;
#41061=EDGE_CURVE('',#33504,#33502,#10952,.T.) ;
#41062=EDGE_CURVE('',#33503,#33505,#27661,.T.) ;
#41063=EDGE_CURVE('',#33505,#33506,#10953,.T.) ;
#41064=EDGE_CURVE('',#33506,#33504,#27662,.T.) ;
#41065=EDGE_CURVE('',#33505,#32063,#10954,.T.) ;
#41066=EDGE_CURVE('',#32063,#33507,#10955,.T.) ;
#41067=EDGE_CURVE('',#33507,#33506,#10956,.T.) ;
#41068=EDGE_CURVE('',#32064,#33508,#10957,.T.) ;
#41069=EDGE_CURVE('',#33508,#33507,#27663,.T.) ;
#41070=EDGE_CURVE('',#32064,#32177,#10958,.T.) ;
#41071=EDGE_CURVE('',#32139,#33508,#10959,.T.) ;
#41072=EDGE_CURVE('',#32178,#33509,#10960,.T.) ;
#41073=EDGE_CURVE('',#33509,#33510,#10961,.T.) ;
#41074=EDGE_CURVE('',#33510,#32140,#10962,.T.) ;
#41075=EDGE_CURVE('',#33509,#33511,#27664,.T.) ;
#41076=EDGE_CURVE('',#33511,#33512,#10963,.T.) ;
#41077=EDGE_CURVE('',#33512,#33510,#27665,.T.) ;
#41078=EDGE_CURVE('',#33511,#33513,#10964,.T.) ;
#41079=EDGE_CURVE('',#33513,#33514,#10965,.T.) ;
#41080=EDGE_CURVE('',#33514,#33512,#10966,.T.) ;
#41081=EDGE_CURVE('',#33513,#33515,#27666,.T.) ;
#41082=EDGE_CURVE('',#33515,#33516,#10967,.T.) ;
#41083=EDGE_CURVE('',#33516,#33514,#27667,.T.) ;
#41084=EDGE_CURVE('',#33515,#33517,#10968,.T.) ;
#41085=EDGE_CURVE('',#33517,#33518,#10969,.T.) ;
#41086=EDGE_CURVE('',#33518,#33516,#10970,.T.) ;
#41087=EDGE_CURVE('',#33517,#33519,#27668,.T.) ;
#41088=EDGE_CURVE('',#33519,#33520,#10971,.T.) ;
#41089=EDGE_CURVE('',#33520,#33518,#27669,.T.) ;
#41090=EDGE_CURVE('',#33519,#33521,#10972,.T.) ;
#41091=EDGE_CURVE('',#33521,#33522,#10973,.T.) ;
#41092=EDGE_CURVE('',#33522,#33520,#10974,.T.) ;
#41093=EDGE_CURVE('',#33521,#33523,#27670,.T.) ;
#41094=EDGE_CURVE('',#33523,#33524,#10975,.T.) ;
#41095=EDGE_CURVE('',#33524,#33522,#27671,.T.) ;
#41096=EDGE_CURVE('',#33523,#33525,#10976,.T.) ;
#41097=EDGE_CURVE('',#33525,#33526,#10977,.T.) ;
#41098=EDGE_CURVE('',#33526,#33524,#10978,.T.) ;
#41099=EDGE_CURVE('',#33525,#33527,#27672,.T.) ;
#41100=EDGE_CURVE('',#33527,#33528,#10979,.T.) ;
#41101=EDGE_CURVE('',#33528,#33526,#27673,.T.) ;
#41102=EDGE_CURVE('',#33527,#33529,#10980,.T.) ;
#41103=EDGE_CURVE('',#33529,#33530,#10981,.T.) ;
#41104=EDGE_CURVE('',#33530,#33528,#10982,.T.) ;
#41105=EDGE_CURVE('',#33529,#33531,#27674,.T.) ;
#41106=EDGE_CURVE('',#33531,#33532,#10983,.T.) ;
#41107=EDGE_CURVE('',#33532,#33530,#27675,.T.) ;
#41108=EDGE_CURVE('',#33531,#33533,#27676,.T.) ;
#41109=EDGE_CURVE('',#33533,#33534,#10984,.T.) ;
#41110=EDGE_CURVE('',#33534,#33532,#27677,.T.) ;
#41111=EDGE_CURVE('',#33533,#33535,#27678,.T.) ;
#41112=EDGE_CURVE('',#33535,#33536,#10985,.T.) ;
#41113=EDGE_CURVE('',#33536,#33534,#27679,.T.) ;
#41114=EDGE_CURVE('',#33535,#33537,#10986,.T.) ;
#41115=EDGE_CURVE('',#33537,#33538,#10987,.T.) ;
#41116=EDGE_CURVE('',#33538,#33536,#10988,.T.) ;
#41117=EDGE_CURVE('',#33537,#33539,#27680,.T.) ;
#41118=EDGE_CURVE('',#33539,#33540,#10989,.T.) ;
#41119=EDGE_CURVE('',#33540,#33538,#27681,.T.) ;
#41120=EDGE_CURVE('',#33539,#33541,#10990,.T.) ;
#41121=EDGE_CURVE('',#33541,#33542,#10991,.T.) ;
#41122=EDGE_CURVE('',#33542,#33540,#10992,.T.) ;
#41123=EDGE_CURVE('',#33541,#33543,#27682,.T.) ;
#41124=EDGE_CURVE('',#33543,#33544,#10993,.T.) ;
#41125=EDGE_CURVE('',#33544,#33542,#27683,.T.) ;
#41126=EDGE_CURVE('',#33543,#33495,#10994,.T.) ;
#41127=EDGE_CURVE('',#33496,#33544,#10995,.T.) ;
#41128=EDGE_CURVE('',#33545,#33546,#27684,.T.) ;
#41129=EDGE_CURVE('',#33546,#33547,#10996,.T.) ;
#41130=EDGE_CURVE('',#33547,#33548,#27685,.T.) ;
#41131=EDGE_CURVE('',#33548,#33549,#10997,.T.) ;
#41132=EDGE_CURVE('',#33549,#33550,#10998,.T.) ;
#41133=EDGE_CURVE('',#33550,#33551,#10999,.T.) ;
#41134=EDGE_CURVE('',#33551,#33552,#27686,.T.) ;
#41135=EDGE_CURVE('',#33552,#33553,#11000,.T.) ;
#41136=EDGE_CURVE('',#33553,#33554,#11001,.T.) ;
#41137=EDGE_CURVE('',#33554,#33555,#11002,.T.) ;
#41138=EDGE_CURVE('',#33555,#33556,#27687,.T.) ;
#41139=EDGE_CURVE('',#33556,#33557,#11003,.T.) ;
#41140=EDGE_CURVE('',#33557,#33558,#27688,.T.) ;
#41141=EDGE_CURVE('',#33558,#33559,#11004,.T.) ;
#41142=EDGE_CURVE('',#33559,#33560,#11005,.T.) ;
#41143=EDGE_CURVE('',#33560,#32065,#11006,.T.) ;
#41144=EDGE_CURVE('',#32065,#33561,#11007,.T.) ;
#41145=EDGE_CURVE('',#33561,#33545,#11008,.T.) ;
#41146=EDGE_CURVE('',#33562,#33563,#11009,.T.) ;
#41147=EDGE_CURVE('',#33562,#33564,#27689,.T.) ;
#41148=EDGE_CURVE('',#33564,#33565,#11010,.T.) ;
#41149=EDGE_CURVE('',#33565,#33563,#27690,.T.) ;
#41150=EDGE_CURVE('',#33564,#33566,#11011,.T.) ;
#41151=EDGE_CURVE('',#33566,#33567,#11012,.T.) ;
#41152=EDGE_CURVE('',#33567,#33565,#11013,.T.) ;
#41153=EDGE_CURVE('',#33566,#33568,#27691,.T.) ;
#41154=EDGE_CURVE('',#33568,#33569,#11014,.T.) ;
#41155=EDGE_CURVE('',#33569,#33567,#27692,.T.) ;
#41156=EDGE_CURVE('',#33568,#33570,#11015,.T.) ;
#41157=EDGE_CURVE('',#33570,#33571,#11016,.T.) ;
#41158=EDGE_CURVE('',#33571,#33569,#11017,.T.) ;
#41159=EDGE_CURVE('',#33570,#33572,#27693,.T.) ;
#41160=EDGE_CURVE('',#33572,#33573,#11018,.T.) ;
#41161=EDGE_CURVE('',#33573,#33571,#27694,.T.) ;
#41162=EDGE_CURVE('',#33572,#32078,#11019,.T.) ;
#41163=EDGE_CURVE('',#32078,#33574,#11020,.T.) ;
#41164=EDGE_CURVE('',#33574,#33573,#11021,.T.) ;
#41165=EDGE_CURVE('',#32079,#33575,#11022,.T.) ;
#41166=EDGE_CURVE('',#33575,#33574,#27695,.T.) ;
#41167=EDGE_CURVE('',#32079,#32175,#11023,.T.) ;
#41168=EDGE_CURVE('',#32135,#33575,#11024,.T.) ;
#41169=EDGE_CURVE('',#32176,#33576,#11025,.T.) ;
#41170=EDGE_CURVE('',#33576,#33577,#11026,.T.) ;
#41171=EDGE_CURVE('',#33577,#32136,#11027,.T.) ;
#41172=EDGE_CURVE('',#33576,#33578,#27696,.T.) ;
#41173=EDGE_CURVE('',#33578,#33579,#11028,.T.) ;
#41174=EDGE_CURVE('',#33579,#33577,#27697,.T.) ;
#41175=EDGE_CURVE('',#33578,#33580,#11029,.T.) ;
#41176=EDGE_CURVE('',#33580,#33581,#11030,.T.) ;
#41177=EDGE_CURVE('',#33581,#33579,#11031,.T.) ;
#41178=EDGE_CURVE('',#33580,#33582,#27698,.T.) ;
#41179=EDGE_CURVE('',#33582,#33583,#11032,.T.) ;
#41180=EDGE_CURVE('',#33583,#33581,#27699,.T.) ;
#41181=EDGE_CURVE('',#33582,#33584,#11033,.T.) ;
#41182=EDGE_CURVE('',#33584,#33585,#11034,.T.) ;
#41183=EDGE_CURVE('',#33585,#33583,#11035,.T.) ;
#41184=EDGE_CURVE('',#33584,#33586,#27700,.T.) ;
#41185=EDGE_CURVE('',#33586,#33587,#11036,.T.) ;
#41186=EDGE_CURVE('',#33587,#33585,#27701,.T.) ;
#41187=EDGE_CURVE('',#33586,#33588,#11037,.T.) ;
#41188=EDGE_CURVE('',#33588,#33589,#11038,.T.) ;
#41189=EDGE_CURVE('',#33589,#33587,#11039,.T.) ;
#41190=EDGE_CURVE('',#33588,#33590,#27702,.T.) ;
#41191=EDGE_CURVE('',#33590,#33591,#11040,.T.) ;
#41192=EDGE_CURVE('',#33591,#33589,#27703,.T.) ;
#41193=EDGE_CURVE('',#33590,#33592,#11041,.T.) ;
#41194=EDGE_CURVE('',#33592,#33593,#11042,.T.) ;
#41195=EDGE_CURVE('',#33593,#33591,#11043,.T.) ;
#41196=EDGE_CURVE('',#33592,#33594,#27704,.T.) ;
#41197=EDGE_CURVE('',#33594,#33595,#11044,.T.) ;
#41198=EDGE_CURVE('',#33595,#33593,#27705,.T.) ;
#41199=EDGE_CURVE('',#33594,#33596,#11045,.T.) ;
#41200=EDGE_CURVE('',#33596,#33597,#11046,.T.) ;
#41201=EDGE_CURVE('',#33597,#33595,#11047,.T.) ;
#41202=EDGE_CURVE('',#33596,#33598,#27706,.T.) ;
#41203=EDGE_CURVE('',#33598,#33599,#11048,.T.) ;
#41204=EDGE_CURVE('',#33599,#33597,#27707,.T.) ;
#41205=EDGE_CURVE('',#33598,#33600,#27708,.T.) ;
#41206=EDGE_CURVE('',#33600,#33601,#11049,.T.) ;
#41207=EDGE_CURVE('',#33601,#33599,#27709,.T.) ;
#41208=EDGE_CURVE('',#33600,#33602,#27710,.T.) ;
#41209=EDGE_CURVE('',#33602,#33603,#11050,.T.) ;
#41210=EDGE_CURVE('',#33603,#33601,#27711,.T.) ;
#41211=EDGE_CURVE('',#33602,#33604,#11051,.T.) ;
#41212=EDGE_CURVE('',#33604,#33605,#11052,.T.) ;
#41213=EDGE_CURVE('',#33605,#33603,#11053,.T.) ;
#41214=EDGE_CURVE('',#33604,#33606,#27712,.T.) ;
#41215=EDGE_CURVE('',#33606,#33607,#11054,.T.) ;
#41216=EDGE_CURVE('',#33607,#33605,#27713,.T.) ;
#41217=EDGE_CURVE('',#33606,#33608,#11055,.T.) ;
#41218=EDGE_CURVE('',#33608,#33609,#11056,.T.) ;
#41219=EDGE_CURVE('',#33609,#33607,#11057,.T.) ;
#41220=EDGE_CURVE('',#33608,#33610,#27714,.T.) ;
#41221=EDGE_CURVE('',#33610,#33611,#11058,.T.) ;
#41222=EDGE_CURVE('',#33611,#33609,#27715,.T.) ;
#41223=EDGE_CURVE('',#33610,#33562,#11059,.T.) ;
#41224=EDGE_CURVE('',#33563,#33611,#11060,.T.) ;
#41225=EDGE_CURVE('',#33612,#33613,#27716,.T.) ;
#41226=EDGE_CURVE('',#33613,#33614,#11061,.T.) ;
#41227=EDGE_CURVE('',#33614,#33615,#27717,.T.) ;
#41228=EDGE_CURVE('',#33615,#33616,#11062,.T.) ;
#41229=EDGE_CURVE('',#33616,#33617,#11063,.T.) ;
#41230=EDGE_CURVE('',#33617,#33618,#11064,.T.) ;
#41231=EDGE_CURVE('',#33618,#33619,#27718,.T.) ;
#41232=EDGE_CURVE('',#33619,#33620,#11065,.T.) ;
#41233=EDGE_CURVE('',#33620,#33621,#11066,.T.) ;
#41234=EDGE_CURVE('',#33621,#33622,#11067,.T.) ;
#41235=EDGE_CURVE('',#33622,#33623,#27719,.T.) ;
#41236=EDGE_CURVE('',#33623,#33624,#11068,.T.) ;
#41237=EDGE_CURVE('',#33624,#33625,#27720,.T.) ;
#41238=EDGE_CURVE('',#33625,#33626,#11069,.T.) ;
#41239=EDGE_CURVE('',#33626,#33627,#11070,.T.) ;
#41240=EDGE_CURVE('',#33627,#32080,#11071,.T.) ;
#41241=EDGE_CURVE('',#32080,#33628,#11072,.T.) ;
#41242=EDGE_CURVE('',#33628,#33612,#11073,.T.) ;
#41243=EDGE_CURVE('',#33629,#33630,#11074,.T.) ;
#41244=EDGE_CURVE('',#33629,#33631,#27721,.T.) ;
#41245=EDGE_CURVE('',#33631,#33632,#11075,.T.) ;
#41246=EDGE_CURVE('',#33632,#33630,#27722,.T.) ;
#41247=EDGE_CURVE('',#33631,#33633,#11076,.T.) ;
#41248=EDGE_CURVE('',#33633,#33634,#11077,.T.) ;
#41249=EDGE_CURVE('',#33634,#33632,#11078,.T.) ;
#41250=EDGE_CURVE('',#33633,#33635,#27723,.T.) ;
#41251=EDGE_CURVE('',#33635,#33636,#11079,.T.) ;
#41252=EDGE_CURVE('',#33636,#33634,#27724,.T.) ;
#41253=EDGE_CURVE('',#33635,#33637,#11080,.T.) ;
#41254=EDGE_CURVE('',#33637,#33638,#11081,.T.) ;
#41255=EDGE_CURVE('',#33638,#33636,#11082,.T.) ;
#41256=EDGE_CURVE('',#33637,#33639,#27725,.T.) ;
#41257=EDGE_CURVE('',#33639,#33640,#11083,.T.) ;
#41258=EDGE_CURVE('',#33640,#33638,#27726,.T.) ;
#41259=EDGE_CURVE('',#33639,#32093,#11084,.T.) ;
#41260=EDGE_CURVE('',#32093,#33641,#11085,.T.) ;
#41261=EDGE_CURVE('',#33641,#33640,#11086,.T.) ;
#41262=EDGE_CURVE('',#32094,#33642,#11087,.T.) ;
#41263=EDGE_CURVE('',#33642,#33641,#27727,.T.) ;
#41264=EDGE_CURVE('',#32094,#32173,#11088,.T.) ;
#41265=EDGE_CURVE('',#32131,#33642,#11089,.T.) ;
#41266=EDGE_CURVE('',#32174,#33643,#11090,.T.) ;
#41267=EDGE_CURVE('',#33643,#33644,#11091,.T.) ;
#41268=EDGE_CURVE('',#33644,#32132,#11092,.T.) ;
#41269=EDGE_CURVE('',#33643,#33645,#27728,.T.) ;
#41270=EDGE_CURVE('',#33645,#33646,#11093,.T.) ;
#41271=EDGE_CURVE('',#33646,#33644,#27729,.T.) ;
#41272=EDGE_CURVE('',#33645,#33647,#11094,.T.) ;
#41273=EDGE_CURVE('',#33647,#33648,#11095,.T.) ;
#41274=EDGE_CURVE('',#33648,#33646,#11096,.T.) ;
#41275=EDGE_CURVE('',#33647,#33649,#27730,.T.) ;
#41276=EDGE_CURVE('',#33649,#33650,#11097,.T.) ;
#41277=EDGE_CURVE('',#33650,#33648,#27731,.T.) ;
#41278=EDGE_CURVE('',#33649,#33651,#11098,.T.) ;
#41279=EDGE_CURVE('',#33651,#33652,#11099,.T.) ;
#41280=EDGE_CURVE('',#33652,#33650,#11100,.T.) ;
#41281=EDGE_CURVE('',#33651,#33653,#27732,.T.) ;
#41282=EDGE_CURVE('',#33653,#33654,#11101,.T.) ;
#41283=EDGE_CURVE('',#33654,#33652,#27733,.T.) ;
#41284=EDGE_CURVE('',#33653,#33655,#11102,.T.) ;
#41285=EDGE_CURVE('',#33655,#33656,#11103,.T.) ;
#41286=EDGE_CURVE('',#33656,#33654,#11104,.T.) ;
#41287=EDGE_CURVE('',#33655,#33657,#27734,.T.) ;
#41288=EDGE_CURVE('',#33657,#33658,#11105,.T.) ;
#41289=EDGE_CURVE('',#33658,#33656,#27735,.T.) ;
#41290=EDGE_CURVE('',#33657,#33659,#11106,.T.) ;
#41291=EDGE_CURVE('',#33659,#33660,#11107,.T.) ;
#41292=EDGE_CURVE('',#33660,#33658,#11108,.T.) ;
#41293=EDGE_CURVE('',#33659,#33661,#27736,.T.) ;
#41294=EDGE_CURVE('',#33661,#33662,#11109,.T.) ;
#41295=EDGE_CURVE('',#33662,#33660,#27737,.T.) ;
#41296=EDGE_CURVE('',#33661,#33663,#11110,.T.) ;
#41297=EDGE_CURVE('',#33663,#33664,#11111,.T.) ;
#41298=EDGE_CURVE('',#33664,#33662,#11112,.T.) ;
#41299=EDGE_CURVE('',#33663,#33665,#27738,.T.) ;
#41300=EDGE_CURVE('',#33665,#33666,#11113,.T.) ;
#41301=EDGE_CURVE('',#33666,#33664,#27739,.T.) ;
#41302=EDGE_CURVE('',#33665,#33667,#27740,.T.) ;
#41303=EDGE_CURVE('',#33667,#33668,#11114,.T.) ;
#41304=EDGE_CURVE('',#33668,#33666,#27741,.T.) ;
#41305=EDGE_CURVE('',#33667,#33669,#27742,.T.) ;
#41306=EDGE_CURVE('',#33669,#33670,#11115,.T.) ;
#41307=EDGE_CURVE('',#33670,#33668,#27743,.T.) ;
#41308=EDGE_CURVE('',#33669,#33671,#11116,.T.) ;
#41309=EDGE_CURVE('',#33671,#33672,#11117,.T.) ;
#41310=EDGE_CURVE('',#33672,#33670,#11118,.T.) ;
#41311=EDGE_CURVE('',#33671,#33673,#27744,.T.) ;
#41312=EDGE_CURVE('',#33673,#33674,#11119,.T.) ;
#41313=EDGE_CURVE('',#33674,#33672,#27745,.T.) ;
#41314=EDGE_CURVE('',#33673,#33675,#11120,.T.) ;
#41315=EDGE_CURVE('',#33675,#33676,#11121,.T.) ;
#41316=EDGE_CURVE('',#33676,#33674,#11122,.T.) ;
#41317=EDGE_CURVE('',#33675,#33677,#27746,.T.) ;
#41318=EDGE_CURVE('',#33677,#33678,#11123,.T.) ;
#41319=EDGE_CURVE('',#33678,#33676,#27747,.T.) ;
#41320=EDGE_CURVE('',#33677,#33629,#11124,.T.) ;
#41321=EDGE_CURVE('',#33630,#33678,#11125,.T.) ;
#41322=EDGE_CURVE('',#33679,#33680,#27748,.T.) ;
#41323=EDGE_CURVE('',#33680,#33681,#11126,.T.) ;
#41324=EDGE_CURVE('',#33681,#33682,#27749,.T.) ;
#41325=EDGE_CURVE('',#33682,#33683,#11127,.T.) ;
#41326=EDGE_CURVE('',#33683,#33684,#11128,.T.) ;
#41327=EDGE_CURVE('',#33684,#33685,#11129,.T.) ;
#41328=EDGE_CURVE('',#33685,#33686,#27750,.T.) ;
#41329=EDGE_CURVE('',#33686,#33687,#11130,.T.) ;
#41330=EDGE_CURVE('',#33687,#33688,#11131,.T.) ;
#41331=EDGE_CURVE('',#33688,#33689,#11132,.T.) ;
#41332=EDGE_CURVE('',#33689,#33690,#27751,.T.) ;
#41333=EDGE_CURVE('',#33690,#33691,#11133,.T.) ;
#41334=EDGE_CURVE('',#33691,#33692,#27752,.T.) ;
#41335=EDGE_CURVE('',#33692,#33693,#11134,.T.) ;
#41336=EDGE_CURVE('',#33693,#33694,#11135,.T.) ;
#41337=EDGE_CURVE('',#33694,#32095,#11136,.T.) ;
#41338=EDGE_CURVE('',#32095,#33695,#11137,.T.) ;
#41339=EDGE_CURVE('',#33695,#33679,#11138,.T.) ;
#41340=EDGE_CURVE('',#33696,#33697,#11139,.T.) ;
#41341=EDGE_CURVE('',#33696,#33698,#27753,.T.) ;
#41342=EDGE_CURVE('',#33698,#33699,#11140,.T.) ;
#41343=EDGE_CURVE('',#33699,#33697,#27754,.T.) ;
#41344=EDGE_CURVE('',#33698,#33700,#11141,.T.) ;
#41345=EDGE_CURVE('',#33700,#33701,#11142,.T.) ;
#41346=EDGE_CURVE('',#33701,#33699,#11143,.T.) ;
#41347=EDGE_CURVE('',#33700,#33702,#27755,.T.) ;
#41348=EDGE_CURVE('',#33702,#33703,#11144,.T.) ;
#41349=EDGE_CURVE('',#33703,#33701,#27756,.T.) ;
#41350=EDGE_CURVE('',#33702,#33704,#11145,.T.) ;
#41351=EDGE_CURVE('',#33704,#33705,#11146,.T.) ;
#41352=EDGE_CURVE('',#33705,#33703,#11147,.T.) ;
#41353=EDGE_CURVE('',#33704,#33706,#27757,.T.) ;
#41354=EDGE_CURVE('',#33706,#33707,#11148,.T.) ;
#41355=EDGE_CURVE('',#33707,#33705,#27758,.T.) ;
#41356=EDGE_CURVE('',#33706,#32108,#11149,.T.) ;
#41357=EDGE_CURVE('',#32108,#33708,#11150,.T.) ;
#41358=EDGE_CURVE('',#33708,#33707,#11151,.T.) ;
#41359=EDGE_CURVE('',#32109,#33709,#11152,.T.) ;
#41360=EDGE_CURVE('',#33709,#33708,#27759,.T.) ;
#41361=EDGE_CURVE('',#32109,#32171,#11153,.T.) ;
#41362=EDGE_CURVE('',#32127,#33709,#11154,.T.) ;
#41363=EDGE_CURVE('',#32172,#33710,#11155,.T.) ;
#41364=EDGE_CURVE('',#33710,#33711,#11156,.T.) ;
#41365=EDGE_CURVE('',#33711,#32128,#11157,.T.) ;
#41366=EDGE_CURVE('',#33710,#33712,#27760,.T.) ;
#41367=EDGE_CURVE('',#33712,#33713,#11158,.T.) ;
#41368=EDGE_CURVE('',#33713,#33711,#27761,.T.) ;
#41369=EDGE_CURVE('',#33712,#33714,#11159,.T.) ;
#41370=EDGE_CURVE('',#33714,#33715,#11160,.T.) ;
#41371=EDGE_CURVE('',#33715,#33713,#11161,.T.) ;
#41372=EDGE_CURVE('',#33714,#33716,#27762,.T.) ;
#41373=EDGE_CURVE('',#33716,#33717,#11162,.T.) ;
#41374=EDGE_CURVE('',#33717,#33715,#27763,.T.) ;
#41375=EDGE_CURVE('',#33716,#33718,#11163,.T.) ;
#41376=EDGE_CURVE('',#33718,#33719,#11164,.T.) ;
#41377=EDGE_CURVE('',#33719,#33717,#11165,.T.) ;
#41378=EDGE_CURVE('',#33718,#33720,#27764,.T.) ;
#41379=EDGE_CURVE('',#33720,#33721,#11166,.T.) ;
#41380=EDGE_CURVE('',#33721,#33719,#27765,.T.) ;
#41381=EDGE_CURVE('',#33720,#33722,#11167,.T.) ;
#41382=EDGE_CURVE('',#33722,#33723,#11168,.T.) ;
#41383=EDGE_CURVE('',#33723,#33721,#11169,.T.) ;
#41384=EDGE_CURVE('',#33722,#33724,#27766,.T.) ;
#41385=EDGE_CURVE('',#33724,#33725,#11170,.T.) ;
#41386=EDGE_CURVE('',#33725,#33723,#27767,.T.) ;
#41387=EDGE_CURVE('',#33724,#33726,#11171,.T.) ;
#41388=EDGE_CURVE('',#33726,#33727,#11172,.T.) ;
#41389=EDGE_CURVE('',#33727,#33725,#11173,.T.) ;
#41390=EDGE_CURVE('',#33726,#33728,#27768,.T.) ;
#41391=EDGE_CURVE('',#33728,#33729,#11174,.T.) ;
#41392=EDGE_CURVE('',#33729,#33727,#27769,.T.) ;
#41393=EDGE_CURVE('',#33728,#33730,#11175,.T.) ;
#41394=EDGE_CURVE('',#33730,#33731,#11176,.T.) ;
#41395=EDGE_CURVE('',#33731,#33729,#11177,.T.) ;
#41396=EDGE_CURVE('',#33730,#33732,#27770,.T.) ;
#41397=EDGE_CURVE('',#33732,#33733,#11178,.T.) ;
#41398=EDGE_CURVE('',#33733,#33731,#27771,.T.) ;
#41399=EDGE_CURVE('',#33732,#33734,#27772,.T.) ;
#41400=EDGE_CURVE('',#33734,#33735,#11179,.T.) ;
#41401=EDGE_CURVE('',#33735,#33733,#27773,.T.) ;
#41402=EDGE_CURVE('',#33734,#33736,#27774,.T.) ;
#41403=EDGE_CURVE('',#33736,#33737,#11180,.T.) ;
#41404=EDGE_CURVE('',#33737,#33735,#27775,.T.) ;
#41405=EDGE_CURVE('',#33736,#33738,#11181,.T.) ;
#41406=EDGE_CURVE('',#33738,#33739,#11182,.T.) ;
#41407=EDGE_CURVE('',#33739,#33737,#11183,.T.) ;
#41408=EDGE_CURVE('',#33738,#33740,#27776,.T.) ;
#41409=EDGE_CURVE('',#33740,#33741,#11184,.T.) ;
#41410=EDGE_CURVE('',#33741,#33739,#27777,.T.) ;
#41411=EDGE_CURVE('',#33740,#33742,#11185,.T.) ;
#41412=EDGE_CURVE('',#33742,#33743,#11186,.T.) ;
#41413=EDGE_CURVE('',#33743,#33741,#11187,.T.) ;
#41414=EDGE_CURVE('',#33742,#33744,#27778,.T.) ;
#41415=EDGE_CURVE('',#33744,#33745,#11188,.T.) ;
#41416=EDGE_CURVE('',#33745,#33743,#27779,.T.) ;
#41417=EDGE_CURVE('',#33744,#33696,#11189,.T.) ;
#41418=EDGE_CURVE('',#33697,#33745,#11190,.T.) ;
#41419=EDGE_CURVE('',#33746,#33747,#27780,.T.) ;
#41420=EDGE_CURVE('',#33747,#33748,#11191,.T.) ;
#41421=EDGE_CURVE('',#33748,#33749,#27781,.T.) ;
#41422=EDGE_CURVE('',#33749,#33750,#11192,.T.) ;
#41423=EDGE_CURVE('',#33750,#33751,#11193,.T.) ;
#41424=EDGE_CURVE('',#33751,#33752,#11194,.T.) ;
#41425=EDGE_CURVE('',#33752,#33753,#27782,.T.) ;
#41426=EDGE_CURVE('',#33753,#33754,#11195,.T.) ;
#41427=EDGE_CURVE('',#33754,#33755,#11196,.T.) ;
#41428=EDGE_CURVE('',#33755,#33756,#11197,.T.) ;
#41429=EDGE_CURVE('',#33756,#33757,#27783,.T.) ;
#41430=EDGE_CURVE('',#33757,#33758,#11198,.T.) ;
#41431=EDGE_CURVE('',#33758,#33759,#27784,.T.) ;
#41432=EDGE_CURVE('',#33759,#33760,#11199,.T.) ;
#41433=EDGE_CURVE('',#33760,#33761,#11200,.T.) ;
#41434=EDGE_CURVE('',#33761,#32110,#11201,.T.) ;
#41435=EDGE_CURVE('',#32110,#33762,#11202,.T.) ;
#41436=EDGE_CURVE('',#33762,#33746,#11203,.T.) ;
#41437=EDGE_CURVE('',#33763,#33764,#11204,.T.) ;
#41438=EDGE_CURVE('',#33763,#33765,#27785,.T.) ;
#41439=EDGE_CURVE('',#33765,#33766,#11205,.T.) ;
#41440=EDGE_CURVE('',#33766,#33764,#27786,.T.) ;
#41441=EDGE_CURVE('',#33765,#33767,#11206,.T.) ;
#41442=EDGE_CURVE('',#33767,#33768,#11207,.T.) ;
#41443=EDGE_CURVE('',#33768,#33766,#11208,.T.) ;
#41444=EDGE_CURVE('',#33767,#33769,#27787,.T.) ;
#41445=EDGE_CURVE('',#33769,#33770,#11209,.T.) ;
#41446=EDGE_CURVE('',#33770,#33768,#27788,.T.) ;
#41447=EDGE_CURVE('',#33769,#33771,#11210,.T.) ;
#41448=EDGE_CURVE('',#33771,#33772,#11211,.T.) ;
#41449=EDGE_CURVE('',#33772,#33770,#11212,.T.) ;
#41450=EDGE_CURVE('',#33771,#33773,#27789,.T.) ;
#41451=EDGE_CURVE('',#33773,#33774,#11213,.T.) ;
#41452=EDGE_CURVE('',#33774,#33772,#27790,.T.) ;
#41453=EDGE_CURVE('',#33773,#32159,#11214,.T.) ;
#41454=EDGE_CURVE('',#32159,#33775,#11215,.T.) ;
#41455=EDGE_CURVE('',#33775,#33774,#11216,.T.) ;
#41456=EDGE_CURVE('',#32160,#33776,#11217,.T.) ;
#41457=EDGE_CURVE('',#33776,#33775,#27791,.T.) ;
#41458=EDGE_CURVE('',#32160,#32169,#11218,.T.) ;
#41459=EDGE_CURVE('',#32123,#33776,#11219,.T.) ;
#41460=EDGE_CURVE('',#32170,#33777,#11220,.T.) ;
#41461=EDGE_CURVE('',#33777,#33778,#11221,.T.) ;
#41462=EDGE_CURVE('',#33778,#32124,#11222,.T.) ;
#41463=EDGE_CURVE('',#33777,#33779,#27792,.T.) ;
#41464=EDGE_CURVE('',#33779,#33780,#11223,.T.) ;
#41465=EDGE_CURVE('',#33780,#33778,#27793,.T.) ;
#41466=EDGE_CURVE('',#33779,#33781,#11224,.T.) ;
#41467=EDGE_CURVE('',#33781,#33782,#11225,.T.) ;
#41468=EDGE_CURVE('',#33782,#33780,#11226,.T.) ;
#41469=EDGE_CURVE('',#33781,#33783,#27794,.T.) ;
#41470=EDGE_CURVE('',#33783,#33784,#11227,.T.) ;
#41471=EDGE_CURVE('',#33784,#33782,#27795,.T.) ;
#41472=EDGE_CURVE('',#33783,#33785,#11228,.T.) ;
#41473=EDGE_CURVE('',#33785,#33786,#11229,.T.) ;
#41474=EDGE_CURVE('',#33786,#33784,#11230,.T.) ;
#41475=EDGE_CURVE('',#33785,#33787,#27796,.T.) ;
#41476=EDGE_CURVE('',#33787,#33788,#11231,.T.) ;
#41477=EDGE_CURVE('',#33788,#33786,#27797,.T.) ;
#41478=EDGE_CURVE('',#33787,#33789,#11232,.T.) ;
#41479=EDGE_CURVE('',#33789,#33790,#11233,.T.) ;
#41480=EDGE_CURVE('',#33790,#33788,#11234,.T.) ;
#41481=EDGE_CURVE('',#33789,#33791,#27798,.T.) ;
#41482=EDGE_CURVE('',#33791,#33792,#11235,.T.) ;
#41483=EDGE_CURVE('',#33792,#33790,#27799,.T.) ;
#41484=EDGE_CURVE('',#33791,#33793,#11236,.T.) ;
#41485=EDGE_CURVE('',#33793,#33794,#11237,.T.) ;
#41486=EDGE_CURVE('',#33794,#33792,#11238,.T.) ;
#41487=EDGE_CURVE('',#33793,#33795,#27800,.T.) ;
#41488=EDGE_CURVE('',#33795,#33796,#11239,.T.) ;
#41489=EDGE_CURVE('',#33796,#33794,#27801,.T.) ;
#41490=EDGE_CURVE('',#33795,#33797,#11240,.T.) ;
#41491=EDGE_CURVE('',#33797,#33798,#11241,.T.) ;
#41492=EDGE_CURVE('',#33798,#33796,#11242,.T.) ;
#41493=EDGE_CURVE('',#33797,#33799,#27802,.T.) ;
#41494=EDGE_CURVE('',#33799,#33800,#11243,.T.) ;
#41495=EDGE_CURVE('',#33800,#33798,#27803,.T.) ;
#41496=EDGE_CURVE('',#33799,#33801,#27804,.T.) ;
#41497=EDGE_CURVE('',#33801,#33802,#11244,.T.) ;
#41498=EDGE_CURVE('',#33802,#33800,#27805,.T.) ;
#41499=EDGE_CURVE('',#33801,#33803,#27806,.T.) ;
#41500=EDGE_CURVE('',#33803,#33804,#11245,.T.) ;
#41501=EDGE_CURVE('',#33804,#33802,#27807,.T.) ;
#41502=EDGE_CURVE('',#33803,#33805,#11246,.T.) ;
#41503=EDGE_CURVE('',#33805,#33806,#11247,.T.) ;
#41504=EDGE_CURVE('',#33806,#33804,#11248,.T.) ;
#41505=EDGE_CURVE('',#33805,#33807,#27808,.T.) ;
#41506=EDGE_CURVE('',#33807,#33808,#11249,.T.) ;
#41507=EDGE_CURVE('',#33808,#33806,#27809,.T.) ;
#41508=EDGE_CURVE('',#33807,#33809,#11250,.T.) ;
#41509=EDGE_CURVE('',#33809,#33810,#11251,.T.) ;
#41510=EDGE_CURVE('',#33810,#33808,#11252,.T.) ;
#41511=EDGE_CURVE('',#33809,#33811,#27810,.T.) ;
#41512=EDGE_CURVE('',#33811,#33812,#11253,.T.) ;
#41513=EDGE_CURVE('',#33812,#33810,#27811,.T.) ;
#41514=EDGE_CURVE('',#33811,#33763,#11254,.T.) ;
#41515=EDGE_CURVE('',#33764,#33812,#11255,.T.) ;
#41516=EDGE_CURVE('',#33813,#33814,#27812,.T.) ;
#41517=EDGE_CURVE('',#33814,#33815,#11256,.T.) ;
#41518=EDGE_CURVE('',#33815,#33816,#27813,.T.) ;
#41519=EDGE_CURVE('',#33816,#33817,#11257,.T.) ;
#41520=EDGE_CURVE('',#33817,#33818,#11258,.T.) ;
#41521=EDGE_CURVE('',#33818,#33819,#11259,.T.) ;
#41522=EDGE_CURVE('',#33819,#33820,#27814,.T.) ;
#41523=EDGE_CURVE('',#33820,#33821,#11260,.T.) ;
#41524=EDGE_CURVE('',#33821,#33822,#11261,.T.) ;
#41525=EDGE_CURVE('',#33822,#33823,#11262,.T.) ;
#41526=EDGE_CURVE('',#33823,#33824,#27815,.T.) ;
#41527=EDGE_CURVE('',#33824,#33825,#11263,.T.) ;
#41528=EDGE_CURVE('',#33825,#33826,#27816,.T.) ;
#41529=EDGE_CURVE('',#33826,#33827,#11264,.T.) ;
#41530=EDGE_CURVE('',#33827,#33828,#11265,.T.) ;
#41531=EDGE_CURVE('',#33828,#32161,#11266,.T.) ;
#41532=EDGE_CURVE('',#32161,#33829,#11267,.T.) ;
#41533=EDGE_CURVE('',#33829,#33813,#11268,.T.) ;
#41534=EDGE_CURVE('',#33830,#33831,#11269,.T.) ;
#41535=EDGE_CURVE('',#33830,#33832,#27817,.T.) ;
#41536=EDGE_CURVE('',#33832,#33833,#11270,.T.) ;
#41537=EDGE_CURVE('',#33833,#33834,#27818,.T.) ;
#41538=EDGE_CURVE('',#33834,#33835,#11271,.T.) ;
#41539=EDGE_CURVE('',#33835,#33836,#27819,.T.) ;
#41540=EDGE_CURVE('',#33836,#33837,#11272,.T.) ;
#41541=EDGE_CURVE('',#33837,#33831,#27820,.T.) ;
#41542=EDGE_CURVE('',#33838,#33839,#11273,.T.) ;
#41543=EDGE_CURVE('',#33838,#33840,#27821,.T.) ;
#41544=EDGE_CURVE('',#33840,#33841,#11274,.T.) ;
#41545=EDGE_CURVE('',#33841,#33842,#27822,.T.) ;
#41546=EDGE_CURVE('',#33842,#33843,#11275,.T.) ;
#41547=EDGE_CURVE('',#33843,#33844,#27823,.T.) ;
#41548=EDGE_CURVE('',#33844,#33845,#11276,.T.) ;
#41549=EDGE_CURVE('',#33845,#33839,#27824,.T.) ;
#41550=EDGE_CURVE('',#33846,#33847,#11277,.T.) ;
#41551=EDGE_CURVE('',#33846,#33848,#27825,.T.) ;
#41552=EDGE_CURVE('',#33848,#33849,#11278,.T.) ;
#41553=EDGE_CURVE('',#33849,#33850,#27826,.T.) ;
#41554=EDGE_CURVE('',#33850,#33851,#11279,.T.) ;
#41555=EDGE_CURVE('',#33851,#33852,#27827,.T.) ;
#41556=EDGE_CURVE('',#33852,#33853,#11280,.T.) ;
#41557=EDGE_CURVE('',#33853,#33847,#27828,.T.) ;
#41558=EDGE_CURVE('',#33854,#33855,#11281,.T.) ;
#41559=EDGE_CURVE('',#33854,#33856,#27829,.T.) ;
#41560=EDGE_CURVE('',#33856,#33857,#11282,.T.) ;
#41561=EDGE_CURVE('',#33857,#33858,#27830,.T.) ;
#41562=EDGE_CURVE('',#33858,#33859,#11283,.T.) ;
#41563=EDGE_CURVE('',#33859,#33860,#27831,.T.) ;
#41564=EDGE_CURVE('',#33860,#33861,#11284,.T.) ;
#41565=EDGE_CURVE('',#33861,#33855,#27832,.T.) ;
#41566=EDGE_CURVE('',#33862,#33863,#11285,.T.) ;
#41567=EDGE_CURVE('',#33862,#33864,#27833,.T.) ;
#41568=EDGE_CURVE('',#33864,#33865,#11286,.T.) ;
#41569=EDGE_CURVE('',#33865,#33866,#27834,.T.) ;
#41570=EDGE_CURVE('',#33866,#33867,#11287,.T.) ;
#41571=EDGE_CURVE('',#33867,#33868,#27835,.T.) ;
#41572=EDGE_CURVE('',#33868,#33869,#11288,.T.) ;
#41573=EDGE_CURVE('',#33869,#33863,#27836,.T.) ;
#41574=EDGE_CURVE('',#33870,#33871,#11289,.T.) ;
#41575=EDGE_CURVE('',#33870,#33872,#27837,.T.) ;
#41576=EDGE_CURVE('',#33872,#33873,#11290,.T.) ;
#41577=EDGE_CURVE('',#33873,#33874,#27838,.T.) ;
#41578=EDGE_CURVE('',#33874,#33875,#11291,.T.) ;
#41579=EDGE_CURVE('',#33875,#33876,#27839,.T.) ;
#41580=EDGE_CURVE('',#33876,#33877,#11292,.T.) ;
#41581=EDGE_CURVE('',#33877,#33871,#27840,.T.) ;
#41582=EDGE_CURVE('',#33878,#33879,#11293,.T.) ;
#41583=EDGE_CURVE('',#33878,#33880,#27841,.T.) ;
#41584=EDGE_CURVE('',#33880,#33881,#11294,.T.) ;
#41585=EDGE_CURVE('',#33881,#33882,#27842,.T.) ;
#41586=EDGE_CURVE('',#33882,#33883,#11295,.T.) ;
#41587=EDGE_CURVE('',#33883,#33884,#27843,.T.) ;
#41588=EDGE_CURVE('',#33884,#33885,#11296,.T.) ;
#41589=EDGE_CURVE('',#33885,#33879,#27844,.T.) ;
#41590=EDGE_CURVE('',#33886,#33887,#11297,.T.) ;
#41591=EDGE_CURVE('',#33886,#33888,#27845,.T.) ;
#41592=EDGE_CURVE('',#33888,#33889,#11298,.T.) ;
#41593=EDGE_CURVE('',#33889,#33890,#27846,.T.) ;
#41594=EDGE_CURVE('',#33890,#33891,#11299,.T.) ;
#41595=EDGE_CURVE('',#33891,#33892,#27847,.T.) ;
#41596=EDGE_CURVE('',#33892,#33893,#11300,.T.) ;
#41597=EDGE_CURVE('',#33893,#33887,#27848,.T.) ;
#41598=EDGE_CURVE('',#33894,#33895,#11301,.T.) ;
#41599=EDGE_CURVE('',#33894,#33896,#27849,.T.) ;
#41600=EDGE_CURVE('',#33896,#33897,#11302,.T.) ;
#41601=EDGE_CURVE('',#33897,#33898,#27850,.T.) ;
#41602=EDGE_CURVE('',#33898,#33899,#11303,.T.) ;
#41603=EDGE_CURVE('',#33899,#33900,#27851,.T.) ;
#41604=EDGE_CURVE('',#33900,#33901,#11304,.T.) ;
#41605=EDGE_CURVE('',#33901,#33895,#27852,.T.) ;
#41606=EDGE_CURVE('',#33077,#33064,#27853,.T.) ;
#41607=EDGE_CURVE('',#33055,#33076,#27854,.T.) ;
#41608=EDGE_CURVE('',#33078,#33071,#27855,.T.) ;
#41609=EDGE_CURVE('',#33072,#33077,#27856,.T.) ;
#41610=EDGE_CURVE('',#33078,#33902,#27857,.T.) ;
#41611=EDGE_CURVE('',#33902,#33071,#27858,.T.) ;
#41612=EDGE_CURVE('',#33055,#33081,#27859,.T.) ;
#41613=EDGE_CURVE('',#33081,#33076,#27860,.T.) ;
#41614=EDGE_CURVE('',#33072,#33063,#27861,.T.) ;
#41615=EDGE_CURVE('',#32162,#33074,#27862,.T.) ;
#41616=EDGE_CURVE('',#32163,#33903,#303,.T.) ;
#41617=EDGE_CURVE('',#33902,#33903,#11305,.T.) ;
#41618=EDGE_CURVE('',#33904,#33902,#304,.T.) ;
#41619=EDGE_CURVE('',#33904,#33905,#305,.T.) ;
#41620=EDGE_CURVE('',#32289,#33905,#11306,.T.) ;
#41621=EDGE_CURVE('',#33075,#32288,#27863,.T.) ;
#41622=EDGE_CURVE('',#33082,#33075,#27864,.T.) ;
#41623=EDGE_CURVE('',#33056,#33080,#27865,.T.) ;
#41624=EDGE_CURVE('',#33073,#33062,#27866,.T.) ;
#41625=EDGE_CURVE('',#33074,#32164,#27867,.T.) ;
#41626=EDGE_CURVE('',#33069,#33073,#27868,.T.) ;
#41627=EDGE_CURVE('',#33082,#32297,#27869,.T.) ;
#41628=EDGE_CURVE('',#33056,#32384,#27870,.T.) ;
#41629=EDGE_CURVE('',#32383,#33080,#27871,.T.) ;
#41630=EDGE_CURVE('',#33069,#33061,#27872,.T.) ;
#41631=EDGE_CURVE('',#33079,#32296,#27873,.T.) ;
#41632=EDGE_CURVE('',#32385,#33079,#27874,.T.) ;
#41633=EDGE_CURVE('',#33906,#32384,#11307,.T.) ;
#41634=EDGE_CURVE('',#33057,#33906,#27875,.T.) ;
#41635=EDGE_CURVE('',#33070,#33060,#27876,.T.) ;
#41636=EDGE_CURVE('',#32165,#33065,#27877,.T.) ;
#41637=EDGE_CURVE('',#33066,#33070,#27878,.T.) ;
#41638=EDGE_CURVE('',#32292,#33065,#27879,.T.) ;
#41639=EDGE_CURVE('',#32385,#32296,#27880,.T.) ;
#41640=EDGE_CURVE('',#32390,#32387,#27881,.T.) ;
#41641=EDGE_CURVE('',#32387,#32388,#27882,.T.) ;
#41642=EDGE_CURVE('',#33906,#32529,#27883,.T.) ;
#41643=EDGE_CURVE('',#33907,#33906,#27884,.T.) ;
#41644=EDGE_CURVE('',#33057,#33907,#27885,.T.) ;
#41645=EDGE_CURVE('',#33066,#33060,#27886,.T.) ;
#41646=EDGE_CURVE('',#32293,#33068,#27887,.T.) ;
#41647=EDGE_CURVE('',#32386,#32295,#27888,.T.) ;
#41648=EDGE_CURVE('',#32460,#32386,#27889,.T.) ;
#41649=EDGE_CURVE('',#33907,#32528,#27890,.T.) ;
#41650=EDGE_CURVE('',#33908,#33907,#11308,.T.) ;
#41651=EDGE_CURVE('',#33058,#33908,#27891,.T.) ;
#41652=EDGE_CURVE('',#33067,#33059,#27892,.T.) ;
#41653=EDGE_CURVE('',#33068,#32382,#27893,.T.) ;
#41654=EDGE_CURVE('',#32379,#33067,#27894,.T.) ;
#41655=EDGE_CURVE('',#32293,#32382,#27895,.T.) ;
#41656=EDGE_CURVE('',#32461,#32295,#27896,.T.) ;
#41657=EDGE_CURVE('',#33908,#32527,#27897,.T.) ;
#41658=EDGE_CURVE('',#33909,#33908,#27898,.T.) ;
#41659=EDGE_CURVE('',#33058,#33909,#27899,.T.) ;
#41660=EDGE_CURVE('',#32378,#33059,#27900,.T.) ;
#41661=EDGE_CURVE('',#32294,#32381,#27901,.T.) ;
#41662=EDGE_CURVE('',#32462,#32294,#27902,.T.) ;
#41663=EDGE_CURVE('',#33909,#32526,#27903,.T.) ;
#41664=EDGE_CURVE('',#32378,#33909,#11309,.T.) ;
#41665=EDGE_CURVE('',#32463,#32381,#27904,.T.) ;
#41666=EDGE_CURVE('',#32380,#32393,#27905,.T.) ;
#41667=EDGE_CURVE('',#32395,#32380,#27906,.T.) ;
#41668=EDGE_CURVE('',#33789,#33822,#27907,.T.) ;
#41669=EDGE_CURVE('',#33823,#33787,#27908,.T.) ;
#41670=EDGE_CURVE('',#33824,#33785,#27909,.T.) ;
#41671=EDGE_CURVE('',#33791,#33822,#27910,.T.) ;
#41672=EDGE_CURVE('',#33825,#33783,#27911,.T.) ;
#41673=EDGE_CURVE('',#33793,#33821,#27912,.T.) ;
#41674=EDGE_CURVE('',#33826,#33781,#27913,.T.) ;
#41675=EDGE_CURVE('',#33795,#33821,#27914,.T.) ;
#41676=EDGE_CURVE('',#33827,#33779,#27915,.T.) ;
#41677=EDGE_CURVE('',#33797,#33820,#27916,.T.) ;
#41678=EDGE_CURVE('',#33827,#33777,#27917,.T.) ;
#41679=EDGE_CURVE('',#33799,#33820,#27918,.T.) ;
#41680=EDGE_CURVE('',#33828,#32170,#27919,.T.) ;
#41681=EDGE_CURVE('',#33801,#33819,#27920,.T.) ;
#41682=EDGE_CURVE('',#33828,#32169,#27921,.T.) ;
#41683=EDGE_CURVE('',#33803,#33819,#27922,.T.) ;
#41684=EDGE_CURVE('',#33805,#33818,#27923,.T.) ;
#41685=EDGE_CURVE('',#33807,#33818,#27924,.T.) ;
#41686=EDGE_CURVE('',#33829,#33773,#27925,.T.) ;
#41687=EDGE_CURVE('',#33809,#33817,#27926,.T.) ;
#41688=EDGE_CURVE('',#33829,#33771,#27927,.T.) ;
#41689=EDGE_CURVE('',#33811,#33817,#27928,.T.) ;
#41690=EDGE_CURVE('',#33813,#33769,#27929,.T.) ;
#41691=EDGE_CURVE('',#33763,#33816,#27930,.T.) ;
#41692=EDGE_CURVE('',#33814,#33767,#27931,.T.) ;
#41693=EDGE_CURVE('',#33765,#33815,#27932,.T.) ;
#41694=EDGE_CURVE('',#33248,#32570,#27933,.T.) ;
#41695=EDGE_CURVE('',#32571,#33250,#27934,.T.) ;
#41696=EDGE_CURVE('',#33246,#32570,#27935,.T.) ;
#41697=EDGE_CURVE('',#32571,#33252,#27936,.T.) ;
#41698=EDGE_CURVE('',#33244,#32569,#27937,.T.) ;
#41699=EDGE_CURVE('',#32572,#33254,#27938,.T.) ;
#41700=EDGE_CURVE('',#33242,#32568,#27939,.T.) ;
#41701=EDGE_CURVE('',#32573,#33256,#27940,.T.) ;
#41702=EDGE_CURVE('',#32574,#33258,#27941,.T.) ;
#41703=EDGE_CURVE('',#32575,#33260,#27942,.T.) ;
#41704=EDGE_CURVE('',#33240,#32567,#27943,.T.) ;
#41705=EDGE_CURVE('',#32576,#33262,#27944,.T.) ;
#41706=EDGE_CURVE('',#33239,#32566,#27945,.T.) ;
#41707=EDGE_CURVE('',#32577,#33264,#27946,.T.) ;
#41708=EDGE_CURVE('',#33238,#32565,#27947,.T.) ;
#41709=EDGE_CURVE('',#32578,#33266,#27948,.T.) ;
#41710=EDGE_CURVE('',#33236,#32564,#27949,.T.) ;
#41711=EDGE_CURVE('',#32579,#33268,#27950,.T.) ;
#41712=EDGE_CURVE('',#33234,#32563,#27951,.T.) ;
#41713=EDGE_CURVE('',#32580,#33270,#27952,.T.) ;
#41714=EDGE_CURVE('',#33232,#32563,#27953,.T.) ;
#41715=EDGE_CURVE('',#32581,#33272,#27954,.T.) ;
#41716=EDGE_CURVE('',#33230,#32562,#27955,.T.) ;
#41717=EDGE_CURVE('',#32560,#33274,#27956,.T.) ;
#41718=EDGE_CURVE('',#33228,#32562,#27957,.T.) ;
#41719=EDGE_CURVE('',#32561,#33276,#27958,.T.) ;
#41720=EDGE_CURVE('',#33315,#32592,#27959,.T.) ;
#41721=EDGE_CURVE('',#32593,#33317,#27960,.T.) ;
#41722=EDGE_CURVE('',#33313,#32592,#27961,.T.) ;
#41723=EDGE_CURVE('',#32593,#33319,#27962,.T.) ;
#41724=EDGE_CURVE('',#33311,#32591,#27963,.T.) ;
#41725=EDGE_CURVE('',#32594,#33321,#27964,.T.) ;
#41726=EDGE_CURVE('',#33309,#32590,#27965,.T.) ;
#41727=EDGE_CURVE('',#32595,#33323,#27966,.T.) ;
#41728=EDGE_CURVE('',#32596,#33325,#27967,.T.) ;
#41729=EDGE_CURVE('',#32597,#33327,#27968,.T.) ;
#41730=EDGE_CURVE('',#33307,#32589,#27969,.T.) ;
#41731=EDGE_CURVE('',#32598,#33329,#27970,.T.) ;
#41732=EDGE_CURVE('',#33306,#32588,#27971,.T.) ;
#41733=EDGE_CURVE('',#32599,#33331,#27972,.T.) ;
#41734=EDGE_CURVE('',#33305,#32587,#27973,.T.) ;
#41735=EDGE_CURVE('',#32600,#33333,#27974,.T.) ;
#41736=EDGE_CURVE('',#33303,#32586,#27975,.T.) ;
#41737=EDGE_CURVE('',#32601,#33335,#27976,.T.) ;
#41738=EDGE_CURVE('',#33301,#32585,#27977,.T.) ;
#41739=EDGE_CURVE('',#32602,#33337,#27978,.T.) ;
#41740=EDGE_CURVE('',#33299,#32585,#27979,.T.) ;
#41741=EDGE_CURVE('',#32603,#33339,#27980,.T.) ;
#41742=EDGE_CURVE('',#33297,#32584,#27981,.T.) ;
#41743=EDGE_CURVE('',#32582,#33341,#27982,.T.) ;
#41744=EDGE_CURVE('',#33295,#32584,#27983,.T.) ;
#41745=EDGE_CURVE('',#32583,#33343,#27984,.T.) ;
#41746=EDGE_CURVE('',#33382,#32614,#27985,.T.) ;
#41747=EDGE_CURVE('',#32615,#33384,#27986,.T.) ;
#41748=EDGE_CURVE('',#33380,#32614,#27987,.T.) ;
#41749=EDGE_CURVE('',#32615,#33386,#27988,.T.) ;
#41750=EDGE_CURVE('',#33378,#32613,#27989,.T.) ;
#41751=EDGE_CURVE('',#32616,#33388,#27990,.T.) ;
#41752=EDGE_CURVE('',#33376,#32612,#27991,.T.) ;
#41753=EDGE_CURVE('',#32617,#33390,#27992,.T.) ;
#41754=EDGE_CURVE('',#32618,#33392,#27993,.T.) ;
#41755=EDGE_CURVE('',#32619,#33394,#27994,.T.) ;
#41756=EDGE_CURVE('',#33374,#32611,#27995,.T.) ;
#41757=EDGE_CURVE('',#32620,#33396,#27996,.T.) ;
#41758=EDGE_CURVE('',#33373,#32610,#27997,.T.) ;
#41759=EDGE_CURVE('',#32621,#33398,#27998,.T.) ;
#41760=EDGE_CURVE('',#33372,#32609,#27999,.T.) ;
#41761=EDGE_CURVE('',#32622,#33400,#28000,.T.) ;
#41762=EDGE_CURVE('',#33370,#32608,#28001,.T.) ;
#41763=EDGE_CURVE('',#32623,#33402,#28002,.T.) ;
#41764=EDGE_CURVE('',#33368,#32607,#28003,.T.) ;
#41765=EDGE_CURVE('',#32624,#33404,#28004,.T.) ;
#41766=EDGE_CURVE('',#33366,#32607,#28005,.T.) ;
#41767=EDGE_CURVE('',#32625,#33406,#28006,.T.) ;
#41768=EDGE_CURVE('',#33364,#32606,#28007,.T.) ;
#41769=EDGE_CURVE('',#32604,#33408,#28008,.T.) ;
#41770=EDGE_CURVE('',#33362,#32606,#28009,.T.) ;
#41771=EDGE_CURVE('',#32605,#33410,#28010,.T.) ;
#41772=EDGE_CURVE('',#33449,#32636,#28011,.T.) ;
#41773=EDGE_CURVE('',#32637,#33451,#28012,.T.) ;
#41774=EDGE_CURVE('',#33447,#32636,#28013,.T.) ;
#41775=EDGE_CURVE('',#32637,#33453,#28014,.T.) ;
#41776=EDGE_CURVE('',#33445,#32635,#28015,.T.) ;
#41777=EDGE_CURVE('',#32638,#33455,#28016,.T.) ;
#41778=EDGE_CURVE('',#33443,#32634,#28017,.T.) ;
#41779=EDGE_CURVE('',#32639,#33457,#28018,.T.) ;
#41780=EDGE_CURVE('',#32640,#33459,#28019,.T.) ;
#41781=EDGE_CURVE('',#32641,#33461,#28020,.T.) ;
#41782=EDGE_CURVE('',#33441,#32633,#28021,.T.) ;
#41783=EDGE_CURVE('',#32642,#33463,#28022,.T.) ;
#41784=EDGE_CURVE('',#33440,#32632,#28023,.T.) ;
#41785=EDGE_CURVE('',#32643,#33465,#28024,.T.) ;
#41786=EDGE_CURVE('',#33439,#32631,#28025,.T.) ;
#41787=EDGE_CURVE('',#32644,#33467,#28026,.T.) ;
#41788=EDGE_CURVE('',#33437,#32630,#28027,.T.) ;
#41789=EDGE_CURVE('',#32645,#33469,#28028,.T.) ;
#41790=EDGE_CURVE('',#33435,#32629,#28029,.T.) ;
#41791=EDGE_CURVE('',#32646,#33471,#28030,.T.) ;
#41792=EDGE_CURVE('',#33433,#32629,#28031,.T.) ;
#41793=EDGE_CURVE('',#32647,#33473,#28032,.T.) ;
#41794=EDGE_CURVE('',#33431,#32628,#28033,.T.) ;
#41795=EDGE_CURVE('',#32626,#33475,#28034,.T.) ;
#41796=EDGE_CURVE('',#33429,#32628,#28035,.T.) ;
#41797=EDGE_CURVE('',#32627,#33477,#28036,.T.) ;
#41798=EDGE_CURVE('',#33516,#32658,#28037,.T.) ;
#41799=EDGE_CURVE('',#32659,#33518,#28038,.T.) ;
#41800=EDGE_CURVE('',#33514,#32658,#28039,.T.) ;
#41801=EDGE_CURVE('',#32659,#33520,#28040,.T.) ;
#41802=EDGE_CURVE('',#33512,#32657,#28041,.T.) ;
#41803=EDGE_CURVE('',#32660,#33522,#28042,.T.) ;
#41804=EDGE_CURVE('',#33510,#32656,#28043,.T.) ;
#41805=EDGE_CURVE('',#32661,#33524,#28044,.T.) ;
#41806=EDGE_CURVE('',#32662,#33526,#28045,.T.) ;
#41807=EDGE_CURVE('',#32663,#33528,#28046,.T.) ;
#41808=EDGE_CURVE('',#33508,#32655,#28047,.T.) ;
#41809=EDGE_CURVE('',#32664,#33530,#28048,.T.) ;
#41810=EDGE_CURVE('',#33507,#32654,#28049,.T.) ;
#41811=EDGE_CURVE('',#32665,#33532,#28050,.T.) ;
#41812=EDGE_CURVE('',#33506,#32653,#28051,.T.) ;
#41813=EDGE_CURVE('',#32666,#33534,#28052,.T.) ;
#41814=EDGE_CURVE('',#33504,#32652,#28053,.T.) ;
#41815=EDGE_CURVE('',#32667,#33536,#28054,.T.) ;
#41816=EDGE_CURVE('',#33502,#32651,#28055,.T.) ;
#41817=EDGE_CURVE('',#32668,#33538,#28056,.T.) ;
#41818=EDGE_CURVE('',#33500,#32651,#28057,.T.) ;
#41819=EDGE_CURVE('',#32669,#33540,#28058,.T.) ;
#41820=EDGE_CURVE('',#33498,#32650,#28059,.T.) ;
#41821=EDGE_CURVE('',#32648,#33542,#28060,.T.) ;
#41822=EDGE_CURVE('',#33496,#32650,#28061,.T.) ;
#41823=EDGE_CURVE('',#32649,#33544,#28062,.T.) ;
#41824=EDGE_CURVE('',#33583,#32680,#28063,.T.) ;
#41825=EDGE_CURVE('',#32681,#33585,#28064,.T.) ;
#41826=EDGE_CURVE('',#33581,#32680,#28065,.T.) ;
#41827=EDGE_CURVE('',#32681,#33587,#28066,.T.) ;
#41828=EDGE_CURVE('',#33579,#32679,#28067,.T.) ;
#41829=EDGE_CURVE('',#32682,#33589,#28068,.T.) ;
#41830=EDGE_CURVE('',#33577,#32678,#28069,.T.) ;
#41831=EDGE_CURVE('',#32683,#33591,#28070,.T.) ;
#41832=EDGE_CURVE('',#32684,#33593,#28071,.T.) ;
#41833=EDGE_CURVE('',#32685,#33595,#28072,.T.) ;
#41834=EDGE_CURVE('',#33575,#32677,#28073,.T.) ;
#41835=EDGE_CURVE('',#32686,#33597,#28074,.T.) ;
#41836=EDGE_CURVE('',#33574,#32676,#28075,.T.) ;
#41837=EDGE_CURVE('',#32687,#33599,#28076,.T.) ;
#41838=EDGE_CURVE('',#33573,#32675,#28077,.T.) ;
#41839=EDGE_CURVE('',#32688,#33601,#28078,.T.) ;
#41840=EDGE_CURVE('',#33571,#32674,#28079,.T.) ;
#41841=EDGE_CURVE('',#32689,#33603,#28080,.T.) ;
#41842=EDGE_CURVE('',#33569,#32673,#28081,.T.) ;
#41843=EDGE_CURVE('',#32690,#33605,#28082,.T.) ;
#41844=EDGE_CURVE('',#33567,#32673,#28083,.T.) ;
#41845=EDGE_CURVE('',#32691,#33607,#28084,.T.) ;
#41846=EDGE_CURVE('',#33565,#32672,#28085,.T.) ;
#41847=EDGE_CURVE('',#32670,#33609,#28086,.T.) ;
#41848=EDGE_CURVE('',#33563,#32672,#28087,.T.) ;
#41849=EDGE_CURVE('',#32671,#33611,#28088,.T.) ;
#41850=EDGE_CURVE('',#33650,#32702,#28089,.T.) ;
#41851=EDGE_CURVE('',#32703,#33652,#28090,.T.) ;
#41852=EDGE_CURVE('',#33648,#32702,#28091,.T.) ;
#41853=EDGE_CURVE('',#32703,#33654,#28092,.T.) ;
#41854=EDGE_CURVE('',#33646,#32701,#28093,.T.) ;
#41855=EDGE_CURVE('',#32704,#33656,#28094,.T.) ;
#41856=EDGE_CURVE('',#33644,#32700,#28095,.T.) ;
#41857=EDGE_CURVE('',#32705,#33658,#28096,.T.) ;
#41858=EDGE_CURVE('',#32706,#33660,#28097,.T.) ;
#41859=EDGE_CURVE('',#32707,#33662,#28098,.T.) ;
#41860=EDGE_CURVE('',#33642,#32699,#28099,.T.) ;
#41861=EDGE_CURVE('',#32708,#33664,#28100,.T.) ;
#41862=EDGE_CURVE('',#33641,#32698,#28101,.T.) ;
#41863=EDGE_CURVE('',#32709,#33666,#28102,.T.) ;
#41864=EDGE_CURVE('',#33640,#32697,#28103,.T.) ;
#41865=EDGE_CURVE('',#32710,#33668,#28104,.T.) ;
#41866=EDGE_CURVE('',#33638,#32696,#28105,.T.) ;
#41867=EDGE_CURVE('',#32711,#33670,#28106,.T.) ;
#41868=EDGE_CURVE('',#33636,#32695,#28107,.T.) ;
#41869=EDGE_CURVE('',#32712,#33672,#28108,.T.) ;
#41870=EDGE_CURVE('',#33634,#32695,#28109,.T.) ;
#41871=EDGE_CURVE('',#32713,#33674,#28110,.T.) ;
#41872=EDGE_CURVE('',#33632,#32694,#28111,.T.) ;
#41873=EDGE_CURVE('',#32692,#33676,#28112,.T.) ;
#41874=EDGE_CURVE('',#33630,#32694,#28113,.T.) ;
#41875=EDGE_CURVE('',#32693,#33678,#28114,.T.) ;
#41876=EDGE_CURVE('',#33717,#32724,#28115,.T.) ;
#41877=EDGE_CURVE('',#32725,#33719,#28116,.T.) ;
#41878=EDGE_CURVE('',#33715,#32724,#28117,.T.) ;
#41879=EDGE_CURVE('',#32725,#33721,#28118,.T.) ;
#41880=EDGE_CURVE('',#33713,#32723,#28119,.T.) ;
#41881=EDGE_CURVE('',#32726,#33723,#28120,.T.) ;
#41882=EDGE_CURVE('',#33711,#32722,#28121,.T.) ;
#41883=EDGE_CURVE('',#32727,#33725,#28122,.T.) ;
#41884=EDGE_CURVE('',#32728,#33727,#28123,.T.) ;
#41885=EDGE_CURVE('',#32729,#33729,#28124,.T.) ;
#41886=EDGE_CURVE('',#33709,#32721,#28125,.T.) ;
#41887=EDGE_CURVE('',#32730,#33731,#28126,.T.) ;
#41888=EDGE_CURVE('',#33708,#32720,#28127,.T.) ;
#41889=EDGE_CURVE('',#32731,#33733,#28128,.T.) ;
#41890=EDGE_CURVE('',#33707,#32719,#28129,.T.) ;
#41891=EDGE_CURVE('',#32732,#33735,#28130,.T.) ;
#41892=EDGE_CURVE('',#33705,#32718,#28131,.T.) ;
#41893=EDGE_CURVE('',#32733,#33737,#28132,.T.) ;
#41894=EDGE_CURVE('',#33703,#32717,#28133,.T.) ;
#41895=EDGE_CURVE('',#32734,#33739,#28134,.T.) ;
#41896=EDGE_CURVE('',#33701,#32717,#28135,.T.) ;
#41897=EDGE_CURVE('',#32735,#33741,#28136,.T.) ;
#41898=EDGE_CURVE('',#33699,#32716,#28137,.T.) ;
#41899=EDGE_CURVE('',#32714,#33743,#28138,.T.) ;
#41900=EDGE_CURVE('',#33697,#32716,#28139,.T.) ;
#41901=EDGE_CURVE('',#32715,#33745,#28140,.T.) ;
#41902=EDGE_CURVE('',#33784,#32746,#28141,.T.) ;
#41903=EDGE_CURVE('',#32747,#33786,#28142,.T.) ;
#41904=EDGE_CURVE('',#33782,#32746,#28143,.T.) ;
#41905=EDGE_CURVE('',#32747,#33788,#28144,.T.) ;
#41906=EDGE_CURVE('',#33780,#32745,#28145,.T.) ;
#41907=EDGE_CURVE('',#32748,#33790,#28146,.T.) ;
#41908=EDGE_CURVE('',#33778,#32744,#28147,.T.) ;
#41909=EDGE_CURVE('',#32749,#33792,#28148,.T.) ;
#41910=EDGE_CURVE('',#32750,#33794,#28149,.T.) ;
#41911=EDGE_CURVE('',#32751,#33796,#28150,.T.) ;
#41912=EDGE_CURVE('',#33776,#32743,#28151,.T.) ;
#41913=EDGE_CURVE('',#32752,#33798,#28152,.T.) ;
#41914=EDGE_CURVE('',#33775,#32742,#28153,.T.) ;
#41915=EDGE_CURVE('',#32753,#33800,#28154,.T.) ;
#41916=EDGE_CURVE('',#33774,#32741,#28155,.T.) ;
#41917=EDGE_CURVE('',#32754,#33802,#28156,.T.) ;
#41918=EDGE_CURVE('',#33772,#32740,#28157,.T.) ;
#41919=EDGE_CURVE('',#32755,#33804,#28158,.T.) ;
#41920=EDGE_CURVE('',#33770,#32739,#28159,.T.) ;
#41921=EDGE_CURVE('',#32756,#33806,#28160,.T.) ;
#41922=EDGE_CURVE('',#33768,#32739,#28161,.T.) ;
#41923=EDGE_CURVE('',#32757,#33808,#28162,.T.) ;
#41924=EDGE_CURVE('',#33766,#32738,#28163,.T.) ;
#41925=EDGE_CURVE('',#32736,#33810,#28164,.T.) ;
#41926=EDGE_CURVE('',#33764,#32738,#28165,.T.) ;
#41927=EDGE_CURVE('',#32737,#33812,#28166,.T.) ;
#41928=EDGE_CURVE('',#33095,#33054,#28167,.T.) ;
#41929=EDGE_CURVE('',#33045,#33094,#28168,.T.) ;
#41930=EDGE_CURVE('',#33096,#33089,#28169,.T.) ;
#41931=EDGE_CURVE('',#33090,#33095,#28170,.T.) ;
#41932=EDGE_CURVE('',#33096,#33910,#28171,.T.) ;
#41933=EDGE_CURVE('',#33910,#33089,#28172,.T.) ;
#41934=EDGE_CURVE('',#33045,#33099,#28173,.T.) ;
#41935=EDGE_CURVE('',#33099,#33094,#28174,.T.) ;
#41936=EDGE_CURVE('',#33090,#33053,#28175,.T.) ;
#41937=EDGE_CURVE('',#32111,#33092,#28176,.T.) ;
#41938=EDGE_CURVE('',#32112,#33911,#306,.T.) ;
#41939=EDGE_CURVE('',#33910,#33911,#11310,.T.) ;
#41940=EDGE_CURVE('',#33912,#33910,#307,.T.) ;
#41941=EDGE_CURVE('',#33912,#33913,#308,.T.) ;
#41942=EDGE_CURVE('',#32279,#33913,#11311,.T.) ;
#41943=EDGE_CURVE('',#33093,#32278,#28177,.T.) ;
#41944=EDGE_CURVE('',#33100,#33093,#28178,.T.) ;
#41945=EDGE_CURVE('',#33046,#33098,#28179,.T.) ;
#41946=EDGE_CURVE('',#33091,#33052,#28180,.T.) ;
#41947=EDGE_CURVE('',#33092,#32113,#28181,.T.) ;
#41948=EDGE_CURVE('',#33087,#33091,#28182,.T.) ;
#41949=EDGE_CURVE('',#33100,#32287,#28183,.T.) ;
#41950=EDGE_CURVE('',#33046,#32374,#28184,.T.) ;
#41951=EDGE_CURVE('',#32373,#33098,#28185,.T.) ;
#41952=EDGE_CURVE('',#33087,#33051,#28186,.T.) ;
#41953=EDGE_CURVE('',#33097,#32286,#28187,.T.) ;
#41954=EDGE_CURVE('',#32375,#33097,#28188,.T.) ;
#41955=EDGE_CURVE('',#33914,#32374,#11312,.T.) ;
#41956=EDGE_CURVE('',#33047,#33914,#28189,.T.) ;
#41957=EDGE_CURVE('',#33088,#33050,#28190,.T.) ;
#41958=EDGE_CURVE('',#32114,#33083,#28191,.T.) ;
#41959=EDGE_CURVE('',#33084,#33088,#28192,.T.) ;
#41960=EDGE_CURVE('',#32282,#33083,#28193,.T.) ;
#41961=EDGE_CURVE('',#32375,#32286,#28194,.T.) ;
#41962=EDGE_CURVE('',#32394,#32377,#28195,.T.) ;
#41963=EDGE_CURVE('',#32377,#32392,#28196,.T.) ;
#41964=EDGE_CURVE('',#33914,#32525,#28197,.T.) ;
#41965=EDGE_CURVE('',#33915,#33914,#28198,.T.) ;
#41966=EDGE_CURVE('',#33047,#33915,#28199,.T.) ;
#41967=EDGE_CURVE('',#33084,#33050,#28200,.T.) ;
#41968=EDGE_CURVE('',#32283,#33086,#28201,.T.) ;
#41969=EDGE_CURVE('',#32376,#32285,#28202,.T.) ;
#41970=EDGE_CURVE('',#32464,#32376,#28203,.T.) ;
#41971=EDGE_CURVE('',#33915,#32524,#28204,.T.) ;
#41972=EDGE_CURVE('',#33916,#33915,#11313,.T.) ;
#41973=EDGE_CURVE('',#33048,#33916,#28205,.T.) ;
#41974=EDGE_CURVE('',#33085,#33049,#28206,.T.) ;
#41975=EDGE_CURVE('',#33086,#32372,#28207,.T.) ;
#41976=EDGE_CURVE('',#32369,#33085,#28208,.T.) ;
#41977=EDGE_CURVE('',#32283,#32372,#28209,.T.) ;
#41978=EDGE_CURVE('',#32465,#32285,#28210,.T.) ;
#41979=EDGE_CURVE('',#33916,#32523,#28211,.T.) ;
#41980=EDGE_CURVE('',#33917,#33916,#28212,.T.) ;
#41981=EDGE_CURVE('',#33048,#33917,#28213,.T.) ;
#41982=EDGE_CURVE('',#32368,#33049,#28214,.T.) ;
#41983=EDGE_CURVE('',#32284,#32371,#28215,.T.) ;
#41984=EDGE_CURVE('',#32466,#32284,#28216,.T.) ;
#41985=EDGE_CURVE('',#33917,#32522,#28217,.T.) ;
#41986=EDGE_CURVE('',#32368,#33917,#11314,.T.) ;
#41987=EDGE_CURVE('',#32467,#32371,#28218,.T.) ;
#41988=EDGE_CURVE('',#32370,#32397,#28219,.T.) ;
#41989=EDGE_CURVE('',#32399,#32370,#28220,.T.) ;
#41990=EDGE_CURVE('',#33722,#33755,#28221,.T.) ;
#41991=EDGE_CURVE('',#33756,#33720,#28222,.T.) ;
#41992=EDGE_CURVE('',#33757,#33718,#28223,.T.) ;
#41993=EDGE_CURVE('',#33724,#33755,#28224,.T.) ;
#41994=EDGE_CURVE('',#33758,#33716,#28225,.T.) ;
#41995=EDGE_CURVE('',#33726,#33754,#28226,.T.) ;
#41996=EDGE_CURVE('',#33759,#33714,#28227,.T.) ;
#41997=EDGE_CURVE('',#33728,#33754,#28228,.T.) ;
#41998=EDGE_CURVE('',#33760,#33712,#28229,.T.) ;
#41999=EDGE_CURVE('',#33730,#33753,#28230,.T.) ;
#42000=EDGE_CURVE('',#33760,#33710,#28231,.T.) ;
#42001=EDGE_CURVE('',#33732,#33753,#28232,.T.) ;
#42002=EDGE_CURVE('',#33761,#32172,#28233,.T.) ;
#42003=EDGE_CURVE('',#33734,#33752,#28234,.T.) ;
#42004=EDGE_CURVE('',#33761,#32171,#28235,.T.) ;
#42005=EDGE_CURVE('',#33736,#33752,#28236,.T.) ;
#42006=EDGE_CURVE('',#33738,#33751,#28237,.T.) ;
#42007=EDGE_CURVE('',#33740,#33751,#28238,.T.) ;
#42008=EDGE_CURVE('',#33762,#33706,#28239,.T.) ;
#42009=EDGE_CURVE('',#33742,#33750,#28240,.T.) ;
#42010=EDGE_CURVE('',#33762,#33704,#28241,.T.) ;
#42011=EDGE_CURVE('',#33744,#33750,#28242,.T.) ;
#42012=EDGE_CURVE('',#33746,#33702,#28243,.T.) ;
#42013=EDGE_CURVE('',#33696,#33749,#28244,.T.) ;
#42014=EDGE_CURVE('',#33747,#33700,#28245,.T.) ;
#42015=EDGE_CURVE('',#33698,#33748,#28246,.T.) ;
#42016=EDGE_CURVE('',#33113,#33044,#28247,.T.) ;
#42017=EDGE_CURVE('',#33035,#33112,#28248,.T.) ;
#42018=EDGE_CURVE('',#33114,#33107,#28249,.T.) ;
#42019=EDGE_CURVE('',#33108,#33113,#28250,.T.) ;
#42020=EDGE_CURVE('',#33114,#33918,#28251,.T.) ;
#42021=EDGE_CURVE('',#33918,#33107,#28252,.T.) ;
#42022=EDGE_CURVE('',#33035,#33117,#28253,.T.) ;
#42023=EDGE_CURVE('',#33117,#33112,#28254,.T.) ;
#42024=EDGE_CURVE('',#33108,#33043,#28255,.T.) ;
#42025=EDGE_CURVE('',#32096,#33110,#28256,.T.) ;
#42026=EDGE_CURVE('',#32097,#33919,#309,.T.) ;
#42027=EDGE_CURVE('',#33918,#33919,#11315,.T.) ;
#42028=EDGE_CURVE('',#33920,#33918,#310,.T.) ;
#42029=EDGE_CURVE('',#33920,#33921,#311,.T.) ;
#42030=EDGE_CURVE('',#32269,#33921,#11316,.T.) ;
#42031=EDGE_CURVE('',#33111,#32268,#28257,.T.) ;
#42032=EDGE_CURVE('',#33118,#33111,#28258,.T.) ;
#42033=EDGE_CURVE('',#33036,#33116,#28259,.T.) ;
#42034=EDGE_CURVE('',#33109,#33042,#28260,.T.) ;
#42035=EDGE_CURVE('',#33110,#32098,#28261,.T.) ;
#42036=EDGE_CURVE('',#33105,#33109,#28262,.T.) ;
#42037=EDGE_CURVE('',#33118,#32277,#28263,.T.) ;
#42038=EDGE_CURVE('',#33036,#32364,#28264,.T.) ;
#42039=EDGE_CURVE('',#32363,#33116,#28265,.T.) ;
#42040=EDGE_CURVE('',#33105,#33041,#28266,.T.) ;
#42041=EDGE_CURVE('',#33115,#32276,#28267,.T.) ;
#42042=EDGE_CURVE('',#32365,#33115,#28268,.T.) ;
#42043=EDGE_CURVE('',#33922,#32364,#11317,.T.) ;
#42044=EDGE_CURVE('',#33037,#33922,#28269,.T.) ;
#42045=EDGE_CURVE('',#33106,#33040,#28270,.T.) ;
#42046=EDGE_CURVE('',#32099,#33101,#28271,.T.) ;
#42047=EDGE_CURVE('',#33102,#33106,#28272,.T.) ;
#42048=EDGE_CURVE('',#32272,#33101,#28273,.T.) ;
#42049=EDGE_CURVE('',#32365,#32276,#28274,.T.) ;
#42050=EDGE_CURVE('',#32398,#32367,#28275,.T.) ;
#42051=EDGE_CURVE('',#32367,#32396,#28276,.T.) ;
#42052=EDGE_CURVE('',#33922,#32521,#28277,.T.) ;
#42053=EDGE_CURVE('',#33923,#33922,#28278,.T.) ;
#42054=EDGE_CURVE('',#33037,#33923,#28279,.T.) ;
#42055=EDGE_CURVE('',#33102,#33040,#28280,.T.) ;
#42056=EDGE_CURVE('',#32273,#33104,#28281,.T.) ;
#42057=EDGE_CURVE('',#32366,#32275,#28282,.T.) ;
#42058=EDGE_CURVE('',#32468,#32366,#28283,.T.) ;
#42059=EDGE_CURVE('',#33923,#32520,#28284,.T.) ;
#42060=EDGE_CURVE('',#33924,#33923,#11318,.T.) ;
#42061=EDGE_CURVE('',#33038,#33924,#28285,.T.) ;
#42062=EDGE_CURVE('',#33103,#33039,#28286,.T.) ;
#42063=EDGE_CURVE('',#33104,#32362,#28287,.T.) ;
#42064=EDGE_CURVE('',#32359,#33103,#28288,.T.) ;
#42065=EDGE_CURVE('',#32273,#32362,#28289,.T.) ;
#42066=EDGE_CURVE('',#32469,#32275,#28290,.T.) ;
#42067=EDGE_CURVE('',#33924,#32519,#28291,.T.) ;
#42068=EDGE_CURVE('',#33925,#33924,#28292,.T.) ;
#42069=EDGE_CURVE('',#33038,#33925,#28293,.T.) ;
#42070=EDGE_CURVE('',#32358,#33039,#28294,.T.) ;
#42071=EDGE_CURVE('',#32274,#32361,#28295,.T.) ;
#42072=EDGE_CURVE('',#32470,#32274,#28296,.T.) ;
#42073=EDGE_CURVE('',#33925,#32518,#28297,.T.) ;
#42074=EDGE_CURVE('',#32358,#33925,#11319,.T.) ;
#42075=EDGE_CURVE('',#32471,#32361,#28298,.T.) ;
#42076=EDGE_CURVE('',#32360,#32401,#28299,.T.) ;
#42077=EDGE_CURVE('',#32403,#32360,#28300,.T.) ;
#42078=EDGE_CURVE('',#33655,#33688,#28301,.T.) ;
#42079=EDGE_CURVE('',#33689,#33653,#28302,.T.) ;
#42080=EDGE_CURVE('',#33690,#33651,#28303,.T.) ;
#42081=EDGE_CURVE('',#33657,#33688,#28304,.T.) ;
#42082=EDGE_CURVE('',#33691,#33649,#28305,.T.) ;
#42083=EDGE_CURVE('',#33659,#33687,#28306,.T.) ;
#42084=EDGE_CURVE('',#33692,#33647,#28307,.T.) ;
#42085=EDGE_CURVE('',#33661,#33687,#28308,.T.) ;
#42086=EDGE_CURVE('',#33693,#33645,#28309,.T.) ;
#42087=EDGE_CURVE('',#33663,#33686,#28310,.T.) ;
#42088=EDGE_CURVE('',#33693,#33643,#28311,.T.) ;
#42089=EDGE_CURVE('',#33665,#33686,#28312,.T.) ;
#42090=EDGE_CURVE('',#33694,#32174,#28313,.T.) ;
#42091=EDGE_CURVE('',#33667,#33685,#28314,.T.) ;
#42092=EDGE_CURVE('',#33694,#32173,#28315,.T.) ;
#42093=EDGE_CURVE('',#33669,#33685,#28316,.T.) ;
#42094=EDGE_CURVE('',#33671,#33684,#28317,.T.) ;
#42095=EDGE_CURVE('',#33673,#33684,#28318,.T.) ;
#42096=EDGE_CURVE('',#33695,#33639,#28319,.T.) ;
#42097=EDGE_CURVE('',#33675,#33683,#28320,.T.) ;
#42098=EDGE_CURVE('',#33695,#33637,#28321,.T.) ;
#42099=EDGE_CURVE('',#33677,#33683,#28322,.T.) ;
#42100=EDGE_CURVE('',#33679,#33635,#28323,.T.) ;
#42101=EDGE_CURVE('',#33629,#33682,#28324,.T.) ;
#42102=EDGE_CURVE('',#33680,#33633,#28325,.T.) ;
#42103=EDGE_CURVE('',#33631,#33681,#28326,.T.) ;
#42104=EDGE_CURVE('',#33131,#33034,#28327,.T.) ;
#42105=EDGE_CURVE('',#33025,#33130,#28328,.T.) ;
#42106=EDGE_CURVE('',#33132,#33125,#28329,.T.) ;
#42107=EDGE_CURVE('',#33126,#33131,#28330,.T.) ;
#42108=EDGE_CURVE('',#33132,#33926,#28331,.T.) ;
#42109=EDGE_CURVE('',#33926,#33125,#28332,.T.) ;
#42110=EDGE_CURVE('',#33025,#33135,#28333,.T.) ;
#42111=EDGE_CURVE('',#33135,#33130,#28334,.T.) ;
#42112=EDGE_CURVE('',#33126,#33033,#28335,.T.) ;
#42113=EDGE_CURVE('',#32081,#33128,#28336,.T.) ;
#42114=EDGE_CURVE('',#32082,#33927,#312,.T.) ;
#42115=EDGE_CURVE('',#33926,#33927,#11320,.T.) ;
#42116=EDGE_CURVE('',#33928,#33926,#313,.T.) ;
#42117=EDGE_CURVE('',#33928,#33929,#314,.T.) ;
#42118=EDGE_CURVE('',#32259,#33929,#11321,.T.) ;
#42119=EDGE_CURVE('',#33129,#32258,#28337,.T.) ;
#42120=EDGE_CURVE('',#33136,#33129,#28338,.T.) ;
#42121=EDGE_CURVE('',#33026,#33134,#28339,.T.) ;
#42122=EDGE_CURVE('',#33127,#33032,#28340,.T.) ;
#42123=EDGE_CURVE('',#33128,#32083,#28341,.T.) ;
#42124=EDGE_CURVE('',#33123,#33127,#28342,.T.) ;
#42125=EDGE_CURVE('',#33136,#32267,#28343,.T.) ;
#42126=EDGE_CURVE('',#33026,#32354,#28344,.T.) ;
#42127=EDGE_CURVE('',#32353,#33134,#28345,.T.) ;
#42128=EDGE_CURVE('',#33123,#33031,#28346,.T.) ;
#42129=EDGE_CURVE('',#33133,#32266,#28347,.T.) ;
#42130=EDGE_CURVE('',#32355,#33133,#28348,.T.) ;
#42131=EDGE_CURVE('',#33930,#32354,#11322,.T.) ;
#42132=EDGE_CURVE('',#33027,#33930,#28349,.T.) ;
#42133=EDGE_CURVE('',#33124,#33030,#28350,.T.) ;
#42134=EDGE_CURVE('',#32084,#33119,#28351,.T.) ;
#42135=EDGE_CURVE('',#33120,#33124,#28352,.T.) ;
#42136=EDGE_CURVE('',#32262,#33119,#28353,.T.) ;
#42137=EDGE_CURVE('',#32355,#32266,#28354,.T.) ;
#42138=EDGE_CURVE('',#32402,#32357,#28355,.T.) ;
#42139=EDGE_CURVE('',#32357,#32400,#28356,.T.) ;
#42140=EDGE_CURVE('',#33930,#32517,#28357,.T.) ;
#42141=EDGE_CURVE('',#33931,#33930,#28358,.T.) ;
#42142=EDGE_CURVE('',#33027,#33931,#28359,.T.) ;
#42143=EDGE_CURVE('',#33120,#33030,#28360,.T.) ;
#42144=EDGE_CURVE('',#32263,#33122,#28361,.T.) ;
#42145=EDGE_CURVE('',#32356,#32265,#28362,.T.) ;
#42146=EDGE_CURVE('',#32472,#32356,#28363,.T.) ;
#42147=EDGE_CURVE('',#33931,#32516,#28364,.T.) ;
#42148=EDGE_CURVE('',#33932,#33931,#11323,.T.) ;
#42149=EDGE_CURVE('',#33028,#33932,#28365,.T.) ;
#42150=EDGE_CURVE('',#33121,#33029,#28366,.T.) ;
#42151=EDGE_CURVE('',#33122,#32352,#28367,.T.) ;
#42152=EDGE_CURVE('',#32349,#33121,#28368,.T.) ;
#42153=EDGE_CURVE('',#32263,#32352,#28369,.T.) ;
#42154=EDGE_CURVE('',#32473,#32265,#28370,.T.) ;
#42155=EDGE_CURVE('',#33932,#32515,#28371,.T.) ;
#42156=EDGE_CURVE('',#33933,#33932,#28372,.T.) ;
#42157=EDGE_CURVE('',#33028,#33933,#28373,.T.) ;
#42158=EDGE_CURVE('',#32348,#33029,#28374,.T.) ;
#42159=EDGE_CURVE('',#32264,#32351,#28375,.T.) ;
#42160=EDGE_CURVE('',#32474,#32264,#28376,.T.) ;
#42161=EDGE_CURVE('',#33933,#32514,#28377,.T.) ;
#42162=EDGE_CURVE('',#32348,#33933,#11324,.T.) ;
#42163=EDGE_CURVE('',#32475,#32351,#28378,.T.) ;
#42164=EDGE_CURVE('',#32350,#32405,#28379,.T.) ;
#42165=EDGE_CURVE('',#32407,#32350,#28380,.T.) ;
#42166=EDGE_CURVE('',#33588,#33621,#28381,.T.) ;
#42167=EDGE_CURVE('',#33622,#33586,#28382,.T.) ;
#42168=EDGE_CURVE('',#33623,#33584,#28383,.T.) ;
#42169=EDGE_CURVE('',#33590,#33621,#28384,.T.) ;
#42170=EDGE_CURVE('',#33624,#33582,#28385,.T.) ;
#42171=EDGE_CURVE('',#33592,#33620,#28386,.T.) ;
#42172=EDGE_CURVE('',#33625,#33580,#28387,.T.) ;
#42173=EDGE_CURVE('',#33594,#33620,#28388,.T.) ;
#42174=EDGE_CURVE('',#33626,#33578,#28389,.T.) ;
#42175=EDGE_CURVE('',#33596,#33619,#28390,.T.) ;
#42176=EDGE_CURVE('',#33626,#33576,#28391,.T.) ;
#42177=EDGE_CURVE('',#33598,#33619,#28392,.T.) ;
#42178=EDGE_CURVE('',#33627,#32176,#28393,.T.) ;
#42179=EDGE_CURVE('',#33600,#33618,#28394,.T.) ;
#42180=EDGE_CURVE('',#33627,#32175,#28395,.T.) ;
#42181=EDGE_CURVE('',#33602,#33618,#28396,.T.) ;
#42182=EDGE_CURVE('',#33604,#33617,#28397,.T.) ;
#42183=EDGE_CURVE('',#33606,#33617,#28398,.T.) ;
#42184=EDGE_CURVE('',#33628,#33572,#28399,.T.) ;
#42185=EDGE_CURVE('',#33608,#33616,#28400,.T.) ;
#42186=EDGE_CURVE('',#33628,#33570,#28401,.T.) ;
#42187=EDGE_CURVE('',#33610,#33616,#28402,.T.) ;
#42188=EDGE_CURVE('',#33612,#33568,#28403,.T.) ;
#42189=EDGE_CURVE('',#33562,#33615,#28404,.T.) ;
#42190=EDGE_CURVE('',#33613,#33566,#28405,.T.) ;
#42191=EDGE_CURVE('',#33564,#33614,#28406,.T.) ;
#42192=EDGE_CURVE('',#33149,#33024,#28407,.T.) ;
#42193=EDGE_CURVE('',#33015,#33148,#28408,.T.) ;
#42194=EDGE_CURVE('',#33150,#33143,#28409,.T.) ;
#42195=EDGE_CURVE('',#33144,#33149,#28410,.T.) ;
#42196=EDGE_CURVE('',#33150,#33934,#28411,.T.) ;
#42197=EDGE_CURVE('',#33934,#33143,#28412,.T.) ;
#42198=EDGE_CURVE('',#33015,#33153,#28413,.T.) ;
#42199=EDGE_CURVE('',#33153,#33148,#28414,.T.) ;
#42200=EDGE_CURVE('',#33144,#33023,#28415,.T.) ;
#42201=EDGE_CURVE('',#32066,#33146,#28416,.T.) ;
#42202=EDGE_CURVE('',#32067,#33935,#315,.T.) ;
#42203=EDGE_CURVE('',#33934,#33935,#11325,.T.) ;
#42204=EDGE_CURVE('',#33936,#33934,#316,.T.) ;
#42205=EDGE_CURVE('',#33936,#33937,#317,.T.) ;
#42206=EDGE_CURVE('',#32249,#33937,#11326,.T.) ;
#42207=EDGE_CURVE('',#33147,#32248,#28417,.T.) ;
#42208=EDGE_CURVE('',#33154,#33147,#28418,.T.) ;
#42209=EDGE_CURVE('',#33016,#33152,#28419,.T.) ;
#42210=EDGE_CURVE('',#33145,#33022,#28420,.T.) ;
#42211=EDGE_CURVE('',#33146,#32068,#28421,.T.) ;
#42212=EDGE_CURVE('',#33141,#33145,#28422,.T.) ;
#42213=EDGE_CURVE('',#33154,#32257,#28423,.T.) ;
#42214=EDGE_CURVE('',#33016,#32344,#28424,.T.) ;
#42215=EDGE_CURVE('',#32343,#33152,#28425,.T.) ;
#42216=EDGE_CURVE('',#33141,#33021,#28426,.T.) ;
#42217=EDGE_CURVE('',#33151,#32256,#28427,.T.) ;
#42218=EDGE_CURVE('',#32345,#33151,#28428,.T.) ;
#42219=EDGE_CURVE('',#33938,#32344,#11327,.T.) ;
#42220=EDGE_CURVE('',#33017,#33938,#28429,.T.) ;
#42221=EDGE_CURVE('',#33142,#33020,#28430,.T.) ;
#42222=EDGE_CURVE('',#32069,#33137,#28431,.T.) ;
#42223=EDGE_CURVE('',#33138,#33142,#28432,.T.) ;
#42224=EDGE_CURVE('',#32252,#33137,#28433,.T.) ;
#42225=EDGE_CURVE('',#32345,#32256,#28434,.T.) ;
#42226=EDGE_CURVE('',#32406,#32347,#28435,.T.) ;
#42227=EDGE_CURVE('',#32347,#32404,#28436,.T.) ;
#42228=EDGE_CURVE('',#33938,#32513,#28437,.T.) ;
#42229=EDGE_CURVE('',#33939,#33938,#28438,.T.) ;
#42230=EDGE_CURVE('',#33017,#33939,#28439,.T.) ;
#42231=EDGE_CURVE('',#33138,#33020,#28440,.T.) ;
#42232=EDGE_CURVE('',#32253,#33140,#28441,.T.) ;
#42233=EDGE_CURVE('',#32346,#32255,#28442,.T.) ;
#42234=EDGE_CURVE('',#32476,#32346,#28443,.T.) ;
#42235=EDGE_CURVE('',#33939,#32512,#28444,.T.) ;
#42236=EDGE_CURVE('',#33940,#33939,#11328,.T.) ;
#42237=EDGE_CURVE('',#33018,#33940,#28445,.T.) ;
#42238=EDGE_CURVE('',#33139,#33019,#28446,.T.) ;
#42239=EDGE_CURVE('',#33140,#32342,#28447,.T.) ;
#42240=EDGE_CURVE('',#32339,#33139,#28448,.T.) ;
#42241=EDGE_CURVE('',#32253,#32342,#28449,.T.) ;
#42242=EDGE_CURVE('',#32477,#32255,#28450,.T.) ;
#42243=EDGE_CURVE('',#33940,#32511,#28451,.T.) ;
#42244=EDGE_CURVE('',#33941,#33940,#28452,.T.) ;
#42245=EDGE_CURVE('',#33018,#33941,#28453,.T.) ;
#42246=EDGE_CURVE('',#32338,#33019,#28454,.T.) ;
#42247=EDGE_CURVE('',#32254,#32341,#28455,.T.) ;
#42248=EDGE_CURVE('',#32478,#32254,#28456,.T.) ;
#42249=EDGE_CURVE('',#33941,#32510,#28457,.T.) ;
#42250=EDGE_CURVE('',#32338,#33941,#11329,.T.) ;
#42251=EDGE_CURVE('',#32479,#32341,#28458,.T.) ;
#42252=EDGE_CURVE('',#32340,#32409,#28459,.T.) ;
#42253=EDGE_CURVE('',#32411,#32340,#28460,.T.) ;
#42254=EDGE_CURVE('',#33521,#33554,#28461,.T.) ;
#42255=EDGE_CURVE('',#33555,#33519,#28462,.T.) ;
#42256=EDGE_CURVE('',#33556,#33517,#28463,.T.) ;
#42257=EDGE_CURVE('',#33523,#33554,#28464,.T.) ;
#42258=EDGE_CURVE('',#33557,#33515,#28465,.T.) ;
#42259=EDGE_CURVE('',#33525,#33553,#28466,.T.) ;
#42260=EDGE_CURVE('',#33558,#33513,#28467,.T.) ;
#42261=EDGE_CURVE('',#33527,#33553,#28468,.T.) ;
#42262=EDGE_CURVE('',#33559,#33511,#28469,.T.) ;
#42263=EDGE_CURVE('',#33529,#33552,#28470,.T.) ;
#42264=EDGE_CURVE('',#33559,#33509,#28471,.T.) ;
#42265=EDGE_CURVE('',#33531,#33552,#28472,.T.) ;
#42266=EDGE_CURVE('',#33560,#32178,#28473,.T.) ;
#42267=EDGE_CURVE('',#33533,#33551,#28474,.T.) ;
#42268=EDGE_CURVE('',#33560,#32177,#28475,.T.) ;
#42269=EDGE_CURVE('',#33535,#33551,#28476,.T.) ;
#42270=EDGE_CURVE('',#33537,#33550,#28477,.T.) ;
#42271=EDGE_CURVE('',#33539,#33550,#28478,.T.) ;
#42272=EDGE_CURVE('',#33561,#33505,#28479,.T.) ;
#42273=EDGE_CURVE('',#33541,#33549,#28480,.T.) ;
#42274=EDGE_CURVE('',#33561,#33503,#28481,.T.) ;
#42275=EDGE_CURVE('',#33543,#33549,#28482,.T.) ;
#42276=EDGE_CURVE('',#33545,#33501,#28483,.T.) ;
#42277=EDGE_CURVE('',#33495,#33548,#28484,.T.) ;
#42278=EDGE_CURVE('',#33546,#33499,#28485,.T.) ;
#42279=EDGE_CURVE('',#33497,#33547,#28486,.T.) ;
#42280=EDGE_CURVE('',#33167,#33014,#28487,.T.) ;
#42281=EDGE_CURVE('',#33005,#33166,#28488,.T.) ;
#42282=EDGE_CURVE('',#33168,#33161,#28489,.T.) ;
#42283=EDGE_CURVE('',#33162,#33167,#28490,.T.) ;
#42284=EDGE_CURVE('',#33168,#33942,#28491,.T.) ;
#42285=EDGE_CURVE('',#33942,#33161,#28492,.T.) ;
#42286=EDGE_CURVE('',#33005,#33171,#28493,.T.) ;
#42287=EDGE_CURVE('',#33171,#33166,#28494,.T.) ;
#42288=EDGE_CURVE('',#33162,#33013,#28495,.T.) ;
#42289=EDGE_CURVE('',#32051,#33164,#28496,.T.) ;
#42290=EDGE_CURVE('',#32052,#33943,#318,.T.) ;
#42291=EDGE_CURVE('',#33942,#33943,#11330,.T.) ;
#42292=EDGE_CURVE('',#33944,#33942,#319,.T.) ;
#42293=EDGE_CURVE('',#33944,#33945,#320,.T.) ;
#42294=EDGE_CURVE('',#32239,#33945,#11331,.T.) ;
#42295=EDGE_CURVE('',#33165,#32238,#28497,.T.) ;
#42296=EDGE_CURVE('',#33172,#33165,#28498,.T.) ;
#42297=EDGE_CURVE('',#33006,#33170,#28499,.T.) ;
#42298=EDGE_CURVE('',#33163,#33012,#28500,.T.) ;
#42299=EDGE_CURVE('',#33164,#32053,#28501,.T.) ;
#42300=EDGE_CURVE('',#33159,#33163,#28502,.T.) ;
#42301=EDGE_CURVE('',#33172,#32247,#28503,.T.) ;
#42302=EDGE_CURVE('',#33006,#32334,#28504,.T.) ;
#42303=EDGE_CURVE('',#32333,#33170,#28505,.T.) ;
#42304=EDGE_CURVE('',#33159,#33011,#28506,.T.) ;
#42305=EDGE_CURVE('',#33169,#32246,#28507,.T.) ;
#42306=EDGE_CURVE('',#32335,#33169,#28508,.T.) ;
#42307=EDGE_CURVE('',#33946,#32334,#11332,.T.) ;
#42308=EDGE_CURVE('',#33007,#33946,#28509,.T.) ;
#42309=EDGE_CURVE('',#33160,#33010,#28510,.T.) ;
#42310=EDGE_CURVE('',#32054,#33155,#28511,.T.) ;
#42311=EDGE_CURVE('',#33156,#33160,#28512,.T.) ;
#42312=EDGE_CURVE('',#32242,#33155,#28513,.T.) ;
#42313=EDGE_CURVE('',#32335,#32246,#28514,.T.) ;
#42314=EDGE_CURVE('',#32410,#32337,#28515,.T.) ;
#42315=EDGE_CURVE('',#32337,#32408,#28516,.T.) ;
#42316=EDGE_CURVE('',#33946,#32509,#28517,.T.) ;
#42317=EDGE_CURVE('',#33947,#33946,#28518,.T.) ;
#42318=EDGE_CURVE('',#33007,#33947,#28519,.T.) ;
#42319=EDGE_CURVE('',#33156,#33010,#28520,.T.) ;
#42320=EDGE_CURVE('',#32243,#33158,#28521,.T.) ;
#42321=EDGE_CURVE('',#32336,#32245,#28522,.T.) ;
#42322=EDGE_CURVE('',#32480,#32336,#28523,.T.) ;
#42323=EDGE_CURVE('',#33947,#32508,#28524,.T.) ;
#42324=EDGE_CURVE('',#33948,#33947,#11333,.T.) ;
#42325=EDGE_CURVE('',#33008,#33948,#28525,.T.) ;
#42326=EDGE_CURVE('',#33157,#33009,#28526,.T.) ;
#42327=EDGE_CURVE('',#33158,#32332,#28527,.T.) ;
#42328=EDGE_CURVE('',#32329,#33157,#28528,.T.) ;
#42329=EDGE_CURVE('',#32243,#32332,#28529,.T.) ;
#42330=EDGE_CURVE('',#32481,#32245,#28530,.T.) ;
#42331=EDGE_CURVE('',#33948,#32507,#28531,.T.) ;
#42332=EDGE_CURVE('',#33949,#33948,#28532,.T.) ;
#42333=EDGE_CURVE('',#33008,#33949,#28533,.T.) ;
#42334=EDGE_CURVE('',#32328,#33009,#28534,.T.) ;
#42335=EDGE_CURVE('',#32244,#32331,#28535,.T.) ;
#42336=EDGE_CURVE('',#32482,#32244,#28536,.T.) ;
#42337=EDGE_CURVE('',#33949,#32506,#28537,.T.) ;
#42338=EDGE_CURVE('',#32328,#33949,#11334,.T.) ;
#42339=EDGE_CURVE('',#32483,#32331,#28538,.T.) ;
#42340=EDGE_CURVE('',#32330,#32413,#28539,.T.) ;
#42341=EDGE_CURVE('',#32415,#32330,#28540,.T.) ;
#42342=EDGE_CURVE('',#33454,#33487,#28541,.T.) ;
#42343=EDGE_CURVE('',#33488,#33452,#28542,.T.) ;
#42344=EDGE_CURVE('',#33489,#33450,#28543,.T.) ;
#42345=EDGE_CURVE('',#33456,#33487,#28544,.T.) ;
#42346=EDGE_CURVE('',#33490,#33448,#28545,.T.) ;
#42347=EDGE_CURVE('',#33458,#33486,#28546,.T.) ;
#42348=EDGE_CURVE('',#33491,#33446,#28547,.T.) ;
#42349=EDGE_CURVE('',#33460,#33486,#28548,.T.) ;
#42350=EDGE_CURVE('',#33492,#33444,#28549,.T.) ;
#42351=EDGE_CURVE('',#33462,#33485,#28550,.T.) ;
#42352=EDGE_CURVE('',#33492,#33442,#28551,.T.) ;
#42353=EDGE_CURVE('',#33464,#33485,#28552,.T.) ;
#42354=EDGE_CURVE('',#33493,#32180,#28553,.T.) ;
#42355=EDGE_CURVE('',#33466,#33484,#28554,.T.) ;
#42356=EDGE_CURVE('',#33493,#32179,#28555,.T.) ;
#42357=EDGE_CURVE('',#33468,#33484,#28556,.T.) ;
#42358=EDGE_CURVE('',#33470,#33483,#28557,.T.) ;
#42359=EDGE_CURVE('',#33472,#33483,#28558,.T.) ;
#42360=EDGE_CURVE('',#33494,#33438,#28559,.T.) ;
#42361=EDGE_CURVE('',#33474,#33482,#28560,.T.) ;
#42362=EDGE_CURVE('',#33494,#33436,#28561,.T.) ;
#42363=EDGE_CURVE('',#33476,#33482,#28562,.T.) ;
#42364=EDGE_CURVE('',#33478,#33434,#28563,.T.) ;
#42365=EDGE_CURVE('',#33428,#33481,#28564,.T.) ;
#42366=EDGE_CURVE('',#33479,#33432,#28565,.T.) ;
#42367=EDGE_CURVE('',#33430,#33480,#28566,.T.) ;
#42368=EDGE_CURVE('',#33185,#33004,#28567,.T.) ;
#42369=EDGE_CURVE('',#32995,#33184,#28568,.T.) ;
#42370=EDGE_CURVE('',#33186,#33179,#28569,.T.) ;
#42371=EDGE_CURVE('',#33180,#33185,#28570,.T.) ;
#42372=EDGE_CURVE('',#33186,#33950,#28571,.T.) ;
#42373=EDGE_CURVE('',#33950,#33179,#28572,.T.) ;
#42374=EDGE_CURVE('',#32995,#33189,#28573,.T.) ;
#42375=EDGE_CURVE('',#33189,#33184,#28574,.T.) ;
#42376=EDGE_CURVE('',#33180,#33003,#28575,.T.) ;
#42377=EDGE_CURVE('',#32036,#33182,#28576,.T.) ;
#42378=EDGE_CURVE('',#32037,#33951,#321,.T.) ;
#42379=EDGE_CURVE('',#33950,#33951,#11335,.T.) ;
#42380=EDGE_CURVE('',#33952,#33950,#322,.T.) ;
#42381=EDGE_CURVE('',#33952,#33953,#323,.T.) ;
#42382=EDGE_CURVE('',#32229,#33953,#11336,.T.) ;
#42383=EDGE_CURVE('',#33183,#32228,#28577,.T.) ;
#42384=EDGE_CURVE('',#33190,#33183,#28578,.T.) ;
#42385=EDGE_CURVE('',#32996,#33188,#28579,.T.) ;
#42386=EDGE_CURVE('',#33181,#33002,#28580,.T.) ;
#42387=EDGE_CURVE('',#33182,#32038,#28581,.T.) ;
#42388=EDGE_CURVE('',#33177,#33181,#28582,.T.) ;
#42389=EDGE_CURVE('',#33190,#32237,#28583,.T.) ;
#42390=EDGE_CURVE('',#32996,#32324,#28584,.T.) ;
#42391=EDGE_CURVE('',#32323,#33188,#28585,.T.) ;
#42392=EDGE_CURVE('',#33177,#33001,#28586,.T.) ;
#42393=EDGE_CURVE('',#33187,#32236,#28587,.T.) ;
#42394=EDGE_CURVE('',#32325,#33187,#28588,.T.) ;
#42395=EDGE_CURVE('',#33954,#32324,#11337,.T.) ;
#42396=EDGE_CURVE('',#32997,#33954,#28589,.T.) ;
#42397=EDGE_CURVE('',#33178,#33000,#28590,.T.) ;
#42398=EDGE_CURVE('',#32039,#33173,#28591,.T.) ;
#42399=EDGE_CURVE('',#33174,#33178,#28592,.T.) ;
#42400=EDGE_CURVE('',#32232,#33173,#28593,.T.) ;
#42401=EDGE_CURVE('',#32325,#32236,#28594,.T.) ;
#42402=EDGE_CURVE('',#32414,#32327,#28595,.T.) ;
#42403=EDGE_CURVE('',#32327,#32412,#28596,.T.) ;
#42404=EDGE_CURVE('',#33954,#32505,#28597,.T.) ;
#42405=EDGE_CURVE('',#33955,#33954,#28598,.T.) ;
#42406=EDGE_CURVE('',#32997,#33955,#28599,.T.) ;
#42407=EDGE_CURVE('',#33174,#33000,#28600,.T.) ;
#42408=EDGE_CURVE('',#32233,#33176,#28601,.T.) ;
#42409=EDGE_CURVE('',#32326,#32235,#28602,.T.) ;
#42410=EDGE_CURVE('',#32484,#32326,#28603,.T.) ;
#42411=EDGE_CURVE('',#33955,#32504,#28604,.T.) ;
#42412=EDGE_CURVE('',#33956,#33955,#11338,.T.) ;
#42413=EDGE_CURVE('',#32998,#33956,#28605,.T.) ;
#42414=EDGE_CURVE('',#33175,#32999,#28606,.T.) ;
#42415=EDGE_CURVE('',#33176,#32322,#28607,.T.) ;
#42416=EDGE_CURVE('',#32319,#33175,#28608,.T.) ;
#42417=EDGE_CURVE('',#32233,#32322,#28609,.T.) ;
#42418=EDGE_CURVE('',#32485,#32235,#28610,.T.) ;
#42419=EDGE_CURVE('',#33956,#32503,#28611,.T.) ;
#42420=EDGE_CURVE('',#33957,#33956,#28612,.T.) ;
#42421=EDGE_CURVE('',#32998,#33957,#28613,.T.) ;
#42422=EDGE_CURVE('',#32318,#32999,#28614,.T.) ;
#42423=EDGE_CURVE('',#32234,#32321,#28615,.T.) ;
#42424=EDGE_CURVE('',#32486,#32234,#28616,.T.) ;
#42425=EDGE_CURVE('',#33957,#32502,#28617,.T.) ;
#42426=EDGE_CURVE('',#32318,#33957,#11339,.T.) ;
#42427=EDGE_CURVE('',#32487,#32321,#28618,.T.) ;
#42428=EDGE_CURVE('',#32320,#32417,#28619,.T.) ;
#42429=EDGE_CURVE('',#32419,#32320,#28620,.T.) ;
#42430=EDGE_CURVE('',#33387,#33420,#28621,.T.) ;
#42431=EDGE_CURVE('',#33421,#33385,#28622,.T.) ;
#42432=EDGE_CURVE('',#33422,#33383,#28623,.T.) ;
#42433=EDGE_CURVE('',#33389,#33420,#28624,.T.) ;
#42434=EDGE_CURVE('',#33423,#33381,#28625,.T.) ;
#42435=EDGE_CURVE('',#33391,#33419,#28626,.T.) ;
#42436=EDGE_CURVE('',#33424,#33379,#28627,.T.) ;
#42437=EDGE_CURVE('',#33393,#33419,#28628,.T.) ;
#42438=EDGE_CURVE('',#33425,#33377,#28629,.T.) ;
#42439=EDGE_CURVE('',#33395,#33418,#28630,.T.) ;
#42440=EDGE_CURVE('',#33425,#33375,#28631,.T.) ;
#42441=EDGE_CURVE('',#33397,#33418,#28632,.T.) ;
#42442=EDGE_CURVE('',#33426,#32182,#28633,.T.) ;
#42443=EDGE_CURVE('',#33399,#33417,#28634,.T.) ;
#42444=EDGE_CURVE('',#33426,#32181,#28635,.T.) ;
#42445=EDGE_CURVE('',#33401,#33417,#28636,.T.) ;
#42446=EDGE_CURVE('',#33403,#33416,#28637,.T.) ;
#42447=EDGE_CURVE('',#33405,#33416,#28638,.T.) ;
#42448=EDGE_CURVE('',#33427,#33371,#28639,.T.) ;
#42449=EDGE_CURVE('',#33407,#33415,#28640,.T.) ;
#42450=EDGE_CURVE('',#33427,#33369,#28641,.T.) ;
#42451=EDGE_CURVE('',#33409,#33415,#28642,.T.) ;
#42452=EDGE_CURVE('',#33411,#33367,#28643,.T.) ;
#42453=EDGE_CURVE('',#33361,#33414,#28644,.T.) ;
#42454=EDGE_CURVE('',#33412,#33365,#28645,.T.) ;
#42455=EDGE_CURVE('',#33363,#33413,#28646,.T.) ;
#42456=EDGE_CURVE('',#33203,#32994,#28647,.T.) ;
#42457=EDGE_CURVE('',#32985,#33202,#28648,.T.) ;
#42458=EDGE_CURVE('',#33204,#33197,#28649,.T.) ;
#42459=EDGE_CURVE('',#33198,#33203,#28650,.T.) ;
#42460=EDGE_CURVE('',#33204,#33958,#28651,.T.) ;
#42461=EDGE_CURVE('',#33958,#33197,#28652,.T.) ;
#42462=EDGE_CURVE('',#32985,#33207,#28653,.T.) ;
#42463=EDGE_CURVE('',#33207,#33202,#28654,.T.) ;
#42464=EDGE_CURVE('',#33198,#32993,#28655,.T.) ;
#42465=EDGE_CURVE('',#32021,#33200,#28656,.T.) ;
#42466=EDGE_CURVE('',#32022,#33959,#324,.T.) ;
#42467=EDGE_CURVE('',#33958,#33959,#11340,.T.) ;
#42468=EDGE_CURVE('',#33960,#33958,#325,.T.) ;
#42469=EDGE_CURVE('',#33960,#33961,#326,.T.) ;
#42470=EDGE_CURVE('',#32219,#33961,#11341,.T.) ;
#42471=EDGE_CURVE('',#33201,#32218,#28657,.T.) ;
#42472=EDGE_CURVE('',#33208,#33201,#28658,.T.) ;
#42473=EDGE_CURVE('',#32986,#33206,#28659,.T.) ;
#42474=EDGE_CURVE('',#33199,#32992,#28660,.T.) ;
#42475=EDGE_CURVE('',#33200,#32023,#28661,.T.) ;
#42476=EDGE_CURVE('',#33195,#33199,#28662,.T.) ;
#42477=EDGE_CURVE('',#33208,#32227,#28663,.T.) ;
#42478=EDGE_CURVE('',#32986,#32314,#28664,.T.) ;
#42479=EDGE_CURVE('',#32313,#33206,#28665,.T.) ;
#42480=EDGE_CURVE('',#33195,#32991,#28666,.T.) ;
#42481=EDGE_CURVE('',#33205,#32226,#28667,.T.) ;
#42482=EDGE_CURVE('',#32315,#33205,#28668,.T.) ;
#42483=EDGE_CURVE('',#33962,#32314,#11342,.T.) ;
#42484=EDGE_CURVE('',#32987,#33962,#28669,.T.) ;
#42485=EDGE_CURVE('',#33196,#32990,#28670,.T.) ;
#42486=EDGE_CURVE('',#32024,#33191,#28671,.T.) ;
#42487=EDGE_CURVE('',#33192,#33196,#28672,.T.) ;
#42488=EDGE_CURVE('',#32222,#33191,#28673,.T.) ;
#42489=EDGE_CURVE('',#32315,#32226,#28674,.T.) ;
#42490=EDGE_CURVE('',#32418,#32317,#28675,.T.) ;
#42491=EDGE_CURVE('',#32317,#32416,#28676,.T.) ;
#42492=EDGE_CURVE('',#33962,#32501,#28677,.T.) ;
#42493=EDGE_CURVE('',#33963,#33962,#28678,.T.) ;
#42494=EDGE_CURVE('',#32987,#33963,#28679,.T.) ;
#42495=EDGE_CURVE('',#33192,#32990,#28680,.T.) ;
#42496=EDGE_CURVE('',#32223,#33194,#28681,.T.) ;
#42497=EDGE_CURVE('',#32316,#32225,#28682,.T.) ;
#42498=EDGE_CURVE('',#32488,#32316,#28683,.T.) ;
#42499=EDGE_CURVE('',#33963,#32500,#28684,.T.) ;
#42500=EDGE_CURVE('',#33964,#33963,#11343,.T.) ;
#42501=EDGE_CURVE('',#32988,#33964,#28685,.T.) ;
#42502=EDGE_CURVE('',#33193,#32989,#28686,.T.) ;
#42503=EDGE_CURVE('',#33194,#32312,#28687,.T.) ;
#42504=EDGE_CURVE('',#32309,#33193,#28688,.T.) ;
#42505=EDGE_CURVE('',#32223,#32312,#28689,.T.) ;
#42506=EDGE_CURVE('',#32489,#32225,#28690,.T.) ;
#42507=EDGE_CURVE('',#33964,#32499,#28691,.T.) ;
#42508=EDGE_CURVE('',#33965,#33964,#28692,.T.) ;
#42509=EDGE_CURVE('',#32988,#33965,#28693,.T.) ;
#42510=EDGE_CURVE('',#32308,#32989,#28694,.T.) ;
#42511=EDGE_CURVE('',#32224,#32311,#28695,.T.) ;
#42512=EDGE_CURVE('',#32490,#32224,#28696,.T.) ;
#42513=EDGE_CURVE('',#33965,#32498,#28697,.T.) ;
#42514=EDGE_CURVE('',#32308,#33965,#11344,.T.) ;
#42515=EDGE_CURVE('',#32491,#32311,#28698,.T.) ;
#42516=EDGE_CURVE('',#32310,#32421,#28699,.T.) ;
#42517=EDGE_CURVE('',#32423,#32310,#28700,.T.) ;
#42518=EDGE_CURVE('',#33320,#33353,#28701,.T.) ;
#42519=EDGE_CURVE('',#33354,#33318,#28702,.T.) ;
#42520=EDGE_CURVE('',#33355,#33316,#28703,.T.) ;
#42521=EDGE_CURVE('',#33322,#33353,#28704,.T.) ;
#42522=EDGE_CURVE('',#33356,#33314,#28705,.T.) ;
#42523=EDGE_CURVE('',#33324,#33352,#28706,.T.) ;
#42524=EDGE_CURVE('',#33357,#33312,#28707,.T.) ;
#42525=EDGE_CURVE('',#33326,#33352,#28708,.T.) ;
#42526=EDGE_CURVE('',#33358,#33310,#28709,.T.) ;
#42527=EDGE_CURVE('',#33328,#33351,#28710,.T.) ;
#42528=EDGE_CURVE('',#33358,#33308,#28711,.T.) ;
#42529=EDGE_CURVE('',#33330,#33351,#28712,.T.) ;
#42530=EDGE_CURVE('',#33359,#32184,#28713,.T.) ;
#42531=EDGE_CURVE('',#33332,#33350,#28714,.T.) ;
#42532=EDGE_CURVE('',#33359,#32183,#28715,.T.) ;
#42533=EDGE_CURVE('',#33334,#33350,#28716,.T.) ;
#42534=EDGE_CURVE('',#33336,#33349,#28717,.T.) ;
#42535=EDGE_CURVE('',#33338,#33349,#28718,.T.) ;
#42536=EDGE_CURVE('',#33360,#33304,#28719,.T.) ;
#42537=EDGE_CURVE('',#33340,#33348,#28720,.T.) ;
#42538=EDGE_CURVE('',#33360,#33302,#28721,.T.) ;
#42539=EDGE_CURVE('',#33342,#33348,#28722,.T.) ;
#42540=EDGE_CURVE('',#33344,#33300,#28723,.T.) ;
#42541=EDGE_CURVE('',#33294,#33347,#28724,.T.) ;
#42542=EDGE_CURVE('',#33345,#33298,#28725,.T.) ;
#42543=EDGE_CURVE('',#33296,#33346,#28726,.T.) ;
#42544=EDGE_CURVE('',#33221,#32984,#28727,.T.) ;
#42545=EDGE_CURVE('',#32975,#33220,#28728,.T.) ;
#42546=EDGE_CURVE('',#33222,#33215,#28729,.T.) ;
#42547=EDGE_CURVE('',#33216,#33221,#28730,.T.) ;
#42548=EDGE_CURVE('',#33222,#33966,#28731,.T.) ;
#42549=EDGE_CURVE('',#33966,#33215,#28732,.T.) ;
#42550=EDGE_CURVE('',#32975,#33225,#28733,.T.) ;
#42551=EDGE_CURVE('',#33225,#33220,#28734,.T.) ;
#42552=EDGE_CURVE('',#33216,#32983,#28735,.T.) ;
#42553=EDGE_CURVE('',#32006,#33218,#28736,.T.) ;
#42554=EDGE_CURVE('',#32007,#33967,#327,.T.) ;
#42555=EDGE_CURVE('',#33966,#33967,#11345,.T.) ;
#42556=EDGE_CURVE('',#33968,#33966,#328,.T.) ;
#42557=EDGE_CURVE('',#33968,#33969,#329,.T.) ;
#42558=EDGE_CURVE('',#32209,#33969,#11346,.T.) ;
#42559=EDGE_CURVE('',#33219,#32208,#28737,.T.) ;
#42560=EDGE_CURVE('',#33226,#33219,#28738,.T.) ;
#42561=EDGE_CURVE('',#32976,#33224,#28739,.T.) ;
#42562=EDGE_CURVE('',#33217,#32982,#28740,.T.) ;
#42563=EDGE_CURVE('',#33218,#32008,#28741,.T.) ;
#42564=EDGE_CURVE('',#33213,#33217,#28742,.T.) ;
#42565=EDGE_CURVE('',#33226,#32217,#28743,.T.) ;
#42566=EDGE_CURVE('',#32976,#32304,#28744,.T.) ;
#42567=EDGE_CURVE('',#32303,#33224,#28745,.T.) ;
#42568=EDGE_CURVE('',#33213,#32981,#28746,.T.) ;
#42569=EDGE_CURVE('',#33223,#32216,#28747,.T.) ;
#42570=EDGE_CURVE('',#32305,#33223,#28748,.T.) ;
#42571=EDGE_CURVE('',#33970,#32304,#11347,.T.) ;
#42572=EDGE_CURVE('',#32977,#33970,#28749,.T.) ;
#42573=EDGE_CURVE('',#33214,#32980,#28750,.T.) ;
#42574=EDGE_CURVE('',#32009,#33209,#28751,.T.) ;
#42575=EDGE_CURVE('',#33210,#33214,#28752,.T.) ;
#42576=EDGE_CURVE('',#32212,#33209,#28753,.T.) ;
#42577=EDGE_CURVE('',#32305,#32216,#28754,.T.) ;
#42578=EDGE_CURVE('',#32422,#32307,#28755,.T.) ;
#42579=EDGE_CURVE('',#32307,#32420,#28756,.T.) ;
#42580=EDGE_CURVE('',#33970,#32496,#28757,.T.) ;
#42581=EDGE_CURVE('',#33971,#33970,#28758,.T.) ;
#42582=EDGE_CURVE('',#32977,#33971,#28759,.T.) ;
#42583=EDGE_CURVE('',#33210,#32980,#28760,.T.) ;
#42584=EDGE_CURVE('',#32213,#33212,#28761,.T.) ;
#42585=EDGE_CURVE('',#32306,#32215,#28762,.T.) ;
#42586=EDGE_CURVE('',#32492,#32306,#28763,.T.) ;
#42587=EDGE_CURVE('',#33971,#32497,#28764,.T.) ;
#42588=EDGE_CURVE('',#33972,#33971,#11348,.T.) ;
#42589=EDGE_CURVE('',#32978,#33972,#28765,.T.) ;
#42590=EDGE_CURVE('',#33211,#32979,#28766,.T.) ;
#42591=EDGE_CURVE('',#33212,#32302,#28767,.T.) ;
#42592=EDGE_CURVE('',#32299,#33211,#28768,.T.) ;
#42593=EDGE_CURVE('',#32213,#32302,#28769,.T.) ;
#42594=EDGE_CURVE('',#32493,#32215,#28770,.T.) ;
#42595=EDGE_CURVE('',#33972,#32537,#28771,.T.) ;
#42596=EDGE_CURVE('',#33973,#33972,#28772,.T.) ;
#42597=EDGE_CURVE('',#32978,#33973,#28773,.T.) ;
#42598=EDGE_CURVE('',#32298,#32979,#28774,.T.) ;
#42599=EDGE_CURVE('',#32214,#32301,#28775,.T.) ;
#42600=EDGE_CURVE('',#32453,#32214,#28776,.T.) ;
#42601=EDGE_CURVE('',#33973,#32536,#28777,.T.) ;
#42602=EDGE_CURVE('',#32298,#33973,#11349,.T.) ;
#42603=EDGE_CURVE('',#32452,#32301,#28778,.T.) ;
#42604=EDGE_CURVE('',#32300,#32494,#28779,.T.) ;
#42605=EDGE_CURVE('',#32454,#32300,#28780,.T.) ;
#42606=EDGE_CURVE('',#33253,#33286,#28781,.T.) ;
#42607=EDGE_CURVE('',#33287,#33251,#28782,.T.) ;
#42608=EDGE_CURVE('',#33288,#33249,#28783,.T.) ;
#42609=EDGE_CURVE('',#33255,#33286,#28784,.T.) ;
#42610=EDGE_CURVE('',#33289,#33247,#28785,.T.) ;
#42611=EDGE_CURVE('',#33257,#33285,#28786,.T.) ;
#42612=EDGE_CURVE('',#33290,#33245,#28787,.T.) ;
#42613=EDGE_CURVE('',#33259,#33285,#28788,.T.) ;
#42614=EDGE_CURVE('',#33291,#33243,#28789,.T.) ;
#42615=EDGE_CURVE('',#33261,#33284,#28790,.T.) ;
#42616=EDGE_CURVE('',#33291,#33241,#28791,.T.) ;
#42617=EDGE_CURVE('',#33263,#33284,#28792,.T.) ;
#42618=EDGE_CURVE('',#33292,#32186,#28793,.T.) ;
#42619=EDGE_CURVE('',#33265,#33283,#28794,.T.) ;
#42620=EDGE_CURVE('',#33292,#32185,#28795,.T.) ;
#42621=EDGE_CURVE('',#33267,#33283,#28796,.T.) ;
#42622=EDGE_CURVE('',#33269,#33282,#28797,.T.) ;
#42623=EDGE_CURVE('',#33271,#33282,#28798,.T.) ;
#42624=EDGE_CURVE('',#33293,#33237,#28799,.T.) ;
#42625=EDGE_CURVE('',#33273,#33281,#28800,.T.) ;
#42626=EDGE_CURVE('',#33293,#33235,#28801,.T.) ;
#42627=EDGE_CURVE('',#33275,#33281,#28802,.T.) ;
#42628=EDGE_CURVE('',#33277,#33233,#28803,.T.) ;
#42629=EDGE_CURVE('',#33227,#33280,#28804,.T.) ;
#42630=EDGE_CURVE('',#33278,#33231,#28805,.T.) ;
#42631=EDGE_CURVE('',#33229,#33279,#28806,.T.) ;
#42632=EDGE_CURVE('',#33974,#33975,#11350,.T.) ;
#42633=EDGE_CURVE('',#33975,#33976,#11351,.T.) ;
#42634=EDGE_CURVE('',#33976,#33977,#11352,.T.) ;
#42635=EDGE_CURVE('',#33977,#33974,#11353,.T.) ;
#42636=EDGE_CURVE('',#33978,#33979,#11354,.T.) ;
#42637=EDGE_CURVE('',#33979,#33980,#11355,.T.) ;
#42638=EDGE_CURVE('',#33980,#33981,#11356,.T.) ;
#42639=EDGE_CURVE('',#33981,#33978,#11357,.T.) ;
#42640=EDGE_CURVE('',#33982,#33983,#11358,.T.) ;
#42641=EDGE_CURVE('',#33983,#33984,#11359,.T.) ;
#42642=EDGE_CURVE('',#33984,#33985,#11360,.T.) ;
#42643=EDGE_CURVE('',#33985,#33982,#11361,.T.) ;
#42644=EDGE_CURVE('',#33986,#33987,#11362,.T.) ;
#42645=EDGE_CURVE('',#33987,#33988,#11363,.T.) ;
#42646=EDGE_CURVE('',#33988,#33989,#11364,.T.) ;
#42647=EDGE_CURVE('',#33989,#33986,#11365,.T.) ;
#42648=EDGE_CURVE('',#33990,#33991,#11366,.T.) ;
#42649=EDGE_CURVE('',#33991,#33992,#11367,.T.) ;
#42650=EDGE_CURVE('',#33993,#33992,#11368,.T.) ;
#42651=EDGE_CURVE('',#33993,#33990,#11369,.T.) ;
#42652=EDGE_CURVE('',#33994,#33995,#11370,.T.) ;
#42653=EDGE_CURVE('',#33995,#32289,#28807,.T.) ;
#42654=EDGE_CURVE('',#33905,#33996,#28808,.T.) ;
#42655=EDGE_CURVE('',#33996,#33997,#11371,.T.) ;
#42656=EDGE_CURVE('',#33997,#33994,#11372,.T.) ;
#42657=EDGE_CURVE('',#33998,#33999,#11373,.T.) ;
#42658=EDGE_CURVE('',#33999,#32168,#28809,.T.) ;
#42659=EDGE_CURVE('',#32167,#34000,#28810,.T.) ;
#42660=EDGE_CURVE('',#34000,#34001,#11374,.T.) ;
#42661=EDGE_CURVE('',#34001,#33998,#11375,.T.) ;
#42662=EDGE_CURVE('',#33903,#33975,#28811,.T.) ;
#42663=EDGE_CURVE('',#33974,#33904,#28812,.T.) ;
#42664=EDGE_CURVE('',#33992,#32291,#28813,.T.) ;
#42665=EDGE_CURVE('',#32290,#33993,#28814,.T.) ;
#42666=EDGE_CURVE('',#34002,#34003,#11376,.T.) ;
#42667=EDGE_CURVE('',#34003,#34004,#11377,.T.) ;
#42668=EDGE_CURVE('',#34004,#34005,#11378,.T.) ;
#42669=EDGE_CURVE('',#34005,#34002,#11379,.T.) ;
#42670=EDGE_CURVE('',#34006,#34007,#11380,.T.) ;
#42671=EDGE_CURVE('',#34007,#33833,#11381,.T.) ;
#42672=EDGE_CURVE('',#33832,#34006,#11382,.T.) ;
#42673=EDGE_CURVE('',#33836,#34008,#11383,.T.) ;
#42674=EDGE_CURVE('',#34008,#34009,#11384,.T.) ;
#42675=EDGE_CURVE('',#34009,#33837,#11385,.T.) ;
#42676=EDGE_CURVE('',#34010,#34011,#11386,.T.) ;
#42677=EDGE_CURVE('',#34011,#34012,#11387,.T.) ;
#42678=EDGE_CURVE('',#34012,#34013,#11388,.T.) ;
#42679=EDGE_CURVE('',#34013,#34010,#11389,.T.) ;
#42680=EDGE_CURVE('',#34014,#34015,#11390,.T.) ;
#42681=EDGE_CURVE('',#34015,#34016,#11391,.T.) ;
#42682=EDGE_CURVE('',#34016,#34017,#11392,.T.) ;
#42683=EDGE_CURVE('',#34017,#34014,#11393,.T.) ;
#42684=EDGE_CURVE('',#34018,#34019,#11394,.T.) ;
#42685=EDGE_CURVE('',#34019,#33830,#11395,.T.) ;
#42686=EDGE_CURVE('',#33831,#34018,#11396,.T.) ;
#42687=EDGE_CURVE('',#33834,#34020,#11397,.T.) ;
#42688=EDGE_CURVE('',#34020,#34021,#11398,.T.) ;
#42689=EDGE_CURVE('',#34021,#33835,#11399,.T.) ;
#42690=EDGE_CURVE('',#34022,#34023,#11400,.T.) ;
#42691=EDGE_CURVE('',#34023,#34024,#11401,.T.) ;
#42692=EDGE_CURVE('',#34024,#34025,#11402,.T.) ;
#42693=EDGE_CURVE('',#34025,#34022,#11403,.T.) ;
#42694=EDGE_CURVE('',#34026,#34027,#11404,.T.) ;
#42695=EDGE_CURVE('',#34027,#34028,#11405,.T.) ;
#42696=EDGE_CURVE('',#34028,#34029,#11406,.T.) ;
#42697=EDGE_CURVE('',#34029,#34026,#11407,.T.) ;
#42698=EDGE_CURVE('',#34030,#34031,#11408,.T.) ;
#42699=EDGE_CURVE('',#34031,#34032,#11409,.T.) ;
#42700=EDGE_CURVE('',#34032,#34033,#11410,.T.) ;
#42701=EDGE_CURVE('',#34033,#34030,#11411,.T.) ;
#42702=EDGE_CURVE('',#34034,#34035,#11412,.T.) ;
#42703=EDGE_CURVE('',#34035,#34036,#11413,.T.) ;
#42704=EDGE_CURVE('',#34036,#34037,#11414,.T.) ;
#42705=EDGE_CURVE('',#34037,#34034,#11415,.T.) ;
#42706=EDGE_CURVE('',#34038,#34039,#11416,.T.) ;
#42707=EDGE_CURVE('',#34039,#34040,#11417,.T.) ;
#42708=EDGE_CURVE('',#34041,#34040,#11418,.T.) ;
#42709=EDGE_CURVE('',#34041,#34038,#11419,.T.) ;
#42710=EDGE_CURVE('',#34042,#34043,#11420,.T.) ;
#42711=EDGE_CURVE('',#34043,#32279,#28815,.T.) ;
#42712=EDGE_CURVE('',#33913,#34044,#28816,.T.) ;
#42713=EDGE_CURVE('',#34044,#34045,#11421,.T.) ;
#42714=EDGE_CURVE('',#34045,#34042,#11422,.T.) ;
#42715=EDGE_CURVE('',#34046,#34047,#11423,.T.) ;
#42716=EDGE_CURVE('',#34047,#32117,#28817,.T.) ;
#42717=EDGE_CURVE('',#32116,#34048,#28818,.T.) ;
#42718=EDGE_CURVE('',#34048,#34049,#11424,.T.) ;
#42719=EDGE_CURVE('',#34049,#34046,#11425,.T.) ;
#42720=EDGE_CURVE('',#33911,#34023,#28819,.T.) ;
#42721=EDGE_CURVE('',#34022,#33912,#28820,.T.) ;
#42722=EDGE_CURVE('',#34040,#32281,#28821,.T.) ;
#42723=EDGE_CURVE('',#32280,#34041,#28822,.T.) ;
#42724=EDGE_CURVE('',#34050,#34051,#11426,.T.) ;
#42725=EDGE_CURVE('',#34051,#34052,#11427,.T.) ;
#42726=EDGE_CURVE('',#34052,#34053,#11428,.T.) ;
#42727=EDGE_CURVE('',#34053,#34050,#11429,.T.) ;
#42728=EDGE_CURVE('',#34054,#34055,#11430,.T.) ;
#42729=EDGE_CURVE('',#34055,#33841,#11431,.T.) ;
#42730=EDGE_CURVE('',#33840,#34054,#11432,.T.) ;
#42731=EDGE_CURVE('',#33844,#34056,#11433,.T.) ;
#42732=EDGE_CURVE('',#34056,#34057,#11434,.T.) ;
#42733=EDGE_CURVE('',#34057,#33845,#11435,.T.) ;
#42734=EDGE_CURVE('',#34058,#34059,#11436,.T.) ;
#42735=EDGE_CURVE('',#34059,#34060,#11437,.T.) ;
#42736=EDGE_CURVE('',#34060,#34061,#11438,.T.) ;
#42737=EDGE_CURVE('',#34061,#34058,#11439,.T.) ;
#42738=EDGE_CURVE('',#34062,#34063,#11440,.T.) ;
#42739=EDGE_CURVE('',#34063,#34064,#11441,.T.) ;
#42740=EDGE_CURVE('',#34064,#34065,#11442,.T.) ;
#42741=EDGE_CURVE('',#34065,#34062,#11443,.T.) ;
#42742=EDGE_CURVE('',#34066,#34067,#11444,.T.) ;
#42743=EDGE_CURVE('',#34067,#33838,#11445,.T.) ;
#42744=EDGE_CURVE('',#33839,#34066,#11446,.T.) ;
#42745=EDGE_CURVE('',#33842,#34068,#11447,.T.) ;
#42746=EDGE_CURVE('',#34068,#34069,#11448,.T.) ;
#42747=EDGE_CURVE('',#34069,#33843,#11449,.T.) ;
#42748=EDGE_CURVE('',#34070,#34071,#11450,.T.) ;
#42749=EDGE_CURVE('',#34071,#34072,#11451,.T.) ;
#42750=EDGE_CURVE('',#34072,#34073,#11452,.T.) ;
#42751=EDGE_CURVE('',#34073,#34070,#11453,.T.) ;
#42752=EDGE_CURVE('',#34074,#34075,#11454,.T.) ;
#42753=EDGE_CURVE('',#34075,#34076,#11455,.T.) ;
#42754=EDGE_CURVE('',#34076,#34077,#11456,.T.) ;
#42755=EDGE_CURVE('',#34077,#34074,#11457,.T.) ;
#42756=EDGE_CURVE('',#34078,#34079,#11458,.T.) ;
#42757=EDGE_CURVE('',#34079,#34080,#11459,.T.) ;
#42758=EDGE_CURVE('',#34080,#34081,#11460,.T.) ;
#42759=EDGE_CURVE('',#34081,#34078,#11461,.T.) ;
#42760=EDGE_CURVE('',#34082,#34083,#11462,.T.) ;
#42761=EDGE_CURVE('',#34083,#34084,#11463,.T.) ;
#42762=EDGE_CURVE('',#34084,#34085,#11464,.T.) ;
#42763=EDGE_CURVE('',#34085,#34082,#11465,.T.) ;
#42764=EDGE_CURVE('',#34086,#34087,#11466,.T.) ;
#42765=EDGE_CURVE('',#34087,#34088,#11467,.T.) ;
#42766=EDGE_CURVE('',#34089,#34088,#11468,.T.) ;
#42767=EDGE_CURVE('',#34089,#34086,#11469,.T.) ;
#42768=EDGE_CURVE('',#34090,#34091,#11470,.T.) ;
#42769=EDGE_CURVE('',#34091,#32269,#28823,.T.) ;
#42770=EDGE_CURVE('',#33921,#34092,#28824,.T.) ;
#42771=EDGE_CURVE('',#34092,#34093,#11471,.T.) ;
#42772=EDGE_CURVE('',#34093,#34090,#11472,.T.) ;
#42773=EDGE_CURVE('',#34094,#34095,#11473,.T.) ;
#42774=EDGE_CURVE('',#34095,#32102,#28825,.T.) ;
#42775=EDGE_CURVE('',#32101,#34096,#28826,.T.) ;
#42776=EDGE_CURVE('',#34096,#34097,#11474,.T.) ;
#42777=EDGE_CURVE('',#34097,#34094,#11475,.T.) ;
#42778=EDGE_CURVE('',#33919,#34071,#28827,.T.) ;
#42779=EDGE_CURVE('',#34070,#33920,#28828,.T.) ;
#42780=EDGE_CURVE('',#34088,#32271,#28829,.T.) ;
#42781=EDGE_CURVE('',#32270,#34089,#28830,.T.) ;
#42782=EDGE_CURVE('',#34098,#34099,#11476,.T.) ;
#42783=EDGE_CURVE('',#34099,#34100,#11477,.T.) ;
#42784=EDGE_CURVE('',#34100,#34101,#11478,.T.) ;
#42785=EDGE_CURVE('',#34101,#34098,#11479,.T.) ;
#42786=EDGE_CURVE('',#34102,#34103,#11480,.T.) ;
#42787=EDGE_CURVE('',#34103,#33849,#11481,.T.) ;
#42788=EDGE_CURVE('',#33848,#34102,#11482,.T.) ;
#42789=EDGE_CURVE('',#33852,#34104,#11483,.T.) ;
#42790=EDGE_CURVE('',#34104,#34105,#11484,.T.) ;
#42791=EDGE_CURVE('',#34105,#33853,#11485,.T.) ;
#42792=EDGE_CURVE('',#34106,#34107,#11486,.T.) ;
#42793=EDGE_CURVE('',#34107,#34108,#11487,.T.) ;
#42794=EDGE_CURVE('',#34108,#34109,#11488,.T.) ;
#42795=EDGE_CURVE('',#34109,#34106,#11489,.T.) ;
#42796=EDGE_CURVE('',#34110,#34111,#11490,.T.) ;
#42797=EDGE_CURVE('',#34111,#34112,#11491,.T.) ;
#42798=EDGE_CURVE('',#34112,#34113,#11492,.T.) ;
#42799=EDGE_CURVE('',#34113,#34110,#11493,.T.) ;
#42800=EDGE_CURVE('',#34114,#34115,#11494,.T.) ;
#42801=EDGE_CURVE('',#34115,#33846,#11495,.T.) ;
#42802=EDGE_CURVE('',#33847,#34114,#11496,.T.) ;
#42803=EDGE_CURVE('',#33850,#34116,#11497,.T.) ;
#42804=EDGE_CURVE('',#34116,#34117,#11498,.T.) ;
#42805=EDGE_CURVE('',#34117,#33851,#11499,.T.) ;
#42806=EDGE_CURVE('',#34118,#34119,#11500,.T.) ;
#42807=EDGE_CURVE('',#34119,#34120,#11501,.T.) ;
#42808=EDGE_CURVE('',#34120,#34121,#11502,.T.) ;
#42809=EDGE_CURVE('',#34121,#34118,#11503,.T.) ;
#42810=EDGE_CURVE('',#34122,#34123,#11504,.T.) ;
#42811=EDGE_CURVE('',#34123,#34124,#11505,.T.) ;
#42812=EDGE_CURVE('',#34124,#34125,#11506,.T.) ;
#42813=EDGE_CURVE('',#34125,#34122,#11507,.T.) ;
#42814=EDGE_CURVE('',#34126,#34127,#11508,.T.) ;
#42815=EDGE_CURVE('',#34127,#34128,#11509,.T.) ;
#42816=EDGE_CURVE('',#34128,#34129,#11510,.T.) ;
#42817=EDGE_CURVE('',#34129,#34126,#11511,.T.) ;
#42818=EDGE_CURVE('',#34130,#34131,#11512,.T.) ;
#42819=EDGE_CURVE('',#34131,#34132,#11513,.T.) ;
#42820=EDGE_CURVE('',#34132,#34133,#11514,.T.) ;
#42821=EDGE_CURVE('',#34133,#34130,#11515,.T.) ;
#42822=EDGE_CURVE('',#34134,#34135,#11516,.T.) ;
#42823=EDGE_CURVE('',#34135,#34136,#11517,.T.) ;
#42824=EDGE_CURVE('',#34137,#34136,#11518,.T.) ;
#42825=EDGE_CURVE('',#34137,#34134,#11519,.T.) ;
#42826=EDGE_CURVE('',#34138,#34139,#11520,.T.) ;
#42827=EDGE_CURVE('',#34139,#32259,#28831,.T.) ;
#42828=EDGE_CURVE('',#33929,#34140,#28832,.T.) ;
#42829=EDGE_CURVE('',#34140,#34141,#11521,.T.) ;
#42830=EDGE_CURVE('',#34141,#34138,#11522,.T.) ;
#42831=EDGE_CURVE('',#34142,#34143,#11523,.T.) ;
#42832=EDGE_CURVE('',#34143,#32087,#28833,.T.) ;
#42833=EDGE_CURVE('',#32086,#34144,#28834,.T.) ;
#42834=EDGE_CURVE('',#34144,#34145,#11524,.T.) ;
#42835=EDGE_CURVE('',#34145,#34142,#11525,.T.) ;
#42836=EDGE_CURVE('',#33927,#34119,#28835,.T.) ;
#42837=EDGE_CURVE('',#34118,#33928,#28836,.T.) ;
#42838=EDGE_CURVE('',#34136,#32261,#28837,.T.) ;
#42839=EDGE_CURVE('',#32260,#34137,#28838,.T.) ;
#42840=EDGE_CURVE('',#34146,#34147,#11526,.T.) ;
#42841=EDGE_CURVE('',#34147,#34148,#11527,.T.) ;
#42842=EDGE_CURVE('',#34148,#34149,#11528,.T.) ;
#42843=EDGE_CURVE('',#34149,#34146,#11529,.T.) ;
#42844=EDGE_CURVE('',#34150,#34151,#11530,.T.) ;
#42845=EDGE_CURVE('',#34151,#33857,#11531,.T.) ;
#42846=EDGE_CURVE('',#33856,#34150,#11532,.T.) ;
#42847=EDGE_CURVE('',#33860,#34152,#11533,.T.) ;
#42848=EDGE_CURVE('',#34152,#34153,#11534,.T.) ;
#42849=EDGE_CURVE('',#34153,#33861,#11535,.T.) ;
#42850=EDGE_CURVE('',#34154,#34155,#11536,.T.) ;
#42851=EDGE_CURVE('',#34155,#34156,#11537,.T.) ;
#42852=EDGE_CURVE('',#34156,#34157,#11538,.T.) ;
#42853=EDGE_CURVE('',#34157,#34154,#11539,.T.) ;
#42854=EDGE_CURVE('',#34158,#34159,#11540,.T.) ;
#42855=EDGE_CURVE('',#34159,#34160,#11541,.T.) ;
#42856=EDGE_CURVE('',#34160,#34161,#11542,.T.) ;
#42857=EDGE_CURVE('',#34161,#34158,#11543,.T.) ;
#42858=EDGE_CURVE('',#34162,#34163,#11544,.T.) ;
#42859=EDGE_CURVE('',#34163,#33854,#11545,.T.) ;
#42860=EDGE_CURVE('',#33855,#34162,#11546,.T.) ;
#42861=EDGE_CURVE('',#33858,#34164,#11547,.T.) ;
#42862=EDGE_CURVE('',#34164,#34165,#11548,.T.) ;
#42863=EDGE_CURVE('',#34165,#33859,#11549,.T.) ;
#42864=EDGE_CURVE('',#34166,#34167,#11550,.T.) ;
#42865=EDGE_CURVE('',#34167,#34168,#11551,.T.) ;
#42866=EDGE_CURVE('',#34168,#34169,#11552,.T.) ;
#42867=EDGE_CURVE('',#34169,#34166,#11553,.T.) ;
#42868=EDGE_CURVE('',#34170,#34171,#11554,.T.) ;
#42869=EDGE_CURVE('',#34171,#34172,#11555,.T.) ;
#42870=EDGE_CURVE('',#34172,#34173,#11556,.T.) ;
#42871=EDGE_CURVE('',#34173,#34170,#11557,.T.) ;
#42872=EDGE_CURVE('',#34174,#34175,#11558,.T.) ;
#42873=EDGE_CURVE('',#34175,#34176,#11559,.T.) ;
#42874=EDGE_CURVE('',#34176,#34177,#11560,.T.) ;
#42875=EDGE_CURVE('',#34177,#34174,#11561,.T.) ;
#42876=EDGE_CURVE('',#34178,#34179,#11562,.T.) ;
#42877=EDGE_CURVE('',#34179,#34180,#11563,.T.) ;
#42878=EDGE_CURVE('',#34180,#34181,#11564,.T.) ;
#42879=EDGE_CURVE('',#34181,#34178,#11565,.T.) ;
#42880=EDGE_CURVE('',#34182,#34183,#11566,.T.) ;
#42881=EDGE_CURVE('',#34183,#34184,#11567,.T.) ;
#42882=EDGE_CURVE('',#34185,#34184,#11568,.T.) ;
#42883=EDGE_CURVE('',#34185,#34182,#11569,.T.) ;
#42884=EDGE_CURVE('',#34186,#34187,#11570,.T.) ;
#42885=EDGE_CURVE('',#34187,#32249,#28839,.T.) ;
#42886=EDGE_CURVE('',#33937,#34188,#28840,.T.) ;
#42887=EDGE_CURVE('',#34188,#34189,#11571,.T.) ;
#42888=EDGE_CURVE('',#34189,#34186,#11572,.T.) ;
#42889=EDGE_CURVE('',#34190,#34191,#11573,.T.) ;
#42890=EDGE_CURVE('',#34191,#32072,#28841,.T.) ;
#42891=EDGE_CURVE('',#32071,#34192,#28842,.T.) ;
#42892=EDGE_CURVE('',#34192,#34193,#11574,.T.) ;
#42893=EDGE_CURVE('',#34193,#34190,#11575,.T.) ;
#42894=EDGE_CURVE('',#33935,#34167,#28843,.T.) ;
#42895=EDGE_CURVE('',#34166,#33936,#28844,.T.) ;
#42896=EDGE_CURVE('',#34184,#32251,#28845,.T.) ;
#42897=EDGE_CURVE('',#32250,#34185,#28846,.T.) ;
#42898=EDGE_CURVE('',#34194,#34195,#11576,.T.) ;
#42899=EDGE_CURVE('',#34195,#34196,#11577,.T.) ;
#42900=EDGE_CURVE('',#34196,#34197,#11578,.T.) ;
#42901=EDGE_CURVE('',#34197,#34194,#11579,.T.) ;
#42902=EDGE_CURVE('',#34198,#34199,#11580,.T.) ;
#42903=EDGE_CURVE('',#34199,#33865,#11581,.T.) ;
#42904=EDGE_CURVE('',#33864,#34198,#11582,.T.) ;
#42905=EDGE_CURVE('',#33868,#34200,#11583,.T.) ;
#42906=EDGE_CURVE('',#34200,#34201,#11584,.T.) ;
#42907=EDGE_CURVE('',#34201,#33869,#11585,.T.) ;
#42908=EDGE_CURVE('',#34202,#34203,#11586,.T.) ;
#42909=EDGE_CURVE('',#34203,#34204,#11587,.T.) ;
#42910=EDGE_CURVE('',#34204,#34205,#11588,.T.) ;
#42911=EDGE_CURVE('',#34205,#34202,#11589,.T.) ;
#42912=EDGE_CURVE('',#34206,#34207,#11590,.T.) ;
#42913=EDGE_CURVE('',#34207,#34208,#11591,.T.) ;
#42914=EDGE_CURVE('',#34208,#34209,#11592,.T.) ;
#42915=EDGE_CURVE('',#34209,#34206,#11593,.T.) ;
#42916=EDGE_CURVE('',#34210,#34211,#11594,.T.) ;
#42917=EDGE_CURVE('',#34211,#33862,#11595,.T.) ;
#42918=EDGE_CURVE('',#33863,#34210,#11596,.T.) ;
#42919=EDGE_CURVE('',#33866,#34212,#11597,.T.) ;
#42920=EDGE_CURVE('',#34212,#34213,#11598,.T.) ;
#42921=EDGE_CURVE('',#34213,#33867,#11599,.T.) ;
#42922=EDGE_CURVE('',#34214,#34215,#11600,.T.) ;
#42923=EDGE_CURVE('',#34215,#34216,#11601,.T.) ;
#42924=EDGE_CURVE('',#34216,#34217,#11602,.T.) ;
#42925=EDGE_CURVE('',#34217,#34214,#11603,.T.) ;
#42926=EDGE_CURVE('',#34218,#34219,#11604,.T.) ;
#42927=EDGE_CURVE('',#34219,#34220,#11605,.T.) ;
#42928=EDGE_CURVE('',#34220,#34221,#11606,.T.) ;
#42929=EDGE_CURVE('',#34221,#34218,#11607,.T.) ;
#42930=EDGE_CURVE('',#34222,#34223,#11608,.T.) ;
#42931=EDGE_CURVE('',#34223,#34224,#11609,.T.) ;
#42932=EDGE_CURVE('',#34224,#34225,#11610,.T.) ;
#42933=EDGE_CURVE('',#34225,#34222,#11611,.T.) ;
#42934=EDGE_CURVE('',#34226,#34227,#11612,.T.) ;
#42935=EDGE_CURVE('',#34227,#34228,#11613,.T.) ;
#42936=EDGE_CURVE('',#34228,#34229,#11614,.T.) ;
#42937=EDGE_CURVE('',#34229,#34226,#11615,.T.) ;
#42938=EDGE_CURVE('',#34230,#34231,#11616,.T.) ;
#42939=EDGE_CURVE('',#34231,#34232,#11617,.T.) ;
#42940=EDGE_CURVE('',#34233,#34232,#11618,.T.) ;
#42941=EDGE_CURVE('',#34233,#34230,#11619,.T.) ;
#42942=EDGE_CURVE('',#34234,#34235,#11620,.T.) ;
#42943=EDGE_CURVE('',#34235,#32239,#28847,.T.) ;
#42944=EDGE_CURVE('',#33945,#34236,#28848,.T.) ;
#42945=EDGE_CURVE('',#34236,#34237,#11621,.T.) ;
#42946=EDGE_CURVE('',#34237,#34234,#11622,.T.) ;
#42947=EDGE_CURVE('',#34238,#34239,#11623,.T.) ;
#42948=EDGE_CURVE('',#34239,#32057,#28849,.T.) ;
#42949=EDGE_CURVE('',#32056,#34240,#28850,.T.) ;
#42950=EDGE_CURVE('',#34240,#34241,#11624,.T.) ;
#42951=EDGE_CURVE('',#34241,#34238,#11625,.T.) ;
#42952=EDGE_CURVE('',#33943,#34215,#28851,.T.) ;
#42953=EDGE_CURVE('',#34214,#33944,#28852,.T.) ;
#42954=EDGE_CURVE('',#34232,#32241,#28853,.T.) ;
#42955=EDGE_CURVE('',#32240,#34233,#28854,.T.) ;
#42956=EDGE_CURVE('',#34242,#34243,#11626,.T.) ;
#42957=EDGE_CURVE('',#34243,#34244,#11627,.T.) ;
#42958=EDGE_CURVE('',#34244,#34245,#11628,.T.) ;
#42959=EDGE_CURVE('',#34245,#34242,#11629,.T.) ;
#42960=EDGE_CURVE('',#34246,#34247,#11630,.T.) ;
#42961=EDGE_CURVE('',#34247,#33873,#11631,.T.) ;
#42962=EDGE_CURVE('',#33872,#34246,#11632,.T.) ;
#42963=EDGE_CURVE('',#33876,#34248,#11633,.T.) ;
#42964=EDGE_CURVE('',#34248,#34249,#11634,.T.) ;
#42965=EDGE_CURVE('',#34249,#33877,#11635,.T.) ;
#42966=EDGE_CURVE('',#34250,#34251,#11636,.T.) ;
#42967=EDGE_CURVE('',#34251,#34252,#11637,.T.) ;
#42968=EDGE_CURVE('',#34252,#34253,#11638,.T.) ;
#42969=EDGE_CURVE('',#34253,#34250,#11639,.T.) ;
#42970=EDGE_CURVE('',#34254,#34255,#11640,.T.) ;
#42971=EDGE_CURVE('',#34255,#34256,#11641,.T.) ;
#42972=EDGE_CURVE('',#34256,#34257,#11642,.T.) ;
#42973=EDGE_CURVE('',#34257,#34254,#11643,.T.) ;
#42974=EDGE_CURVE('',#34258,#34259,#11644,.T.) ;
#42975=EDGE_CURVE('',#34259,#33870,#11645,.T.) ;
#42976=EDGE_CURVE('',#33871,#34258,#11646,.T.) ;
#42977=EDGE_CURVE('',#33874,#34260,#11647,.T.) ;
#42978=EDGE_CURVE('',#34260,#34261,#11648,.T.) ;
#42979=EDGE_CURVE('',#34261,#33875,#11649,.T.) ;
#42980=EDGE_CURVE('',#34262,#34263,#11650,.T.) ;
#42981=EDGE_CURVE('',#34263,#34264,#11651,.T.) ;
#42982=EDGE_CURVE('',#34264,#34265,#11652,.T.) ;
#42983=EDGE_CURVE('',#34265,#34262,#11653,.T.) ;
#42984=EDGE_CURVE('',#34266,#34267,#11654,.T.) ;
#42985=EDGE_CURVE('',#34267,#34268,#11655,.T.) ;
#42986=EDGE_CURVE('',#34268,#34269,#11656,.T.) ;
#42987=EDGE_CURVE('',#34269,#34266,#11657,.T.) ;
#42988=EDGE_CURVE('',#34270,#34271,#11658,.T.) ;
#42989=EDGE_CURVE('',#34271,#34272,#11659,.T.) ;
#42990=EDGE_CURVE('',#34272,#34273,#11660,.T.) ;
#42991=EDGE_CURVE('',#34273,#34270,#11661,.T.) ;
#42992=EDGE_CURVE('',#34274,#34275,#11662,.T.) ;
#42993=EDGE_CURVE('',#34275,#34276,#11663,.T.) ;
#42994=EDGE_CURVE('',#34276,#34277,#11664,.T.) ;
#42995=EDGE_CURVE('',#34277,#34274,#11665,.T.) ;
#42996=EDGE_CURVE('',#34278,#34279,#11666,.T.) ;
#42997=EDGE_CURVE('',#34279,#34280,#11667,.T.) ;
#42998=EDGE_CURVE('',#34281,#34280,#11668,.T.) ;
#42999=EDGE_CURVE('',#34281,#34278,#11669,.T.) ;
#43000=EDGE_CURVE('',#34282,#34283,#11670,.T.) ;
#43001=EDGE_CURVE('',#34283,#32229,#28855,.T.) ;
#43002=EDGE_CURVE('',#33953,#34284,#28856,.T.) ;
#43003=EDGE_CURVE('',#34284,#34285,#11671,.T.) ;
#43004=EDGE_CURVE('',#34285,#34282,#11672,.T.) ;
#43005=EDGE_CURVE('',#34286,#34287,#11673,.T.) ;
#43006=EDGE_CURVE('',#34287,#32042,#28857,.T.) ;
#43007=EDGE_CURVE('',#32041,#34288,#28858,.T.) ;
#43008=EDGE_CURVE('',#34288,#34289,#11674,.T.) ;
#43009=EDGE_CURVE('',#34289,#34286,#11675,.T.) ;
#43010=EDGE_CURVE('',#33951,#34263,#28859,.T.) ;
#43011=EDGE_CURVE('',#34262,#33952,#28860,.T.) ;
#43012=EDGE_CURVE('',#34280,#32231,#28861,.T.) ;
#43013=EDGE_CURVE('',#32230,#34281,#28862,.T.) ;
#43014=EDGE_CURVE('',#34290,#34291,#11676,.T.) ;
#43015=EDGE_CURVE('',#34291,#34292,#11677,.T.) ;
#43016=EDGE_CURVE('',#34292,#34293,#11678,.T.) ;
#43017=EDGE_CURVE('',#34293,#34290,#11679,.T.) ;
#43018=EDGE_CURVE('',#34294,#34295,#11680,.T.) ;
#43019=EDGE_CURVE('',#34295,#33881,#11681,.T.) ;
#43020=EDGE_CURVE('',#33880,#34294,#11682,.T.) ;
#43021=EDGE_CURVE('',#33884,#34296,#11683,.T.) ;
#43022=EDGE_CURVE('',#34296,#34297,#11684,.T.) ;
#43023=EDGE_CURVE('',#34297,#33885,#11685,.T.) ;
#43024=EDGE_CURVE('',#34298,#34299,#11686,.T.) ;
#43025=EDGE_CURVE('',#34299,#34300,#11687,.T.) ;
#43026=EDGE_CURVE('',#34300,#34301,#11688,.T.) ;
#43027=EDGE_CURVE('',#34301,#34298,#11689,.T.) ;
#43028=EDGE_CURVE('',#34302,#34303,#11690,.T.) ;
#43029=EDGE_CURVE('',#34303,#34304,#11691,.T.) ;
#43030=EDGE_CURVE('',#34304,#34305,#11692,.T.) ;
#43031=EDGE_CURVE('',#34305,#34302,#11693,.T.) ;
#43032=EDGE_CURVE('',#34306,#34307,#11694,.T.) ;
#43033=EDGE_CURVE('',#34307,#33878,#11695,.T.) ;
#43034=EDGE_CURVE('',#33879,#34306,#11696,.T.) ;
#43035=EDGE_CURVE('',#33882,#34308,#11697,.T.) ;
#43036=EDGE_CURVE('',#34308,#34309,#11698,.T.) ;
#43037=EDGE_CURVE('',#34309,#33883,#11699,.T.) ;
#43038=EDGE_CURVE('',#34310,#34311,#11700,.T.) ;
#43039=EDGE_CURVE('',#34311,#34312,#11701,.T.) ;
#43040=EDGE_CURVE('',#34312,#34313,#11702,.T.) ;
#43041=EDGE_CURVE('',#34313,#34310,#11703,.T.) ;
#43042=EDGE_CURVE('',#34314,#34315,#11704,.T.) ;
#43043=EDGE_CURVE('',#34315,#34316,#11705,.T.) ;
#43044=EDGE_CURVE('',#34316,#34317,#11706,.T.) ;
#43045=EDGE_CURVE('',#34317,#34314,#11707,.T.) ;
#43046=EDGE_CURVE('',#34318,#34319,#11708,.T.) ;
#43047=EDGE_CURVE('',#34319,#34320,#11709,.T.) ;
#43048=EDGE_CURVE('',#34320,#34321,#11710,.T.) ;
#43049=EDGE_CURVE('',#34321,#34318,#11711,.T.) ;
#43050=EDGE_CURVE('',#34322,#34323,#11712,.T.) ;
#43051=EDGE_CURVE('',#34323,#34324,#11713,.T.) ;
#43052=EDGE_CURVE('',#34324,#34325,#11714,.T.) ;
#43053=EDGE_CURVE('',#34325,#34322,#11715,.T.) ;
#43054=EDGE_CURVE('',#34326,#34327,#11716,.T.) ;
#43055=EDGE_CURVE('',#34327,#34328,#11717,.T.) ;
#43056=EDGE_CURVE('',#34329,#34328,#11718,.T.) ;
#43057=EDGE_CURVE('',#34329,#34326,#11719,.T.) ;
#43058=EDGE_CURVE('',#34330,#34331,#11720,.T.) ;
#43059=EDGE_CURVE('',#34331,#32219,#28863,.T.) ;
#43060=EDGE_CURVE('',#33961,#34332,#28864,.T.) ;
#43061=EDGE_CURVE('',#34332,#34333,#11721,.T.) ;
#43062=EDGE_CURVE('',#34333,#34330,#11722,.T.) ;
#43063=EDGE_CURVE('',#34334,#34335,#11723,.T.) ;
#43064=EDGE_CURVE('',#34335,#32027,#28865,.T.) ;
#43065=EDGE_CURVE('',#32026,#34336,#28866,.T.) ;
#43066=EDGE_CURVE('',#34336,#34337,#11724,.T.) ;
#43067=EDGE_CURVE('',#34337,#34334,#11725,.T.) ;
#43068=EDGE_CURVE('',#33959,#34311,#28867,.T.) ;
#43069=EDGE_CURVE('',#34310,#33960,#28868,.T.) ;
#43070=EDGE_CURVE('',#34328,#32221,#28869,.T.) ;
#43071=EDGE_CURVE('',#32220,#34329,#28870,.T.) ;
#43072=EDGE_CURVE('',#34338,#34339,#11726,.T.) ;
#43073=EDGE_CURVE('',#34339,#34340,#11727,.T.) ;
#43074=EDGE_CURVE('',#34340,#34341,#11728,.T.) ;
#43075=EDGE_CURVE('',#34341,#34338,#11729,.T.) ;
#43076=EDGE_CURVE('',#34342,#34343,#11730,.T.) ;
#43077=EDGE_CURVE('',#34343,#33889,#11731,.T.) ;
#43078=EDGE_CURVE('',#33888,#34342,#11732,.T.) ;
#43079=EDGE_CURVE('',#33892,#34344,#11733,.T.) ;
#43080=EDGE_CURVE('',#34344,#34345,#11734,.T.) ;
#43081=EDGE_CURVE('',#34345,#33893,#11735,.T.) ;
#43082=EDGE_CURVE('',#34346,#34347,#11736,.T.) ;
#43083=EDGE_CURVE('',#34347,#34348,#11737,.T.) ;
#43084=EDGE_CURVE('',#34348,#34349,#11738,.T.) ;
#43085=EDGE_CURVE('',#34349,#34346,#11739,.T.) ;
#43086=EDGE_CURVE('',#34350,#34351,#11740,.T.) ;
#43087=EDGE_CURVE('',#34351,#34352,#11741,.T.) ;
#43088=EDGE_CURVE('',#34352,#34353,#11742,.T.) ;
#43089=EDGE_CURVE('',#34353,#34350,#11743,.T.) ;
#43090=EDGE_CURVE('',#34354,#34355,#11744,.T.) ;
#43091=EDGE_CURVE('',#34355,#33886,#11745,.T.) ;
#43092=EDGE_CURVE('',#33887,#34354,#11746,.T.) ;
#43093=EDGE_CURVE('',#33890,#34356,#11747,.T.) ;
#43094=EDGE_CURVE('',#34356,#34357,#11748,.T.) ;
#43095=EDGE_CURVE('',#34357,#33891,#11749,.T.) ;
#43096=EDGE_CURVE('',#34358,#34359,#11750,.T.) ;
#43097=EDGE_CURVE('',#34359,#34360,#11751,.T.) ;
#43098=EDGE_CURVE('',#34360,#34361,#11752,.T.) ;
#43099=EDGE_CURVE('',#34361,#34358,#11753,.T.) ;
#43100=EDGE_CURVE('',#34362,#34363,#11754,.T.) ;
#43101=EDGE_CURVE('',#34363,#34364,#11755,.T.) ;
#43102=EDGE_CURVE('',#34364,#34365,#11756,.T.) ;
#43103=EDGE_CURVE('',#34365,#34362,#11757,.T.) ;
#43104=EDGE_CURVE('',#34366,#34367,#11758,.T.) ;
#43105=EDGE_CURVE('',#34367,#34368,#11759,.T.) ;
#43106=EDGE_CURVE('',#34368,#34369,#11760,.T.) ;
#43107=EDGE_CURVE('',#34369,#34366,#11761,.T.) ;
#43108=EDGE_CURVE('',#34370,#34371,#11762,.T.) ;
#43109=EDGE_CURVE('',#34371,#34372,#11763,.T.) ;
#43110=EDGE_CURVE('',#34372,#34373,#11764,.T.) ;
#43111=EDGE_CURVE('',#34373,#34370,#11765,.T.) ;
#43112=EDGE_CURVE('',#34374,#34375,#11766,.T.) ;
#43113=EDGE_CURVE('',#34375,#34376,#11767,.T.) ;
#43114=EDGE_CURVE('',#34377,#34376,#11768,.T.) ;
#43115=EDGE_CURVE('',#34377,#34374,#11769,.T.) ;
#43116=EDGE_CURVE('',#34378,#34379,#11770,.T.) ;
#43117=EDGE_CURVE('',#34379,#32209,#28871,.T.) ;
#43118=EDGE_CURVE('',#33969,#34380,#28872,.T.) ;
#43119=EDGE_CURVE('',#34380,#34381,#11771,.T.) ;
#43120=EDGE_CURVE('',#34381,#34378,#11772,.T.) ;
#43121=EDGE_CURVE('',#34382,#34383,#11773,.T.) ;
#43122=EDGE_CURVE('',#34383,#32012,#28873,.T.) ;
#43123=EDGE_CURVE('',#32011,#34384,#28874,.T.) ;
#43124=EDGE_CURVE('',#34384,#34385,#11774,.T.) ;
#43125=EDGE_CURVE('',#34385,#34382,#11775,.T.) ;
#43126=EDGE_CURVE('',#33967,#34359,#28875,.T.) ;
#43127=EDGE_CURVE('',#34358,#33968,#28876,.T.) ;
#43128=EDGE_CURVE('',#34376,#32211,#28877,.T.) ;
#43129=EDGE_CURVE('',#32210,#34377,#28878,.T.) ;
#43130=EDGE_CURVE('',#34386,#34387,#11776,.T.) ;
#43131=EDGE_CURVE('',#34387,#34388,#11777,.T.) ;
#43132=EDGE_CURVE('',#34388,#34389,#11778,.T.) ;
#43133=EDGE_CURVE('',#34389,#34386,#11779,.T.) ;
#43134=EDGE_CURVE('',#34390,#34391,#11780,.T.) ;
#43135=EDGE_CURVE('',#34391,#33897,#11781,.T.) ;
#43136=EDGE_CURVE('',#33896,#34390,#11782,.T.) ;
#43137=EDGE_CURVE('',#33900,#34392,#11783,.T.) ;
#43138=EDGE_CURVE('',#34392,#34393,#11784,.T.) ;
#43139=EDGE_CURVE('',#34393,#33901,#11785,.T.) ;
#43140=EDGE_CURVE('',#34394,#34395,#11786,.T.) ;
#43141=EDGE_CURVE('',#34395,#34396,#11787,.T.) ;
#43142=EDGE_CURVE('',#34396,#34397,#11788,.T.) ;
#43143=EDGE_CURVE('',#34397,#34394,#11789,.T.) ;
#43144=EDGE_CURVE('',#34398,#34399,#11790,.T.) ;
#43145=EDGE_CURVE('',#34399,#34400,#11791,.T.) ;
#43146=EDGE_CURVE('',#34400,#34401,#11792,.T.) ;
#43147=EDGE_CURVE('',#34401,#34398,#11793,.T.) ;
#43148=EDGE_CURVE('',#34402,#34403,#11794,.T.) ;
#43149=EDGE_CURVE('',#34403,#33894,#11795,.T.) ;
#43150=EDGE_CURVE('',#33895,#34402,#11796,.T.) ;
#43151=EDGE_CURVE('',#33898,#34404,#11797,.T.) ;
#43152=EDGE_CURVE('',#34404,#34405,#11798,.T.) ;
#43153=EDGE_CURVE('',#34405,#33899,#11799,.T.) ;
#43154=EDGE_CURVE('',#34406,#34407,#11800,.T.) ;
#43155=EDGE_CURVE('',#34407,#34408,#11801,.T.) ;
#43156=EDGE_CURVE('',#34408,#34409,#11802,.T.) ;
#43157=EDGE_CURVE('',#34409,#34406,#11803,.T.) ;
#43158=EDGE_CURVE('',#34410,#34411,#11804,.T.) ;
#43159=EDGE_CURVE('',#34411,#34412,#11805,.T.) ;
#43160=EDGE_CURVE('',#34412,#34413,#11806,.T.) ;
#43161=EDGE_CURVE('',#34413,#34410,#11807,.T.) ;
#43162=EDGE_CURVE('',#34414,#34415,#11808,.T.) ;
#43163=EDGE_CURVE('',#34415,#34416,#11809,.T.) ;
#43164=EDGE_CURVE('',#34416,#34417,#11810,.T.) ;
#43165=EDGE_CURVE('',#34417,#34414,#11811,.T.) ;
#43166=EDGE_CURVE('',#34418,#34419,#11812,.T.) ;
#43167=EDGE_CURVE('',#34419,#34420,#11813,.T.) ;
#43168=EDGE_CURVE('',#34420,#34421,#11814,.T.) ;
#43169=EDGE_CURVE('',#34421,#34418,#11815,.T.) ;
#43170=EDGE_CURVE('',#34422,#34423,#11816,.T.) ;
#43171=EDGE_CURVE('',#34423,#34424,#11817,.T.) ;
#43172=EDGE_CURVE('',#34424,#34425,#11818,.T.) ;
#43173=EDGE_CURVE('',#34425,#34422,#11819,.T.) ;
#43174=EDGE_CURVE('',#34426,#34427,#11820,.T.) ;
#43175=EDGE_CURVE('',#34427,#34428,#11821,.T.) ;
#43176=EDGE_CURVE('',#34428,#34429,#11822,.T.) ;
#43177=EDGE_CURVE('',#34429,#34426,#11823,.T.) ;
#43178=EDGE_CURVE('',#34430,#34431,#11824,.T.) ;
#43179=EDGE_CURVE('',#34431,#34432,#11825,.T.) ;
#43180=EDGE_CURVE('',#34432,#34433,#11826,.T.) ;
#43181=EDGE_CURVE('',#34433,#34430,#11827,.T.) ;
#43182=EDGE_CURVE('',#34434,#34435,#11828,.T.) ;
#43183=EDGE_CURVE('',#34435,#34436,#11829,.T.) ;
#43184=EDGE_CURVE('',#34436,#34437,#11830,.T.) ;
#43185=EDGE_CURVE('',#34437,#34434,#11831,.T.) ;
#43186=EDGE_CURVE('',#34438,#34439,#11832,.T.) ;
#43187=EDGE_CURVE('',#34439,#34440,#11833,.T.) ;
#43188=EDGE_CURVE('',#34440,#34441,#11834,.T.) ;
#43189=EDGE_CURVE('',#34441,#34438,#11835,.T.) ;
#43190=EDGE_CURVE('',#34442,#34443,#11836,.T.) ;
#43191=EDGE_CURVE('',#34443,#34444,#11837,.T.) ;
#43192=EDGE_CURVE('',#34444,#34445,#11838,.T.) ;
#43193=EDGE_CURVE('',#34445,#34442,#11839,.T.) ;
#43194=EDGE_CURVE('',#34446,#34447,#11840,.T.) ;
#43195=EDGE_CURVE('',#34447,#34448,#11841,.T.) ;
#43196=EDGE_CURVE('',#34448,#34449,#11842,.T.) ;
#43197=EDGE_CURVE('',#34449,#34446,#11843,.T.) ;
#43198=EDGE_CURVE('',#34450,#34451,#11844,.T.) ;
#43199=EDGE_CURVE('',#34451,#34452,#11845,.T.) ;
#43200=EDGE_CURVE('',#34452,#34453,#11846,.T.) ;
#43201=EDGE_CURVE('',#34453,#34450,#11847,.T.) ;
#43202=EDGE_CURVE('',#34454,#34455,#11848,.T.) ;
#43203=EDGE_CURVE('',#34455,#34456,#11849,.T.) ;
#43204=EDGE_CURVE('',#34456,#34457,#11850,.T.) ;
#43205=EDGE_CURVE('',#34457,#34454,#11851,.T.) ;
#43206=EDGE_CURVE('',#34458,#34459,#11852,.T.) ;
#43207=EDGE_CURVE('',#34459,#34460,#11853,.T.) ;
#43208=EDGE_CURVE('',#34460,#34461,#11854,.T.) ;
#43209=EDGE_CURVE('',#34461,#34458,#11855,.T.) ;
#43210=EDGE_CURVE('',#34462,#34463,#11856,.T.) ;
#43211=EDGE_CURVE('',#34463,#34464,#11857,.T.) ;
#43212=EDGE_CURVE('',#34464,#34465,#11858,.T.) ;
#43213=EDGE_CURVE('',#34465,#34462,#11859,.T.) ;
#43214=EDGE_CURVE('',#34466,#34467,#11860,.T.) ;
#43215=EDGE_CURVE('',#34467,#34468,#11861,.T.) ;
#43216=EDGE_CURVE('',#34468,#34469,#11862,.T.) ;
#43217=EDGE_CURVE('',#34469,#34466,#11863,.T.) ;
#43218=EDGE_CURVE('',#34470,#34471,#11864,.T.) ;
#43219=EDGE_CURVE('',#34471,#34472,#11865,.T.) ;
#43220=EDGE_CURVE('',#34472,#34473,#11866,.T.) ;
#43221=EDGE_CURVE('',#34473,#34470,#11867,.T.) ;
#43222=EDGE_CURVE('',#34474,#34475,#11868,.T.) ;
#43223=EDGE_CURVE('',#34475,#34476,#11869,.T.) ;
#43224=EDGE_CURVE('',#34476,#34477,#11870,.T.) ;
#43225=EDGE_CURVE('',#34477,#34474,#11871,.T.) ;
#43226=EDGE_CURVE('',#34478,#34479,#11872,.T.) ;
#43227=EDGE_CURVE('',#34479,#34480,#11873,.T.) ;
#43228=EDGE_CURVE('',#34480,#34481,#11874,.T.) ;
#43229=EDGE_CURVE('',#34481,#34478,#11875,.T.) ;
#43230=EDGE_CURVE('',#34482,#34483,#11876,.T.) ;
#43231=EDGE_CURVE('',#34483,#34484,#11877,.T.) ;
#43232=EDGE_CURVE('',#34484,#34485,#11878,.T.) ;
#43233=EDGE_CURVE('',#34485,#34482,#11879,.T.) ;
#43234=EDGE_CURVE('',#34486,#34487,#11880,.T.) ;
#43235=EDGE_CURVE('',#34487,#34488,#11881,.T.) ;
#43236=EDGE_CURVE('',#34488,#34489,#11882,.T.) ;
#43237=EDGE_CURVE('',#34489,#34486,#11883,.T.) ;
#43238=EDGE_CURVE('',#34490,#34491,#11884,.T.) ;
#43239=EDGE_CURVE('',#34491,#34492,#11885,.T.) ;
#43240=EDGE_CURVE('',#34492,#34493,#11886,.T.) ;
#43241=EDGE_CURVE('',#34493,#34490,#11887,.T.) ;
#43242=EDGE_CURVE('',#34494,#34495,#11888,.T.) ;
#43243=EDGE_CURVE('',#34495,#34496,#11889,.T.) ;
#43244=EDGE_CURVE('',#34496,#34497,#11890,.T.) ;
#43245=EDGE_CURVE('',#34497,#34494,#11891,.T.) ;
#43246=EDGE_CURVE('',#34498,#34499,#11892,.T.) ;
#43247=EDGE_CURVE('',#34499,#34500,#11893,.T.) ;
#43248=EDGE_CURVE('',#34500,#34501,#11894,.T.) ;
#43249=EDGE_CURVE('',#34501,#34498,#11895,.T.) ;
#43250=EDGE_CURVE('',#34502,#34503,#11896,.T.) ;
#43251=EDGE_CURVE('',#34503,#34504,#11897,.T.) ;
#43252=EDGE_CURVE('',#34504,#34505,#11898,.T.) ;
#43253=EDGE_CURVE('',#34505,#34502,#11899,.T.) ;
#43254=EDGE_CURVE('',#34506,#34507,#11900,.T.) ;
#43255=EDGE_CURVE('',#34507,#34508,#11901,.T.) ;
#43256=EDGE_CURVE('',#34508,#34509,#11902,.T.) ;
#43257=EDGE_CURVE('',#34509,#34506,#11903,.T.) ;
#43258=EDGE_CURVE('',#34510,#34511,#11904,.T.) ;
#43259=EDGE_CURVE('',#34511,#34512,#11905,.T.) ;
#43260=EDGE_CURVE('',#34512,#34513,#11906,.T.) ;
#43261=EDGE_CURVE('',#34513,#34510,#11907,.T.) ;
#43262=EDGE_CURVE('',#34514,#34515,#11908,.T.) ;
#43263=EDGE_CURVE('',#34515,#34516,#11909,.T.) ;
#43264=EDGE_CURVE('',#34516,#34517,#11910,.T.) ;
#43265=EDGE_CURVE('',#34517,#34514,#11911,.T.) ;
#43266=EDGE_CURVE('',#34518,#34519,#11912,.T.) ;
#43267=EDGE_CURVE('',#34519,#34520,#11913,.T.) ;
#43268=EDGE_CURVE('',#34520,#34521,#11914,.T.) ;
#43269=EDGE_CURVE('',#34521,#34518,#11915,.T.) ;
#43270=EDGE_CURVE('',#34522,#34523,#11916,.T.) ;
#43271=EDGE_CURVE('',#34523,#34524,#11917,.T.) ;
#43272=EDGE_CURVE('',#34524,#34525,#11918,.T.) ;
#43273=EDGE_CURVE('',#34525,#34522,#11919,.T.) ;
#43274=EDGE_CURVE('',#34526,#34527,#11920,.T.) ;
#43275=EDGE_CURVE('',#34527,#34528,#11921,.T.) ;
#43276=EDGE_CURVE('',#34528,#34529,#11922,.T.) ;
#43277=EDGE_CURVE('',#34529,#34526,#11923,.T.) ;
#43278=EDGE_CURVE('',#34530,#34531,#11924,.T.) ;
#43279=EDGE_CURVE('',#34531,#34532,#11925,.T.) ;
#43280=EDGE_CURVE('',#34532,#34533,#11926,.T.) ;
#43281=EDGE_CURVE('',#34533,#34530,#11927,.T.) ;
#43282=EDGE_CURVE('',#34534,#34535,#11928,.T.) ;
#43283=EDGE_CURVE('',#34535,#34536,#11929,.T.) ;
#43284=EDGE_CURVE('',#34536,#34537,#11930,.T.) ;
#43285=EDGE_CURVE('',#34537,#34534,#11931,.T.) ;
#43286=EDGE_CURVE('',#34538,#34539,#11932,.T.) ;
#43287=EDGE_CURVE('',#34539,#34540,#11933,.T.) ;
#43288=EDGE_CURVE('',#34540,#34541,#11934,.T.) ;
#43289=EDGE_CURVE('',#34541,#34538,#11935,.T.) ;
#43290=EDGE_CURVE('',#34542,#34543,#11936,.T.) ;
#43291=EDGE_CURVE('',#34543,#34544,#11937,.T.) ;
#43292=EDGE_CURVE('',#34544,#34545,#11938,.T.) ;
#43293=EDGE_CURVE('',#34545,#34542,#11939,.T.) ;
#43294=EDGE_CURVE('',#34546,#34547,#11940,.T.) ;
#43295=EDGE_CURVE('',#34547,#34548,#11941,.T.) ;
#43296=EDGE_CURVE('',#34548,#34549,#11942,.T.) ;
#43297=EDGE_CURVE('',#34549,#34546,#11943,.T.) ;
#43298=EDGE_CURVE('',#34472,#33986,#28879,.T.) ;
#43299=EDGE_CURVE('',#34473,#33989,#28880,.T.) ;
#43300=EDGE_CURVE('',#33986,#33991,#28881,.T.) ;
#43301=EDGE_CURVE('',#33990,#33987,#28882,.T.) ;
#43302=EDGE_CURVE('',#34473,#33982,#28883,.T.) ;
#43303=EDGE_CURVE('',#33982,#33989,#28884,.T.) ;
#43304=EDGE_CURVE('',#33987,#34475,#28885,.T.) ;
#43305=EDGE_CURVE('',#33988,#34474,#28886,.T.) ;
#43306=EDGE_CURVE('',#33983,#33988,#28887,.T.) ;
#43307=EDGE_CURVE('',#34470,#33985,#28888,.T.) ;
#43308=EDGE_CURVE('',#33983,#34474,#28889,.T.) ;
#43309=EDGE_CURVE('',#34470,#33978,#28890,.T.) ;
#43310=EDGE_CURVE('',#33978,#33985,#28891,.T.) ;
#43311=EDGE_CURVE('',#33984,#34477,#28892,.T.) ;
#43312=EDGE_CURVE('',#33979,#33984,#28893,.T.) ;
#43313=EDGE_CURVE('',#33981,#34471,#28894,.T.) ;
#43314=EDGE_CURVE('',#33979,#34477,#28895,.T.) ;
#43315=EDGE_CURVE('',#33976,#33981,#28896,.T.) ;
#43316=EDGE_CURVE('',#33980,#33977,#28897,.T.) ;
#43317=EDGE_CURVE('',#34476,#33980,#28898,.T.) ;
#43318=EDGE_CURVE('',#34544,#34002,#28899,.T.) ;
#43319=EDGE_CURVE('',#34545,#34005,#28900,.T.) ;
#43320=EDGE_CURVE('',#34002,#34007,#28901,.T.) ;
#43321=EDGE_CURVE('',#34006,#34003,#28902,.T.) ;
#43322=EDGE_CURVE('',#34545,#34016,#28903,.T.) ;
#43323=EDGE_CURVE('',#34016,#34005,#28904,.T.) ;
#43324=EDGE_CURVE('',#34003,#34547,#28905,.T.) ;
#43325=EDGE_CURVE('',#34004,#34546,#28906,.T.) ;
#43326=EDGE_CURVE('',#34017,#34004,#28907,.T.) ;
#43327=EDGE_CURVE('',#34542,#34015,#28908,.T.) ;
#43328=EDGE_CURVE('',#34017,#34546,#28909,.T.) ;
#43329=EDGE_CURVE('',#34542,#34010,#28910,.T.) ;
#43330=EDGE_CURVE('',#34010,#34015,#28911,.T.) ;
#43331=EDGE_CURVE('',#34014,#34549,#28912,.T.) ;
#43332=EDGE_CURVE('',#34011,#34014,#28913,.T.) ;
#43333=EDGE_CURVE('',#34013,#34543,#28914,.T.) ;
#43334=EDGE_CURVE('',#34011,#34549,#28915,.T.) ;
#43335=EDGE_CURVE('',#34008,#34013,#28916,.T.) ;
#43336=EDGE_CURVE('',#34012,#34009,#28917,.T.) ;
#43337=EDGE_CURVE('',#34548,#34012,#28918,.T.) ;
#43338=EDGE_CURVE('',#34464,#34034,#28919,.T.) ;
#43339=EDGE_CURVE('',#34465,#34037,#28920,.T.) ;
#43340=EDGE_CURVE('',#34034,#34039,#28921,.T.) ;
#43341=EDGE_CURVE('',#34038,#34035,#28922,.T.) ;
#43342=EDGE_CURVE('',#34465,#34030,#28923,.T.) ;
#43343=EDGE_CURVE('',#34030,#34037,#28924,.T.) ;
#43344=EDGE_CURVE('',#34035,#34467,#28925,.T.) ;
#43345=EDGE_CURVE('',#34036,#34466,#28926,.T.) ;
#43346=EDGE_CURVE('',#34031,#34036,#28927,.T.) ;
#43347=EDGE_CURVE('',#34462,#34033,#28928,.T.) ;
#43348=EDGE_CURVE('',#34031,#34466,#28929,.T.) ;
#43349=EDGE_CURVE('',#34462,#34026,#28930,.T.) ;
#43350=EDGE_CURVE('',#34026,#34033,#28931,.T.) ;
#43351=EDGE_CURVE('',#34032,#34469,#28932,.T.) ;
#43352=EDGE_CURVE('',#34027,#34032,#28933,.T.) ;
#43353=EDGE_CURVE('',#34029,#34463,#28934,.T.) ;
#43354=EDGE_CURVE('',#34027,#34469,#28935,.T.) ;
#43355=EDGE_CURVE('',#34024,#34029,#28936,.T.) ;
#43356=EDGE_CURVE('',#34028,#34025,#28937,.T.) ;
#43357=EDGE_CURVE('',#34468,#34028,#28938,.T.) ;
#43358=EDGE_CURVE('',#34536,#34050,#28939,.T.) ;
#43359=EDGE_CURVE('',#34537,#34053,#28940,.T.) ;
#43360=EDGE_CURVE('',#34050,#34055,#28941,.T.) ;
#43361=EDGE_CURVE('',#34054,#34051,#28942,.T.) ;
#43362=EDGE_CURVE('',#34537,#34064,#28943,.T.) ;
#43363=EDGE_CURVE('',#34064,#34053,#28944,.T.) ;
#43364=EDGE_CURVE('',#34051,#34539,#28945,.T.) ;
#43365=EDGE_CURVE('',#34052,#34538,#28946,.T.) ;
#43366=EDGE_CURVE('',#34065,#34052,#28947,.T.) ;
#43367=EDGE_CURVE('',#34534,#34063,#28948,.T.) ;
#43368=EDGE_CURVE('',#34065,#34538,#28949,.T.) ;
#43369=EDGE_CURVE('',#34534,#34058,#28950,.T.) ;
#43370=EDGE_CURVE('',#34058,#34063,#28951,.T.) ;
#43371=EDGE_CURVE('',#34062,#34541,#28952,.T.) ;
#43372=EDGE_CURVE('',#34059,#34062,#28953,.T.) ;
#43373=EDGE_CURVE('',#34061,#34535,#28954,.T.) ;
#43374=EDGE_CURVE('',#34059,#34541,#28955,.T.) ;
#43375=EDGE_CURVE('',#34056,#34061,#28956,.T.) ;
#43376=EDGE_CURVE('',#34060,#34057,#28957,.T.) ;
#43377=EDGE_CURVE('',#34540,#34060,#28958,.T.) ;
#43378=EDGE_CURVE('',#34456,#34082,#28959,.T.) ;
#43379=EDGE_CURVE('',#34457,#34085,#28960,.T.) ;
#43380=EDGE_CURVE('',#34082,#34087,#28961,.T.) ;
#43381=EDGE_CURVE('',#34086,#34083,#28962,.T.) ;
#43382=EDGE_CURVE('',#34457,#34078,#28963,.T.) ;
#43383=EDGE_CURVE('',#34078,#34085,#28964,.T.) ;
#43384=EDGE_CURVE('',#34083,#34459,#28965,.T.) ;
#43385=EDGE_CURVE('',#34084,#34458,#28966,.T.) ;
#43386=EDGE_CURVE('',#34079,#34084,#28967,.T.) ;
#43387=EDGE_CURVE('',#34454,#34081,#28968,.T.) ;
#43388=EDGE_CURVE('',#34079,#34458,#28969,.T.) ;
#43389=EDGE_CURVE('',#34454,#34074,#28970,.T.) ;
#43390=EDGE_CURVE('',#34074,#34081,#28971,.T.) ;
#43391=EDGE_CURVE('',#34080,#34461,#28972,.T.) ;
#43392=EDGE_CURVE('',#34075,#34080,#28973,.T.) ;
#43393=EDGE_CURVE('',#34077,#34455,#28974,.T.) ;
#43394=EDGE_CURVE('',#34075,#34461,#28975,.T.) ;
#43395=EDGE_CURVE('',#34072,#34077,#28976,.T.) ;
#43396=EDGE_CURVE('',#34076,#34073,#28977,.T.) ;
#43397=EDGE_CURVE('',#34460,#34076,#28978,.T.) ;
#43398=EDGE_CURVE('',#34528,#34098,#28979,.T.) ;
#43399=EDGE_CURVE('',#34529,#34101,#28980,.T.) ;
#43400=EDGE_CURVE('',#34098,#34103,#28981,.T.) ;
#43401=EDGE_CURVE('',#34102,#34099,#28982,.T.) ;
#43402=EDGE_CURVE('',#34529,#34112,#28983,.T.) ;
#43403=EDGE_CURVE('',#34112,#34101,#28984,.T.) ;
#43404=EDGE_CURVE('',#34099,#34531,#28985,.T.) ;
#43405=EDGE_CURVE('',#34100,#34530,#28986,.T.) ;
#43406=EDGE_CURVE('',#34113,#34100,#28987,.T.) ;
#43407=EDGE_CURVE('',#34526,#34111,#28988,.T.) ;
#43408=EDGE_CURVE('',#34113,#34530,#28989,.T.) ;
#43409=EDGE_CURVE('',#34526,#34106,#28990,.T.) ;
#43410=EDGE_CURVE('',#34106,#34111,#28991,.T.) ;
#43411=EDGE_CURVE('',#34110,#34533,#28992,.T.) ;
#43412=EDGE_CURVE('',#34107,#34110,#28993,.T.) ;
#43413=EDGE_CURVE('',#34109,#34527,#28994,.T.) ;
#43414=EDGE_CURVE('',#34107,#34533,#28995,.T.) ;
#43415=EDGE_CURVE('',#34104,#34109,#28996,.T.) ;
#43416=EDGE_CURVE('',#34108,#34105,#28997,.T.) ;
#43417=EDGE_CURVE('',#34532,#34108,#28998,.T.) ;
#43418=EDGE_CURVE('',#34448,#34130,#28999,.T.) ;
#43419=EDGE_CURVE('',#34449,#34133,#29000,.T.) ;
#43420=EDGE_CURVE('',#34130,#34135,#29001,.T.) ;
#43421=EDGE_CURVE('',#34134,#34131,#29002,.T.) ;
#43422=EDGE_CURVE('',#34449,#34126,#29003,.T.) ;
#43423=EDGE_CURVE('',#34126,#34133,#29004,.T.) ;
#43424=EDGE_CURVE('',#34131,#34451,#29005,.T.) ;
#43425=EDGE_CURVE('',#34132,#34450,#29006,.T.) ;
#43426=EDGE_CURVE('',#34127,#34132,#29007,.T.) ;
#43427=EDGE_CURVE('',#34446,#34129,#29008,.T.) ;
#43428=EDGE_CURVE('',#34127,#34450,#29009,.T.) ;
#43429=EDGE_CURVE('',#34446,#34122,#29010,.T.) ;
#43430=EDGE_CURVE('',#34122,#34129,#29011,.T.) ;
#43431=EDGE_CURVE('',#34128,#34453,#29012,.T.) ;
#43432=EDGE_CURVE('',#34123,#34128,#29013,.T.) ;
#43433=EDGE_CURVE('',#34125,#34447,#29014,.T.) ;
#43434=EDGE_CURVE('',#34123,#34453,#29015,.T.) ;
#43435=EDGE_CURVE('',#34120,#34125,#29016,.T.) ;
#43436=EDGE_CURVE('',#34124,#34121,#29017,.T.) ;
#43437=EDGE_CURVE('',#34452,#34124,#29018,.T.) ;
#43438=EDGE_CURVE('',#34520,#34146,#29019,.T.) ;
#43439=EDGE_CURVE('',#34521,#34149,#29020,.T.) ;
#43440=EDGE_CURVE('',#34146,#34151,#29021,.T.) ;
#43441=EDGE_CURVE('',#34150,#34147,#29022,.T.) ;
#43442=EDGE_CURVE('',#34521,#34160,#29023,.T.) ;
#43443=EDGE_CURVE('',#34160,#34149,#29024,.T.) ;
#43444=EDGE_CURVE('',#34147,#34523,#29025,.T.) ;
#43445=EDGE_CURVE('',#34148,#34522,#29026,.T.) ;
#43446=EDGE_CURVE('',#34161,#34148,#29027,.T.) ;
#43447=EDGE_CURVE('',#34518,#34159,#29028,.T.) ;
#43448=EDGE_CURVE('',#34161,#34522,#29029,.T.) ;
#43449=EDGE_CURVE('',#34518,#34154,#29030,.T.) ;
#43450=EDGE_CURVE('',#34154,#34159,#29031,.T.) ;
#43451=EDGE_CURVE('',#34158,#34525,#29032,.T.) ;
#43452=EDGE_CURVE('',#34155,#34158,#29033,.T.) ;
#43453=EDGE_CURVE('',#34157,#34519,#29034,.T.) ;
#43454=EDGE_CURVE('',#34155,#34525,#29035,.T.) ;
#43455=EDGE_CURVE('',#34152,#34157,#29036,.T.) ;
#43456=EDGE_CURVE('',#34156,#34153,#29037,.T.) ;
#43457=EDGE_CURVE('',#34524,#34156,#29038,.T.) ;
#43458=EDGE_CURVE('',#34440,#34178,#29039,.T.) ;
#43459=EDGE_CURVE('',#34441,#34181,#29040,.T.) ;
#43460=EDGE_CURVE('',#34178,#34183,#29041,.T.) ;
#43461=EDGE_CURVE('',#34182,#34179,#29042,.T.) ;
#43462=EDGE_CURVE('',#34441,#34174,#29043,.T.) ;
#43463=EDGE_CURVE('',#34174,#34181,#29044,.T.) ;
#43464=EDGE_CURVE('',#34179,#34443,#29045,.T.) ;
#43465=EDGE_CURVE('',#34180,#34442,#29046,.T.) ;
#43466=EDGE_CURVE('',#34175,#34180,#29047,.T.) ;
#43467=EDGE_CURVE('',#34438,#34177,#29048,.T.) ;
#43468=EDGE_CURVE('',#34175,#34442,#29049,.T.) ;
#43469=EDGE_CURVE('',#34438,#34170,#29050,.T.) ;
#43470=EDGE_CURVE('',#34170,#34177,#29051,.T.) ;
#43471=EDGE_CURVE('',#34176,#34445,#29052,.T.) ;
#43472=EDGE_CURVE('',#34171,#34176,#29053,.T.) ;
#43473=EDGE_CURVE('',#34173,#34439,#29054,.T.) ;
#43474=EDGE_CURVE('',#34171,#34445,#29055,.T.) ;
#43475=EDGE_CURVE('',#34168,#34173,#29056,.T.) ;
#43476=EDGE_CURVE('',#34172,#34169,#29057,.T.) ;
#43477=EDGE_CURVE('',#34444,#34172,#29058,.T.) ;
#43478=EDGE_CURVE('',#34512,#34194,#29059,.T.) ;
#43479=EDGE_CURVE('',#34513,#34197,#29060,.T.) ;
#43480=EDGE_CURVE('',#34194,#34199,#29061,.T.) ;
#43481=EDGE_CURVE('',#34198,#34195,#29062,.T.) ;
#43482=EDGE_CURVE('',#34513,#34208,#29063,.T.) ;
#43483=EDGE_CURVE('',#34208,#34197,#29064,.T.) ;
#43484=EDGE_CURVE('',#34195,#34515,#29065,.T.) ;
#43485=EDGE_CURVE('',#34196,#34514,#29066,.T.) ;
#43486=EDGE_CURVE('',#34209,#34196,#29067,.T.) ;
#43487=EDGE_CURVE('',#34510,#34207,#29068,.T.) ;
#43488=EDGE_CURVE('',#34209,#34514,#29069,.T.) ;
#43489=EDGE_CURVE('',#34510,#34202,#29070,.T.) ;
#43490=EDGE_CURVE('',#34202,#34207,#29071,.T.) ;
#43491=EDGE_CURVE('',#34206,#34517,#29072,.T.) ;
#43492=EDGE_CURVE('',#34203,#34206,#29073,.T.) ;
#43493=EDGE_CURVE('',#34205,#34511,#29074,.T.) ;
#43494=EDGE_CURVE('',#34203,#34517,#29075,.T.) ;
#43495=EDGE_CURVE('',#34200,#34205,#29076,.T.) ;
#43496=EDGE_CURVE('',#34204,#34201,#29077,.T.) ;
#43497=EDGE_CURVE('',#34516,#34204,#29078,.T.) ;
#43498=EDGE_CURVE('',#34432,#34226,#29079,.T.) ;
#43499=EDGE_CURVE('',#34433,#34229,#29080,.T.) ;
#43500=EDGE_CURVE('',#34226,#34231,#29081,.T.) ;
#43501=EDGE_CURVE('',#34230,#34227,#29082,.T.) ;
#43502=EDGE_CURVE('',#34433,#34222,#29083,.T.) ;
#43503=EDGE_CURVE('',#34222,#34229,#29084,.T.) ;
#43504=EDGE_CURVE('',#34227,#34435,#29085,.T.) ;
#43505=EDGE_CURVE('',#34228,#34434,#29086,.T.) ;
#43506=EDGE_CURVE('',#34223,#34228,#29087,.T.) ;
#43507=EDGE_CURVE('',#34430,#34225,#29088,.T.) ;
#43508=EDGE_CURVE('',#34223,#34434,#29089,.T.) ;
#43509=EDGE_CURVE('',#34430,#34218,#29090,.T.) ;
#43510=EDGE_CURVE('',#34218,#34225,#29091,.T.) ;
#43511=EDGE_CURVE('',#34224,#34437,#29092,.T.) ;
#43512=EDGE_CURVE('',#34219,#34224,#29093,.T.) ;
#43513=EDGE_CURVE('',#34221,#34431,#29094,.T.) ;
#43514=EDGE_CURVE('',#34219,#34437,#29095,.T.) ;
#43515=EDGE_CURVE('',#34216,#34221,#29096,.T.) ;
#43516=EDGE_CURVE('',#34220,#34217,#29097,.T.) ;
#43517=EDGE_CURVE('',#34436,#34220,#29098,.T.) ;
#43518=EDGE_CURVE('',#34504,#34242,#29099,.T.) ;
#43519=EDGE_CURVE('',#34505,#34245,#29100,.T.) ;
#43520=EDGE_CURVE('',#34242,#34247,#29101,.T.) ;
#43521=EDGE_CURVE('',#34246,#34243,#29102,.T.) ;
#43522=EDGE_CURVE('',#34505,#34256,#29103,.T.) ;
#43523=EDGE_CURVE('',#34256,#34245,#29104,.T.) ;
#43524=EDGE_CURVE('',#34243,#34507,#29105,.T.) ;
#43525=EDGE_CURVE('',#34244,#34506,#29106,.T.) ;
#43526=EDGE_CURVE('',#34257,#34244,#29107,.T.) ;
#43527=EDGE_CURVE('',#34502,#34255,#29108,.T.) ;
#43528=EDGE_CURVE('',#34257,#34506,#29109,.T.) ;
#43529=EDGE_CURVE('',#34502,#34250,#29110,.T.) ;
#43530=EDGE_CURVE('',#34250,#34255,#29111,.T.) ;
#43531=EDGE_CURVE('',#34254,#34509,#29112,.T.) ;
#43532=EDGE_CURVE('',#34251,#34254,#29113,.T.) ;
#43533=EDGE_CURVE('',#34253,#34503,#29114,.T.) ;
#43534=EDGE_CURVE('',#34251,#34509,#29115,.T.) ;
#43535=EDGE_CURVE('',#34248,#34253,#29116,.T.) ;
#43536=EDGE_CURVE('',#34252,#34249,#29117,.T.) ;
#43537=EDGE_CURVE('',#34508,#34252,#29118,.T.) ;
#43538=EDGE_CURVE('',#34424,#34274,#29119,.T.) ;
#43539=EDGE_CURVE('',#34425,#34277,#29120,.T.) ;
#43540=EDGE_CURVE('',#34274,#34279,#29121,.T.) ;
#43541=EDGE_CURVE('',#34278,#34275,#29122,.T.) ;
#43542=EDGE_CURVE('',#34425,#34270,#29123,.T.) ;
#43543=EDGE_CURVE('',#34270,#34277,#29124,.T.) ;
#43544=EDGE_CURVE('',#34275,#34427,#29125,.T.) ;
#43545=EDGE_CURVE('',#34276,#34426,#29126,.T.) ;
#43546=EDGE_CURVE('',#34271,#34276,#29127,.T.) ;
#43547=EDGE_CURVE('',#34422,#34273,#29128,.T.) ;
#43548=EDGE_CURVE('',#34271,#34426,#29129,.T.) ;
#43549=EDGE_CURVE('',#34422,#34266,#29130,.T.) ;
#43550=EDGE_CURVE('',#34266,#34273,#29131,.T.) ;
#43551=EDGE_CURVE('',#34272,#34429,#29132,.T.) ;
#43552=EDGE_CURVE('',#34267,#34272,#29133,.T.) ;
#43553=EDGE_CURVE('',#34269,#34423,#29134,.T.) ;
#43554=EDGE_CURVE('',#34267,#34429,#29135,.T.) ;
#43555=EDGE_CURVE('',#34264,#34269,#29136,.T.) ;
#43556=EDGE_CURVE('',#34268,#34265,#29137,.T.) ;
#43557=EDGE_CURVE('',#34428,#34268,#29138,.T.) ;
#43558=EDGE_CURVE('',#34496,#34290,#29139,.T.) ;
#43559=EDGE_CURVE('',#34497,#34293,#29140,.T.) ;
#43560=EDGE_CURVE('',#34290,#34295,#29141,.T.) ;
#43561=EDGE_CURVE('',#34294,#34291,#29142,.T.) ;
#43562=EDGE_CURVE('',#34497,#34304,#29143,.T.) ;
#43563=EDGE_CURVE('',#34304,#34293,#29144,.T.) ;
#43564=EDGE_CURVE('',#34291,#34499,#29145,.T.) ;
#43565=EDGE_CURVE('',#34292,#34498,#29146,.T.) ;
#43566=EDGE_CURVE('',#34305,#34292,#29147,.T.) ;
#43567=EDGE_CURVE('',#34494,#34303,#29148,.T.) ;
#43568=EDGE_CURVE('',#34305,#34498,#29149,.T.) ;
#43569=EDGE_CURVE('',#34494,#34298,#29150,.T.) ;
#43570=EDGE_CURVE('',#34298,#34303,#29151,.T.) ;
#43571=EDGE_CURVE('',#34302,#34501,#29152,.T.) ;
#43572=EDGE_CURVE('',#34299,#34302,#29153,.T.) ;
#43573=EDGE_CURVE('',#34301,#34495,#29154,.T.) ;
#43574=EDGE_CURVE('',#34299,#34501,#29155,.T.) ;
#43575=EDGE_CURVE('',#34296,#34301,#29156,.T.) ;
#43576=EDGE_CURVE('',#34300,#34297,#29157,.T.) ;
#43577=EDGE_CURVE('',#34500,#34300,#29158,.T.) ;
#43578=EDGE_CURVE('',#34416,#34322,#29159,.T.) ;
#43579=EDGE_CURVE('',#34417,#34325,#29160,.T.) ;
#43580=EDGE_CURVE('',#34322,#34327,#29161,.T.) ;
#43581=EDGE_CURVE('',#34326,#34323,#29162,.T.) ;
#43582=EDGE_CURVE('',#34417,#34318,#29163,.T.) ;
#43583=EDGE_CURVE('',#34318,#34325,#29164,.T.) ;
#43584=EDGE_CURVE('',#34323,#34419,#29165,.T.) ;
#43585=EDGE_CURVE('',#34324,#34418,#29166,.T.) ;
#43586=EDGE_CURVE('',#34319,#34324,#29167,.T.) ;
#43587=EDGE_CURVE('',#34414,#34321,#29168,.T.) ;
#43588=EDGE_CURVE('',#34319,#34418,#29169,.T.) ;
#43589=EDGE_CURVE('',#34414,#34314,#29170,.T.) ;
#43590=EDGE_CURVE('',#34314,#34321,#29171,.T.) ;
#43591=EDGE_CURVE('',#34320,#34421,#29172,.T.) ;
#43592=EDGE_CURVE('',#34315,#34320,#29173,.T.) ;
#43593=EDGE_CURVE('',#34317,#34415,#29174,.T.) ;
#43594=EDGE_CURVE('',#34315,#34421,#29175,.T.) ;
#43595=EDGE_CURVE('',#34312,#34317,#29176,.T.) ;
#43596=EDGE_CURVE('',#34316,#34313,#29177,.T.) ;
#43597=EDGE_CURVE('',#34420,#34316,#29178,.T.) ;
#43598=EDGE_CURVE('',#34488,#34338,#29179,.T.) ;
#43599=EDGE_CURVE('',#34489,#34341,#29180,.T.) ;
#43600=EDGE_CURVE('',#34338,#34343,#29181,.T.) ;
#43601=EDGE_CURVE('',#34342,#34339,#29182,.T.) ;
#43602=EDGE_CURVE('',#34489,#34352,#29183,.T.) ;
#43603=EDGE_CURVE('',#34352,#34341,#29184,.T.) ;
#43604=EDGE_CURVE('',#34339,#34491,#29185,.T.) ;
#43605=EDGE_CURVE('',#34340,#34490,#29186,.T.) ;
#43606=EDGE_CURVE('',#34353,#34340,#29187,.T.) ;
#43607=EDGE_CURVE('',#34486,#34351,#29188,.T.) ;
#43608=EDGE_CURVE('',#34353,#34490,#29189,.T.) ;
#43609=EDGE_CURVE('',#34486,#34346,#29190,.T.) ;
#43610=EDGE_CURVE('',#34346,#34351,#29191,.T.) ;
#43611=EDGE_CURVE('',#34350,#34493,#29192,.T.) ;
#43612=EDGE_CURVE('',#34347,#34350,#29193,.T.) ;
#43613=EDGE_CURVE('',#34349,#34487,#29194,.T.) ;
#43614=EDGE_CURVE('',#34347,#34493,#29195,.T.) ;
#43615=EDGE_CURVE('',#34344,#34349,#29196,.T.) ;
#43616=EDGE_CURVE('',#34348,#34345,#29197,.T.) ;
#43617=EDGE_CURVE('',#34492,#34348,#29198,.T.) ;
#43618=EDGE_CURVE('',#34408,#34370,#29199,.T.) ;
#43619=EDGE_CURVE('',#34409,#34373,#29200,.T.) ;
#43620=EDGE_CURVE('',#34370,#34375,#29201,.T.) ;
#43621=EDGE_CURVE('',#34374,#34371,#29202,.T.) ;
#43622=EDGE_CURVE('',#34409,#34366,#29203,.T.) ;
#43623=EDGE_CURVE('',#34366,#34373,#29204,.T.) ;
#43624=EDGE_CURVE('',#34371,#34411,#29205,.T.) ;
#43625=EDGE_CURVE('',#34372,#34410,#29206,.T.) ;
#43626=EDGE_CURVE('',#34367,#34372,#29207,.T.) ;
#43627=EDGE_CURVE('',#34406,#34369,#29208,.T.) ;
#43628=EDGE_CURVE('',#34367,#34410,#29209,.T.) ;
#43629=EDGE_CURVE('',#34406,#34362,#29210,.T.) ;
#43630=EDGE_CURVE('',#34362,#34369,#29211,.T.) ;
#43631=EDGE_CURVE('',#34368,#34413,#29212,.T.) ;
#43632=EDGE_CURVE('',#34363,#34368,#29213,.T.) ;
#43633=EDGE_CURVE('',#34365,#34407,#29214,.T.) ;
#43634=EDGE_CURVE('',#34363,#34413,#29215,.T.) ;
#43635=EDGE_CURVE('',#34360,#34365,#29216,.T.) ;
#43636=EDGE_CURVE('',#34364,#34361,#29217,.T.) ;
#43637=EDGE_CURVE('',#34412,#34364,#29218,.T.) ;
#43638=EDGE_CURVE('',#34480,#34386,#29219,.T.) ;
#43639=EDGE_CURVE('',#34481,#34389,#29220,.T.) ;
#43640=EDGE_CURVE('',#34386,#34391,#29221,.T.) ;
#43641=EDGE_CURVE('',#34390,#34387,#29222,.T.) ;
#43642=EDGE_CURVE('',#34481,#34400,#29223,.T.) ;
#43643=EDGE_CURVE('',#34400,#34389,#29224,.T.) ;
#43644=EDGE_CURVE('',#34387,#34483,#29225,.T.) ;
#43645=EDGE_CURVE('',#34388,#34482,#29226,.T.) ;
#43646=EDGE_CURVE('',#34401,#34388,#29227,.T.) ;
#43647=EDGE_CURVE('',#34478,#34399,#29228,.T.) ;
#43648=EDGE_CURVE('',#34401,#34482,#29229,.T.) ;
#43649=EDGE_CURVE('',#34478,#34394,#29230,.T.) ;
#43650=EDGE_CURVE('',#34394,#34399,#29231,.T.) ;
#43651=EDGE_CURVE('',#34398,#34485,#29232,.T.) ;
#43652=EDGE_CURVE('',#34395,#34398,#29233,.T.) ;
#43653=EDGE_CURVE('',#34397,#34479,#29234,.T.) ;
#43654=EDGE_CURVE('',#34395,#34485,#29235,.T.) ;
#43655=EDGE_CURVE('',#34392,#34397,#29236,.T.) ;
#43656=EDGE_CURVE('',#34396,#34393,#29237,.T.) ;
#43657=EDGE_CURVE('',#34484,#34396,#29238,.T.) ;
#43658=EDGE_CURVE('',#34000,#33992,#29239,.T.) ;
#43659=EDGE_CURVE('',#34001,#33991,#29240,.T.) ;
#43660=EDGE_CURVE('',#34001,#34472,#29241,.T.) ;
#43661=EDGE_CURVE('',#33998,#34471,#29242,.T.) ;
#43662=EDGE_CURVE('',#33998,#33976,#29243,.T.) ;
#43663=EDGE_CURVE('',#33999,#33975,#29244,.T.) ;
#43664=EDGE_CURVE('',#33996,#33974,#29245,.T.) ;
#43665=EDGE_CURVE('',#33997,#33977,#29246,.T.) ;
#43666=EDGE_CURVE('',#33997,#34476,#29247,.T.) ;
#43667=EDGE_CURVE('',#33994,#34475,#29248,.T.) ;
#43668=EDGE_CURVE('',#33994,#33990,#29249,.T.) ;
#43669=EDGE_CURVE('',#33995,#33993,#29250,.T.) ;
#43670=EDGE_CURVE('',#34020,#34007,#29251,.T.) ;
#43671=EDGE_CURVE('',#34020,#34544,#29252,.T.) ;
#43672=EDGE_CURVE('',#34021,#34543,#29253,.T.) ;
#43673=EDGE_CURVE('',#34021,#34008,#29254,.T.) ;
#43674=EDGE_CURVE('',#34006,#34019,#29255,.T.) ;
#43675=EDGE_CURVE('',#34547,#34019,#29256,.T.) ;
#43676=EDGE_CURVE('',#34548,#34018,#29257,.T.) ;
#43677=EDGE_CURVE('',#34018,#34009,#29258,.T.) ;
#43678=EDGE_CURVE('',#34048,#34040,#29259,.T.) ;
#43679=EDGE_CURVE('',#34049,#34039,#29260,.T.) ;
#43680=EDGE_CURVE('',#34049,#34464,#29261,.T.) ;
#43681=EDGE_CURVE('',#34046,#34463,#29262,.T.) ;
#43682=EDGE_CURVE('',#34046,#34024,#29263,.T.) ;
#43683=EDGE_CURVE('',#34047,#34023,#29264,.T.) ;
#43684=EDGE_CURVE('',#34044,#34022,#29265,.T.) ;
#43685=EDGE_CURVE('',#34045,#34025,#29266,.T.) ;
#43686=EDGE_CURVE('',#34045,#34468,#29267,.T.) ;
#43687=EDGE_CURVE('',#34042,#34467,#29268,.T.) ;
#43688=EDGE_CURVE('',#34042,#34038,#29269,.T.) ;
#43689=EDGE_CURVE('',#34043,#34041,#29270,.T.) ;
#43690=EDGE_CURVE('',#34068,#34055,#29271,.T.) ;
#43691=EDGE_CURVE('',#34068,#34536,#29272,.T.) ;
#43692=EDGE_CURVE('',#34069,#34535,#29273,.T.) ;
#43693=EDGE_CURVE('',#34069,#34056,#29274,.T.) ;
#43694=EDGE_CURVE('',#34054,#34067,#29275,.T.) ;
#43695=EDGE_CURVE('',#34539,#34067,#29276,.T.) ;
#43696=EDGE_CURVE('',#34540,#34066,#29277,.T.) ;
#43697=EDGE_CURVE('',#34066,#34057,#29278,.T.) ;
#43698=EDGE_CURVE('',#34096,#34088,#29279,.T.) ;
#43699=EDGE_CURVE('',#34097,#34087,#29280,.T.) ;
#43700=EDGE_CURVE('',#34097,#34456,#29281,.T.) ;
#43701=EDGE_CURVE('',#34094,#34455,#29282,.T.) ;
#43702=EDGE_CURVE('',#34094,#34072,#29283,.T.) ;
#43703=EDGE_CURVE('',#34095,#34071,#29284,.T.) ;
#43704=EDGE_CURVE('',#34092,#34070,#29285,.T.) ;
#43705=EDGE_CURVE('',#34093,#34073,#29286,.T.) ;
#43706=EDGE_CURVE('',#34093,#34460,#29287,.T.) ;
#43707=EDGE_CURVE('',#34090,#34459,#29288,.T.) ;
#43708=EDGE_CURVE('',#34090,#34086,#29289,.T.) ;
#43709=EDGE_CURVE('',#34091,#34089,#29290,.T.) ;
#43710=EDGE_CURVE('',#34116,#34103,#29291,.T.) ;
#43711=EDGE_CURVE('',#34116,#34528,#29292,.T.) ;
#43712=EDGE_CURVE('',#34117,#34527,#29293,.T.) ;
#43713=EDGE_CURVE('',#34117,#34104,#29294,.T.) ;
#43714=EDGE_CURVE('',#34102,#34115,#29295,.T.) ;
#43715=EDGE_CURVE('',#34531,#34115,#29296,.T.) ;
#43716=EDGE_CURVE('',#34532,#34114,#29297,.T.) ;
#43717=EDGE_CURVE('',#34114,#34105,#29298,.T.) ;
#43718=EDGE_CURVE('',#34144,#34136,#29299,.T.) ;
#43719=EDGE_CURVE('',#34145,#34135,#29300,.T.) ;
#43720=EDGE_CURVE('',#34145,#34448,#29301,.T.) ;
#43721=EDGE_CURVE('',#34142,#34447,#29302,.T.) ;
#43722=EDGE_CURVE('',#34142,#34120,#29303,.T.) ;
#43723=EDGE_CURVE('',#34143,#34119,#29304,.T.) ;
#43724=EDGE_CURVE('',#34140,#34118,#29305,.T.) ;
#43725=EDGE_CURVE('',#34141,#34121,#29306,.T.) ;
#43726=EDGE_CURVE('',#34141,#34452,#29307,.T.) ;
#43727=EDGE_CURVE('',#34138,#34451,#29308,.T.) ;
#43728=EDGE_CURVE('',#34138,#34134,#29309,.T.) ;
#43729=EDGE_CURVE('',#34139,#34137,#29310,.T.) ;
#43730=EDGE_CURVE('',#34164,#34151,#29311,.T.) ;
#43731=EDGE_CURVE('',#34164,#34520,#29312,.T.) ;
#43732=EDGE_CURVE('',#34165,#34519,#29313,.T.) ;
#43733=EDGE_CURVE('',#34165,#34152,#29314,.T.) ;
#43734=EDGE_CURVE('',#34150,#34163,#29315,.T.) ;
#43735=EDGE_CURVE('',#34523,#34163,#29316,.T.) ;
#43736=EDGE_CURVE('',#34524,#34162,#29317,.T.) ;
#43737=EDGE_CURVE('',#34162,#34153,#29318,.T.) ;
#43738=EDGE_CURVE('',#34192,#34184,#29319,.T.) ;
#43739=EDGE_CURVE('',#34193,#34183,#29320,.T.) ;
#43740=EDGE_CURVE('',#34193,#34440,#29321,.T.) ;
#43741=EDGE_CURVE('',#34190,#34439,#29322,.T.) ;
#43742=EDGE_CURVE('',#34190,#34168,#29323,.T.) ;
#43743=EDGE_CURVE('',#34191,#34167,#29324,.T.) ;
#43744=EDGE_CURVE('',#34188,#34166,#29325,.T.) ;
#43745=EDGE_CURVE('',#34189,#34169,#29326,.T.) ;
#43746=EDGE_CURVE('',#34189,#34444,#29327,.T.) ;
#43747=EDGE_CURVE('',#34186,#34443,#29328,.T.) ;
#43748=EDGE_CURVE('',#34186,#34182,#29329,.T.) ;
#43749=EDGE_CURVE('',#34187,#34185,#29330,.T.) ;
#43750=EDGE_CURVE('',#34212,#34199,#29331,.T.) ;
#43751=EDGE_CURVE('',#34212,#34512,#29332,.T.) ;
#43752=EDGE_CURVE('',#34213,#34511,#29333,.T.) ;
#43753=EDGE_CURVE('',#34213,#34200,#29334,.T.) ;
#43754=EDGE_CURVE('',#34198,#34211,#29335,.T.) ;
#43755=EDGE_CURVE('',#34515,#34211,#29336,.T.) ;
#43756=EDGE_CURVE('',#34516,#34210,#29337,.T.) ;
#43757=EDGE_CURVE('',#34210,#34201,#29338,.T.) ;
#43758=EDGE_CURVE('',#34240,#34232,#29339,.T.) ;
#43759=EDGE_CURVE('',#34241,#34231,#29340,.T.) ;
#43760=EDGE_CURVE('',#34241,#34432,#29341,.T.) ;
#43761=EDGE_CURVE('',#34238,#34431,#29342,.T.) ;
#43762=EDGE_CURVE('',#34238,#34216,#29343,.T.) ;
#43763=EDGE_CURVE('',#34239,#34215,#29344,.T.) ;
#43764=EDGE_CURVE('',#34236,#34214,#29345,.T.) ;
#43765=EDGE_CURVE('',#34237,#34217,#29346,.T.) ;
#43766=EDGE_CURVE('',#34237,#34436,#29347,.T.) ;
#43767=EDGE_CURVE('',#34234,#34435,#29348,.T.) ;
#43768=EDGE_CURVE('',#34234,#34230,#29349,.T.) ;
#43769=EDGE_CURVE('',#34235,#34233,#29350,.T.) ;
#43770=EDGE_CURVE('',#34260,#34247,#29351,.T.) ;
#43771=EDGE_CURVE('',#34260,#34504,#29352,.T.) ;
#43772=EDGE_CURVE('',#34261,#34503,#29353,.T.) ;
#43773=EDGE_CURVE('',#34261,#34248,#29354,.T.) ;
#43774=EDGE_CURVE('',#34246,#34259,#29355,.T.) ;
#43775=EDGE_CURVE('',#34507,#34259,#29356,.T.) ;
#43776=EDGE_CURVE('',#34508,#34258,#29357,.T.) ;
#43777=EDGE_CURVE('',#34258,#34249,#29358,.T.) ;
#43778=EDGE_CURVE('',#34288,#34280,#29359,.T.) ;
#43779=EDGE_CURVE('',#34289,#34279,#29360,.T.) ;
#43780=EDGE_CURVE('',#34289,#34424,#29361,.T.) ;
#43781=EDGE_CURVE('',#34286,#34423,#29362,.T.) ;
#43782=EDGE_CURVE('',#34286,#34264,#29363,.T.) ;
#43783=EDGE_CURVE('',#34287,#34263,#29364,.T.) ;
#43784=EDGE_CURVE('',#34284,#34262,#29365,.T.) ;
#43785=EDGE_CURVE('',#34285,#34265,#29366,.T.) ;
#43786=EDGE_CURVE('',#34285,#34428,#29367,.T.) ;
#43787=EDGE_CURVE('',#34282,#34427,#29368,.T.) ;
#43788=EDGE_CURVE('',#34282,#34278,#29369,.T.) ;
#43789=EDGE_CURVE('',#34283,#34281,#29370,.T.) ;
#43790=EDGE_CURVE('',#34308,#34295,#29371,.T.) ;
#43791=EDGE_CURVE('',#34308,#34496,#29372,.T.) ;
#43792=EDGE_CURVE('',#34309,#34495,#29373,.T.) ;
#43793=EDGE_CURVE('',#34309,#34296,#29374,.T.) ;
#43794=EDGE_CURVE('',#34294,#34307,#29375,.T.) ;
#43795=EDGE_CURVE('',#34499,#34307,#29376,.T.) ;
#43796=EDGE_CURVE('',#34500,#34306,#29377,.T.) ;
#43797=EDGE_CURVE('',#34306,#34297,#29378,.T.) ;
#43798=EDGE_CURVE('',#34336,#34328,#29379,.T.) ;
#43799=EDGE_CURVE('',#34337,#34327,#29380,.T.) ;
#43800=EDGE_CURVE('',#34337,#34416,#29381,.T.) ;
#43801=EDGE_CURVE('',#34334,#34415,#29382,.T.) ;
#43802=EDGE_CURVE('',#34334,#34312,#29383,.T.) ;
#43803=EDGE_CURVE('',#34335,#34311,#29384,.T.) ;
#43804=EDGE_CURVE('',#34332,#34310,#29385,.T.) ;
#43805=EDGE_CURVE('',#34333,#34313,#29386,.T.) ;
#43806=EDGE_CURVE('',#34333,#34420,#29387,.T.) ;
#43807=EDGE_CURVE('',#34330,#34419,#29388,.T.) ;
#43808=EDGE_CURVE('',#34330,#34326,#29389,.T.) ;
#43809=EDGE_CURVE('',#34331,#34329,#29390,.T.) ;
#43810=EDGE_CURVE('',#34356,#34343,#29391,.T.) ;
#43811=EDGE_CURVE('',#34356,#34488,#29392,.T.) ;
#43812=EDGE_CURVE('',#34357,#34487,#29393,.T.) ;
#43813=EDGE_CURVE('',#34357,#34344,#29394,.T.) ;
#43814=EDGE_CURVE('',#34342,#34355,#29395,.T.) ;
#43815=EDGE_CURVE('',#34491,#34355,#29396,.T.) ;
#43816=EDGE_CURVE('',#34492,#34354,#29397,.T.) ;
#43817=EDGE_CURVE('',#34354,#34345,#29398,.T.) ;
#43818=EDGE_CURVE('',#34384,#34376,#29399,.T.) ;
#43819=EDGE_CURVE('',#34385,#34375,#29400,.T.) ;
#43820=EDGE_CURVE('',#34385,#34408,#29401,.T.) ;
#43821=EDGE_CURVE('',#34382,#34407,#29402,.T.) ;
#43822=EDGE_CURVE('',#34382,#34360,#29403,.T.) ;
#43823=EDGE_CURVE('',#34383,#34359,#29404,.T.) ;
#43824=EDGE_CURVE('',#34380,#34358,#29405,.T.) ;
#43825=EDGE_CURVE('',#34381,#34361,#29406,.T.) ;
#43826=EDGE_CURVE('',#34381,#34412,#29407,.T.) ;
#43827=EDGE_CURVE('',#34378,#34411,#29408,.T.) ;
#43828=EDGE_CURVE('',#34378,#34374,#29409,.T.) ;
#43829=EDGE_CURVE('',#34379,#34377,#29410,.T.) ;
#43830=EDGE_CURVE('',#34404,#34391,#29411,.T.) ;
#43831=EDGE_CURVE('',#34404,#34480,#29412,.T.) ;
#43832=EDGE_CURVE('',#34405,#34479,#29413,.T.) ;
#43833=EDGE_CURVE('',#34405,#34392,#29414,.T.) ;
#43834=EDGE_CURVE('',#34390,#34403,#29415,.T.) ;
#43835=EDGE_CURVE('',#34483,#34403,#29416,.T.) ;
#43836=EDGE_CURVE('',#34484,#34402,#29417,.T.) ;
#43837=EDGE_CURVE('',#34402,#34393,#29418,.T.) ;
#52858=ORIENTED_EDGE('',*,*,#39088,.F.) ;
#52859=ORIENTED_EDGE('',*,*,#39089,.T.) ;
#52860=ORIENTED_EDGE('',*,*,#39090,.F.) ;
#52861=ORIENTED_EDGE('',*,*,#39091,.F.) ;
#52862=ORIENTED_EDGE('',*,*,#39089,.F.) ;
#52863=ORIENTED_EDGE('',*,*,#39092,.F.) ;
#52864=ORIENTED_EDGE('',*,*,#39093,.T.) ;
#52865=ORIENTED_EDGE('',*,*,#39094,.F.) ;
#52866=ORIENTED_EDGE('',*,*,#39093,.F.) ;
#52867=ORIENTED_EDGE('',*,*,#39095,.F.) ;
#52868=ORIENTED_EDGE('',*,*,#39096,.F.) ;
#52869=ORIENTED_EDGE('',*,*,#39097,.T.) ;
#52870=ORIENTED_EDGE('',*,*,#39098,.F.) ;
#52871=ORIENTED_EDGE('',*,*,#39099,.T.) ;
#52872=ORIENTED_EDGE('',*,*,#39100,.F.) ;
#52873=ORIENTED_EDGE('',*,*,#39101,.F.) ;
#52874=ORIENTED_EDGE('',*,*,#39102,.F.) ;
#52875=ORIENTED_EDGE('',*,*,#39103,.F.) ;
#52876=ORIENTED_EDGE('',*,*,#39104,.T.) ;
#52877=ORIENTED_EDGE('',*,*,#39105,.F.) ;
#52878=ORIENTED_EDGE('',*,*,#39106,.T.) ;
#52879=ORIENTED_EDGE('',*,*,#39107,.F.) ;
#52880=ORIENTED_EDGE('',*,*,#39108,.F.) ;
#52881=ORIENTED_EDGE('',*,*,#39106,.F.) ;
#52882=ORIENTED_EDGE('',*,*,#39109,.F.) ;
#52883=ORIENTED_EDGE('',*,*,#39110,.T.) ;
#52884=ORIENTED_EDGE('',*,*,#39111,.F.) ;
#52885=ORIENTED_EDGE('',*,*,#39110,.F.) ;
#52886=ORIENTED_EDGE('',*,*,#39112,.F.) ;
#52887=ORIENTED_EDGE('',*,*,#39113,.F.) ;
#52888=ORIENTED_EDGE('',*,*,#39114,.T.) ;
#52889=ORIENTED_EDGE('',*,*,#39115,.F.) ;
#52890=ORIENTED_EDGE('',*,*,#39116,.T.) ;
#52891=ORIENTED_EDGE('',*,*,#39117,.F.) ;
#52892=ORIENTED_EDGE('',*,*,#39118,.F.) ;
#52893=ORIENTED_EDGE('',*,*,#39119,.F.) ;
#52894=ORIENTED_EDGE('',*,*,#39120,.F.) ;
#52895=ORIENTED_EDGE('',*,*,#39121,.T.) ;
#52896=ORIENTED_EDGE('',*,*,#39122,.F.) ;
#52897=ORIENTED_EDGE('',*,*,#39123,.T.) ;
#52898=ORIENTED_EDGE('',*,*,#39124,.F.) ;
#52899=ORIENTED_EDGE('',*,*,#39125,.F.) ;
#52900=ORIENTED_EDGE('',*,*,#39123,.F.) ;
#52901=ORIENTED_EDGE('',*,*,#39126,.F.) ;
#52902=ORIENTED_EDGE('',*,*,#39127,.T.) ;
#52903=ORIENTED_EDGE('',*,*,#39128,.F.) ;
#52904=ORIENTED_EDGE('',*,*,#39127,.F.) ;
#52905=ORIENTED_EDGE('',*,*,#39129,.F.) ;
#52906=ORIENTED_EDGE('',*,*,#39130,.F.) ;
#52907=ORIENTED_EDGE('',*,*,#39131,.T.) ;
#52908=ORIENTED_EDGE('',*,*,#39132,.F.) ;
#52909=ORIENTED_EDGE('',*,*,#39133,.T.) ;
#52910=ORIENTED_EDGE('',*,*,#39134,.F.) ;
#52911=ORIENTED_EDGE('',*,*,#39135,.F.) ;
#52912=ORIENTED_EDGE('',*,*,#39136,.F.) ;
#52913=ORIENTED_EDGE('',*,*,#39137,.F.) ;
#52914=ORIENTED_EDGE('',*,*,#39138,.T.) ;
#52915=ORIENTED_EDGE('',*,*,#39139,.F.) ;
#52916=ORIENTED_EDGE('',*,*,#39140,.T.) ;
#52917=ORIENTED_EDGE('',*,*,#39141,.F.) ;
#52918=ORIENTED_EDGE('',*,*,#39142,.F.) ;
#52919=ORIENTED_EDGE('',*,*,#39140,.F.) ;
#52920=ORIENTED_EDGE('',*,*,#39143,.F.) ;
#52921=ORIENTED_EDGE('',*,*,#39144,.T.) ;
#52922=ORIENTED_EDGE('',*,*,#39145,.F.) ;
#52923=ORIENTED_EDGE('',*,*,#39144,.F.) ;
#52924=ORIENTED_EDGE('',*,*,#39146,.F.) ;
#52925=ORIENTED_EDGE('',*,*,#39147,.F.) ;
#52926=ORIENTED_EDGE('',*,*,#39148,.T.) ;
#52927=ORIENTED_EDGE('',*,*,#39149,.F.) ;
#52928=ORIENTED_EDGE('',*,*,#39150,.T.) ;
#52929=ORIENTED_EDGE('',*,*,#39151,.F.) ;
#52930=ORIENTED_EDGE('',*,*,#39152,.F.) ;
#52931=ORIENTED_EDGE('',*,*,#39153,.F.) ;
#52932=ORIENTED_EDGE('',*,*,#39154,.F.) ;
#52933=ORIENTED_EDGE('',*,*,#39155,.T.) ;
#52934=ORIENTED_EDGE('',*,*,#39156,.F.) ;
#52935=ORIENTED_EDGE('',*,*,#39157,.T.) ;
#52936=ORIENTED_EDGE('',*,*,#39158,.F.) ;
#52937=ORIENTED_EDGE('',*,*,#39159,.F.) ;
#52938=ORIENTED_EDGE('',*,*,#39157,.F.) ;
#52939=ORIENTED_EDGE('',*,*,#39160,.F.) ;
#52940=ORIENTED_EDGE('',*,*,#39161,.T.) ;
#52941=ORIENTED_EDGE('',*,*,#39162,.F.) ;
#52942=ORIENTED_EDGE('',*,*,#39161,.F.) ;
#52943=ORIENTED_EDGE('',*,*,#39163,.F.) ;
#52944=ORIENTED_EDGE('',*,*,#39164,.F.) ;
#52945=ORIENTED_EDGE('',*,*,#39165,.T.) ;
#52946=ORIENTED_EDGE('',*,*,#39166,.F.) ;
#52947=ORIENTED_EDGE('',*,*,#39167,.T.) ;
#52948=ORIENTED_EDGE('',*,*,#39168,.F.) ;
#52949=ORIENTED_EDGE('',*,*,#39169,.F.) ;
#52950=ORIENTED_EDGE('',*,*,#39170,.F.) ;
#52951=ORIENTED_EDGE('',*,*,#39171,.F.) ;
#52952=ORIENTED_EDGE('',*,*,#39172,.T.) ;
#52953=ORIENTED_EDGE('',*,*,#39173,.F.) ;
#52954=ORIENTED_EDGE('',*,*,#39174,.T.) ;
#52955=ORIENTED_EDGE('',*,*,#39175,.F.) ;
#52956=ORIENTED_EDGE('',*,*,#39176,.F.) ;
#52957=ORIENTED_EDGE('',*,*,#39174,.F.) ;
#52958=ORIENTED_EDGE('',*,*,#39177,.F.) ;
#52959=ORIENTED_EDGE('',*,*,#39178,.T.) ;
#52960=ORIENTED_EDGE('',*,*,#39179,.F.) ;
#52961=ORIENTED_EDGE('',*,*,#39178,.F.) ;
#52962=ORIENTED_EDGE('',*,*,#39180,.F.) ;
#52963=ORIENTED_EDGE('',*,*,#39181,.F.) ;
#52964=ORIENTED_EDGE('',*,*,#39182,.T.) ;
#52965=ORIENTED_EDGE('',*,*,#39183,.F.) ;
#52966=ORIENTED_EDGE('',*,*,#39184,.T.) ;
#52967=ORIENTED_EDGE('',*,*,#39185,.F.) ;
#52968=ORIENTED_EDGE('',*,*,#39186,.F.) ;
#52969=ORIENTED_EDGE('',*,*,#39187,.F.) ;
#52970=ORIENTED_EDGE('',*,*,#39188,.F.) ;
#52971=ORIENTED_EDGE('',*,*,#39189,.T.) ;
#52972=ORIENTED_EDGE('',*,*,#39190,.F.) ;
#52973=ORIENTED_EDGE('',*,*,#39191,.T.) ;
#52974=ORIENTED_EDGE('',*,*,#39192,.F.) ;
#52975=ORIENTED_EDGE('',*,*,#39193,.F.) ;
#52976=ORIENTED_EDGE('',*,*,#39191,.F.) ;
#52977=ORIENTED_EDGE('',*,*,#39194,.F.) ;
#52978=ORIENTED_EDGE('',*,*,#39195,.T.) ;
#52979=ORIENTED_EDGE('',*,*,#39196,.F.) ;
#52980=ORIENTED_EDGE('',*,*,#39195,.F.) ;
#52981=ORIENTED_EDGE('',*,*,#39197,.F.) ;
#52982=ORIENTED_EDGE('',*,*,#39198,.F.) ;
#52983=ORIENTED_EDGE('',*,*,#39199,.T.) ;
#52984=ORIENTED_EDGE('',*,*,#39200,.F.) ;
#52985=ORIENTED_EDGE('',*,*,#39201,.T.) ;
#52986=ORIENTED_EDGE('',*,*,#39202,.F.) ;
#52987=ORIENTED_EDGE('',*,*,#39203,.F.) ;
#52988=ORIENTED_EDGE('',*,*,#39204,.F.) ;
#52989=ORIENTED_EDGE('',*,*,#39205,.F.) ;
#52990=ORIENTED_EDGE('',*,*,#39206,.T.) ;
#52991=ORIENTED_EDGE('',*,*,#39207,.F.) ;
#52992=ORIENTED_EDGE('',*,*,#39208,.T.) ;
#52993=ORIENTED_EDGE('',*,*,#39209,.F.) ;
#52994=ORIENTED_EDGE('',*,*,#39210,.F.) ;
#52995=ORIENTED_EDGE('',*,*,#39208,.F.) ;
#52996=ORIENTED_EDGE('',*,*,#39211,.F.) ;
#52997=ORIENTED_EDGE('',*,*,#39212,.T.) ;
#52998=ORIENTED_EDGE('',*,*,#39213,.F.) ;
#52999=ORIENTED_EDGE('',*,*,#39212,.F.) ;
#53000=ORIENTED_EDGE('',*,*,#39214,.F.) ;
#53001=ORIENTED_EDGE('',*,*,#39215,.F.) ;
#53002=ORIENTED_EDGE('',*,*,#39216,.T.) ;
#53003=ORIENTED_EDGE('',*,*,#39217,.F.) ;
#53004=ORIENTED_EDGE('',*,*,#39218,.T.) ;
#53005=ORIENTED_EDGE('',*,*,#39219,.F.) ;
#53006=ORIENTED_EDGE('',*,*,#39220,.F.) ;
#53007=ORIENTED_EDGE('',*,*,#39221,.F.) ;
#53008=ORIENTED_EDGE('',*,*,#39222,.F.) ;
#53009=ORIENTED_EDGE('',*,*,#39223,.T.) ;
#53010=ORIENTED_EDGE('',*,*,#39224,.F.) ;
#53011=ORIENTED_EDGE('',*,*,#39225,.T.) ;
#53012=ORIENTED_EDGE('',*,*,#39226,.F.) ;
#53013=ORIENTED_EDGE('',*,*,#39227,.F.) ;
#53014=ORIENTED_EDGE('',*,*,#39225,.F.) ;
#53015=ORIENTED_EDGE('',*,*,#39228,.F.) ;
#53016=ORIENTED_EDGE('',*,*,#39229,.F.) ;
#53017=ORIENTED_EDGE('',*,*,#39230,.F.) ;
#53018=ORIENTED_EDGE('',*,*,#39231,.T.) ;
#53019=ORIENTED_EDGE('',*,*,#39232,.F.) ;
#53020=ORIENTED_EDGE('',*,*,#39233,.F.) ;
#53021=ORIENTED_EDGE('',*,*,#39234,.F.) ;
#53022=ORIENTED_EDGE('',*,*,#39235,.T.) ;
#53023=ORIENTED_EDGE('',*,*,#39236,.F.) ;
#53024=ORIENTED_EDGE('',*,*,#39237,.F.) ;
#53025=ORIENTED_EDGE('',*,*,#39238,.F.) ;
#53026=ORIENTED_EDGE('',*,*,#39239,.T.) ;
#53027=ORIENTED_EDGE('',*,*,#39240,.F.) ;
#53028=ORIENTED_EDGE('',*,*,#39241,.F.) ;
#53029=ORIENTED_EDGE('',*,*,#39242,.F.) ;
#53030=ORIENTED_EDGE('',*,*,#39243,.T.) ;
#53031=ORIENTED_EDGE('',*,*,#39244,.F.) ;
#53032=ORIENTED_EDGE('',*,*,#39245,.F.) ;
#53033=ORIENTED_EDGE('',*,*,#39246,.F.) ;
#53034=ORIENTED_EDGE('',*,*,#39247,.T.) ;
#53035=ORIENTED_EDGE('',*,*,#39248,.F.) ;
#53036=ORIENTED_EDGE('',*,*,#39249,.F.) ;
#53037=ORIENTED_EDGE('',*,*,#39250,.F.) ;
#53038=ORIENTED_EDGE('',*,*,#39251,.T.) ;
#53039=ORIENTED_EDGE('',*,*,#39252,.F.) ;
#53040=ORIENTED_EDGE('',*,*,#39253,.F.) ;
#53041=ORIENTED_EDGE('',*,*,#39254,.F.) ;
#53042=ORIENTED_EDGE('',*,*,#39255,.T.) ;
#53043=ORIENTED_EDGE('',*,*,#39256,.F.) ;
#53044=ORIENTED_EDGE('',*,*,#39257,.F.) ;
#53045=ORIENTED_EDGE('',*,*,#39258,.F.) ;
#53046=ORIENTED_EDGE('',*,*,#39259,.T.) ;
#53047=ORIENTED_EDGE('',*,*,#39260,.F.) ;
#53048=ORIENTED_EDGE('',*,*,#39261,.F.) ;
#53049=ORIENTED_EDGE('',*,*,#39262,.F.) ;
#53050=ORIENTED_EDGE('',*,*,#39263,.T.) ;
#53051=ORIENTED_EDGE('',*,*,#39264,.F.) ;
#53052=ORIENTED_EDGE('',*,*,#39265,.T.) ;
#53053=ORIENTED_EDGE('',*,*,#39266,.F.) ;
#53054=ORIENTED_EDGE('',*,*,#39265,.F.) ;
#53055=ORIENTED_EDGE('',*,*,#39267,.F.) ;
#53056=ORIENTED_EDGE('',*,*,#39268,.F.) ;
#53057=ORIENTED_EDGE('',*,*,#39269,.T.) ;
#53058=ORIENTED_EDGE('',*,*,#39270,.F.) ;
#53059=ORIENTED_EDGE('',*,*,#39271,.T.) ;
#53060=ORIENTED_EDGE('',*,*,#39272,.F.) ;
#53061=ORIENTED_EDGE('',*,*,#39273,.F.) ;
#53062=ORIENTED_EDGE('',*,*,#39274,.F.) ;
#53063=ORIENTED_EDGE('',*,*,#39275,.F.) ;
#53064=ORIENTED_EDGE('',*,*,#39276,.T.) ;
#53065=ORIENTED_EDGE('',*,*,#39094,.T.) ;
#53066=ORIENTED_EDGE('',*,*,#39277,.T.) ;
#53067=ORIENTED_EDGE('',*,*,#39090,.T.) ;
#53068=ORIENTED_EDGE('',*,*,#39091,.T.) ;
#53069=ORIENTED_EDGE('',*,*,#39277,.F.) ;
#53070=ORIENTED_EDGE('',*,*,#39111,.T.) ;
#53071=ORIENTED_EDGE('',*,*,#39278,.T.) ;
#53072=ORIENTED_EDGE('',*,*,#39107,.T.) ;
#53073=ORIENTED_EDGE('',*,*,#39108,.T.) ;
#53074=ORIENTED_EDGE('',*,*,#39278,.F.) ;
#53075=ORIENTED_EDGE('',*,*,#39128,.T.) ;
#53076=ORIENTED_EDGE('',*,*,#39279,.T.) ;
#53077=ORIENTED_EDGE('',*,*,#39124,.T.) ;
#53078=ORIENTED_EDGE('',*,*,#39125,.T.) ;
#53079=ORIENTED_EDGE('',*,*,#39279,.F.) ;
#53080=ORIENTED_EDGE('',*,*,#39145,.T.) ;
#53081=ORIENTED_EDGE('',*,*,#39280,.T.) ;
#53082=ORIENTED_EDGE('',*,*,#39141,.T.) ;
#53083=ORIENTED_EDGE('',*,*,#39142,.T.) ;
#53084=ORIENTED_EDGE('',*,*,#39280,.F.) ;
#53085=ORIENTED_EDGE('',*,*,#39162,.T.) ;
#53086=ORIENTED_EDGE('',*,*,#39281,.T.) ;
#53087=ORIENTED_EDGE('',*,*,#39158,.T.) ;
#53088=ORIENTED_EDGE('',*,*,#39159,.T.) ;
#53089=ORIENTED_EDGE('',*,*,#39281,.F.) ;
#53090=ORIENTED_EDGE('',*,*,#39179,.T.) ;
#53091=ORIENTED_EDGE('',*,*,#39282,.T.) ;
#53092=ORIENTED_EDGE('',*,*,#39175,.T.) ;
#53093=ORIENTED_EDGE('',*,*,#39176,.T.) ;
#53094=ORIENTED_EDGE('',*,*,#39282,.F.) ;
#53095=ORIENTED_EDGE('',*,*,#39196,.T.) ;
#53096=ORIENTED_EDGE('',*,*,#39283,.T.) ;
#53097=ORIENTED_EDGE('',*,*,#39192,.T.) ;
#53098=ORIENTED_EDGE('',*,*,#39193,.T.) ;
#53099=ORIENTED_EDGE('',*,*,#39283,.F.) ;
#53100=ORIENTED_EDGE('',*,*,#39213,.T.) ;
#53101=ORIENTED_EDGE('',*,*,#39284,.T.) ;
#53102=ORIENTED_EDGE('',*,*,#39209,.T.) ;
#53103=ORIENTED_EDGE('',*,*,#39210,.T.) ;
#53104=ORIENTED_EDGE('',*,*,#39284,.F.) ;
#53105=ORIENTED_EDGE('',*,*,#39266,.T.) ;
#53106=ORIENTED_EDGE('',*,*,#39285,.T.) ;
#53107=ORIENTED_EDGE('',*,*,#39226,.T.) ;
#53108=ORIENTED_EDGE('',*,*,#39227,.T.) ;
#53109=ORIENTED_EDGE('',*,*,#39285,.F.) ;
#53110=ORIENTED_EDGE('',*,*,#39286,.T.) ;
#53111=ORIENTED_EDGE('',*,*,#39287,.T.) ;
#53112=ORIENTED_EDGE('',*,*,#39230,.T.) ;
#53113=ORIENTED_EDGE('',*,*,#39288,.F.) ;
#53114=ORIENTED_EDGE('',*,*,#39289,.T.) ;
#53115=ORIENTED_EDGE('',*,*,#39290,.T.) ;
#53116=ORIENTED_EDGE('',*,*,#39234,.T.) ;
#53117=ORIENTED_EDGE('',*,*,#39291,.F.) ;
#53118=ORIENTED_EDGE('',*,*,#39292,.T.) ;
#53119=ORIENTED_EDGE('',*,*,#39293,.T.) ;
#53120=ORIENTED_EDGE('',*,*,#39238,.T.) ;
#53121=ORIENTED_EDGE('',*,*,#39294,.F.) ;
#53122=ORIENTED_EDGE('',*,*,#39295,.T.) ;
#53123=ORIENTED_EDGE('',*,*,#39296,.T.) ;
#53124=ORIENTED_EDGE('',*,*,#39242,.T.) ;
#53125=ORIENTED_EDGE('',*,*,#39297,.F.) ;
#53126=ORIENTED_EDGE('',*,*,#39298,.T.) ;
#53127=ORIENTED_EDGE('',*,*,#39299,.T.) ;
#53128=ORIENTED_EDGE('',*,*,#39246,.T.) ;
#53129=ORIENTED_EDGE('',*,*,#39300,.F.) ;
#53130=ORIENTED_EDGE('',*,*,#39301,.T.) ;
#53131=ORIENTED_EDGE('',*,*,#39302,.T.) ;
#53132=ORIENTED_EDGE('',*,*,#39250,.T.) ;
#53133=ORIENTED_EDGE('',*,*,#39303,.F.) ;
#53134=ORIENTED_EDGE('',*,*,#39304,.T.) ;
#53135=ORIENTED_EDGE('',*,*,#39305,.T.) ;
#53136=ORIENTED_EDGE('',*,*,#39254,.T.) ;
#53137=ORIENTED_EDGE('',*,*,#39306,.F.) ;
#53138=ORIENTED_EDGE('',*,*,#39307,.T.) ;
#53139=ORIENTED_EDGE('',*,*,#39308,.T.) ;
#53140=ORIENTED_EDGE('',*,*,#39258,.T.) ;
#53141=ORIENTED_EDGE('',*,*,#39309,.F.) ;
#53142=ORIENTED_EDGE('',*,*,#39310,.T.) ;
#53143=ORIENTED_EDGE('',*,*,#39311,.T.) ;
#53144=ORIENTED_EDGE('',*,*,#39262,.T.) ;
#53145=ORIENTED_EDGE('',*,*,#39312,.F.) ;
#53146=ORIENTED_EDGE('',*,*,#39313,.F.) ;
#53147=ORIENTED_EDGE('',*,*,#39314,.T.) ;
#53148=ORIENTED_EDGE('',*,*,#39315,.F.) ;
#53149=ORIENTED_EDGE('',*,*,#39316,.F.) ;
#53150=ORIENTED_EDGE('',*,*,#39314,.F.) ;
#53151=ORIENTED_EDGE('',*,*,#39317,.F.) ;
#53152=ORIENTED_EDGE('',*,*,#39318,.F.) ;
#53153=ORIENTED_EDGE('',*,*,#39319,.F.) ;
#53154=ORIENTED_EDGE('',*,*,#39320,.T.) ;
#53155=ORIENTED_EDGE('',*,*,#39321,.F.) ;
#53156=ORIENTED_EDGE('',*,*,#39322,.T.) ;
#53157=ORIENTED_EDGE('',*,*,#39323,.F.) ;
#53158=ORIENTED_EDGE('',*,*,#39322,.F.) ;
#53159=ORIENTED_EDGE('',*,*,#39324,.F.) ;
#53160=ORIENTED_EDGE('',*,*,#39325,.F.) ;
#53161=ORIENTED_EDGE('',*,*,#39326,.T.) ;
#53162=ORIENTED_EDGE('',*,*,#39327,.F.) ;
#53163=ORIENTED_EDGE('',*,*,#39328,.T.) ;
#53164=ORIENTED_EDGE('',*,*,#39329,.F.) ;
#53165=ORIENTED_EDGE('',*,*,#39330,.F.) ;
#53166=ORIENTED_EDGE('',*,*,#39331,.F.) ;
#53167=ORIENTED_EDGE('',*,*,#39332,.F.) ;
#53168=ORIENTED_EDGE('',*,*,#39333,.T.) ;
#53169=ORIENTED_EDGE('',*,*,#39323,.T.) ;
#53170=ORIENTED_EDGE('',*,*,#39334,.T.) ;
#53171=ORIENTED_EDGE('',*,*,#39315,.T.) ;
#53172=ORIENTED_EDGE('',*,*,#39316,.T.) ;
#53173=ORIENTED_EDGE('',*,*,#39334,.F.) ;
#53174=ORIENTED_EDGE('',*,*,#39335,.T.) ;
#53175=ORIENTED_EDGE('',*,*,#39336,.T.) ;
#53176=ORIENTED_EDGE('',*,*,#39319,.T.) ;
#53177=ORIENTED_EDGE('',*,*,#39337,.F.) ;
#53178=ORIENTED_EDGE('',*,*,#39338,.T.) ;
#53179=ORIENTED_EDGE('',*,*,#39339,.T.) ;
#53180=ORIENTED_EDGE('',*,*,#39340,.T.) ;
#53181=ORIENTED_EDGE('',*,*,#39341,.T.) ;
#53182=ORIENTED_EDGE('',*,*,#39102,.T.) ;
#53183=ORIENTED_EDGE('',*,*,#39342,.F.) ;
#53184=ORIENTED_EDGE('',*,*,#39343,.T.) ;
#53185=ORIENTED_EDGE('',*,*,#39344,.T.) ;
#53186=ORIENTED_EDGE('',*,*,#39345,.T.) ;
#53187=ORIENTED_EDGE('',*,*,#39346,.T.) ;
#53188=ORIENTED_EDGE('',*,*,#39347,.T.) ;
#53189=ORIENTED_EDGE('',*,*,#39348,.F.) ;
#53190=ORIENTED_EDGE('',*,*,#39349,.T.) ;
#53191=ORIENTED_EDGE('',*,*,#39350,.T.) ;
#53192=ORIENTED_EDGE('',*,*,#39351,.T.) ;
#53193=ORIENTED_EDGE('',*,*,#39352,.T.) ;
#53194=ORIENTED_EDGE('',*,*,#39119,.T.) ;
#53195=ORIENTED_EDGE('',*,*,#39353,.F.) ;
#53196=ORIENTED_EDGE('',*,*,#39354,.T.) ;
#53197=ORIENTED_EDGE('',*,*,#39355,.T.) ;
#53198=ORIENTED_EDGE('',*,*,#39356,.T.) ;
#53199=ORIENTED_EDGE('',*,*,#39357,.T.) ;
#53200=ORIENTED_EDGE('',*,*,#39358,.T.) ;
#53201=ORIENTED_EDGE('',*,*,#39359,.F.) ;
#53202=ORIENTED_EDGE('',*,*,#39360,.T.) ;
#53203=ORIENTED_EDGE('',*,*,#39361,.T.) ;
#53204=ORIENTED_EDGE('',*,*,#39362,.T.) ;
#53205=ORIENTED_EDGE('',*,*,#39363,.T.) ;
#53206=ORIENTED_EDGE('',*,*,#39136,.T.) ;
#53207=ORIENTED_EDGE('',*,*,#39364,.F.) ;
#53208=ORIENTED_EDGE('',*,*,#39365,.T.) ;
#53209=ORIENTED_EDGE('',*,*,#39366,.T.) ;
#53210=ORIENTED_EDGE('',*,*,#39367,.T.) ;
#53211=ORIENTED_EDGE('',*,*,#39368,.T.) ;
#53212=ORIENTED_EDGE('',*,*,#39369,.T.) ;
#53213=ORIENTED_EDGE('',*,*,#39370,.F.) ;
#53214=ORIENTED_EDGE('',*,*,#39371,.T.) ;
#53215=ORIENTED_EDGE('',*,*,#39372,.T.) ;
#53216=ORIENTED_EDGE('',*,*,#39373,.T.) ;
#53217=ORIENTED_EDGE('',*,*,#39374,.T.) ;
#53218=ORIENTED_EDGE('',*,*,#39153,.T.) ;
#53219=ORIENTED_EDGE('',*,*,#39375,.F.) ;
#53220=ORIENTED_EDGE('',*,*,#39376,.T.) ;
#53221=ORIENTED_EDGE('',*,*,#39377,.T.) ;
#53222=ORIENTED_EDGE('',*,*,#39378,.T.) ;
#53223=ORIENTED_EDGE('',*,*,#39379,.T.) ;
#53224=ORIENTED_EDGE('',*,*,#39380,.T.) ;
#53225=ORIENTED_EDGE('',*,*,#39381,.F.) ;
#53226=ORIENTED_EDGE('',*,*,#39382,.T.) ;
#53227=ORIENTED_EDGE('',*,*,#39383,.T.) ;
#53228=ORIENTED_EDGE('',*,*,#39384,.T.) ;
#53229=ORIENTED_EDGE('',*,*,#39385,.T.) ;
#53230=ORIENTED_EDGE('',*,*,#39170,.T.) ;
#53231=ORIENTED_EDGE('',*,*,#39386,.F.) ;
#53232=ORIENTED_EDGE('',*,*,#39387,.T.) ;
#53233=ORIENTED_EDGE('',*,*,#39388,.T.) ;
#53234=ORIENTED_EDGE('',*,*,#39389,.T.) ;
#53235=ORIENTED_EDGE('',*,*,#39390,.T.) ;
#53236=ORIENTED_EDGE('',*,*,#39391,.T.) ;
#53237=ORIENTED_EDGE('',*,*,#39392,.F.) ;
#53238=ORIENTED_EDGE('',*,*,#39393,.T.) ;
#53239=ORIENTED_EDGE('',*,*,#39394,.T.) ;
#53240=ORIENTED_EDGE('',*,*,#39395,.T.) ;
#53241=ORIENTED_EDGE('',*,*,#39396,.T.) ;
#53242=ORIENTED_EDGE('',*,*,#39187,.T.) ;
#53243=ORIENTED_EDGE('',*,*,#39397,.F.) ;
#53244=ORIENTED_EDGE('',*,*,#39398,.T.) ;
#53245=ORIENTED_EDGE('',*,*,#39399,.T.) ;
#53246=ORIENTED_EDGE('',*,*,#39400,.T.) ;
#53247=ORIENTED_EDGE('',*,*,#39401,.T.) ;
#53248=ORIENTED_EDGE('',*,*,#39402,.T.) ;
#53249=ORIENTED_EDGE('',*,*,#39403,.F.) ;
#53250=ORIENTED_EDGE('',*,*,#39404,.T.) ;
#53251=ORIENTED_EDGE('',*,*,#39405,.T.) ;
#53252=ORIENTED_EDGE('',*,*,#39406,.T.) ;
#53253=ORIENTED_EDGE('',*,*,#39407,.T.) ;
#53254=ORIENTED_EDGE('',*,*,#39204,.T.) ;
#53255=ORIENTED_EDGE('',*,*,#39408,.F.) ;
#53256=ORIENTED_EDGE('',*,*,#39409,.T.) ;
#53257=ORIENTED_EDGE('',*,*,#39410,.T.) ;
#53258=ORIENTED_EDGE('',*,*,#39411,.T.) ;
#53259=ORIENTED_EDGE('',*,*,#39412,.T.) ;
#53260=ORIENTED_EDGE('',*,*,#39413,.T.) ;
#53261=ORIENTED_EDGE('',*,*,#39414,.F.) ;
#53262=ORIENTED_EDGE('',*,*,#39415,.T.) ;
#53263=ORIENTED_EDGE('',*,*,#39416,.T.) ;
#53264=ORIENTED_EDGE('',*,*,#39417,.T.) ;
#53265=ORIENTED_EDGE('',*,*,#39418,.T.) ;
#53266=ORIENTED_EDGE('',*,*,#39221,.T.) ;
#53267=ORIENTED_EDGE('',*,*,#39419,.F.) ;
#53268=ORIENTED_EDGE('',*,*,#39420,.T.) ;
#53269=ORIENTED_EDGE('',*,*,#39421,.T.) ;
#53270=ORIENTED_EDGE('',*,*,#39422,.T.) ;
#53271=ORIENTED_EDGE('',*,*,#39423,.T.) ;
#53272=ORIENTED_EDGE('',*,*,#39424,.T.) ;
#53273=ORIENTED_EDGE('',*,*,#39425,.F.) ;
#53274=ORIENTED_EDGE('',*,*,#39426,.T.) ;
#53275=ORIENTED_EDGE('',*,*,#39427,.T.) ;
#53276=ORIENTED_EDGE('',*,*,#39428,.T.) ;
#53277=ORIENTED_EDGE('',*,*,#39429,.T.) ;
#53278=ORIENTED_EDGE('',*,*,#39274,.T.) ;
#53279=ORIENTED_EDGE('',*,*,#39430,.F.) ;
#53280=ORIENTED_EDGE('',*,*,#39431,.T.) ;
#53281=ORIENTED_EDGE('',*,*,#39432,.T.) ;
#53282=ORIENTED_EDGE('',*,*,#39433,.T.) ;
#53283=ORIENTED_EDGE('',*,*,#39434,.T.) ;
#53284=ORIENTED_EDGE('',*,*,#39435,.T.) ;
#53285=ORIENTED_EDGE('',*,*,#39436,.F.) ;
#53286=ORIENTED_EDGE('',*,*,#39437,.F.) ;
#53287=ORIENTED_EDGE('',*,*,#39438,.T.) ;
#53288=ORIENTED_EDGE('',*,*,#39439,.T.) ;
#53289=ORIENTED_EDGE('',*,*,#39440,.T.) ;
#53290=ORIENTED_EDGE('',*,*,#39441,.T.) ;
#53291=ORIENTED_EDGE('',*,*,#39442,.F.) ;
#53292=ORIENTED_EDGE('',*,*,#39443,.T.) ;
#53293=ORIENTED_EDGE('',*,*,#39444,.T.) ;
#53294=ORIENTED_EDGE('',*,*,#39445,.T.) ;
#53295=ORIENTED_EDGE('',*,*,#39446,.T.) ;
#53296=ORIENTED_EDGE('',*,*,#39447,.F.) ;
#53297=ORIENTED_EDGE('',*,*,#39448,.T.) ;
#53298=ORIENTED_EDGE('',*,*,#39449,.T.) ;
#53299=ORIENTED_EDGE('',*,*,#39450,.T.) ;
#53300=ORIENTED_EDGE('',*,*,#39451,.T.) ;
#53301=ORIENTED_EDGE('',*,*,#39452,.F.) ;
#53302=ORIENTED_EDGE('',*,*,#39453,.T.) ;
#53303=ORIENTED_EDGE('',*,*,#39454,.T.) ;
#53304=ORIENTED_EDGE('',*,*,#39455,.T.) ;
#53305=ORIENTED_EDGE('',*,*,#39456,.T.) ;
#53306=ORIENTED_EDGE('',*,*,#39457,.F.) ;
#53307=ORIENTED_EDGE('',*,*,#39458,.T.) ;
#53308=ORIENTED_EDGE('',*,*,#39459,.T.) ;
#53309=ORIENTED_EDGE('',*,*,#39460,.T.) ;
#53310=ORIENTED_EDGE('',*,*,#39461,.T.) ;
#53311=ORIENTED_EDGE('',*,*,#39462,.F.) ;
#53312=ORIENTED_EDGE('',*,*,#39463,.T.) ;
#53313=ORIENTED_EDGE('',*,*,#39464,.T.) ;
#53314=ORIENTED_EDGE('',*,*,#39465,.T.) ;
#53315=ORIENTED_EDGE('',*,*,#39466,.T.) ;
#53316=ORIENTED_EDGE('',*,*,#39467,.F.) ;
#53317=ORIENTED_EDGE('',*,*,#39468,.T.) ;
#53318=ORIENTED_EDGE('',*,*,#39469,.T.) ;
#53319=ORIENTED_EDGE('',*,*,#39470,.T.) ;
#53320=ORIENTED_EDGE('',*,*,#39471,.T.) ;
#53321=ORIENTED_EDGE('',*,*,#39472,.F.) ;
#53322=ORIENTED_EDGE('',*,*,#39473,.T.) ;
#53323=ORIENTED_EDGE('',*,*,#39474,.T.) ;
#53324=ORIENTED_EDGE('',*,*,#39475,.T.) ;
#53325=ORIENTED_EDGE('',*,*,#39476,.T.) ;
#53326=ORIENTED_EDGE('',*,*,#39477,.F.) ;
#53327=ORIENTED_EDGE('',*,*,#39478,.T.) ;
#53328=ORIENTED_EDGE('',*,*,#39479,.T.) ;
#53329=ORIENTED_EDGE('',*,*,#39480,.T.) ;
#53330=ORIENTED_EDGE('',*,*,#39481,.T.) ;
#53331=ORIENTED_EDGE('',*,*,#39482,.F.) ;
#53332=ORIENTED_EDGE('',*,*,#39483,.T.) ;
#53333=ORIENTED_EDGE('',*,*,#39484,.T.) ;
#53334=ORIENTED_EDGE('',*,*,#39485,.T.) ;
#53335=ORIENTED_EDGE('',*,*,#39486,.T.) ;
#53336=ORIENTED_EDGE('',*,*,#39487,.F.) ;
#53337=ORIENTED_EDGE('',*,*,#39488,.T.) ;
#53338=ORIENTED_EDGE('',*,*,#39489,.T.) ;
#53339=ORIENTED_EDGE('',*,*,#39490,.T.) ;
#53340=ORIENTED_EDGE('',*,*,#39491,.T.) ;
#53341=ORIENTED_EDGE('',*,*,#39492,.F.) ;
#53342=ORIENTED_EDGE('',*,*,#39493,.T.) ;
#53343=ORIENTED_EDGE('',*,*,#39494,.T.) ;
#53344=ORIENTED_EDGE('',*,*,#39495,.T.) ;
#53345=ORIENTED_EDGE('',*,*,#39496,.T.) ;
#53346=ORIENTED_EDGE('',*,*,#39497,.F.) ;
#53347=ORIENTED_EDGE('',*,*,#39498,.T.) ;
#53348=ORIENTED_EDGE('',*,*,#39499,.T.) ;
#53349=ORIENTED_EDGE('',*,*,#39500,.T.) ;
#53350=ORIENTED_EDGE('',*,*,#39501,.T.) ;
#53351=ORIENTED_EDGE('',*,*,#39502,.F.) ;
#53352=ORIENTED_EDGE('',*,*,#39503,.T.) ;
#53353=ORIENTED_EDGE('',*,*,#39504,.T.) ;
#53354=ORIENTED_EDGE('',*,*,#39505,.T.) ;
#53355=ORIENTED_EDGE('',*,*,#39506,.T.) ;
#53356=ORIENTED_EDGE('',*,*,#39507,.F.) ;
#53357=ORIENTED_EDGE('',*,*,#39508,.T.) ;
#53358=ORIENTED_EDGE('',*,*,#39509,.T.) ;
#53359=ORIENTED_EDGE('',*,*,#39510,.T.) ;
#53360=ORIENTED_EDGE('',*,*,#39511,.T.) ;
#53361=ORIENTED_EDGE('',*,*,#39512,.F.) ;
#53362=ORIENTED_EDGE('',*,*,#39513,.T.) ;
#53363=ORIENTED_EDGE('',*,*,#39514,.T.) ;
#53364=ORIENTED_EDGE('',*,*,#39515,.T.) ;
#53365=ORIENTED_EDGE('',*,*,#39516,.T.) ;
#53366=ORIENTED_EDGE('',*,*,#39517,.F.) ;
#53367=ORIENTED_EDGE('',*,*,#39518,.T.) ;
#53368=ORIENTED_EDGE('',*,*,#39519,.T.) ;
#53369=ORIENTED_EDGE('',*,*,#39520,.T.) ;
#53370=ORIENTED_EDGE('',*,*,#39521,.T.) ;
#53371=ORIENTED_EDGE('',*,*,#39522,.F.) ;
#53372=ORIENTED_EDGE('',*,*,#39523,.T.) ;
#53373=ORIENTED_EDGE('',*,*,#39524,.T.) ;
#53374=ORIENTED_EDGE('',*,*,#39525,.T.) ;
#53375=ORIENTED_EDGE('',*,*,#39526,.T.) ;
#53376=ORIENTED_EDGE('',*,*,#39527,.F.) ;
#53377=ORIENTED_EDGE('',*,*,#39528,.T.) ;
#53378=ORIENTED_EDGE('',*,*,#39529,.T.) ;
#53379=ORIENTED_EDGE('',*,*,#39530,.T.) ;
#53380=ORIENTED_EDGE('',*,*,#39531,.F.) ;
#53381=ORIENTED_EDGE('',*,*,#39532,.T.) ;
#53382=ORIENTED_EDGE('',*,*,#39533,.T.) ;
#53383=ORIENTED_EDGE('',*,*,#39534,.T.) ;
#53384=ORIENTED_EDGE('',*,*,#39535,.F.) ;
#53385=ORIENTED_EDGE('',*,*,#39536,.T.) ;
#53386=ORIENTED_EDGE('',*,*,#39537,.T.) ;
#53387=ORIENTED_EDGE('',*,*,#39538,.T.) ;
#53388=ORIENTED_EDGE('',*,*,#39539,.F.) ;
#53389=ORIENTED_EDGE('',*,*,#39540,.T.) ;
#53390=ORIENTED_EDGE('',*,*,#39541,.T.) ;
#53391=ORIENTED_EDGE('',*,*,#39542,.T.) ;
#53392=ORIENTED_EDGE('',*,*,#39543,.F.) ;
#53393=ORIENTED_EDGE('',*,*,#39544,.T.) ;
#53394=ORIENTED_EDGE('',*,*,#39545,.T.) ;
#53395=ORIENTED_EDGE('',*,*,#39546,.T.) ;
#53396=ORIENTED_EDGE('',*,*,#39547,.F.) ;
#53397=ORIENTED_EDGE('',*,*,#39548,.T.) ;
#53398=ORIENTED_EDGE('',*,*,#39549,.T.) ;
#53399=ORIENTED_EDGE('',*,*,#39550,.T.) ;
#53400=ORIENTED_EDGE('',*,*,#39551,.F.) ;
#53401=ORIENTED_EDGE('',*,*,#39552,.T.) ;
#53402=ORIENTED_EDGE('',*,*,#39553,.T.) ;
#53403=ORIENTED_EDGE('',*,*,#39554,.T.) ;
#53404=ORIENTED_EDGE('',*,*,#39555,.F.) ;
#53405=ORIENTED_EDGE('',*,*,#39556,.T.) ;
#53406=ORIENTED_EDGE('',*,*,#39557,.T.) ;
#53407=ORIENTED_EDGE('',*,*,#39558,.T.) ;
#53408=ORIENTED_EDGE('',*,*,#39559,.F.) ;
#53409=ORIENTED_EDGE('',*,*,#39560,.T.) ;
#53410=ORIENTED_EDGE('',*,*,#39561,.T.) ;
#53411=ORIENTED_EDGE('',*,*,#39562,.T.) ;
#53412=ORIENTED_EDGE('',*,*,#39563,.T.) ;
#53413=ORIENTED_EDGE('',*,*,#39564,.T.) ;
#53414=ORIENTED_EDGE('',*,*,#39565,.T.) ;
#53415=ORIENTED_EDGE('',*,*,#39566,.T.) ;
#53416=ORIENTED_EDGE('',*,*,#39331,.T.) ;
#53417=ORIENTED_EDGE('',*,*,#39567,.F.) ;
#53418=ORIENTED_EDGE('',*,*,#39568,.T.) ;
#53419=ORIENTED_EDGE('',*,*,#39569,.T.) ;
#53420=ORIENTED_EDGE('',*,*,#39570,.T.) ;
#53421=ORIENTED_EDGE('',*,*,#39571,.T.) ;
#53422=ORIENTED_EDGE('',*,*,#39572,.T.) ;
#53423=ORIENTED_EDGE('',*,*,#39573,.F.) ;
#53424=ORIENTED_EDGE('',*,*,#39574,.F.) ;
#53425=ORIENTED_EDGE('',*,*,#39575,.T.) ;
#53426=ORIENTED_EDGE('',*,*,#39576,.T.) ;
#53427=ORIENTED_EDGE('',*,*,#39577,.T.) ;
#53428=ORIENTED_EDGE('',*,*,#39578,.T.) ;
#53429=ORIENTED_EDGE('',*,*,#39579,.F.) ;
#53430=ORIENTED_EDGE('',*,*,#39580,.T.) ;
#53431=ORIENTED_EDGE('',*,*,#39581,.T.) ;
#53432=ORIENTED_EDGE('',*,*,#39582,.T.) ;
#53433=ORIENTED_EDGE('',*,*,#39583,.T.) ;
#53434=ORIENTED_EDGE('',*,*,#39584,.F.) ;
#53435=ORIENTED_EDGE('',*,*,#39585,.T.) ;
#53436=ORIENTED_EDGE('',*,*,#39586,.T.) ;
#53437=ORIENTED_EDGE('',*,*,#39587,.T.) ;
#53438=ORIENTED_EDGE('',*,*,#39588,.F.) ;
#53439=ORIENTED_EDGE('',*,*,#39589,.T.) ;
#53440=ORIENTED_EDGE('',*,*,#39590,.T.) ;
#53441=ORIENTED_EDGE('',*,*,#39591,.T.) ;
#53442=ORIENTED_EDGE('',*,*,#39592,.F.) ;
#53443=ORIENTED_EDGE('',*,*,#39593,.T.) ;
#53444=ORIENTED_EDGE('',*,*,#39594,.F.) ;
#53445=ORIENTED_EDGE('',*,*,#39595,.T.) ;
#53446=ORIENTED_EDGE('',*,*,#39588,.T.) ;
#53447=ORIENTED_EDGE('',*,*,#39596,.T.) ;
#53448=ORIENTED_EDGE('',*,*,#39586,.F.) ;
#53449=ORIENTED_EDGE('',*,*,#39597,.T.) ;
#53450=ORIENTED_EDGE('',*,*,#39598,.F.) ;
#53451=ORIENTED_EDGE('',*,*,#39599,.T.) ;
#53452=ORIENTED_EDGE('',*,*,#39600,.F.) ;
#53453=ORIENTED_EDGE('',*,*,#39601,.T.) ;
#53454=ORIENTED_EDGE('',*,*,#39529,.F.) ;
#53455=ORIENTED_EDGE('',*,*,#39602,.T.) ;
#53456=ORIENTED_EDGE('',*,*,#39603,.F.) ;
#53457=ORIENTED_EDGE('',*,*,#39604,.T.) ;
#53458=ORIENTED_EDGE('',*,*,#39605,.F.) ;
#53459=ORIENTED_EDGE('',*,*,#39606,.T.) ;
#53460=ORIENTED_EDGE('',*,*,#39533,.F.) ;
#53461=ORIENTED_EDGE('',*,*,#39607,.T.) ;
#53462=ORIENTED_EDGE('',*,*,#39608,.F.) ;
#53463=ORIENTED_EDGE('',*,*,#39609,.T.) ;
#53464=ORIENTED_EDGE('',*,*,#39610,.F.) ;
#53465=ORIENTED_EDGE('',*,*,#39611,.T.) ;
#53466=ORIENTED_EDGE('',*,*,#39537,.F.) ;
#53467=ORIENTED_EDGE('',*,*,#39612,.T.) ;
#53468=ORIENTED_EDGE('',*,*,#39613,.F.) ;
#53469=ORIENTED_EDGE('',*,*,#39614,.T.) ;
#53470=ORIENTED_EDGE('',*,*,#39615,.F.) ;
#53471=ORIENTED_EDGE('',*,*,#39616,.T.) ;
#53472=ORIENTED_EDGE('',*,*,#39541,.F.) ;
#53473=ORIENTED_EDGE('',*,*,#39617,.T.) ;
#53474=ORIENTED_EDGE('',*,*,#39618,.F.) ;
#53475=ORIENTED_EDGE('',*,*,#39619,.T.) ;
#53476=ORIENTED_EDGE('',*,*,#39620,.F.) ;
#53477=ORIENTED_EDGE('',*,*,#39621,.T.) ;
#53478=ORIENTED_EDGE('',*,*,#39545,.F.) ;
#53479=ORIENTED_EDGE('',*,*,#39622,.T.) ;
#53480=ORIENTED_EDGE('',*,*,#39623,.F.) ;
#53481=ORIENTED_EDGE('',*,*,#39624,.T.) ;
#53482=ORIENTED_EDGE('',*,*,#39625,.F.) ;
#53483=ORIENTED_EDGE('',*,*,#39626,.T.) ;
#53484=ORIENTED_EDGE('',*,*,#39549,.F.) ;
#53485=ORIENTED_EDGE('',*,*,#39627,.T.) ;
#53486=ORIENTED_EDGE('',*,*,#39628,.F.) ;
#53487=ORIENTED_EDGE('',*,*,#39629,.T.) ;
#53488=ORIENTED_EDGE('',*,*,#39630,.F.) ;
#53489=ORIENTED_EDGE('',*,*,#39631,.T.) ;
#53490=ORIENTED_EDGE('',*,*,#39553,.F.) ;
#53491=ORIENTED_EDGE('',*,*,#39632,.T.) ;
#53492=ORIENTED_EDGE('',*,*,#39633,.F.) ;
#53493=ORIENTED_EDGE('',*,*,#39634,.T.) ;
#53494=ORIENTED_EDGE('',*,*,#39635,.F.) ;
#53495=ORIENTED_EDGE('',*,*,#39636,.T.) ;
#53496=ORIENTED_EDGE('',*,*,#39557,.F.) ;
#53497=ORIENTED_EDGE('',*,*,#39637,.T.) ;
#53498=ORIENTED_EDGE('',*,*,#39638,.F.) ;
#53499=ORIENTED_EDGE('',*,*,#39639,.T.) ;
#53500=ORIENTED_EDGE('',*,*,#39640,.F.) ;
#53501=ORIENTED_EDGE('',*,*,#39641,.T.) ;
#53502=ORIENTED_EDGE('',*,*,#39561,.F.) ;
#53503=ORIENTED_EDGE('',*,*,#39642,.T.) ;
#53504=ORIENTED_EDGE('',*,*,#39643,.F.) ;
#53505=ORIENTED_EDGE('',*,*,#39644,.T.) ;
#53506=ORIENTED_EDGE('',*,*,#39594,.T.) ;
#53507=ORIENTED_EDGE('',*,*,#39645,.T.) ;
#53508=ORIENTED_EDGE('',*,*,#39646,.F.) ;
#53509=ORIENTED_EDGE('',*,*,#39647,.T.) ;
#53510=ORIENTED_EDGE('',*,*,#39648,.F.) ;
#53511=ORIENTED_EDGE('',*,*,#39649,.T.) ;
#53512=ORIENTED_EDGE('',*,*,#39559,.T.) ;
#53513=ORIENTED_EDGE('',*,*,#39650,.T.) ;
#53514=ORIENTED_EDGE('',*,*,#39651,.F.) ;
#53515=ORIENTED_EDGE('',*,*,#39652,.T.) ;
#53516=ORIENTED_EDGE('',*,*,#39653,.F.) ;
#53517=ORIENTED_EDGE('',*,*,#39654,.T.) ;
#53518=ORIENTED_EDGE('',*,*,#39555,.T.) ;
#53519=ORIENTED_EDGE('',*,*,#39655,.T.) ;
#53520=ORIENTED_EDGE('',*,*,#39656,.F.) ;
#53521=ORIENTED_EDGE('',*,*,#39657,.T.) ;
#53522=ORIENTED_EDGE('',*,*,#39658,.F.) ;
#53523=ORIENTED_EDGE('',*,*,#39659,.T.) ;
#53524=ORIENTED_EDGE('',*,*,#39551,.T.) ;
#53525=ORIENTED_EDGE('',*,*,#39660,.T.) ;
#53526=ORIENTED_EDGE('',*,*,#39661,.F.) ;
#53527=ORIENTED_EDGE('',*,*,#39662,.T.) ;
#53528=ORIENTED_EDGE('',*,*,#39663,.F.) ;
#53529=ORIENTED_EDGE('',*,*,#39664,.T.) ;
#53530=ORIENTED_EDGE('',*,*,#39547,.T.) ;
#53531=ORIENTED_EDGE('',*,*,#39665,.T.) ;
#53532=ORIENTED_EDGE('',*,*,#39666,.F.) ;
#53533=ORIENTED_EDGE('',*,*,#39667,.T.) ;
#53534=ORIENTED_EDGE('',*,*,#39668,.F.) ;
#53535=ORIENTED_EDGE('',*,*,#39669,.T.) ;
#53536=ORIENTED_EDGE('',*,*,#39543,.T.) ;
#53537=ORIENTED_EDGE('',*,*,#39670,.T.) ;
#53538=ORIENTED_EDGE('',*,*,#39671,.F.) ;
#53539=ORIENTED_EDGE('',*,*,#39672,.T.) ;
#53540=ORIENTED_EDGE('',*,*,#39673,.F.) ;
#53541=ORIENTED_EDGE('',*,*,#39674,.T.) ;
#53542=ORIENTED_EDGE('',*,*,#39539,.T.) ;
#53543=ORIENTED_EDGE('',*,*,#39675,.T.) ;
#53544=ORIENTED_EDGE('',*,*,#39676,.F.) ;
#53545=ORIENTED_EDGE('',*,*,#39677,.T.) ;
#53546=ORIENTED_EDGE('',*,*,#39678,.F.) ;
#53547=ORIENTED_EDGE('',*,*,#39679,.T.) ;
#53548=ORIENTED_EDGE('',*,*,#39535,.T.) ;
#53549=ORIENTED_EDGE('',*,*,#39680,.T.) ;
#53550=ORIENTED_EDGE('',*,*,#39681,.F.) ;
#53551=ORIENTED_EDGE('',*,*,#39682,.T.) ;
#53552=ORIENTED_EDGE('',*,*,#39683,.F.) ;
#53553=ORIENTED_EDGE('',*,*,#39684,.T.) ;
#53554=ORIENTED_EDGE('',*,*,#39531,.T.) ;
#53555=ORIENTED_EDGE('',*,*,#39685,.T.) ;
#53556=ORIENTED_EDGE('',*,*,#39686,.F.) ;
#53557=ORIENTED_EDGE('',*,*,#39687,.T.) ;
#53558=ORIENTED_EDGE('',*,*,#39688,.F.) ;
#53559=ORIENTED_EDGE('',*,*,#39689,.T.) ;
#53560=ORIENTED_EDGE('',*,*,#39527,.T.) ;
#53561=ORIENTED_EDGE('',*,*,#39690,.T.) ;
#53562=ORIENTED_EDGE('',*,*,#39691,.F.) ;
#53563=ORIENTED_EDGE('',*,*,#39692,.T.) ;
#53564=ORIENTED_EDGE('',*,*,#39693,.F.) ;
#53565=ORIENTED_EDGE('',*,*,#39694,.T.) ;
#53566=ORIENTED_EDGE('',*,*,#39584,.T.) ;
#53567=ORIENTED_EDGE('',*,*,#39695,.T.) ;
#53568=ORIENTED_EDGE('',*,*,#39696,.F.) ;
#53569=ORIENTED_EDGE('',*,*,#39697,.T.) ;
#53570=ORIENTED_EDGE('',*,*,#39646,.T.) ;
#53571=ORIENTED_EDGE('',*,*,#39698,.T.) ;
#53572=ORIENTED_EDGE('',*,*,#39699,.F.) ;
#53573=ORIENTED_EDGE('',*,*,#39700,.T.) ;
#53574=ORIENTED_EDGE('',*,*,#39701,.F.) ;
#53575=ORIENTED_EDGE('',*,*,#39702,.T.) ;
#53576=ORIENTED_EDGE('',*,*,#39696,.T.) ;
#53577=ORIENTED_EDGE('',*,*,#39703,.T.) ;
#53578=ORIENTED_EDGE('',*,*,#39704,.F.) ;
#53579=ORIENTED_EDGE('',*,*,#39705,.T.) ;
#53580=ORIENTED_EDGE('',*,*,#39701,.T.) ;
#53581=ORIENTED_EDGE('',*,*,#39706,.T.) ;
#53582=ORIENTED_EDGE('',*,*,#39707,.F.) ;
#53583=ORIENTED_EDGE('',*,*,#39708,.T.) ;
#53584=ORIENTED_EDGE('',*,*,#39704,.T.) ;
#53585=ORIENTED_EDGE('',*,*,#39709,.T.) ;
#53586=ORIENTED_EDGE('',*,*,#39710,.F.) ;
#53587=ORIENTED_EDGE('',*,*,#39711,.T.) ;
#53588=ORIENTED_EDGE('',*,*,#39707,.T.) ;
#53589=ORIENTED_EDGE('',*,*,#39712,.T.) ;
#53590=ORIENTED_EDGE('',*,*,#39713,.F.) ;
#53591=ORIENTED_EDGE('',*,*,#39714,.T.) ;
#53592=ORIENTED_EDGE('',*,*,#39710,.T.) ;
#53593=ORIENTED_EDGE('',*,*,#39715,.T.) ;
#53594=ORIENTED_EDGE('',*,*,#39716,.F.) ;
#53595=ORIENTED_EDGE('',*,*,#39717,.T.) ;
#53596=ORIENTED_EDGE('',*,*,#39713,.T.) ;
#53597=ORIENTED_EDGE('',*,*,#39718,.T.) ;
#53598=ORIENTED_EDGE('',*,*,#39719,.F.) ;
#53599=ORIENTED_EDGE('',*,*,#39720,.T.) ;
#53600=ORIENTED_EDGE('',*,*,#39716,.T.) ;
#53601=ORIENTED_EDGE('',*,*,#39721,.T.) ;
#53602=ORIENTED_EDGE('',*,*,#39722,.F.) ;
#53603=ORIENTED_EDGE('',*,*,#39723,.T.) ;
#53604=ORIENTED_EDGE('',*,*,#39719,.T.) ;
#53605=ORIENTED_EDGE('',*,*,#39724,.T.) ;
#53606=ORIENTED_EDGE('',*,*,#39725,.F.) ;
#53607=ORIENTED_EDGE('',*,*,#39726,.T.) ;
#53608=ORIENTED_EDGE('',*,*,#39722,.T.) ;
#53609=ORIENTED_EDGE('',*,*,#39727,.T.) ;
#53610=ORIENTED_EDGE('',*,*,#39728,.F.) ;
#53611=ORIENTED_EDGE('',*,*,#39729,.T.) ;
#53612=ORIENTED_EDGE('',*,*,#39725,.T.) ;
#53613=ORIENTED_EDGE('',*,*,#39730,.T.) ;
#53614=ORIENTED_EDGE('',*,*,#39731,.F.) ;
#53615=ORIENTED_EDGE('',*,*,#39732,.T.) ;
#53616=ORIENTED_EDGE('',*,*,#39728,.T.) ;
#53617=ORIENTED_EDGE('',*,*,#39733,.T.) ;
#53618=ORIENTED_EDGE('',*,*,#39590,.F.) ;
#53619=ORIENTED_EDGE('',*,*,#39734,.T.) ;
#53620=ORIENTED_EDGE('',*,*,#39731,.T.) ;
#53621=ORIENTED_EDGE('',*,*,#39735,.T.) ;
#53622=ORIENTED_EDGE('',*,*,#39736,.T.) ;
#53623=ORIENTED_EDGE('',*,*,#39737,.T.) ;
#53624=ORIENTED_EDGE('',*,*,#39738,.T.) ;
#53625=ORIENTED_EDGE('',*,*,#39739,.T.) ;
#53626=ORIENTED_EDGE('',*,*,#39740,.T.) ;
#53627=ORIENTED_EDGE('',*,*,#39741,.T.) ;
#53628=ORIENTED_EDGE('',*,*,#39742,.T.) ;
#53629=ORIENTED_EDGE('',*,*,#39743,.T.) ;
#53630=ORIENTED_EDGE('',*,*,#39260,.T.) ;
#53631=ORIENTED_EDGE('',*,*,#39744,.T.) ;
#53632=ORIENTED_EDGE('',*,*,#39745,.T.) ;
#53633=ORIENTED_EDGE('',*,*,#39746,.T.) ;
#53634=ORIENTED_EDGE('',*,*,#39747,.T.) ;
#53635=ORIENTED_EDGE('',*,*,#39748,.T.) ;
#53636=ORIENTED_EDGE('',*,*,#39749,.T.) ;
#53637=ORIENTED_EDGE('',*,*,#39750,.T.) ;
#53638=ORIENTED_EDGE('',*,*,#39751,.T.) ;
#53639=ORIENTED_EDGE('',*,*,#39752,.T.) ;
#53640=ORIENTED_EDGE('',*,*,#39753,.T.) ;
#53641=ORIENTED_EDGE('',*,*,#39754,.T.) ;
#53642=ORIENTED_EDGE('',*,*,#39755,.T.) ;
#53643=ORIENTED_EDGE('',*,*,#39756,.T.) ;
#53644=ORIENTED_EDGE('',*,*,#39757,.T.) ;
#53645=ORIENTED_EDGE('',*,*,#39758,.T.) ;
#53646=ORIENTED_EDGE('',*,*,#39759,.T.) ;
#53647=ORIENTED_EDGE('',*,*,#39760,.T.) ;
#53648=ORIENTED_EDGE('',*,*,#39761,.T.) ;
#53649=ORIENTED_EDGE('',*,*,#39762,.T.) ;
#53650=ORIENTED_EDGE('',*,*,#39763,.T.) ;
#53651=ORIENTED_EDGE('',*,*,#39764,.T.) ;
#53652=ORIENTED_EDGE('',*,*,#39765,.T.) ;
#53653=ORIENTED_EDGE('',*,*,#39766,.T.) ;
#53654=ORIENTED_EDGE('',*,*,#39256,.T.) ;
#53655=ORIENTED_EDGE('',*,*,#39767,.T.) ;
#53656=ORIENTED_EDGE('',*,*,#39768,.T.) ;
#53657=ORIENTED_EDGE('',*,*,#39769,.T.) ;
#53658=ORIENTED_EDGE('',*,*,#39770,.T.) ;
#53659=ORIENTED_EDGE('',*,*,#39771,.T.) ;
#53660=ORIENTED_EDGE('',*,*,#39772,.T.) ;
#53661=ORIENTED_EDGE('',*,*,#39773,.T.) ;
#53662=ORIENTED_EDGE('',*,*,#39774,.T.) ;
#53663=ORIENTED_EDGE('',*,*,#39775,.T.) ;
#53664=ORIENTED_EDGE('',*,*,#39776,.T.) ;
#53665=ORIENTED_EDGE('',*,*,#39777,.T.) ;
#53666=ORIENTED_EDGE('',*,*,#39778,.T.) ;
#53667=ORIENTED_EDGE('',*,*,#39779,.T.) ;
#53668=ORIENTED_EDGE('',*,*,#39780,.T.) ;
#53669=ORIENTED_EDGE('',*,*,#39781,.T.) ;
#53670=ORIENTED_EDGE('',*,*,#39782,.T.) ;
#53671=ORIENTED_EDGE('',*,*,#39783,.T.) ;
#53672=ORIENTED_EDGE('',*,*,#39784,.T.) ;
#53673=ORIENTED_EDGE('',*,*,#39785,.T.) ;
#53674=ORIENTED_EDGE('',*,*,#39786,.T.) ;
#53675=ORIENTED_EDGE('',*,*,#39787,.T.) ;
#53676=ORIENTED_EDGE('',*,*,#39788,.T.) ;
#53677=ORIENTED_EDGE('',*,*,#39789,.T.) ;
#53678=ORIENTED_EDGE('',*,*,#39252,.T.) ;
#53679=ORIENTED_EDGE('',*,*,#39790,.T.) ;
#53680=ORIENTED_EDGE('',*,*,#39791,.T.) ;
#53681=ORIENTED_EDGE('',*,*,#39792,.T.) ;
#53682=ORIENTED_EDGE('',*,*,#39793,.T.) ;
#53683=ORIENTED_EDGE('',*,*,#39794,.T.) ;
#53684=ORIENTED_EDGE('',*,*,#39795,.T.) ;
#53685=ORIENTED_EDGE('',*,*,#39796,.T.) ;
#53686=ORIENTED_EDGE('',*,*,#39797,.T.) ;
#53687=ORIENTED_EDGE('',*,*,#39798,.T.) ;
#53688=ORIENTED_EDGE('',*,*,#39799,.T.) ;
#53689=ORIENTED_EDGE('',*,*,#39800,.T.) ;
#53690=ORIENTED_EDGE('',*,*,#39801,.T.) ;
#53691=ORIENTED_EDGE('',*,*,#39802,.T.) ;
#53692=ORIENTED_EDGE('',*,*,#39803,.T.) ;
#53693=ORIENTED_EDGE('',*,*,#39804,.T.) ;
#53694=ORIENTED_EDGE('',*,*,#39805,.T.) ;
#53695=ORIENTED_EDGE('',*,*,#39806,.T.) ;
#53696=ORIENTED_EDGE('',*,*,#39807,.T.) ;
#53697=ORIENTED_EDGE('',*,*,#39808,.T.) ;
#53698=ORIENTED_EDGE('',*,*,#39809,.T.) ;
#53699=ORIENTED_EDGE('',*,*,#39810,.T.) ;
#53700=ORIENTED_EDGE('',*,*,#39811,.T.) ;
#53701=ORIENTED_EDGE('',*,*,#39812,.T.) ;
#53702=ORIENTED_EDGE('',*,*,#39248,.T.) ;
#53703=ORIENTED_EDGE('',*,*,#39813,.T.) ;
#53704=ORIENTED_EDGE('',*,*,#39814,.T.) ;
#53705=ORIENTED_EDGE('',*,*,#39815,.T.) ;
#53706=ORIENTED_EDGE('',*,*,#39816,.T.) ;
#53707=ORIENTED_EDGE('',*,*,#39817,.T.) ;
#53708=ORIENTED_EDGE('',*,*,#39818,.T.) ;
#53709=ORIENTED_EDGE('',*,*,#39819,.T.) ;
#53710=ORIENTED_EDGE('',*,*,#39820,.T.) ;
#53711=ORIENTED_EDGE('',*,*,#39821,.T.) ;
#53712=ORIENTED_EDGE('',*,*,#39822,.T.) ;
#53713=ORIENTED_EDGE('',*,*,#39823,.T.) ;
#53714=ORIENTED_EDGE('',*,*,#39824,.T.) ;
#53715=ORIENTED_EDGE('',*,*,#39825,.T.) ;
#53716=ORIENTED_EDGE('',*,*,#39826,.T.) ;
#53717=ORIENTED_EDGE('',*,*,#39827,.T.) ;
#53718=ORIENTED_EDGE('',*,*,#39828,.T.) ;
#53719=ORIENTED_EDGE('',*,*,#39829,.T.) ;
#53720=ORIENTED_EDGE('',*,*,#39830,.T.) ;
#53721=ORIENTED_EDGE('',*,*,#39831,.T.) ;
#53722=ORIENTED_EDGE('',*,*,#39832,.T.) ;
#53723=ORIENTED_EDGE('',*,*,#39833,.T.) ;
#53724=ORIENTED_EDGE('',*,*,#39834,.T.) ;
#53725=ORIENTED_EDGE('',*,*,#39835,.T.) ;
#53726=ORIENTED_EDGE('',*,*,#39244,.T.) ;
#53727=ORIENTED_EDGE('',*,*,#39836,.T.) ;
#53728=ORIENTED_EDGE('',*,*,#39837,.T.) ;
#53729=ORIENTED_EDGE('',*,*,#39838,.T.) ;
#53730=ORIENTED_EDGE('',*,*,#39839,.T.) ;
#53731=ORIENTED_EDGE('',*,*,#39840,.T.) ;
#53732=ORIENTED_EDGE('',*,*,#39841,.T.) ;
#53733=ORIENTED_EDGE('',*,*,#39842,.T.) ;
#53734=ORIENTED_EDGE('',*,*,#39843,.T.) ;
#53735=ORIENTED_EDGE('',*,*,#39844,.T.) ;
#53736=ORIENTED_EDGE('',*,*,#39845,.T.) ;
#53737=ORIENTED_EDGE('',*,*,#39846,.T.) ;
#53738=ORIENTED_EDGE('',*,*,#39847,.T.) ;
#53739=ORIENTED_EDGE('',*,*,#39848,.T.) ;
#53740=ORIENTED_EDGE('',*,*,#39849,.T.) ;
#53741=ORIENTED_EDGE('',*,*,#39850,.T.) ;
#53742=ORIENTED_EDGE('',*,*,#39851,.T.) ;
#53743=ORIENTED_EDGE('',*,*,#39852,.T.) ;
#53744=ORIENTED_EDGE('',*,*,#39853,.T.) ;
#53745=ORIENTED_EDGE('',*,*,#39854,.T.) ;
#53746=ORIENTED_EDGE('',*,*,#39855,.T.) ;
#53747=ORIENTED_EDGE('',*,*,#39856,.T.) ;
#53748=ORIENTED_EDGE('',*,*,#39857,.T.) ;
#53749=ORIENTED_EDGE('',*,*,#39858,.T.) ;
#53750=ORIENTED_EDGE('',*,*,#39240,.T.) ;
#53751=ORIENTED_EDGE('',*,*,#39859,.T.) ;
#53752=ORIENTED_EDGE('',*,*,#39860,.T.) ;
#53753=ORIENTED_EDGE('',*,*,#39861,.T.) ;
#53754=ORIENTED_EDGE('',*,*,#39862,.T.) ;
#53755=ORIENTED_EDGE('',*,*,#39863,.T.) ;
#53756=ORIENTED_EDGE('',*,*,#39864,.T.) ;
#53757=ORIENTED_EDGE('',*,*,#39865,.T.) ;
#53758=ORIENTED_EDGE('',*,*,#39866,.T.) ;
#53759=ORIENTED_EDGE('',*,*,#39867,.T.) ;
#53760=ORIENTED_EDGE('',*,*,#39868,.T.) ;
#53761=ORIENTED_EDGE('',*,*,#39869,.T.) ;
#53762=ORIENTED_EDGE('',*,*,#39870,.T.) ;
#53763=ORIENTED_EDGE('',*,*,#39871,.T.) ;
#53764=ORIENTED_EDGE('',*,*,#39872,.T.) ;
#53765=ORIENTED_EDGE('',*,*,#39873,.T.) ;
#53766=ORIENTED_EDGE('',*,*,#39874,.T.) ;
#53767=ORIENTED_EDGE('',*,*,#39875,.T.) ;
#53768=ORIENTED_EDGE('',*,*,#39876,.T.) ;
#53769=ORIENTED_EDGE('',*,*,#39877,.T.) ;
#53770=ORIENTED_EDGE('',*,*,#39878,.T.) ;
#53771=ORIENTED_EDGE('',*,*,#39879,.T.) ;
#53772=ORIENTED_EDGE('',*,*,#39880,.T.) ;
#53773=ORIENTED_EDGE('',*,*,#39881,.T.) ;
#53774=ORIENTED_EDGE('',*,*,#39236,.T.) ;
#53775=ORIENTED_EDGE('',*,*,#39882,.T.) ;
#53776=ORIENTED_EDGE('',*,*,#39883,.T.) ;
#53777=ORIENTED_EDGE('',*,*,#39884,.T.) ;
#53778=ORIENTED_EDGE('',*,*,#39885,.T.) ;
#53779=ORIENTED_EDGE('',*,*,#39886,.T.) ;
#53780=ORIENTED_EDGE('',*,*,#39887,.T.) ;
#53781=ORIENTED_EDGE('',*,*,#39888,.T.) ;
#53782=ORIENTED_EDGE('',*,*,#39889,.T.) ;
#53783=ORIENTED_EDGE('',*,*,#39890,.T.) ;
#53784=ORIENTED_EDGE('',*,*,#39891,.T.) ;
#53785=ORIENTED_EDGE('',*,*,#39892,.T.) ;
#53786=ORIENTED_EDGE('',*,*,#39893,.T.) ;
#53787=ORIENTED_EDGE('',*,*,#39894,.T.) ;
#53788=ORIENTED_EDGE('',*,*,#39895,.T.) ;
#53789=ORIENTED_EDGE('',*,*,#39896,.T.) ;
#53790=ORIENTED_EDGE('',*,*,#39897,.T.) ;
#53791=ORIENTED_EDGE('',*,*,#39898,.T.) ;
#53792=ORIENTED_EDGE('',*,*,#39899,.T.) ;
#53793=ORIENTED_EDGE('',*,*,#39900,.T.) ;
#53794=ORIENTED_EDGE('',*,*,#39901,.T.) ;
#53795=ORIENTED_EDGE('',*,*,#39902,.T.) ;
#53796=ORIENTED_EDGE('',*,*,#39903,.T.) ;
#53797=ORIENTED_EDGE('',*,*,#39904,.T.) ;
#53798=ORIENTED_EDGE('',*,*,#39232,.T.) ;
#53799=ORIENTED_EDGE('',*,*,#39905,.T.) ;
#53800=ORIENTED_EDGE('',*,*,#39906,.T.) ;
#53801=ORIENTED_EDGE('',*,*,#39907,.T.) ;
#53802=ORIENTED_EDGE('',*,*,#39908,.T.) ;
#53803=ORIENTED_EDGE('',*,*,#39909,.T.) ;
#53804=ORIENTED_EDGE('',*,*,#39910,.T.) ;
#53805=ORIENTED_EDGE('',*,*,#39911,.T.) ;
#53806=ORIENTED_EDGE('',*,*,#39912,.T.) ;
#53807=ORIENTED_EDGE('',*,*,#39913,.T.) ;
#53808=ORIENTED_EDGE('',*,*,#39914,.T.) ;
#53809=ORIENTED_EDGE('',*,*,#39915,.T.) ;
#53810=ORIENTED_EDGE('',*,*,#39916,.T.) ;
#53811=ORIENTED_EDGE('',*,*,#39917,.T.) ;
#53812=ORIENTED_EDGE('',*,*,#39918,.T.) ;
#53813=ORIENTED_EDGE('',*,*,#39919,.T.) ;
#53814=ORIENTED_EDGE('',*,*,#39920,.T.) ;
#53815=ORIENTED_EDGE('',*,*,#39921,.T.) ;
#53816=ORIENTED_EDGE('',*,*,#39922,.T.) ;
#53817=ORIENTED_EDGE('',*,*,#39923,.T.) ;
#53818=ORIENTED_EDGE('',*,*,#39924,.T.) ;
#53819=ORIENTED_EDGE('',*,*,#39925,.T.) ;
#53820=ORIENTED_EDGE('',*,*,#39926,.T.) ;
#53821=ORIENTED_EDGE('',*,*,#39927,.T.) ;
#53822=ORIENTED_EDGE('',*,*,#39228,.T.) ;
#53823=ORIENTED_EDGE('',*,*,#39928,.T.) ;
#53824=ORIENTED_EDGE('',*,*,#39929,.T.) ;
#53825=ORIENTED_EDGE('',*,*,#39930,.T.) ;
#53826=ORIENTED_EDGE('',*,*,#39931,.T.) ;
#53827=ORIENTED_EDGE('',*,*,#39932,.T.) ;
#53828=ORIENTED_EDGE('',*,*,#39933,.T.) ;
#53829=ORIENTED_EDGE('',*,*,#39934,.T.) ;
#53830=ORIENTED_EDGE('',*,*,#39935,.T.) ;
#53831=ORIENTED_EDGE('',*,*,#39936,.T.) ;
#53832=ORIENTED_EDGE('',*,*,#39937,.T.) ;
#53833=ORIENTED_EDGE('',*,*,#39938,.T.) ;
#53834=ORIENTED_EDGE('',*,*,#39939,.T.) ;
#53835=ORIENTED_EDGE('',*,*,#39940,.T.) ;
#53836=ORIENTED_EDGE('',*,*,#39941,.T.) ;
#53837=ORIENTED_EDGE('',*,*,#39942,.T.) ;
#53838=ORIENTED_EDGE('',*,*,#39943,.T.) ;
#53839=ORIENTED_EDGE('',*,*,#39944,.T.) ;
#53840=ORIENTED_EDGE('',*,*,#39945,.T.) ;
#53841=ORIENTED_EDGE('',*,*,#39946,.T.) ;
#53842=ORIENTED_EDGE('',*,*,#39947,.T.) ;
#53843=ORIENTED_EDGE('',*,*,#39948,.T.) ;
#53844=ORIENTED_EDGE('',*,*,#39949,.T.) ;
#53845=ORIENTED_EDGE('',*,*,#39950,.T.) ;
#53846=ORIENTED_EDGE('',*,*,#39317,.T.) ;
#53847=ORIENTED_EDGE('',*,*,#39951,.T.) ;
#53848=ORIENTED_EDGE('',*,*,#39952,.T.) ;
#53849=ORIENTED_EDGE('',*,*,#39953,.T.) ;
#53850=ORIENTED_EDGE('',*,*,#39954,.T.) ;
#53851=ORIENTED_EDGE('',*,*,#39955,.T.) ;
#53852=ORIENTED_EDGE('',*,*,#39956,.T.) ;
#53853=ORIENTED_EDGE('',*,*,#39957,.T.) ;
#53854=ORIENTED_EDGE('',*,*,#39958,.T.) ;
#53855=ORIENTED_EDGE('',*,*,#39959,.T.) ;
#53856=ORIENTED_EDGE('',*,*,#39960,.T.) ;
#53857=ORIENTED_EDGE('',*,*,#39961,.T.) ;
#53858=ORIENTED_EDGE('',*,*,#39962,.T.) ;
#53859=ORIENTED_EDGE('',*,*,#39963,.T.) ;
#53860=ORIENTED_EDGE('',*,*,#39964,.T.) ;
#53861=ORIENTED_EDGE('',*,*,#39965,.T.) ;
#53862=ORIENTED_EDGE('',*,*,#39966,.T.) ;
#53863=ORIENTED_EDGE('',*,*,#39967,.T.) ;
#53864=ORIENTED_EDGE('',*,*,#39968,.T.) ;
#53865=ORIENTED_EDGE('',*,*,#39969,.T.) ;
#53866=ORIENTED_EDGE('',*,*,#39970,.T.) ;
#53867=ORIENTED_EDGE('',*,*,#39971,.T.) ;
#53868=ORIENTED_EDGE('',*,*,#39972,.T.) ;
#53869=ORIENTED_EDGE('',*,*,#39973,.T.) ;
#53870=ORIENTED_EDGE('',*,*,#39974,.T.) ;
#53871=ORIENTED_EDGE('',*,*,#39975,.T.) ;
#53872=ORIENTED_EDGE('',*,*,#39976,.T.) ;
#53873=ORIENTED_EDGE('',*,*,#39977,.T.) ;
#53874=ORIENTED_EDGE('',*,*,#39978,.T.) ;
#53875=ORIENTED_EDGE('',*,*,#39979,.T.) ;
#53876=ORIENTED_EDGE('',*,*,#39980,.T.) ;
#53877=ORIENTED_EDGE('',*,*,#39981,.T.) ;
#53878=ORIENTED_EDGE('',*,*,#39982,.T.) ;
#53879=ORIENTED_EDGE('',*,*,#39983,.T.) ;
#53880=ORIENTED_EDGE('',*,*,#39984,.T.) ;
#53881=ORIENTED_EDGE('',*,*,#39985,.T.) ;
#53882=ORIENTED_EDGE('',*,*,#39986,.T.) ;
#53883=ORIENTED_EDGE('',*,*,#39987,.T.) ;
#53884=ORIENTED_EDGE('',*,*,#39988,.T.) ;
#53885=ORIENTED_EDGE('',*,*,#39989,.T.) ;
#53886=ORIENTED_EDGE('',*,*,#39990,.T.) ;
#53887=ORIENTED_EDGE('',*,*,#39991,.T.) ;
#53888=ORIENTED_EDGE('',*,*,#39992,.F.) ;
#53889=ORIENTED_EDGE('',*,*,#39993,.T.) ;
#53890=ORIENTED_EDGE('',*,*,#39994,.F.) ;
#53891=ORIENTED_EDGE('',*,*,#39995,.T.) ;
#53892=ORIENTED_EDGE('',*,*,#39996,.T.) ;
#53893=ORIENTED_EDGE('',*,*,#39997,.T.) ;
#53894=ORIENTED_EDGE('',*,*,#39998,.T.) ;
#53895=ORIENTED_EDGE('',*,*,#39999,.T.) ;
#53896=ORIENTED_EDGE('',*,*,#40000,.T.) ;
#53897=ORIENTED_EDGE('',*,*,#40001,.T.) ;
#53898=ORIENTED_EDGE('',*,*,#40002,.T.) ;
#53899=ORIENTED_EDGE('',*,*,#39329,.T.) ;
#53900=ORIENTED_EDGE('',*,*,#40003,.T.) ;
#53901=ORIENTED_EDGE('',*,*,#40004,.T.) ;
#53902=ORIENTED_EDGE('',*,*,#40005,.T.) ;
#53903=ORIENTED_EDGE('',*,*,#40006,.T.) ;
#53904=ORIENTED_EDGE('',*,*,#40007,.T.) ;
#53905=ORIENTED_EDGE('',*,*,#40008,.T.) ;
#53906=ORIENTED_EDGE('',*,*,#40009,.T.) ;
#53907=ORIENTED_EDGE('',*,*,#40010,.T.) ;
#53908=ORIENTED_EDGE('',*,*,#40011,.T.) ;
#53909=ORIENTED_EDGE('',*,*,#40012,.T.) ;
#53910=ORIENTED_EDGE('',*,*,#40013,.T.) ;
#53911=ORIENTED_EDGE('',*,*,#40014,.T.) ;
#53912=ORIENTED_EDGE('',*,*,#40015,.F.) ;
#53913=ORIENTED_EDGE('',*,*,#40016,.T.) ;
#53914=ORIENTED_EDGE('',*,*,#40017,.T.) ;
#53915=ORIENTED_EDGE('',*,*,#40018,.T.) ;
#53916=ORIENTED_EDGE('',*,*,#40017,.F.) ;
#53917=ORIENTED_EDGE('',*,*,#40019,.T.) ;
#53918=ORIENTED_EDGE('',*,*,#40020,.T.) ;
#53919=ORIENTED_EDGE('',*,*,#40021,.T.) ;
#53920=ORIENTED_EDGE('',*,*,#40020,.F.) ;
#53921=ORIENTED_EDGE('',*,*,#40022,.T.) ;
#53922=ORIENTED_EDGE('',*,*,#40023,.T.) ;
#53923=ORIENTED_EDGE('',*,*,#40024,.T.) ;
#53924=ORIENTED_EDGE('',*,*,#40023,.F.) ;
#53925=ORIENTED_EDGE('',*,*,#40025,.T.) ;
#53926=ORIENTED_EDGE('',*,*,#40026,.T.) ;
#53927=ORIENTED_EDGE('',*,*,#40027,.T.) ;
#53928=ORIENTED_EDGE('',*,*,#40026,.F.) ;
#53929=ORIENTED_EDGE('',*,*,#40028,.T.) ;
#53930=ORIENTED_EDGE('',*,*,#40029,.T.) ;
#53931=ORIENTED_EDGE('',*,*,#40030,.T.) ;
#53932=ORIENTED_EDGE('',*,*,#40029,.F.) ;
#53933=ORIENTED_EDGE('',*,*,#40031,.T.) ;
#53934=ORIENTED_EDGE('',*,*,#40032,.T.) ;
#53935=ORIENTED_EDGE('',*,*,#40033,.T.) ;
#53936=ORIENTED_EDGE('',*,*,#40032,.F.) ;
#53937=ORIENTED_EDGE('',*,*,#39324,.T.) ;
#53938=ORIENTED_EDGE('',*,*,#40034,.T.) ;
#53939=ORIENTED_EDGE('',*,*,#40035,.T.) ;
#53940=ORIENTED_EDGE('',*,*,#40034,.F.) ;
#53941=ORIENTED_EDGE('',*,*,#40036,.T.) ;
#53942=ORIENTED_EDGE('',*,*,#39337,.T.) ;
#53943=ORIENTED_EDGE('',*,*,#40037,.T.) ;
#53944=ORIENTED_EDGE('',*,*,#39336,.F.) ;
#53945=ORIENTED_EDGE('',*,*,#40038,.T.) ;
#53946=ORIENTED_EDGE('',*,*,#40039,.T.) ;
#53947=ORIENTED_EDGE('',*,*,#40040,.T.) ;
#53948=ORIENTED_EDGE('',*,*,#40039,.F.) ;
#53949=ORIENTED_EDGE('',*,*,#40041,.T.) ;
#53950=ORIENTED_EDGE('',*,*,#40042,.T.) ;
#53951=ORIENTED_EDGE('',*,*,#40043,.T.) ;
#53952=ORIENTED_EDGE('',*,*,#40042,.F.) ;
#53953=ORIENTED_EDGE('',*,*,#40044,.T.) ;
#53954=ORIENTED_EDGE('',*,*,#40045,.T.) ;
#53955=ORIENTED_EDGE('',*,*,#40046,.T.) ;
#53956=ORIENTED_EDGE('',*,*,#40045,.F.) ;
#53957=ORIENTED_EDGE('',*,*,#40047,.T.) ;
#53958=ORIENTED_EDGE('',*,*,#40048,.T.) ;
#53959=ORIENTED_EDGE('',*,*,#40049,.T.) ;
#53960=ORIENTED_EDGE('',*,*,#40048,.F.) ;
#53961=ORIENTED_EDGE('',*,*,#40050,.T.) ;
#53962=ORIENTED_EDGE('',*,*,#40051,.T.) ;
#53963=ORIENTED_EDGE('',*,*,#40052,.T.) ;
#53964=ORIENTED_EDGE('',*,*,#40051,.F.) ;
#53965=ORIENTED_EDGE('',*,*,#40053,.T.) ;
#53966=ORIENTED_EDGE('',*,*,#40054,.T.) ;
#53967=ORIENTED_EDGE('',*,*,#40055,.T.) ;
#53968=ORIENTED_EDGE('',*,*,#40054,.F.) ;
#53969=ORIENTED_EDGE('',*,*,#40056,.T.) ;
#53970=ORIENTED_EDGE('',*,*,#40057,.T.) ;
#53971=ORIENTED_EDGE('',*,*,#40058,.T.) ;
#53972=ORIENTED_EDGE('',*,*,#40057,.F.) ;
#53973=ORIENTED_EDGE('',*,*,#40059,.T.) ;
#53974=ORIENTED_EDGE('',*,*,#40060,.T.) ;
#53975=ORIENTED_EDGE('',*,*,#40061,.T.) ;
#53976=ORIENTED_EDGE('',*,*,#40060,.F.) ;
#53977=ORIENTED_EDGE('',*,*,#40062,.T.) ;
#53978=ORIENTED_EDGE('',*,*,#40063,.T.) ;
#53979=ORIENTED_EDGE('',*,*,#40064,.T.) ;
#53980=ORIENTED_EDGE('',*,*,#40063,.F.) ;
#53981=ORIENTED_EDGE('',*,*,#40065,.T.) ;
#53982=ORIENTED_EDGE('',*,*,#40066,.T.) ;
#53983=ORIENTED_EDGE('',*,*,#40067,.T.) ;
#53984=ORIENTED_EDGE('',*,*,#40066,.F.) ;
#53985=ORIENTED_EDGE('',*,*,#40068,.T.) ;
#53986=ORIENTED_EDGE('',*,*,#40069,.T.) ;
#53987=ORIENTED_EDGE('',*,*,#40070,.T.) ;
#53988=ORIENTED_EDGE('',*,*,#40069,.F.) ;
#53989=ORIENTED_EDGE('',*,*,#40071,.T.) ;
#53990=ORIENTED_EDGE('',*,*,#40072,.T.) ;
#53991=ORIENTED_EDGE('',*,*,#40073,.T.) ;
#53992=ORIENTED_EDGE('',*,*,#40072,.F.) ;
#53993=ORIENTED_EDGE('',*,*,#40074,.T.) ;
#53994=ORIENTED_EDGE('',*,*,#40075,.T.) ;
#53995=ORIENTED_EDGE('',*,*,#40076,.T.) ;
#53996=ORIENTED_EDGE('',*,*,#40075,.F.) ;
#53997=ORIENTED_EDGE('',*,*,#40077,.T.) ;
#53998=ORIENTED_EDGE('',*,*,#40078,.T.) ;
#53999=ORIENTED_EDGE('',*,*,#40079,.T.) ;
#54000=ORIENTED_EDGE('',*,*,#40078,.F.) ;
#54001=ORIENTED_EDGE('',*,*,#40080,.T.) ;
#54002=ORIENTED_EDGE('',*,*,#40081,.T.) ;
#54003=ORIENTED_EDGE('',*,*,#40082,.T.) ;
#54004=ORIENTED_EDGE('',*,*,#40081,.F.) ;
#54005=ORIENTED_EDGE('',*,*,#40083,.T.) ;
#54006=ORIENTED_EDGE('',*,*,#40084,.T.) ;
#54007=ORIENTED_EDGE('',*,*,#40085,.T.) ;
#54008=ORIENTED_EDGE('',*,*,#40084,.F.) ;
#54009=ORIENTED_EDGE('',*,*,#40086,.T.) ;
#54010=ORIENTED_EDGE('',*,*,#40087,.T.) ;
#54011=ORIENTED_EDGE('',*,*,#40088,.T.) ;
#54012=ORIENTED_EDGE('',*,*,#40087,.F.) ;
#54013=ORIENTED_EDGE('',*,*,#40089,.T.) ;
#54014=ORIENTED_EDGE('',*,*,#40090,.T.) ;
#54015=ORIENTED_EDGE('',*,*,#40091,.T.) ;
#54016=ORIENTED_EDGE('',*,*,#40090,.F.) ;
#54017=ORIENTED_EDGE('',*,*,#40092,.T.) ;
#54018=ORIENTED_EDGE('',*,*,#40015,.T.) ;
#54019=ORIENTED_EDGE('',*,*,#40093,.T.) ;
#54020=ORIENTED_EDGE('',*,*,#40094,.T.) ;
#54021=ORIENTED_EDGE('',*,*,#40095,.T.) ;
#54022=ORIENTED_EDGE('',*,*,#40096,.T.) ;
#54023=ORIENTED_EDGE('',*,*,#40097,.T.) ;
#54024=ORIENTED_EDGE('',*,*,#40098,.T.) ;
#54025=ORIENTED_EDGE('',*,*,#40099,.T.) ;
#54026=ORIENTED_EDGE('',*,*,#40100,.T.) ;
#54027=ORIENTED_EDGE('',*,*,#40101,.T.) ;
#54028=ORIENTED_EDGE('',*,*,#40102,.T.) ;
#54029=ORIENTED_EDGE('',*,*,#40103,.T.) ;
#54030=ORIENTED_EDGE('',*,*,#40104,.T.) ;
#54031=ORIENTED_EDGE('',*,*,#40105,.T.) ;
#54032=ORIENTED_EDGE('',*,*,#40106,.T.) ;
#54033=ORIENTED_EDGE('',*,*,#40107,.T.) ;
#54034=ORIENTED_EDGE('',*,*,#40108,.T.) ;
#54035=ORIENTED_EDGE('',*,*,#40109,.T.) ;
#54036=ORIENTED_EDGE('',*,*,#40110,.T.) ;
#54037=ORIENTED_EDGE('',*,*,#40111,.T.) ;
#54038=ORIENTED_EDGE('',*,*,#39321,.T.) ;
#54039=ORIENTED_EDGE('',*,*,#39313,.T.) ;
#54040=ORIENTED_EDGE('',*,*,#40112,.F.) ;
#54041=ORIENTED_EDGE('',*,*,#40113,.T.) ;
#54042=ORIENTED_EDGE('',*,*,#40114,.T.) ;
#54043=ORIENTED_EDGE('',*,*,#40115,.T.) ;
#54044=ORIENTED_EDGE('',*,*,#40116,.T.) ;
#54045=ORIENTED_EDGE('',*,*,#40117,.T.) ;
#54046=ORIENTED_EDGE('',*,*,#40118,.T.) ;
#54047=ORIENTED_EDGE('',*,*,#40119,.T.) ;
#54048=ORIENTED_EDGE('',*,*,#40120,.F.) ;
#54049=ORIENTED_EDGE('',*,*,#40008,.F.) ;
#54050=ORIENTED_EDGE('',*,*,#40121,.F.) ;
#54051=ORIENTED_EDGE('',*,*,#39995,.F.) ;
#54052=ORIENTED_EDGE('',*,*,#40122,.F.) ;
#54053=ORIENTED_EDGE('',*,*,#40009,.F.) ;
#54054=ORIENTED_EDGE('',*,*,#40123,.F.) ;
#54055=ORIENTED_EDGE('',*,*,#40003,.F.) ;
#54056=ORIENTED_EDGE('',*,*,#40124,.F.) ;
#54057=ORIENTED_EDGE('',*,*,#40122,.T.) ;
#54058=ORIENTED_EDGE('',*,*,#40125,.F.) ;
#54059=ORIENTED_EDGE('',*,*,#40126,.F.) ;
#54060=ORIENTED_EDGE('',*,*,#40121,.T.) ;
#54061=ORIENTED_EDGE('',*,*,#40127,.F.) ;
#54062=ORIENTED_EDGE('',*,*,#40120,.T.) ;
#54063=ORIENTED_EDGE('',*,*,#39994,.T.) ;
#54064=ORIENTED_EDGE('',*,*,#40128,.F.) ;
#54065=ORIENTED_EDGE('',*,*,#40123,.T.) ;
#54066=ORIENTED_EDGE('',*,*,#40125,.T.) ;
#54067=ORIENTED_EDGE('',*,*,#40006,.F.) ;
#54068=ORIENTED_EDGE('',*,*,#40129,.F.) ;
#54069=ORIENTED_EDGE('',*,*,#39327,.T.) ;
#54070=ORIENTED_EDGE('',*,*,#40130,.T.) ;
#54071=ORIENTED_EDGE('',*,*,#40131,.F.) ;
#54072=ORIENTED_EDGE('',*,*,#40124,.T.) ;
#54073=ORIENTED_EDGE('',*,*,#40132,.F.) ;
#54074=ORIENTED_EDGE('',*,*,#40133,.T.) ;
#54075=ORIENTED_EDGE('',*,*,#40134,.F.) ;
#54076=ORIENTED_EDGE('',*,*,#39563,.F.) ;
#54077=ORIENTED_EDGE('',*,*,#40135,.F.) ;
#54078=ORIENTED_EDGE('',*,*,#40010,.F.) ;
#54079=ORIENTED_EDGE('',*,*,#40127,.T.) ;
#54080=ORIENTED_EDGE('',*,*,#40007,.F.) ;
#54081=ORIENTED_EDGE('',*,*,#40136,.F.) ;
#54082=ORIENTED_EDGE('',*,*,#40013,.F.) ;
#54083=ORIENTED_EDGE('',*,*,#40126,.T.) ;
#54084=ORIENTED_EDGE('',*,*,#40012,.F.) ;
#54085=ORIENTED_EDGE('',*,*,#40137,.F.) ;
#54086=ORIENTED_EDGE('',*,*,#39986,.F.) ;
#54087=ORIENTED_EDGE('',*,*,#40128,.T.) ;
#54088=ORIENTED_EDGE('',*,*,#39993,.F.) ;
#54089=ORIENTED_EDGE('',*,*,#40138,.F.) ;
#54090=ORIENTED_EDGE('',*,*,#40004,.F.) ;
#54091=ORIENTED_EDGE('',*,*,#40139,.F.) ;
#54092=ORIENTED_EDGE('',*,*,#40005,.F.) ;
#54093=ORIENTED_EDGE('',*,*,#40140,.F.) ;
#54094=ORIENTED_EDGE('',*,*,#40000,.F.) ;
#54095=ORIENTED_EDGE('',*,*,#40129,.T.) ;
#54096=ORIENTED_EDGE('',*,*,#40139,.T.) ;
#54097=ORIENTED_EDGE('',*,*,#39328,.F.) ;
#54098=ORIENTED_EDGE('',*,*,#40135,.T.) ;
#54099=ORIENTED_EDGE('',*,*,#39573,.T.) ;
#54100=ORIENTED_EDGE('',*,*,#40141,.F.) ;
#54101=ORIENTED_EDGE('',*,*,#40136,.T.) ;
#54102=ORIENTED_EDGE('',*,*,#40142,.F.) ;
#54103=ORIENTED_EDGE('',*,*,#40137,.T.) ;
#54104=ORIENTED_EDGE('',*,*,#40143,.F.) ;
#54105=ORIENTED_EDGE('',*,*,#39579,.T.) ;
#54106=ORIENTED_EDGE('',*,*,#40138,.T.) ;
#54107=ORIENTED_EDGE('',*,*,#39992,.T.) ;
#54108=ORIENTED_EDGE('',*,*,#40144,.F.) ;
#54109=ORIENTED_EDGE('',*,*,#40140,.T.) ;
#54110=ORIENTED_EDGE('',*,*,#40141,.T.) ;
#54111=ORIENTED_EDGE('',*,*,#39572,.F.) ;
#54112=ORIENTED_EDGE('',*,*,#40145,.F.) ;
#54113=ORIENTED_EDGE('',*,*,#40014,.F.) ;
#54114=ORIENTED_EDGE('',*,*,#40143,.T.) ;
#54115=ORIENTED_EDGE('',*,*,#40011,.F.) ;
#54116=ORIENTED_EDGE('',*,*,#40146,.F.) ;
#54117=ORIENTED_EDGE('',*,*,#39580,.F.) ;
#54118=ORIENTED_EDGE('',*,*,#39987,.F.) ;
#54119=ORIENTED_EDGE('',*,*,#40142,.T.) ;
#54120=ORIENTED_EDGE('',*,*,#40147,.F.) ;
#54121=ORIENTED_EDGE('',*,*,#40148,.F.) ;
#54122=ORIENTED_EDGE('',*,*,#40144,.T.) ;
#54123=ORIENTED_EDGE('',*,*,#39991,.F.) ;
#54124=ORIENTED_EDGE('',*,*,#40149,.F.) ;
#54125=ORIENTED_EDGE('',*,*,#40001,.F.) ;
#54126=ORIENTED_EDGE('',*,*,#40150,.F.) ;
#54127=ORIENTED_EDGE('',*,*,#40002,.F.) ;
#54128=ORIENTED_EDGE('',*,*,#40151,.F.) ;
#54129=ORIENTED_EDGE('',*,*,#39996,.F.) ;
#54130=ORIENTED_EDGE('',*,*,#39330,.T.) ;
#54131=ORIENTED_EDGE('',*,*,#40150,.T.) ;
#54132=ORIENTED_EDGE('',*,*,#40152,.F.) ;
#54133=ORIENTED_EDGE('',*,*,#39567,.T.) ;
#54134=ORIENTED_EDGE('',*,*,#40146,.T.) ;
#54135=ORIENTED_EDGE('',*,*,#40145,.T.) ;
#54136=ORIENTED_EDGE('',*,*,#40153,.F.) ;
#54137=ORIENTED_EDGE('',*,*,#40154,.F.) ;
#54138=ORIENTED_EDGE('',*,*,#39585,.F.) ;
#54139=ORIENTED_EDGE('',*,*,#40155,.F.) ;
#54140=ORIENTED_EDGE('',*,*,#40156,.F.) ;
#54141=ORIENTED_EDGE('',*,*,#40147,.T.) ;
#54142=ORIENTED_EDGE('',*,*,#39583,.F.) ;
#54143=ORIENTED_EDGE('',*,*,#40155,.T.) ;
#54144=ORIENTED_EDGE('',*,*,#39694,.F.) ;
#54145=ORIENTED_EDGE('',*,*,#40148,.T.) ;
#54146=ORIENTED_EDGE('',*,*,#40157,.F.) ;
#54147=ORIENTED_EDGE('',*,*,#40158,.F.) ;
#54148=ORIENTED_EDGE('',*,*,#40151,.T.) ;
#54149=ORIENTED_EDGE('',*,*,#40149,.T.) ;
#54150=ORIENTED_EDGE('',*,*,#40159,.F.) ;
#54151=ORIENTED_EDGE('',*,*,#40152,.T.) ;
#54152=ORIENTED_EDGE('',*,*,#39999,.F.) ;
#54153=ORIENTED_EDGE('',*,*,#40160,.F.) ;
#54154=ORIENTED_EDGE('',*,*,#39568,.F.) ;
#54155=ORIENTED_EDGE('',*,*,#40153,.T.) ;
#54156=ORIENTED_EDGE('',*,*,#39571,.F.) ;
#54157=ORIENTED_EDGE('',*,*,#40161,.F.) ;
#54158=ORIENTED_EDGE('',*,*,#39581,.F.) ;
#54159=ORIENTED_EDGE('',*,*,#40154,.T.) ;
#54160=ORIENTED_EDGE('',*,*,#39582,.F.) ;
#54161=ORIENTED_EDGE('',*,*,#40162,.F.) ;
#54162=ORIENTED_EDGE('',*,*,#39597,.F.) ;
#54163=ORIENTED_EDGE('',*,*,#40156,.T.) ;
#54164=ORIENTED_EDGE('',*,*,#39693,.T.) ;
#54165=ORIENTED_EDGE('',*,*,#40163,.F.) ;
#54166=ORIENTED_EDGE('',*,*,#40157,.T.) ;
#54167=ORIENTED_EDGE('',*,*,#39988,.F.) ;
#54168=ORIENTED_EDGE('',*,*,#40158,.T.) ;
#54169=ORIENTED_EDGE('',*,*,#40164,.F.) ;
#54170=ORIENTED_EDGE('',*,*,#40165,.F.) ;
#54171=ORIENTED_EDGE('',*,*,#40159,.T.) ;
#54172=ORIENTED_EDGE('',*,*,#39990,.F.) ;
#54173=ORIENTED_EDGE('',*,*,#40166,.F.) ;
#54174=ORIENTED_EDGE('',*,*,#39997,.F.) ;
#54175=ORIENTED_EDGE('',*,*,#40167,.F.) ;
#54176=ORIENTED_EDGE('',*,*,#39998,.F.) ;
#54177=ORIENTED_EDGE('',*,*,#40168,.F.) ;
#54178=ORIENTED_EDGE('',*,*,#39578,.F.) ;
#54179=ORIENTED_EDGE('',*,*,#40160,.T.) ;
#54180=ORIENTED_EDGE('',*,*,#40167,.T.) ;
#54181=ORIENTED_EDGE('',*,*,#40169,.F.) ;
#54182=ORIENTED_EDGE('',*,*,#40162,.T.) ;
#54183=ORIENTED_EDGE('',*,*,#40161,.T.) ;
#54184=ORIENTED_EDGE('',*,*,#40170,.F.) ;
#54185=ORIENTED_EDGE('',*,*,#39598,.T.) ;
#54186=ORIENTED_EDGE('',*,*,#40171,.F.) ;
#54187=ORIENTED_EDGE('',*,*,#40164,.T.) ;
#54188=ORIENTED_EDGE('',*,*,#40163,.T.) ;
#54189=ORIENTED_EDGE('',*,*,#39692,.F.) ;
#54190=ORIENTED_EDGE('',*,*,#40165,.T.) ;
#54191=ORIENTED_EDGE('',*,*,#40172,.F.) ;
#54192=ORIENTED_EDGE('',*,*,#40173,.F.) ;
#54193=ORIENTED_EDGE('',*,*,#40168,.T.) ;
#54194=ORIENTED_EDGE('',*,*,#40166,.T.) ;
#54195=ORIENTED_EDGE('',*,*,#40174,.F.) ;
#54196=ORIENTED_EDGE('',*,*,#39574,.T.) ;
#54197=ORIENTED_EDGE('',*,*,#40169,.T.) ;
#54198=ORIENTED_EDGE('',*,*,#39577,.F.) ;
#54199=ORIENTED_EDGE('',*,*,#40175,.F.) ;
#54200=ORIENTED_EDGE('',*,*,#39569,.F.) ;
#54201=ORIENTED_EDGE('',*,*,#40170,.T.) ;
#54202=ORIENTED_EDGE('',*,*,#39570,.F.) ;
#54203=ORIENTED_EDGE('',*,*,#40176,.F.) ;
#54204=ORIENTED_EDGE('',*,*,#39599,.F.) ;
#54205=ORIENTED_EDGE('',*,*,#40171,.T.) ;
#54206=ORIENTED_EDGE('',*,*,#39691,.T.) ;
#54207=ORIENTED_EDGE('',*,*,#40177,.F.) ;
#54208=ORIENTED_EDGE('',*,*,#40172,.T.) ;
#54209=ORIENTED_EDGE('',*,*,#39989,.F.) ;
#54210=ORIENTED_EDGE('',*,*,#40173,.T.) ;
#54211=ORIENTED_EDGE('',*,*,#40178,.F.) ;
#54212=ORIENTED_EDGE('',*,*,#40174,.T.) ;
#54213=ORIENTED_EDGE('',*,*,#40176,.T.) ;
#54214=ORIENTED_EDGE('',*,*,#40175,.T.) ;
#54215=ORIENTED_EDGE('',*,*,#40179,.F.) ;
#54216=ORIENTED_EDGE('',*,*,#39600,.T.) ;
#54217=ORIENTED_EDGE('',*,*,#40177,.T.) ;
#54218=ORIENTED_EDGE('',*,*,#39690,.F.) ;
#54219=ORIENTED_EDGE('',*,*,#40180,.F.) ;
#54220=ORIENTED_EDGE('',*,*,#39575,.F.) ;
#54221=ORIENTED_EDGE('',*,*,#40178,.T.) ;
#54222=ORIENTED_EDGE('',*,*,#40179,.T.) ;
#54223=ORIENTED_EDGE('',*,*,#39576,.F.) ;
#54224=ORIENTED_EDGE('',*,*,#40181,.F.) ;
#54225=ORIENTED_EDGE('',*,*,#39601,.F.) ;
#54226=ORIENTED_EDGE('',*,*,#40180,.T.) ;
#54227=ORIENTED_EDGE('',*,*,#39530,.F.) ;
#54228=ORIENTED_EDGE('',*,*,#40181,.T.) ;
#54229=ORIENTED_EDGE('',*,*,#40182,.F.) ;
#54230=ORIENTED_EDGE('',*,*,#40183,.F.) ;
#54231=ORIENTED_EDGE('',*,*,#39714,.F.) ;
#54232=ORIENTED_EDGE('',*,*,#40183,.T.) ;
#54233=ORIENTED_EDGE('',*,*,#39971,.F.) ;
#54234=ORIENTED_EDGE('',*,*,#40184,.F.) ;
#54235=ORIENTED_EDGE('',*,*,#39711,.F.) ;
#54236=ORIENTED_EDGE('',*,*,#40182,.T.) ;
#54237=ORIENTED_EDGE('',*,*,#39717,.F.) ;
#54238=ORIENTED_EDGE('',*,*,#40185,.F.) ;
#54239=ORIENTED_EDGE('',*,*,#39972,.F.) ;
#54240=ORIENTED_EDGE('',*,*,#40184,.T.) ;
#54241=ORIENTED_EDGE('',*,*,#39970,.F.) ;
#54242=ORIENTED_EDGE('',*,*,#40186,.F.) ;
#54243=ORIENTED_EDGE('',*,*,#39708,.F.) ;
#54244=ORIENTED_EDGE('',*,*,#40185,.T.) ;
#54245=ORIENTED_EDGE('',*,*,#39720,.F.) ;
#54246=ORIENTED_EDGE('',*,*,#40187,.F.) ;
#54247=ORIENTED_EDGE('',*,*,#40186,.T.) ;
#54248=ORIENTED_EDGE('',*,*,#39969,.F.) ;
#54249=ORIENTED_EDGE('',*,*,#40188,.F.) ;
#54250=ORIENTED_EDGE('',*,*,#39705,.F.) ;
#54251=ORIENTED_EDGE('',*,*,#40187,.T.) ;
#54252=ORIENTED_EDGE('',*,*,#39723,.F.) ;
#54253=ORIENTED_EDGE('',*,*,#40189,.F.) ;
#54254=ORIENTED_EDGE('',*,*,#39973,.F.) ;
#54255=ORIENTED_EDGE('',*,*,#39702,.F.) ;
#54256=ORIENTED_EDGE('',*,*,#40188,.T.) ;
#54257=ORIENTED_EDGE('',*,*,#40190,.F.) ;
#54258=ORIENTED_EDGE('',*,*,#40189,.T.) ;
#54259=ORIENTED_EDGE('',*,*,#39726,.F.) ;
#54260=ORIENTED_EDGE('',*,*,#40191,.F.) ;
#54261=ORIENTED_EDGE('',*,*,#39974,.F.) ;
#54262=ORIENTED_EDGE('',*,*,#40190,.T.) ;
#54263=ORIENTED_EDGE('',*,*,#39968,.F.) ;
#54264=ORIENTED_EDGE('',*,*,#40192,.F.) ;
#54265=ORIENTED_EDGE('',*,*,#39697,.F.) ;
#54266=ORIENTED_EDGE('',*,*,#40191,.T.) ;
#54267=ORIENTED_EDGE('',*,*,#39729,.F.) ;
#54268=ORIENTED_EDGE('',*,*,#40193,.F.) ;
#54269=ORIENTED_EDGE('',*,*,#39975,.F.) ;
#54270=ORIENTED_EDGE('',*,*,#39647,.F.) ;
#54271=ORIENTED_EDGE('',*,*,#40192,.T.) ;
#54272=ORIENTED_EDGE('',*,*,#40194,.F.) ;
#54273=ORIENTED_EDGE('',*,*,#40193,.T.) ;
#54274=ORIENTED_EDGE('',*,*,#39732,.F.) ;
#54275=ORIENTED_EDGE('',*,*,#40195,.F.) ;
#54276=ORIENTED_EDGE('',*,*,#40194,.T.) ;
#54277=ORIENTED_EDGE('',*,*,#39967,.F.) ;
#54278=ORIENTED_EDGE('',*,*,#40196,.F.) ;
#54279=ORIENTED_EDGE('',*,*,#39595,.F.) ;
#54280=ORIENTED_EDGE('',*,*,#40195,.T.) ;
#54281=ORIENTED_EDGE('',*,*,#39734,.F.) ;
#54282=ORIENTED_EDGE('',*,*,#40197,.F.) ;
#54283=ORIENTED_EDGE('',*,*,#39966,.F.) ;
#54284=ORIENTED_EDGE('',*,*,#39589,.F.) ;
#54285=ORIENTED_EDGE('',*,*,#40196,.T.) ;
#54286=ORIENTED_EDGE('',*,*,#40197,.T.) ;
#54287=ORIENTED_EDGE('',*,*,#40198,.F.) ;
#54288=ORIENTED_EDGE('',*,*,#39715,.F.) ;
#54289=ORIENTED_EDGE('',*,*,#40199,.F.) ;
#54290=ORIENTED_EDGE('',*,*,#40199,.T.) ;
#54291=ORIENTED_EDGE('',*,*,#39712,.F.) ;
#54292=ORIENTED_EDGE('',*,*,#40200,.F.) ;
#54293=ORIENTED_EDGE('',*,*,#39983,.F.) ;
#54294=ORIENTED_EDGE('',*,*,#40198,.T.) ;
#54295=ORIENTED_EDGE('',*,*,#39982,.F.) ;
#54296=ORIENTED_EDGE('',*,*,#40201,.F.) ;
#54297=ORIENTED_EDGE('',*,*,#39718,.F.) ;
#54298=ORIENTED_EDGE('',*,*,#40200,.T.) ;
#54299=ORIENTED_EDGE('',*,*,#39709,.F.) ;
#54300=ORIENTED_EDGE('',*,*,#40202,.F.) ;
#54301=ORIENTED_EDGE('',*,*,#39984,.F.) ;
#54302=ORIENTED_EDGE('',*,*,#39721,.F.) ;
#54303=ORIENTED_EDGE('',*,*,#40201,.T.) ;
#54304=ORIENTED_EDGE('',*,*,#40203,.F.) ;
#54305=ORIENTED_EDGE('',*,*,#40202,.T.) ;
#54306=ORIENTED_EDGE('',*,*,#39706,.F.) ;
#54307=ORIENTED_EDGE('',*,*,#40204,.F.) ;
#54308=ORIENTED_EDGE('',*,*,#39985,.F.) ;
#54309=ORIENTED_EDGE('',*,*,#40203,.T.) ;
#54310=ORIENTED_EDGE('',*,*,#39981,.F.) ;
#54311=ORIENTED_EDGE('',*,*,#40205,.F.) ;
#54312=ORIENTED_EDGE('',*,*,#39724,.F.) ;
#54313=ORIENTED_EDGE('',*,*,#40204,.T.) ;
#54314=ORIENTED_EDGE('',*,*,#39703,.F.) ;
#54315=ORIENTED_EDGE('',*,*,#40206,.F.) ;
#54316=ORIENTED_EDGE('',*,*,#40205,.T.) ;
#54317=ORIENTED_EDGE('',*,*,#39980,.F.) ;
#54318=ORIENTED_EDGE('',*,*,#40207,.F.) ;
#54319=ORIENTED_EDGE('',*,*,#39727,.F.) ;
#54320=ORIENTED_EDGE('',*,*,#40206,.T.) ;
#54321=ORIENTED_EDGE('',*,*,#39695,.F.) ;
#54322=ORIENTED_EDGE('',*,*,#40208,.F.) ;
#54323=ORIENTED_EDGE('',*,*,#39976,.F.) ;
#54324=ORIENTED_EDGE('',*,*,#40207,.T.) ;
#54325=ORIENTED_EDGE('',*,*,#39979,.F.) ;
#54326=ORIENTED_EDGE('',*,*,#40209,.F.) ;
#54327=ORIENTED_EDGE('',*,*,#39730,.F.) ;
#54328=ORIENTED_EDGE('',*,*,#40208,.T.) ;
#54329=ORIENTED_EDGE('',*,*,#39587,.F.) ;
#54330=ORIENTED_EDGE('',*,*,#40210,.F.) ;
#54331=ORIENTED_EDGE('',*,*,#39733,.F.) ;
#54332=ORIENTED_EDGE('',*,*,#40209,.T.) ;
#54333=ORIENTED_EDGE('',*,*,#40211,.F.) ;
#54334=ORIENTED_EDGE('',*,*,#40210,.T.) ;
#54335=ORIENTED_EDGE('',*,*,#39596,.F.) ;
#54336=ORIENTED_EDGE('',*,*,#40212,.F.) ;
#54337=ORIENTED_EDGE('',*,*,#39977,.F.) ;
#54338=ORIENTED_EDGE('',*,*,#40211,.T.) ;
#54339=ORIENTED_EDGE('',*,*,#39978,.F.) ;
#54340=ORIENTED_EDGE('',*,*,#40213,.F.) ;
#54341=ORIENTED_EDGE('',*,*,#39735,.F.) ;
#54342=ORIENTED_EDGE('',*,*,#40212,.T.) ;
#54343=ORIENTED_EDGE('',*,*,#39591,.F.) ;
#54344=ORIENTED_EDGE('',*,*,#40213,.T.) ;
#54345=ORIENTED_EDGE('',*,*,#40214,.F.) ;
#54346=ORIENTED_EDGE('',*,*,#40056,.F.) ;
#54347=ORIENTED_EDGE('',*,*,#40215,.F.) ;
#54348=ORIENTED_EDGE('',*,*,#40103,.F.) ;
#54349=ORIENTED_EDGE('',*,*,#40215,.T.) ;
#54350=ORIENTED_EDGE('',*,*,#40053,.F.) ;
#54351=ORIENTED_EDGE('',*,*,#40216,.F.) ;
#54352=ORIENTED_EDGE('',*,*,#40104,.F.) ;
#54353=ORIENTED_EDGE('',*,*,#40059,.F.) ;
#54354=ORIENTED_EDGE('',*,*,#40214,.T.) ;
#54355=ORIENTED_EDGE('',*,*,#40217,.F.) ;
#54356=ORIENTED_EDGE('',*,*,#40216,.T.) ;
#54357=ORIENTED_EDGE('',*,*,#40050,.F.) ;
#54358=ORIENTED_EDGE('',*,*,#40218,.F.) ;
#54359=ORIENTED_EDGE('',*,*,#40105,.F.) ;
#54360=ORIENTED_EDGE('',*,*,#40217,.T.) ;
#54361=ORIENTED_EDGE('',*,*,#40102,.F.) ;
#54362=ORIENTED_EDGE('',*,*,#40219,.F.) ;
#54363=ORIENTED_EDGE('',*,*,#40062,.F.) ;
#54364=ORIENTED_EDGE('',*,*,#40218,.T.) ;
#54365=ORIENTED_EDGE('',*,*,#40047,.F.) ;
#54366=ORIENTED_EDGE('',*,*,#40220,.F.) ;
#54367=ORIENTED_EDGE('',*,*,#40106,.F.) ;
#54368=ORIENTED_EDGE('',*,*,#40065,.F.) ;
#54369=ORIENTED_EDGE('',*,*,#40219,.T.) ;
#54370=ORIENTED_EDGE('',*,*,#40221,.F.) ;
#54371=ORIENTED_EDGE('',*,*,#40220,.T.) ;
#54372=ORIENTED_EDGE('',*,*,#40044,.F.) ;
#54373=ORIENTED_EDGE('',*,*,#40222,.F.) ;
#54374=ORIENTED_EDGE('',*,*,#40107,.F.) ;
#54375=ORIENTED_EDGE('',*,*,#40221,.T.) ;
#54376=ORIENTED_EDGE('',*,*,#40101,.F.) ;
#54377=ORIENTED_EDGE('',*,*,#40223,.F.) ;
#54378=ORIENTED_EDGE('',*,*,#40068,.F.) ;
#54379=ORIENTED_EDGE('',*,*,#40222,.T.) ;
#54380=ORIENTED_EDGE('',*,*,#40041,.F.) ;
#54381=ORIENTED_EDGE('',*,*,#40224,.F.) ;
#54382=ORIENTED_EDGE('',*,*,#40071,.F.) ;
#54383=ORIENTED_EDGE('',*,*,#40223,.T.) ;
#54384=ORIENTED_EDGE('',*,*,#40225,.F.) ;
#54385=ORIENTED_EDGE('',*,*,#40224,.T.) ;
#54386=ORIENTED_EDGE('',*,*,#40038,.F.) ;
#54387=ORIENTED_EDGE('',*,*,#40226,.F.) ;
#54388=ORIENTED_EDGE('',*,*,#40108,.F.) ;
#54389=ORIENTED_EDGE('',*,*,#40225,.T.) ;
#54390=ORIENTED_EDGE('',*,*,#40100,.F.) ;
#54391=ORIENTED_EDGE('',*,*,#40227,.F.) ;
#54392=ORIENTED_EDGE('',*,*,#40074,.F.) ;
#54393=ORIENTED_EDGE('',*,*,#40226,.T.) ;
#54394=ORIENTED_EDGE('',*,*,#39335,.F.) ;
#54395=ORIENTED_EDGE('',*,*,#40228,.F.) ;
#54396=ORIENTED_EDGE('',*,*,#40077,.F.) ;
#54397=ORIENTED_EDGE('',*,*,#40227,.T.) ;
#54398=ORIENTED_EDGE('',*,*,#40229,.F.) ;
#54399=ORIENTED_EDGE('',*,*,#40228,.T.) ;
#54400=ORIENTED_EDGE('',*,*,#40036,.F.) ;
#54401=ORIENTED_EDGE('',*,*,#39326,.F.) ;
#54402=ORIENTED_EDGE('',*,*,#40109,.F.) ;
#54403=ORIENTED_EDGE('',*,*,#40229,.T.) ;
#54404=ORIENTED_EDGE('',*,*,#40099,.F.) ;
#54405=ORIENTED_EDGE('',*,*,#40230,.F.) ;
#54406=ORIENTED_EDGE('',*,*,#40080,.F.) ;
#54407=ORIENTED_EDGE('',*,*,#40083,.F.) ;
#54408=ORIENTED_EDGE('',*,*,#40230,.T.) ;
#54409=ORIENTED_EDGE('',*,*,#40231,.F.) ;
#54410=ORIENTED_EDGE('',*,*,#39325,.T.) ;
#54411=ORIENTED_EDGE('',*,*,#40031,.F.) ;
#54412=ORIENTED_EDGE('',*,*,#40232,.F.) ;
#54413=ORIENTED_EDGE('',*,*,#40110,.F.) ;
#54414=ORIENTED_EDGE('',*,*,#40231,.T.) ;
#54415=ORIENTED_EDGE('',*,*,#40098,.F.) ;
#54416=ORIENTED_EDGE('',*,*,#40233,.F.) ;
#54417=ORIENTED_EDGE('',*,*,#40086,.F.) ;
#54418=ORIENTED_EDGE('',*,*,#40232,.T.) ;
#54419=ORIENTED_EDGE('',*,*,#40028,.F.) ;
#54420=ORIENTED_EDGE('',*,*,#40234,.F.) ;
#54421=ORIENTED_EDGE('',*,*,#40089,.F.) ;
#54422=ORIENTED_EDGE('',*,*,#40233,.T.) ;
#54423=ORIENTED_EDGE('',*,*,#40235,.F.) ;
#54424=ORIENTED_EDGE('',*,*,#40234,.T.) ;
#54425=ORIENTED_EDGE('',*,*,#40025,.F.) ;
#54426=ORIENTED_EDGE('',*,*,#40236,.F.) ;
#54427=ORIENTED_EDGE('',*,*,#40111,.F.) ;
#54428=ORIENTED_EDGE('',*,*,#40235,.T.) ;
#54429=ORIENTED_EDGE('',*,*,#40097,.F.) ;
#54430=ORIENTED_EDGE('',*,*,#40237,.F.) ;
#54431=ORIENTED_EDGE('',*,*,#40092,.F.) ;
#54432=ORIENTED_EDGE('',*,*,#40236,.T.) ;
#54433=ORIENTED_EDGE('',*,*,#40022,.F.) ;
#54434=ORIENTED_EDGE('',*,*,#40238,.F.) ;
#54435=ORIENTED_EDGE('',*,*,#40094,.F.) ;
#54436=ORIENTED_EDGE('',*,*,#40237,.T.) ;
#54437=ORIENTED_EDGE('',*,*,#40096,.F.) ;
#54438=ORIENTED_EDGE('',*,*,#40239,.F.) ;
#54439=ORIENTED_EDGE('',*,*,#40016,.F.) ;
#54440=ORIENTED_EDGE('',*,*,#40238,.T.) ;
#54441=ORIENTED_EDGE('',*,*,#40019,.F.) ;
#54442=ORIENTED_EDGE('',*,*,#40239,.T.) ;
#54443=ORIENTED_EDGE('',*,*,#40095,.F.) ;
#54444=ORIENTED_EDGE('',*,*,#40240,.F.) ;
#54445=ORIENTED_EDGE('',*,*,#40052,.F.) ;
#54446=ORIENTED_EDGE('',*,*,#40241,.F.) ;
#54447=ORIENTED_EDGE('',*,*,#39954,.F.) ;
#54448=ORIENTED_EDGE('',*,*,#40049,.F.) ;
#54449=ORIENTED_EDGE('',*,*,#40240,.T.) ;
#54450=ORIENTED_EDGE('',*,*,#40242,.F.) ;
#54451=ORIENTED_EDGE('',*,*,#40241,.T.) ;
#54452=ORIENTED_EDGE('',*,*,#40055,.F.) ;
#54453=ORIENTED_EDGE('',*,*,#40243,.F.) ;
#54454=ORIENTED_EDGE('',*,*,#40242,.T.) ;
#54455=ORIENTED_EDGE('',*,*,#39953,.F.) ;
#54456=ORIENTED_EDGE('',*,*,#40244,.F.) ;
#54457=ORIENTED_EDGE('',*,*,#40046,.F.) ;
#54458=ORIENTED_EDGE('',*,*,#40243,.T.) ;
#54459=ORIENTED_EDGE('',*,*,#40058,.F.) ;
#54460=ORIENTED_EDGE('',*,*,#40245,.F.) ;
#54461=ORIENTED_EDGE('',*,*,#39955,.F.) ;
#54462=ORIENTED_EDGE('',*,*,#40244,.T.) ;
#54463=ORIENTED_EDGE('',*,*,#39952,.F.) ;
#54464=ORIENTED_EDGE('',*,*,#40246,.F.) ;
#54465=ORIENTED_EDGE('',*,*,#40043,.F.) ;
#54466=ORIENTED_EDGE('',*,*,#40245,.T.) ;
#54467=ORIENTED_EDGE('',*,*,#40061,.F.) ;
#54468=ORIENTED_EDGE('',*,*,#40247,.F.) ;
#54469=ORIENTED_EDGE('',*,*,#39956,.F.) ;
#54470=ORIENTED_EDGE('',*,*,#40246,.T.) ;
#54471=ORIENTED_EDGE('',*,*,#39951,.F.) ;
#54472=ORIENTED_EDGE('',*,*,#39320,.F.) ;
#54473=ORIENTED_EDGE('',*,*,#40040,.F.) ;
#54474=ORIENTED_EDGE('',*,*,#40247,.T.) ;
#54475=ORIENTED_EDGE('',*,*,#40064,.F.) ;
#54476=ORIENTED_EDGE('',*,*,#40248,.F.) ;
#54477=ORIENTED_EDGE('',*,*,#39957,.F.) ;
#54478=ORIENTED_EDGE('',*,*,#40248,.T.) ;
#54479=ORIENTED_EDGE('',*,*,#40067,.F.) ;
#54480=ORIENTED_EDGE('',*,*,#40249,.F.) ;
#54481=ORIENTED_EDGE('',*,*,#39958,.F.) ;
#54482=ORIENTED_EDGE('',*,*,#39318,.T.) ;
#54483=ORIENTED_EDGE('',*,*,#39950,.F.) ;
#54484=ORIENTED_EDGE('',*,*,#40250,.F.) ;
#54485=ORIENTED_EDGE('',*,*,#40037,.F.) ;
#54486=ORIENTED_EDGE('',*,*,#40249,.T.) ;
#54487=ORIENTED_EDGE('',*,*,#40070,.F.) ;
#54488=ORIENTED_EDGE('',*,*,#40251,.F.) ;
#54489=ORIENTED_EDGE('',*,*,#39959,.F.) ;
#54490=ORIENTED_EDGE('',*,*,#40250,.T.) ;
#54491=ORIENTED_EDGE('',*,*,#39949,.F.) ;
#54492=ORIENTED_EDGE('',*,*,#40252,.F.) ;
#54493=ORIENTED_EDGE('',*,*,#40035,.F.) ;
#54494=ORIENTED_EDGE('',*,*,#40251,.T.) ;
#54495=ORIENTED_EDGE('',*,*,#40073,.F.) ;
#54496=ORIENTED_EDGE('',*,*,#40253,.F.) ;
#54497=ORIENTED_EDGE('',*,*,#39960,.F.) ;
#54498=ORIENTED_EDGE('',*,*,#40252,.T.) ;
#54499=ORIENTED_EDGE('',*,*,#39948,.F.) ;
#54500=ORIENTED_EDGE('',*,*,#40254,.F.) ;
#54501=ORIENTED_EDGE('',*,*,#40033,.F.) ;
#54502=ORIENTED_EDGE('',*,*,#40253,.T.) ;
#54503=ORIENTED_EDGE('',*,*,#40076,.F.) ;
#54504=ORIENTED_EDGE('',*,*,#40255,.F.) ;
#54505=ORIENTED_EDGE('',*,*,#39961,.F.) ;
#54506=ORIENTED_EDGE('',*,*,#40254,.T.) ;
#54507=ORIENTED_EDGE('',*,*,#39947,.F.) ;
#54508=ORIENTED_EDGE('',*,*,#40256,.F.) ;
#54509=ORIENTED_EDGE('',*,*,#40030,.F.) ;
#54510=ORIENTED_EDGE('',*,*,#40255,.T.) ;
#54511=ORIENTED_EDGE('',*,*,#40079,.F.) ;
#54512=ORIENTED_EDGE('',*,*,#40257,.F.) ;
#54513=ORIENTED_EDGE('',*,*,#39962,.F.) ;
#54514=ORIENTED_EDGE('',*,*,#40256,.T.) ;
#54515=ORIENTED_EDGE('',*,*,#39946,.F.) ;
#54516=ORIENTED_EDGE('',*,*,#40258,.F.) ;
#54517=ORIENTED_EDGE('',*,*,#40027,.F.) ;
#54518=ORIENTED_EDGE('',*,*,#40257,.T.) ;
#54519=ORIENTED_EDGE('',*,*,#40082,.F.) ;
#54520=ORIENTED_EDGE('',*,*,#40259,.F.) ;
#54521=ORIENTED_EDGE('',*,*,#39963,.F.) ;
#54522=ORIENTED_EDGE('',*,*,#40024,.F.) ;
#54523=ORIENTED_EDGE('',*,*,#40258,.T.) ;
#54524=ORIENTED_EDGE('',*,*,#40260,.F.) ;
#54525=ORIENTED_EDGE('',*,*,#40259,.T.) ;
#54526=ORIENTED_EDGE('',*,*,#40085,.F.) ;
#54527=ORIENTED_EDGE('',*,*,#40261,.F.) ;
#54528=ORIENTED_EDGE('',*,*,#39964,.F.) ;
#54529=ORIENTED_EDGE('',*,*,#40260,.T.) ;
#54530=ORIENTED_EDGE('',*,*,#39945,.F.) ;
#54531=ORIENTED_EDGE('',*,*,#40262,.F.) ;
#54532=ORIENTED_EDGE('',*,*,#40021,.F.) ;
#54533=ORIENTED_EDGE('',*,*,#40261,.T.) ;
#54534=ORIENTED_EDGE('',*,*,#40088,.F.) ;
#54535=ORIENTED_EDGE('',*,*,#40263,.F.) ;
#54536=ORIENTED_EDGE('',*,*,#39965,.F.) ;
#54537=ORIENTED_EDGE('',*,*,#40018,.F.) ;
#54538=ORIENTED_EDGE('',*,*,#40262,.T.) ;
#54539=ORIENTED_EDGE('',*,*,#40264,.F.) ;
#54540=ORIENTED_EDGE('',*,*,#40263,.T.) ;
#54541=ORIENTED_EDGE('',*,*,#40091,.F.) ;
#54542=ORIENTED_EDGE('',*,*,#40265,.F.) ;
#54543=ORIENTED_EDGE('',*,*,#39943,.F.) ;
#54544=ORIENTED_EDGE('',*,*,#40264,.T.) ;
#54545=ORIENTED_EDGE('',*,*,#39944,.F.) ;
#54546=ORIENTED_EDGE('',*,*,#40265,.T.) ;
#54547=ORIENTED_EDGE('',*,*,#40093,.F.) ;
#54548=ORIENTED_EDGE('',*,*,#40266,.T.) ;
#54549=ORIENTED_EDGE('',*,*,#40267,.T.) ;
#54550=ORIENTED_EDGE('',*,*,#40268,.T.) ;
#54551=ORIENTED_EDGE('',*,*,#40269,.T.) ;
#54552=ORIENTED_EDGE('',*,*,#40270,.T.) ;
#54553=ORIENTED_EDGE('',*,*,#40271,.T.) ;
#54554=ORIENTED_EDGE('',*,*,#40272,.T.) ;
#54555=ORIENTED_EDGE('',*,*,#40273,.T.) ;
#54556=ORIENTED_EDGE('',*,*,#40274,.T.) ;
#54557=ORIENTED_EDGE('',*,*,#40275,.T.) ;
#54558=ORIENTED_EDGE('',*,*,#40276,.T.) ;
#54559=ORIENTED_EDGE('',*,*,#40277,.T.) ;
#54560=ORIENTED_EDGE('',*,*,#40278,.T.) ;
#54561=ORIENTED_EDGE('',*,*,#40279,.T.) ;
#54562=ORIENTED_EDGE('',*,*,#40280,.T.) ;
#54563=ORIENTED_EDGE('',*,*,#40281,.T.) ;
#54564=ORIENTED_EDGE('',*,*,#40282,.T.) ;
#54565=ORIENTED_EDGE('',*,*,#40283,.T.) ;
#54566=ORIENTED_EDGE('',*,*,#40284,.F.) ;
#54567=ORIENTED_EDGE('',*,*,#40285,.T.) ;
#54568=ORIENTED_EDGE('',*,*,#40286,.T.) ;
#54569=ORIENTED_EDGE('',*,*,#40287,.T.) ;
#54570=ORIENTED_EDGE('',*,*,#40134,.T.) ;
#54571=ORIENTED_EDGE('',*,*,#40288,.T.) ;
#54572=ORIENTED_EDGE('',*,*,#40289,.T.) ;
#54573=ORIENTED_EDGE('',*,*,#40290,.T.) ;
#54574=ORIENTED_EDGE('',*,*,#40291,.T.) ;
#54575=ORIENTED_EDGE('',*,*,#40292,.T.) ;
#54576=ORIENTED_EDGE('',*,*,#39332,.T.) ;
#54577=ORIENTED_EDGE('',*,*,#40293,.T.) ;
#54578=ORIENTED_EDGE('',*,*,#40294,.T.) ;
#54579=ORIENTED_EDGE('',*,*,#40295,.T.) ;
#54580=ORIENTED_EDGE('',*,*,#40131,.T.) ;
#54581=ORIENTED_EDGE('',*,*,#40296,.T.) ;
#54582=ORIENTED_EDGE('',*,*,#40266,.F.) ;
#54583=ORIENTED_EDGE('',*,*,#40297,.T.) ;
#54584=ORIENTED_EDGE('',*,*,#40132,.T.) ;
#54585=ORIENTED_EDGE('',*,*,#40284,.T.) ;
#54586=ORIENTED_EDGE('',*,*,#40298,.T.) ;
#54587=ORIENTED_EDGE('',*,*,#39565,.F.) ;
#54588=ORIENTED_EDGE('',*,*,#40299,.T.) ;
#54589=ORIENTED_EDGE('',*,*,#40300,.T.) ;
#54590=ORIENTED_EDGE('',*,*,#40301,.T.) ;
#54591=ORIENTED_EDGE('',*,*,#40302,.T.) ;
#54592=ORIENTED_EDGE('',*,*,#40303,.T.) ;
#54593=ORIENTED_EDGE('',*,*,#40304,.T.) ;
#54594=ORIENTED_EDGE('',*,*,#40305,.T.) ;
#54595=ORIENTED_EDGE('',*,*,#40114,.F.) ;
#54596=ORIENTED_EDGE('',*,*,#40306,.T.) ;
#54597=ORIENTED_EDGE('',*,*,#40118,.F.) ;
#54598=ORIENTED_EDGE('',*,*,#40307,.T.) ;
#54599=ORIENTED_EDGE('',*,*,#40308,.T.) ;
#54600=ORIENTED_EDGE('',*,*,#40309,.T.) ;
#54601=ORIENTED_EDGE('',*,*,#40310,.T.) ;
#54602=ORIENTED_EDGE('',*,*,#40311,.T.) ;
#54603=ORIENTED_EDGE('',*,*,#40312,.T.) ;
#54604=ORIENTED_EDGE('',*,*,#40313,.T.) ;
#54605=ORIENTED_EDGE('',*,*,#40314,.T.) ;
#54606=ORIENTED_EDGE('',*,*,#40315,.T.) ;
#54607=ORIENTED_EDGE('',*,*,#40316,.T.) ;
#54608=ORIENTED_EDGE('',*,*,#40317,.T.) ;
#54609=ORIENTED_EDGE('',*,*,#40318,.T.) ;
#54610=ORIENTED_EDGE('',*,*,#40319,.T.) ;
#54611=ORIENTED_EDGE('',*,*,#40112,.T.) ;
#54612=ORIENTED_EDGE('',*,*,#40320,.T.) ;
#54613=ORIENTED_EDGE('',*,*,#40116,.F.) ;
#54614=ORIENTED_EDGE('',*,*,#40321,.T.) ;
#54615=ORIENTED_EDGE('',*,*,#40322,.T.) ;
#54616=ORIENTED_EDGE('',*,*,#40323,.T.) ;
#54617=ORIENTED_EDGE('',*,*,#40324,.T.) ;
#54618=ORIENTED_EDGE('',*,*,#40325,.T.) ;
#54619=ORIENTED_EDGE('',*,*,#40326,.T.) ;
#54620=ORIENTED_EDGE('',*,*,#40327,.T.) ;
#54621=ORIENTED_EDGE('',*,*,#40328,.T.) ;
#54622=ORIENTED_EDGE('',*,*,#40329,.T.) ;
#54623=ORIENTED_EDGE('',*,*,#40330,.T.) ;
#54624=ORIENTED_EDGE('',*,*,#40331,.T.) ;
#54625=ORIENTED_EDGE('',*,*,#40332,.T.) ;
#54626=ORIENTED_EDGE('',*,*,#40333,.T.) ;
#54627=ORIENTED_EDGE('',*,*,#40334,.T.) ;
#54628=ORIENTED_EDGE('',*,*,#40335,.T.) ;
#54629=ORIENTED_EDGE('',*,*,#40336,.T.) ;
#54630=ORIENTED_EDGE('',*,*,#40337,.T.) ;
#54631=ORIENTED_EDGE('',*,*,#40338,.T.) ;
#54632=ORIENTED_EDGE('',*,*,#40339,.T.) ;
#54633=ORIENTED_EDGE('',*,*,#40326,.F.) ;
#54634=ORIENTED_EDGE('',*,*,#40340,.T.) ;
#54635=ORIENTED_EDGE('',*,*,#40281,.F.) ;
#54636=ORIENTED_EDGE('',*,*,#40341,.F.) ;
#54637=ORIENTED_EDGE('',*,*,#40278,.F.) ;
#54638=ORIENTED_EDGE('',*,*,#40342,.T.) ;
#54639=ORIENTED_EDGE('',*,*,#40282,.F.) ;
#54640=ORIENTED_EDGE('',*,*,#40343,.T.) ;
#54641=ORIENTED_EDGE('',*,*,#40344,.F.) ;
#54642=ORIENTED_EDGE('',*,*,#40341,.T.) ;
#54643=ORIENTED_EDGE('',*,*,#40345,.F.) ;
#54644=ORIENTED_EDGE('',*,*,#40279,.F.) ;
#54645=ORIENTED_EDGE('',*,*,#40346,.T.) ;
#54646=ORIENTED_EDGE('',*,*,#40328,.F.) ;
#54647=ORIENTED_EDGE('',*,*,#40347,.F.) ;
#54648=ORIENTED_EDGE('',*,*,#40345,.T.) ;
#54649=ORIENTED_EDGE('',*,*,#40280,.F.) ;
#54650=ORIENTED_EDGE('',*,*,#40348,.F.) ;
#54651=ORIENTED_EDGE('',*,*,#40274,.F.) ;
#54652=ORIENTED_EDGE('',*,*,#40344,.T.) ;
#54653=ORIENTED_EDGE('',*,*,#40277,.F.) ;
#54654=ORIENTED_EDGE('',*,*,#40349,.F.) ;
#54655=ORIENTED_EDGE('',*,*,#40327,.F.) ;
#54656=ORIENTED_EDGE('',*,*,#40348,.T.) ;
#54657=ORIENTED_EDGE('',*,*,#40347,.T.) ;
#54658=ORIENTED_EDGE('',*,*,#40350,.F.) ;
#54659=ORIENTED_EDGE('',*,*,#40351,.F.) ;
#54660=ORIENTED_EDGE('',*,*,#40349,.T.) ;
#54661=ORIENTED_EDGE('',*,*,#40352,.F.) ;
#54662=ORIENTED_EDGE('',*,*,#40350,.T.) ;
#54663=ORIENTED_EDGE('',*,*,#40331,.F.) ;
#54664=ORIENTED_EDGE('',*,*,#40353,.F.) ;
#54665=ORIENTED_EDGE('',*,*,#40275,.F.) ;
#54666=ORIENTED_EDGE('',*,*,#40352,.T.) ;
#54667=ORIENTED_EDGE('',*,*,#40276,.F.) ;
#54668=ORIENTED_EDGE('',*,*,#40354,.F.) ;
#54669=ORIENTED_EDGE('',*,*,#40270,.F.) ;
#54670=ORIENTED_EDGE('',*,*,#40273,.F.) ;
#54671=ORIENTED_EDGE('',*,*,#40355,.T.) ;
#54672=ORIENTED_EDGE('',*,*,#40324,.F.) ;
#54673=ORIENTED_EDGE('',*,*,#40351,.T.) ;
#54674=ORIENTED_EDGE('',*,*,#40354,.T.) ;
#54675=ORIENTED_EDGE('',*,*,#40353,.T.) ;
#54676=ORIENTED_EDGE('',*,*,#40356,.F.) ;
#54677=ORIENTED_EDGE('',*,*,#40268,.F.) ;
#54678=ORIENTED_EDGE('',*,*,#40357,.T.) ;
#54679=ORIENTED_EDGE('',*,*,#40272,.F.) ;
#54680=ORIENTED_EDGE('',*,*,#40358,.T.) ;
#54681=ORIENTED_EDGE('',*,*,#40330,.F.) ;
#54682=ORIENTED_EDGE('',*,*,#40359,.T.) ;
#54683=ORIENTED_EDGE('',*,*,#40271,.F.) ;
#54684=ORIENTED_EDGE('',*,*,#40356,.T.) ;
#54685=ORIENTED_EDGE('',*,*,#40334,.F.) ;
#54686=ORIENTED_EDGE('',*,*,#40360,.T.) ;
#54687=ORIENTED_EDGE('',*,*,#40303,.F.) ;
#54688=ORIENTED_EDGE('',*,*,#40361,.F.) ;
#54689=ORIENTED_EDGE('',*,*,#40300,.F.) ;
#54690=ORIENTED_EDGE('',*,*,#40362,.T.) ;
#54691=ORIENTED_EDGE('',*,*,#40304,.F.) ;
#54692=ORIENTED_EDGE('',*,*,#40363,.T.) ;
#54693=ORIENTED_EDGE('',*,*,#40364,.F.) ;
#54694=ORIENTED_EDGE('',*,*,#40361,.T.) ;
#54695=ORIENTED_EDGE('',*,*,#40365,.F.) ;
#54696=ORIENTED_EDGE('',*,*,#40301,.F.) ;
#54697=ORIENTED_EDGE('',*,*,#40366,.T.) ;
#54698=ORIENTED_EDGE('',*,*,#40336,.F.) ;
#54699=ORIENTED_EDGE('',*,*,#40367,.F.) ;
#54700=ORIENTED_EDGE('',*,*,#40365,.T.) ;
#54701=ORIENTED_EDGE('',*,*,#40302,.F.) ;
#54702=ORIENTED_EDGE('',*,*,#40368,.F.) ;
#54703=ORIENTED_EDGE('',*,*,#40316,.F.) ;
#54704=ORIENTED_EDGE('',*,*,#40364,.T.) ;
#54705=ORIENTED_EDGE('',*,*,#40315,.F.) ;
#54706=ORIENTED_EDGE('',*,*,#40369,.F.) ;
#54707=ORIENTED_EDGE('',*,*,#40335,.F.) ;
#54708=ORIENTED_EDGE('',*,*,#40368,.T.) ;
#54709=ORIENTED_EDGE('',*,*,#40367,.T.) ;
#54710=ORIENTED_EDGE('',*,*,#40370,.F.) ;
#54711=ORIENTED_EDGE('',*,*,#40371,.F.) ;
#54712=ORIENTED_EDGE('',*,*,#40369,.T.) ;
#54713=ORIENTED_EDGE('',*,*,#40372,.F.) ;
#54714=ORIENTED_EDGE('',*,*,#40370,.T.) ;
#54715=ORIENTED_EDGE('',*,*,#40339,.F.) ;
#54716=ORIENTED_EDGE('',*,*,#40373,.F.) ;
#54717=ORIENTED_EDGE('',*,*,#40317,.F.) ;
#54718=ORIENTED_EDGE('',*,*,#40372,.T.) ;
#54719=ORIENTED_EDGE('',*,*,#40314,.F.) ;
#54720=ORIENTED_EDGE('',*,*,#40374,.F.) ;
#54721=ORIENTED_EDGE('',*,*,#40310,.F.) ;
#54722=ORIENTED_EDGE('',*,*,#40313,.F.) ;
#54723=ORIENTED_EDGE('',*,*,#40375,.T.) ;
#54724=ORIENTED_EDGE('',*,*,#40332,.F.) ;
#54725=ORIENTED_EDGE('',*,*,#40371,.T.) ;
#54726=ORIENTED_EDGE('',*,*,#40374,.T.) ;
#54727=ORIENTED_EDGE('',*,*,#40373,.T.) ;
#54728=ORIENTED_EDGE('',*,*,#40376,.F.) ;
#54729=ORIENTED_EDGE('',*,*,#40308,.F.) ;
#54730=ORIENTED_EDGE('',*,*,#40377,.T.) ;
#54731=ORIENTED_EDGE('',*,*,#40312,.F.) ;
#54732=ORIENTED_EDGE('',*,*,#40378,.T.) ;
#54733=ORIENTED_EDGE('',*,*,#40338,.F.) ;
#54734=ORIENTED_EDGE('',*,*,#40379,.T.) ;
#54735=ORIENTED_EDGE('',*,*,#40311,.F.) ;
#54736=ORIENTED_EDGE('',*,*,#40376,.T.) ;
#54737=ORIENTED_EDGE('',*,*,#39566,.F.) ;
#54738=ORIENTED_EDGE('',*,*,#40298,.F.) ;
#54739=ORIENTED_EDGE('',*,*,#40380,.F.) ;
#54740=ORIENTED_EDGE('',*,*,#40293,.F.) ;
#54741=ORIENTED_EDGE('',*,*,#40380,.T.) ;
#54742=ORIENTED_EDGE('',*,*,#40283,.F.) ;
#54743=ORIENTED_EDGE('',*,*,#40381,.F.) ;
#54744=ORIENTED_EDGE('',*,*,#40294,.F.) ;
#54745=ORIENTED_EDGE('',*,*,#40381,.T.) ;
#54746=ORIENTED_EDGE('',*,*,#40342,.F.) ;
#54747=ORIENTED_EDGE('',*,*,#40340,.F.) ;
#54748=ORIENTED_EDGE('',*,*,#40382,.F.) ;
#54749=ORIENTED_EDGE('',*,*,#40382,.T.) ;
#54750=ORIENTED_EDGE('',*,*,#40325,.F.) ;
#54751=ORIENTED_EDGE('',*,*,#40383,.F.) ;
#54752=ORIENTED_EDGE('',*,*,#40295,.F.) ;
#54753=ORIENTED_EDGE('',*,*,#40383,.T.) ;
#54754=ORIENTED_EDGE('',*,*,#40355,.F.) ;
#54755=ORIENTED_EDGE('',*,*,#40357,.F.) ;
#54756=ORIENTED_EDGE('',*,*,#40384,.F.) ;
#54757=ORIENTED_EDGE('',*,*,#40384,.T.) ;
#54758=ORIENTED_EDGE('',*,*,#40267,.F.) ;
#54759=ORIENTED_EDGE('',*,*,#40385,.F.) ;
#54760=ORIENTED_EDGE('',*,*,#40291,.F.) ;
#54761=ORIENTED_EDGE('',*,*,#39333,.F.) ;
#54762=ORIENTED_EDGE('',*,*,#40292,.F.) ;
#54763=ORIENTED_EDGE('',*,*,#40385,.T.) ;
#54764=ORIENTED_EDGE('',*,*,#40296,.F.) ;
#54765=ORIENTED_EDGE('',*,*,#40130,.F.) ;
#54766=ORIENTED_EDGE('',*,*,#40133,.F.) ;
#54767=ORIENTED_EDGE('',*,*,#40297,.F.) ;
#54768=ORIENTED_EDGE('',*,*,#40386,.F.) ;
#54769=ORIENTED_EDGE('',*,*,#40288,.F.) ;
#54770=ORIENTED_EDGE('',*,*,#40386,.T.) ;
#54771=ORIENTED_EDGE('',*,*,#40269,.F.) ;
#54772=ORIENTED_EDGE('',*,*,#40387,.F.) ;
#54773=ORIENTED_EDGE('',*,*,#40289,.F.) ;
#54774=ORIENTED_EDGE('',*,*,#40387,.T.) ;
#54775=ORIENTED_EDGE('',*,*,#40358,.F.) ;
#54776=ORIENTED_EDGE('',*,*,#40359,.F.) ;
#54777=ORIENTED_EDGE('',*,*,#40388,.F.) ;
#54778=ORIENTED_EDGE('',*,*,#40388,.T.) ;
#54779=ORIENTED_EDGE('',*,*,#40329,.F.) ;
#54780=ORIENTED_EDGE('',*,*,#40389,.F.) ;
#54781=ORIENTED_EDGE('',*,*,#40290,.F.) ;
#54782=ORIENTED_EDGE('',*,*,#40389,.T.) ;
#54783=ORIENTED_EDGE('',*,*,#40346,.F.) ;
#54784=ORIENTED_EDGE('',*,*,#40343,.F.) ;
#54785=ORIENTED_EDGE('',*,*,#40390,.F.) ;
#54786=ORIENTED_EDGE('',*,*,#40390,.T.) ;
#54787=ORIENTED_EDGE('',*,*,#40285,.F.) ;
#54788=ORIENTED_EDGE('',*,*,#40391,.F.) ;
#54789=ORIENTED_EDGE('',*,*,#40286,.F.) ;
#54790=ORIENTED_EDGE('',*,*,#40391,.T.) ;
#54791=ORIENTED_EDGE('',*,*,#40299,.F.) ;
#54792=ORIENTED_EDGE('',*,*,#39564,.F.) ;
#54793=ORIENTED_EDGE('',*,*,#40287,.F.) ;
#54794=ORIENTED_EDGE('',*,*,#40115,.F.) ;
#54795=ORIENTED_EDGE('',*,*,#40305,.F.) ;
#54796=ORIENTED_EDGE('',*,*,#40392,.F.) ;
#54797=ORIENTED_EDGE('',*,*,#40321,.F.) ;
#54798=ORIENTED_EDGE('',*,*,#40392,.T.) ;
#54799=ORIENTED_EDGE('',*,*,#40362,.F.) ;
#54800=ORIENTED_EDGE('',*,*,#40360,.F.) ;
#54801=ORIENTED_EDGE('',*,*,#40393,.F.) ;
#54802=ORIENTED_EDGE('',*,*,#40393,.T.) ;
#54803=ORIENTED_EDGE('',*,*,#40333,.F.) ;
#54804=ORIENTED_EDGE('',*,*,#40394,.F.) ;
#54805=ORIENTED_EDGE('',*,*,#40322,.F.) ;
#54806=ORIENTED_EDGE('',*,*,#40394,.T.) ;
#54807=ORIENTED_EDGE('',*,*,#40375,.F.) ;
#54808=ORIENTED_EDGE('',*,*,#40377,.F.) ;
#54809=ORIENTED_EDGE('',*,*,#40395,.F.) ;
#54810=ORIENTED_EDGE('',*,*,#40117,.F.) ;
#54811=ORIENTED_EDGE('',*,*,#40323,.F.) ;
#54812=ORIENTED_EDGE('',*,*,#40395,.T.) ;
#54813=ORIENTED_EDGE('',*,*,#40307,.F.) ;
#54814=ORIENTED_EDGE('',*,*,#40396,.F.) ;
#54815=ORIENTED_EDGE('',*,*,#40306,.F.) ;
#54816=ORIENTED_EDGE('',*,*,#40113,.F.) ;
#54817=ORIENTED_EDGE('',*,*,#40319,.F.) ;
#54818=ORIENTED_EDGE('',*,*,#40363,.F.) ;
#54819=ORIENTED_EDGE('',*,*,#40396,.T.) ;
#54820=ORIENTED_EDGE('',*,*,#40397,.F.) ;
#54821=ORIENTED_EDGE('',*,*,#40366,.F.) ;
#54822=ORIENTED_EDGE('',*,*,#40397,.T.) ;
#54823=ORIENTED_EDGE('',*,*,#40318,.F.) ;
#54824=ORIENTED_EDGE('',*,*,#40398,.F.) ;
#54825=ORIENTED_EDGE('',*,*,#40337,.F.) ;
#54826=ORIENTED_EDGE('',*,*,#40119,.F.) ;
#54827=ORIENTED_EDGE('',*,*,#40309,.F.) ;
#54828=ORIENTED_EDGE('',*,*,#40399,.F.) ;
#54829=ORIENTED_EDGE('',*,*,#40320,.F.) ;
#54830=ORIENTED_EDGE('',*,*,#40379,.F.) ;
#54831=ORIENTED_EDGE('',*,*,#40398,.T.) ;
#54832=ORIENTED_EDGE('',*,*,#40399,.T.) ;
#54833=ORIENTED_EDGE('',*,*,#40378,.F.) ;
#54834=ORIENTED_EDGE('',*,*,#40400,.T.) ;
#54835=ORIENTED_EDGE('',*,*,#40401,.T.) ;
#54836=ORIENTED_EDGE('',*,*,#40402,.T.) ;
#54837=ORIENTED_EDGE('',*,*,#40403,.T.) ;
#54838=ORIENTED_EDGE('',*,*,#40404,.T.) ;
#54839=ORIENTED_EDGE('',*,*,#40405,.T.) ;
#54840=ORIENTED_EDGE('',*,*,#40406,.F.) ;
#54841=ORIENTED_EDGE('',*,*,#40407,.T.) ;
#54842=ORIENTED_EDGE('',*,*,#40408,.F.) ;
#54843=ORIENTED_EDGE('',*,*,#40409,.T.) ;
#54844=ORIENTED_EDGE('',*,*,#40410,.T.) ;
#54845=ORIENTED_EDGE('',*,*,#40411,.T.) ;
#54846=ORIENTED_EDGE('',*,*,#40412,.T.) ;
#54847=ORIENTED_EDGE('',*,*,#40413,.T.) ;
#54848=ORIENTED_EDGE('',*,*,#40414,.T.) ;
#54849=ORIENTED_EDGE('',*,*,#40415,.T.) ;
#54850=ORIENTED_EDGE('',*,*,#40416,.F.) ;
#54851=ORIENTED_EDGE('',*,*,#40417,.T.) ;
#54852=ORIENTED_EDGE('',*,*,#40418,.F.) ;
#54853=ORIENTED_EDGE('',*,*,#40419,.T.) ;
#54854=ORIENTED_EDGE('',*,*,#40420,.T.) ;
#54855=ORIENTED_EDGE('',*,*,#40421,.T.) ;
#54856=ORIENTED_EDGE('',*,*,#40422,.T.) ;
#54857=ORIENTED_EDGE('',*,*,#40423,.T.) ;
#54858=ORIENTED_EDGE('',*,*,#40424,.T.) ;
#54859=ORIENTED_EDGE('',*,*,#40425,.T.) ;
#54860=ORIENTED_EDGE('',*,*,#40426,.F.) ;
#54861=ORIENTED_EDGE('',*,*,#40427,.T.) ;
#54862=ORIENTED_EDGE('',*,*,#40428,.F.) ;
#54863=ORIENTED_EDGE('',*,*,#40429,.T.) ;
#54864=ORIENTED_EDGE('',*,*,#40430,.T.) ;
#54865=ORIENTED_EDGE('',*,*,#40431,.T.) ;
#54866=ORIENTED_EDGE('',*,*,#40432,.T.) ;
#54867=ORIENTED_EDGE('',*,*,#40433,.T.) ;
#54868=ORIENTED_EDGE('',*,*,#40434,.T.) ;
#54869=ORIENTED_EDGE('',*,*,#40435,.T.) ;
#54870=ORIENTED_EDGE('',*,*,#40436,.F.) ;
#54871=ORIENTED_EDGE('',*,*,#40437,.T.) ;
#54872=ORIENTED_EDGE('',*,*,#40438,.F.) ;
#54873=ORIENTED_EDGE('',*,*,#40439,.T.) ;
#54874=ORIENTED_EDGE('',*,*,#40440,.T.) ;
#54875=ORIENTED_EDGE('',*,*,#40441,.T.) ;
#54876=ORIENTED_EDGE('',*,*,#40442,.T.) ;
#54877=ORIENTED_EDGE('',*,*,#40443,.T.) ;
#54878=ORIENTED_EDGE('',*,*,#40444,.T.) ;
#54879=ORIENTED_EDGE('',*,*,#40445,.T.) ;
#54880=ORIENTED_EDGE('',*,*,#40446,.F.) ;
#54881=ORIENTED_EDGE('',*,*,#40447,.T.) ;
#54882=ORIENTED_EDGE('',*,*,#40448,.F.) ;
#54883=ORIENTED_EDGE('',*,*,#40449,.T.) ;
#54884=ORIENTED_EDGE('',*,*,#40450,.T.) ;
#54885=ORIENTED_EDGE('',*,*,#40451,.T.) ;
#54886=ORIENTED_EDGE('',*,*,#40452,.T.) ;
#54887=ORIENTED_EDGE('',*,*,#40453,.T.) ;
#54888=ORIENTED_EDGE('',*,*,#40454,.T.) ;
#54889=ORIENTED_EDGE('',*,*,#40455,.T.) ;
#54890=ORIENTED_EDGE('',*,*,#40456,.F.) ;
#54891=ORIENTED_EDGE('',*,*,#40457,.T.) ;
#54892=ORIENTED_EDGE('',*,*,#40458,.F.) ;
#54893=ORIENTED_EDGE('',*,*,#40459,.T.) ;
#54894=ORIENTED_EDGE('',*,*,#40460,.T.) ;
#54895=ORIENTED_EDGE('',*,*,#40461,.T.) ;
#54896=ORIENTED_EDGE('',*,*,#40462,.T.) ;
#54897=ORIENTED_EDGE('',*,*,#40463,.T.) ;
#54898=ORIENTED_EDGE('',*,*,#40464,.T.) ;
#54899=ORIENTED_EDGE('',*,*,#40465,.T.) ;
#54900=ORIENTED_EDGE('',*,*,#40466,.F.) ;
#54901=ORIENTED_EDGE('',*,*,#40467,.T.) ;
#54902=ORIENTED_EDGE('',*,*,#40468,.F.) ;
#54903=ORIENTED_EDGE('',*,*,#40469,.T.) ;
#54904=ORIENTED_EDGE('',*,*,#40470,.T.) ;
#54905=ORIENTED_EDGE('',*,*,#40471,.T.) ;
#54906=ORIENTED_EDGE('',*,*,#40472,.T.) ;
#54907=ORIENTED_EDGE('',*,*,#40473,.T.) ;
#54908=ORIENTED_EDGE('',*,*,#40474,.T.) ;
#54909=ORIENTED_EDGE('',*,*,#40475,.T.) ;
#54910=ORIENTED_EDGE('',*,*,#40476,.F.) ;
#54911=ORIENTED_EDGE('',*,*,#40477,.T.) ;
#54912=ORIENTED_EDGE('',*,*,#40478,.F.) ;
#54913=ORIENTED_EDGE('',*,*,#40479,.T.) ;
#54914=ORIENTED_EDGE('',*,*,#40480,.T.) ;
#54915=ORIENTED_EDGE('',*,*,#40481,.T.) ;
#54916=ORIENTED_EDGE('',*,*,#40482,.T.) ;
#54917=ORIENTED_EDGE('',*,*,#40483,.T.) ;
#54918=ORIENTED_EDGE('',*,*,#40484,.T.) ;
#54919=ORIENTED_EDGE('',*,*,#40485,.T.) ;
#54920=ORIENTED_EDGE('',*,*,#40486,.F.) ;
#54921=ORIENTED_EDGE('',*,*,#40487,.T.) ;
#54922=ORIENTED_EDGE('',*,*,#40488,.F.) ;
#54923=ORIENTED_EDGE('',*,*,#40489,.T.) ;
#54924=ORIENTED_EDGE('',*,*,#40490,.T.) ;
#54925=ORIENTED_EDGE('',*,*,#40491,.T.) ;
#54926=ORIENTED_EDGE('',*,*,#40492,.T.) ;
#54927=ORIENTED_EDGE('',*,*,#40493,.T.) ;
#54928=ORIENTED_EDGE('',*,*,#40494,.T.) ;
#54929=ORIENTED_EDGE('',*,*,#40495,.T.) ;
#54930=ORIENTED_EDGE('',*,*,#40496,.T.) ;
#54931=ORIENTED_EDGE('',*,*,#39272,.T.) ;
#54932=ORIENTED_EDGE('',*,*,#40497,.T.) ;
#54933=ORIENTED_EDGE('',*,*,#40498,.T.) ;
#54934=ORIENTED_EDGE('',*,*,#40499,.T.) ;
#54935=ORIENTED_EDGE('',*,*,#40500,.T.) ;
#54936=ORIENTED_EDGE('',*,*,#40501,.T.) ;
#54937=ORIENTED_EDGE('',*,*,#40502,.T.) ;
#54938=ORIENTED_EDGE('',*,*,#40503,.T.) ;
#54939=ORIENTED_EDGE('',*,*,#40504,.T.) ;
#54940=ORIENTED_EDGE('',*,*,#40505,.T.) ;
#54941=ORIENTED_EDGE('',*,*,#40506,.T.) ;
#54942=ORIENTED_EDGE('',*,*,#40507,.T.) ;
#54943=ORIENTED_EDGE('',*,*,#40508,.T.) ;
#54944=ORIENTED_EDGE('',*,*,#40509,.T.) ;
#54945=ORIENTED_EDGE('',*,*,#40510,.T.) ;
#54946=ORIENTED_EDGE('',*,*,#40511,.T.) ;
#54947=ORIENTED_EDGE('',*,*,#40512,.T.) ;
#54948=ORIENTED_EDGE('',*,*,#40513,.T.) ;
#54949=ORIENTED_EDGE('',*,*,#40514,.T.) ;
#54950=ORIENTED_EDGE('',*,*,#40515,.T.) ;
#54951=ORIENTED_EDGE('',*,*,#39219,.T.) ;
#54952=ORIENTED_EDGE('',*,*,#40516,.T.) ;
#54953=ORIENTED_EDGE('',*,*,#40517,.T.) ;
#54954=ORIENTED_EDGE('',*,*,#40518,.T.) ;
#54955=ORIENTED_EDGE('',*,*,#40519,.T.) ;
#54956=ORIENTED_EDGE('',*,*,#40520,.T.) ;
#54957=ORIENTED_EDGE('',*,*,#40521,.T.) ;
#54958=ORIENTED_EDGE('',*,*,#40522,.T.) ;
#54959=ORIENTED_EDGE('',*,*,#40523,.T.) ;
#54960=ORIENTED_EDGE('',*,*,#40524,.T.) ;
#54961=ORIENTED_EDGE('',*,*,#40525,.T.) ;
#54962=ORIENTED_EDGE('',*,*,#40526,.T.) ;
#54963=ORIENTED_EDGE('',*,*,#40527,.T.) ;
#54964=ORIENTED_EDGE('',*,*,#40528,.T.) ;
#54965=ORIENTED_EDGE('',*,*,#40529,.T.) ;
#54966=ORIENTED_EDGE('',*,*,#40530,.T.) ;
#54967=ORIENTED_EDGE('',*,*,#40531,.T.) ;
#54968=ORIENTED_EDGE('',*,*,#40532,.T.) ;
#54969=ORIENTED_EDGE('',*,*,#40533,.T.) ;
#54970=ORIENTED_EDGE('',*,*,#40534,.T.) ;
#54971=ORIENTED_EDGE('',*,*,#39202,.T.) ;
#54972=ORIENTED_EDGE('',*,*,#40535,.T.) ;
#54973=ORIENTED_EDGE('',*,*,#40536,.T.) ;
#54974=ORIENTED_EDGE('',*,*,#40537,.T.) ;
#54975=ORIENTED_EDGE('',*,*,#40538,.T.) ;
#54976=ORIENTED_EDGE('',*,*,#40539,.T.) ;
#54977=ORIENTED_EDGE('',*,*,#40540,.T.) ;
#54978=ORIENTED_EDGE('',*,*,#40541,.T.) ;
#54979=ORIENTED_EDGE('',*,*,#40542,.T.) ;
#54980=ORIENTED_EDGE('',*,*,#40543,.T.) ;
#54981=ORIENTED_EDGE('',*,*,#40544,.T.) ;
#54982=ORIENTED_EDGE('',*,*,#40545,.T.) ;
#54983=ORIENTED_EDGE('',*,*,#40546,.T.) ;
#54984=ORIENTED_EDGE('',*,*,#40547,.T.) ;
#54985=ORIENTED_EDGE('',*,*,#40548,.T.) ;
#54986=ORIENTED_EDGE('',*,*,#40549,.T.) ;
#54987=ORIENTED_EDGE('',*,*,#40550,.T.) ;
#54988=ORIENTED_EDGE('',*,*,#40551,.T.) ;
#54989=ORIENTED_EDGE('',*,*,#40552,.T.) ;
#54990=ORIENTED_EDGE('',*,*,#40553,.T.) ;
#54991=ORIENTED_EDGE('',*,*,#39185,.T.) ;
#54992=ORIENTED_EDGE('',*,*,#40554,.T.) ;
#54993=ORIENTED_EDGE('',*,*,#40555,.T.) ;
#54994=ORIENTED_EDGE('',*,*,#40556,.T.) ;
#54995=ORIENTED_EDGE('',*,*,#40557,.T.) ;
#54996=ORIENTED_EDGE('',*,*,#40558,.T.) ;
#54997=ORIENTED_EDGE('',*,*,#40559,.T.) ;
#54998=ORIENTED_EDGE('',*,*,#40560,.T.) ;
#54999=ORIENTED_EDGE('',*,*,#40561,.T.) ;
#55000=ORIENTED_EDGE('',*,*,#40562,.T.) ;
#55001=ORIENTED_EDGE('',*,*,#40563,.T.) ;
#55002=ORIENTED_EDGE('',*,*,#40564,.T.) ;
#55003=ORIENTED_EDGE('',*,*,#40565,.T.) ;
#55004=ORIENTED_EDGE('',*,*,#40566,.T.) ;
#55005=ORIENTED_EDGE('',*,*,#40567,.T.) ;
#55006=ORIENTED_EDGE('',*,*,#40568,.T.) ;
#55007=ORIENTED_EDGE('',*,*,#40569,.T.) ;
#55008=ORIENTED_EDGE('',*,*,#40570,.T.) ;
#55009=ORIENTED_EDGE('',*,*,#40571,.T.) ;
#55010=ORIENTED_EDGE('',*,*,#40572,.T.) ;
#55011=ORIENTED_EDGE('',*,*,#39168,.T.) ;
#55012=ORIENTED_EDGE('',*,*,#40573,.T.) ;
#55013=ORIENTED_EDGE('',*,*,#40574,.T.) ;
#55014=ORIENTED_EDGE('',*,*,#40575,.T.) ;
#55015=ORIENTED_EDGE('',*,*,#40576,.T.) ;
#55016=ORIENTED_EDGE('',*,*,#40577,.T.) ;
#55017=ORIENTED_EDGE('',*,*,#40578,.T.) ;
#55018=ORIENTED_EDGE('',*,*,#40579,.T.) ;
#55019=ORIENTED_EDGE('',*,*,#40580,.T.) ;
#55020=ORIENTED_EDGE('',*,*,#40581,.T.) ;
#55021=ORIENTED_EDGE('',*,*,#40582,.T.) ;
#55022=ORIENTED_EDGE('',*,*,#40583,.T.) ;
#55023=ORIENTED_EDGE('',*,*,#40584,.T.) ;
#55024=ORIENTED_EDGE('',*,*,#40585,.T.) ;
#55025=ORIENTED_EDGE('',*,*,#40586,.T.) ;
#55026=ORIENTED_EDGE('',*,*,#40587,.T.) ;
#55027=ORIENTED_EDGE('',*,*,#40588,.T.) ;
#55028=ORIENTED_EDGE('',*,*,#40589,.T.) ;
#55029=ORIENTED_EDGE('',*,*,#40590,.T.) ;
#55030=ORIENTED_EDGE('',*,*,#40591,.T.) ;
#55031=ORIENTED_EDGE('',*,*,#39151,.T.) ;
#55032=ORIENTED_EDGE('',*,*,#40592,.T.) ;
#55033=ORIENTED_EDGE('',*,*,#40593,.T.) ;
#55034=ORIENTED_EDGE('',*,*,#40594,.T.) ;
#55035=ORIENTED_EDGE('',*,*,#40595,.T.) ;
#55036=ORIENTED_EDGE('',*,*,#40596,.T.) ;
#55037=ORIENTED_EDGE('',*,*,#40597,.T.) ;
#55038=ORIENTED_EDGE('',*,*,#40598,.T.) ;
#55039=ORIENTED_EDGE('',*,*,#40599,.T.) ;
#55040=ORIENTED_EDGE('',*,*,#40600,.T.) ;
#55041=ORIENTED_EDGE('',*,*,#40601,.T.) ;
#55042=ORIENTED_EDGE('',*,*,#40602,.T.) ;
#55043=ORIENTED_EDGE('',*,*,#40603,.T.) ;
#55044=ORIENTED_EDGE('',*,*,#40604,.T.) ;
#55045=ORIENTED_EDGE('',*,*,#40605,.T.) ;
#55046=ORIENTED_EDGE('',*,*,#40606,.T.) ;
#55047=ORIENTED_EDGE('',*,*,#40607,.T.) ;
#55048=ORIENTED_EDGE('',*,*,#40608,.T.) ;
#55049=ORIENTED_EDGE('',*,*,#40609,.T.) ;
#55050=ORIENTED_EDGE('',*,*,#40610,.T.) ;
#55051=ORIENTED_EDGE('',*,*,#39134,.T.) ;
#55052=ORIENTED_EDGE('',*,*,#40611,.T.) ;
#55053=ORIENTED_EDGE('',*,*,#40612,.T.) ;
#55054=ORIENTED_EDGE('',*,*,#40613,.T.) ;
#55055=ORIENTED_EDGE('',*,*,#40614,.T.) ;
#55056=ORIENTED_EDGE('',*,*,#40615,.T.) ;
#55057=ORIENTED_EDGE('',*,*,#40616,.T.) ;
#55058=ORIENTED_EDGE('',*,*,#40617,.T.) ;
#55059=ORIENTED_EDGE('',*,*,#40618,.T.) ;
#55060=ORIENTED_EDGE('',*,*,#40619,.T.) ;
#55061=ORIENTED_EDGE('',*,*,#40620,.T.) ;
#55062=ORIENTED_EDGE('',*,*,#40621,.T.) ;
#55063=ORIENTED_EDGE('',*,*,#40622,.T.) ;
#55064=ORIENTED_EDGE('',*,*,#40623,.T.) ;
#55065=ORIENTED_EDGE('',*,*,#40624,.T.) ;
#55066=ORIENTED_EDGE('',*,*,#40625,.T.) ;
#55067=ORIENTED_EDGE('',*,*,#40626,.T.) ;
#55068=ORIENTED_EDGE('',*,*,#40627,.T.) ;
#55069=ORIENTED_EDGE('',*,*,#40628,.T.) ;
#55070=ORIENTED_EDGE('',*,*,#40629,.T.) ;
#55071=ORIENTED_EDGE('',*,*,#39117,.T.) ;
#55072=ORIENTED_EDGE('',*,*,#40630,.T.) ;
#55073=ORIENTED_EDGE('',*,*,#40631,.T.) ;
#55074=ORIENTED_EDGE('',*,*,#40632,.T.) ;
#55075=ORIENTED_EDGE('',*,*,#40633,.T.) ;
#55076=ORIENTED_EDGE('',*,*,#40634,.T.) ;
#55077=ORIENTED_EDGE('',*,*,#40635,.T.) ;
#55078=ORIENTED_EDGE('',*,*,#40636,.T.) ;
#55079=ORIENTED_EDGE('',*,*,#40637,.T.) ;
#55080=ORIENTED_EDGE('',*,*,#40638,.T.) ;
#55081=ORIENTED_EDGE('',*,*,#40639,.T.) ;
#55082=ORIENTED_EDGE('',*,*,#40640,.T.) ;
#55083=ORIENTED_EDGE('',*,*,#40641,.T.) ;
#55084=ORIENTED_EDGE('',*,*,#40642,.T.) ;
#55085=ORIENTED_EDGE('',*,*,#40643,.T.) ;
#55086=ORIENTED_EDGE('',*,*,#40644,.T.) ;
#55087=ORIENTED_EDGE('',*,*,#40645,.T.) ;
#55088=ORIENTED_EDGE('',*,*,#40646,.T.) ;
#55089=ORIENTED_EDGE('',*,*,#40647,.T.) ;
#55090=ORIENTED_EDGE('',*,*,#40648,.T.) ;
#55091=ORIENTED_EDGE('',*,*,#39100,.T.) ;
#55092=ORIENTED_EDGE('',*,*,#40649,.T.) ;
#55093=ORIENTED_EDGE('',*,*,#40650,.T.) ;
#55094=ORIENTED_EDGE('',*,*,#40651,.T.) ;
#55095=ORIENTED_EDGE('',*,*,#40652,.T.) ;
#55096=ORIENTED_EDGE('',*,*,#40653,.T.) ;
#55097=ORIENTED_EDGE('',*,*,#40654,.T.) ;
#55098=ORIENTED_EDGE('',*,*,#40655,.T.) ;
#55099=ORIENTED_EDGE('',*,*,#40656,.T.) ;
#55100=ORIENTED_EDGE('',*,*,#40657,.T.) ;
#55101=ORIENTED_EDGE('',*,*,#40658,.T.) ;
#55102=ORIENTED_EDGE('',*,*,#40659,.T.) ;
#55103=ORIENTED_EDGE('',*,*,#40660,.T.) ;
#55104=ORIENTED_EDGE('',*,*,#40661,.F.) ;
#55105=ORIENTED_EDGE('',*,*,#40662,.T.) ;
#55106=ORIENTED_EDGE('',*,*,#40663,.T.) ;
#55107=ORIENTED_EDGE('',*,*,#40664,.T.) ;
#55108=ORIENTED_EDGE('',*,*,#40663,.F.) ;
#55109=ORIENTED_EDGE('',*,*,#40665,.T.) ;
#55110=ORIENTED_EDGE('',*,*,#40666,.T.) ;
#55111=ORIENTED_EDGE('',*,*,#40667,.T.) ;
#55112=ORIENTED_EDGE('',*,*,#40666,.F.) ;
#55113=ORIENTED_EDGE('',*,*,#40668,.T.) ;
#55114=ORIENTED_EDGE('',*,*,#40669,.T.) ;
#55115=ORIENTED_EDGE('',*,*,#40670,.T.) ;
#55116=ORIENTED_EDGE('',*,*,#40669,.F.) ;
#55117=ORIENTED_EDGE('',*,*,#40671,.T.) ;
#55118=ORIENTED_EDGE('',*,*,#40672,.T.) ;
#55119=ORIENTED_EDGE('',*,*,#40673,.T.) ;
#55120=ORIENTED_EDGE('',*,*,#40672,.F.) ;
#55121=ORIENTED_EDGE('',*,*,#40674,.T.) ;
#55122=ORIENTED_EDGE('',*,*,#40675,.T.) ;
#55123=ORIENTED_EDGE('',*,*,#40676,.T.) ;
#55124=ORIENTED_EDGE('',*,*,#40675,.F.) ;
#55125=ORIENTED_EDGE('',*,*,#40677,.T.) ;
#55126=ORIENTED_EDGE('',*,*,#40678,.T.) ;
#55127=ORIENTED_EDGE('',*,*,#40679,.T.) ;
#55128=ORIENTED_EDGE('',*,*,#40678,.F.) ;
#55129=ORIENTED_EDGE('',*,*,#39095,.T.) ;
#55130=ORIENTED_EDGE('',*,*,#40680,.T.) ;
#55131=ORIENTED_EDGE('',*,*,#40681,.T.) ;
#55132=ORIENTED_EDGE('',*,*,#40680,.F.) ;
#55133=ORIENTED_EDGE('',*,*,#40682,.T.) ;
#55134=ORIENTED_EDGE('',*,*,#39312,.T.) ;
#55135=ORIENTED_EDGE('',*,*,#40683,.T.) ;
#55136=ORIENTED_EDGE('',*,*,#39311,.F.) ;
#55137=ORIENTED_EDGE('',*,*,#40684,.T.) ;
#55138=ORIENTED_EDGE('',*,*,#40685,.T.) ;
#55139=ORIENTED_EDGE('',*,*,#40686,.T.) ;
#55140=ORIENTED_EDGE('',*,*,#40685,.F.) ;
#55141=ORIENTED_EDGE('',*,*,#40687,.T.) ;
#55142=ORIENTED_EDGE('',*,*,#40688,.T.) ;
#55143=ORIENTED_EDGE('',*,*,#40689,.T.) ;
#55144=ORIENTED_EDGE('',*,*,#40688,.F.) ;
#55145=ORIENTED_EDGE('',*,*,#40690,.T.) ;
#55146=ORIENTED_EDGE('',*,*,#40691,.T.) ;
#55147=ORIENTED_EDGE('',*,*,#40692,.T.) ;
#55148=ORIENTED_EDGE('',*,*,#40691,.F.) ;
#55149=ORIENTED_EDGE('',*,*,#40693,.T.) ;
#55150=ORIENTED_EDGE('',*,*,#40694,.T.) ;
#55151=ORIENTED_EDGE('',*,*,#40695,.T.) ;
#55152=ORIENTED_EDGE('',*,*,#40694,.F.) ;
#55153=ORIENTED_EDGE('',*,*,#40696,.T.) ;
#55154=ORIENTED_EDGE('',*,*,#40697,.T.) ;
#55155=ORIENTED_EDGE('',*,*,#40698,.T.) ;
#55156=ORIENTED_EDGE('',*,*,#40697,.F.) ;
#55157=ORIENTED_EDGE('',*,*,#40699,.T.) ;
#55158=ORIENTED_EDGE('',*,*,#40700,.T.) ;
#55159=ORIENTED_EDGE('',*,*,#40701,.T.) ;
#55160=ORIENTED_EDGE('',*,*,#40700,.F.) ;
#55161=ORIENTED_EDGE('',*,*,#40702,.T.) ;
#55162=ORIENTED_EDGE('',*,*,#40703,.T.) ;
#55163=ORIENTED_EDGE('',*,*,#40704,.T.) ;
#55164=ORIENTED_EDGE('',*,*,#40703,.F.) ;
#55165=ORIENTED_EDGE('',*,*,#40705,.T.) ;
#55166=ORIENTED_EDGE('',*,*,#40706,.T.) ;
#55167=ORIENTED_EDGE('',*,*,#40707,.T.) ;
#55168=ORIENTED_EDGE('',*,*,#40706,.F.) ;
#55169=ORIENTED_EDGE('',*,*,#40708,.T.) ;
#55170=ORIENTED_EDGE('',*,*,#40709,.T.) ;
#55171=ORIENTED_EDGE('',*,*,#40710,.T.) ;
#55172=ORIENTED_EDGE('',*,*,#40709,.F.) ;
#55173=ORIENTED_EDGE('',*,*,#40711,.T.) ;
#55174=ORIENTED_EDGE('',*,*,#40712,.T.) ;
#55175=ORIENTED_EDGE('',*,*,#40713,.T.) ;
#55176=ORIENTED_EDGE('',*,*,#40712,.F.) ;
#55177=ORIENTED_EDGE('',*,*,#40714,.T.) ;
#55178=ORIENTED_EDGE('',*,*,#40715,.T.) ;
#55179=ORIENTED_EDGE('',*,*,#40716,.T.) ;
#55180=ORIENTED_EDGE('',*,*,#40715,.F.) ;
#55181=ORIENTED_EDGE('',*,*,#40717,.T.) ;
#55182=ORIENTED_EDGE('',*,*,#40718,.T.) ;
#55183=ORIENTED_EDGE('',*,*,#40719,.T.) ;
#55184=ORIENTED_EDGE('',*,*,#40718,.F.) ;
#55185=ORIENTED_EDGE('',*,*,#40720,.T.) ;
#55186=ORIENTED_EDGE('',*,*,#40721,.T.) ;
#55187=ORIENTED_EDGE('',*,*,#40722,.T.) ;
#55188=ORIENTED_EDGE('',*,*,#40721,.F.) ;
#55189=ORIENTED_EDGE('',*,*,#40723,.T.) ;
#55190=ORIENTED_EDGE('',*,*,#40724,.T.) ;
#55191=ORIENTED_EDGE('',*,*,#40725,.T.) ;
#55192=ORIENTED_EDGE('',*,*,#40724,.F.) ;
#55193=ORIENTED_EDGE('',*,*,#40726,.T.) ;
#55194=ORIENTED_EDGE('',*,*,#40727,.T.) ;
#55195=ORIENTED_EDGE('',*,*,#40728,.T.) ;
#55196=ORIENTED_EDGE('',*,*,#40727,.F.) ;
#55197=ORIENTED_EDGE('',*,*,#40729,.T.) ;
#55198=ORIENTED_EDGE('',*,*,#40730,.T.) ;
#55199=ORIENTED_EDGE('',*,*,#40731,.T.) ;
#55200=ORIENTED_EDGE('',*,*,#40730,.F.) ;
#55201=ORIENTED_EDGE('',*,*,#40732,.T.) ;
#55202=ORIENTED_EDGE('',*,*,#40733,.T.) ;
#55203=ORIENTED_EDGE('',*,*,#40734,.T.) ;
#55204=ORIENTED_EDGE('',*,*,#40733,.F.) ;
#55205=ORIENTED_EDGE('',*,*,#40735,.T.) ;
#55206=ORIENTED_EDGE('',*,*,#40736,.T.) ;
#55207=ORIENTED_EDGE('',*,*,#40737,.T.) ;
#55208=ORIENTED_EDGE('',*,*,#40736,.F.) ;
#55209=ORIENTED_EDGE('',*,*,#40738,.T.) ;
#55210=ORIENTED_EDGE('',*,*,#40661,.T.) ;
#55211=ORIENTED_EDGE('',*,*,#40739,.T.) ;
#55212=ORIENTED_EDGE('',*,*,#40740,.T.) ;
#55213=ORIENTED_EDGE('',*,*,#40741,.T.) ;
#55214=ORIENTED_EDGE('',*,*,#40742,.T.) ;
#55215=ORIENTED_EDGE('',*,*,#40743,.T.) ;
#55216=ORIENTED_EDGE('',*,*,#40744,.T.) ;
#55217=ORIENTED_EDGE('',*,*,#40745,.T.) ;
#55218=ORIENTED_EDGE('',*,*,#40746,.T.) ;
#55219=ORIENTED_EDGE('',*,*,#40747,.T.) ;
#55220=ORIENTED_EDGE('',*,*,#40748,.T.) ;
#55221=ORIENTED_EDGE('',*,*,#40749,.T.) ;
#55222=ORIENTED_EDGE('',*,*,#40750,.T.) ;
#55223=ORIENTED_EDGE('',*,*,#40751,.T.) ;
#55224=ORIENTED_EDGE('',*,*,#40752,.T.) ;
#55225=ORIENTED_EDGE('',*,*,#40753,.T.) ;
#55226=ORIENTED_EDGE('',*,*,#40754,.T.) ;
#55227=ORIENTED_EDGE('',*,*,#40755,.T.) ;
#55228=ORIENTED_EDGE('',*,*,#40756,.T.) ;
#55229=ORIENTED_EDGE('',*,*,#40757,.T.) ;
#55230=ORIENTED_EDGE('',*,*,#39092,.T.) ;
#55231=ORIENTED_EDGE('',*,*,#40758,.F.) ;
#55232=ORIENTED_EDGE('',*,*,#40759,.T.) ;
#55233=ORIENTED_EDGE('',*,*,#40760,.T.) ;
#55234=ORIENTED_EDGE('',*,*,#40761,.T.) ;
#55235=ORIENTED_EDGE('',*,*,#40760,.F.) ;
#55236=ORIENTED_EDGE('',*,*,#40762,.T.) ;
#55237=ORIENTED_EDGE('',*,*,#40763,.T.) ;
#55238=ORIENTED_EDGE('',*,*,#40764,.T.) ;
#55239=ORIENTED_EDGE('',*,*,#40763,.F.) ;
#55240=ORIENTED_EDGE('',*,*,#40765,.T.) ;
#55241=ORIENTED_EDGE('',*,*,#40766,.T.) ;
#55242=ORIENTED_EDGE('',*,*,#40767,.T.) ;
#55243=ORIENTED_EDGE('',*,*,#40766,.F.) ;
#55244=ORIENTED_EDGE('',*,*,#40768,.T.) ;
#55245=ORIENTED_EDGE('',*,*,#40769,.T.) ;
#55246=ORIENTED_EDGE('',*,*,#40770,.T.) ;
#55247=ORIENTED_EDGE('',*,*,#40769,.F.) ;
#55248=ORIENTED_EDGE('',*,*,#40771,.T.) ;
#55249=ORIENTED_EDGE('',*,*,#40772,.T.) ;
#55250=ORIENTED_EDGE('',*,*,#40773,.T.) ;
#55251=ORIENTED_EDGE('',*,*,#40772,.F.) ;
#55252=ORIENTED_EDGE('',*,*,#40774,.T.) ;
#55253=ORIENTED_EDGE('',*,*,#40775,.T.) ;
#55254=ORIENTED_EDGE('',*,*,#40776,.T.) ;
#55255=ORIENTED_EDGE('',*,*,#40775,.F.) ;
#55256=ORIENTED_EDGE('',*,*,#39112,.T.) ;
#55257=ORIENTED_EDGE('',*,*,#40777,.T.) ;
#55258=ORIENTED_EDGE('',*,*,#40778,.T.) ;
#55259=ORIENTED_EDGE('',*,*,#40777,.F.) ;
#55260=ORIENTED_EDGE('',*,*,#40779,.T.) ;
#55261=ORIENTED_EDGE('',*,*,#39309,.T.) ;
#55262=ORIENTED_EDGE('',*,*,#40780,.T.) ;
#55263=ORIENTED_EDGE('',*,*,#39308,.F.) ;
#55264=ORIENTED_EDGE('',*,*,#40781,.T.) ;
#55265=ORIENTED_EDGE('',*,*,#40782,.T.) ;
#55266=ORIENTED_EDGE('',*,*,#40783,.T.) ;
#55267=ORIENTED_EDGE('',*,*,#40782,.F.) ;
#55268=ORIENTED_EDGE('',*,*,#40784,.T.) ;
#55269=ORIENTED_EDGE('',*,*,#40785,.T.) ;
#55270=ORIENTED_EDGE('',*,*,#40786,.T.) ;
#55271=ORIENTED_EDGE('',*,*,#40785,.F.) ;
#55272=ORIENTED_EDGE('',*,*,#40787,.T.) ;
#55273=ORIENTED_EDGE('',*,*,#40788,.T.) ;
#55274=ORIENTED_EDGE('',*,*,#40789,.T.) ;
#55275=ORIENTED_EDGE('',*,*,#40788,.F.) ;
#55276=ORIENTED_EDGE('',*,*,#40790,.T.) ;
#55277=ORIENTED_EDGE('',*,*,#40791,.T.) ;
#55278=ORIENTED_EDGE('',*,*,#40792,.T.) ;
#55279=ORIENTED_EDGE('',*,*,#40791,.F.) ;
#55280=ORIENTED_EDGE('',*,*,#40793,.T.) ;
#55281=ORIENTED_EDGE('',*,*,#40794,.T.) ;
#55282=ORIENTED_EDGE('',*,*,#40795,.T.) ;
#55283=ORIENTED_EDGE('',*,*,#40794,.F.) ;
#55284=ORIENTED_EDGE('',*,*,#40796,.T.) ;
#55285=ORIENTED_EDGE('',*,*,#40797,.T.) ;
#55286=ORIENTED_EDGE('',*,*,#40798,.T.) ;
#55287=ORIENTED_EDGE('',*,*,#40797,.F.) ;
#55288=ORIENTED_EDGE('',*,*,#40799,.T.) ;
#55289=ORIENTED_EDGE('',*,*,#40800,.T.) ;
#55290=ORIENTED_EDGE('',*,*,#40801,.T.) ;
#55291=ORIENTED_EDGE('',*,*,#40800,.F.) ;
#55292=ORIENTED_EDGE('',*,*,#40802,.T.) ;
#55293=ORIENTED_EDGE('',*,*,#40803,.T.) ;
#55294=ORIENTED_EDGE('',*,*,#40804,.T.) ;
#55295=ORIENTED_EDGE('',*,*,#40803,.F.) ;
#55296=ORIENTED_EDGE('',*,*,#40805,.T.) ;
#55297=ORIENTED_EDGE('',*,*,#40806,.T.) ;
#55298=ORIENTED_EDGE('',*,*,#40807,.T.) ;
#55299=ORIENTED_EDGE('',*,*,#40806,.F.) ;
#55300=ORIENTED_EDGE('',*,*,#40808,.T.) ;
#55301=ORIENTED_EDGE('',*,*,#40809,.T.) ;
#55302=ORIENTED_EDGE('',*,*,#40810,.T.) ;
#55303=ORIENTED_EDGE('',*,*,#40809,.F.) ;
#55304=ORIENTED_EDGE('',*,*,#40811,.T.) ;
#55305=ORIENTED_EDGE('',*,*,#40812,.T.) ;
#55306=ORIENTED_EDGE('',*,*,#40813,.T.) ;
#55307=ORIENTED_EDGE('',*,*,#40812,.F.) ;
#55308=ORIENTED_EDGE('',*,*,#40814,.T.) ;
#55309=ORIENTED_EDGE('',*,*,#40815,.T.) ;
#55310=ORIENTED_EDGE('',*,*,#40816,.T.) ;
#55311=ORIENTED_EDGE('',*,*,#40815,.F.) ;
#55312=ORIENTED_EDGE('',*,*,#40817,.T.) ;
#55313=ORIENTED_EDGE('',*,*,#40818,.T.) ;
#55314=ORIENTED_EDGE('',*,*,#40819,.T.) ;
#55315=ORIENTED_EDGE('',*,*,#40818,.F.) ;
#55316=ORIENTED_EDGE('',*,*,#40820,.T.) ;
#55317=ORIENTED_EDGE('',*,*,#40821,.T.) ;
#55318=ORIENTED_EDGE('',*,*,#40822,.T.) ;
#55319=ORIENTED_EDGE('',*,*,#40821,.F.) ;
#55320=ORIENTED_EDGE('',*,*,#40823,.T.) ;
#55321=ORIENTED_EDGE('',*,*,#40824,.T.) ;
#55322=ORIENTED_EDGE('',*,*,#40825,.T.) ;
#55323=ORIENTED_EDGE('',*,*,#40824,.F.) ;
#55324=ORIENTED_EDGE('',*,*,#40826,.T.) ;
#55325=ORIENTED_EDGE('',*,*,#40827,.T.) ;
#55326=ORIENTED_EDGE('',*,*,#40828,.T.) ;
#55327=ORIENTED_EDGE('',*,*,#40827,.F.) ;
#55328=ORIENTED_EDGE('',*,*,#40829,.T.) ;
#55329=ORIENTED_EDGE('',*,*,#40830,.T.) ;
#55330=ORIENTED_EDGE('',*,*,#40831,.T.) ;
#55331=ORIENTED_EDGE('',*,*,#40830,.F.) ;
#55332=ORIENTED_EDGE('',*,*,#40832,.T.) ;
#55333=ORIENTED_EDGE('',*,*,#40833,.T.) ;
#55334=ORIENTED_EDGE('',*,*,#40834,.T.) ;
#55335=ORIENTED_EDGE('',*,*,#40833,.F.) ;
#55336=ORIENTED_EDGE('',*,*,#40835,.T.) ;
#55337=ORIENTED_EDGE('',*,*,#40758,.T.) ;
#55338=ORIENTED_EDGE('',*,*,#40836,.T.) ;
#55339=ORIENTED_EDGE('',*,*,#40837,.T.) ;
#55340=ORIENTED_EDGE('',*,*,#40838,.T.) ;
#55341=ORIENTED_EDGE('',*,*,#40839,.T.) ;
#55342=ORIENTED_EDGE('',*,*,#40840,.T.) ;
#55343=ORIENTED_EDGE('',*,*,#40841,.T.) ;
#55344=ORIENTED_EDGE('',*,*,#40842,.T.) ;
#55345=ORIENTED_EDGE('',*,*,#40843,.T.) ;
#55346=ORIENTED_EDGE('',*,*,#40844,.T.) ;
#55347=ORIENTED_EDGE('',*,*,#40845,.T.) ;
#55348=ORIENTED_EDGE('',*,*,#40846,.T.) ;
#55349=ORIENTED_EDGE('',*,*,#40847,.T.) ;
#55350=ORIENTED_EDGE('',*,*,#40848,.T.) ;
#55351=ORIENTED_EDGE('',*,*,#40849,.T.) ;
#55352=ORIENTED_EDGE('',*,*,#40850,.T.) ;
#55353=ORIENTED_EDGE('',*,*,#40851,.T.) ;
#55354=ORIENTED_EDGE('',*,*,#40852,.T.) ;
#55355=ORIENTED_EDGE('',*,*,#40853,.T.) ;
#55356=ORIENTED_EDGE('',*,*,#40854,.T.) ;
#55357=ORIENTED_EDGE('',*,*,#39109,.T.) ;
#55358=ORIENTED_EDGE('',*,*,#40855,.F.) ;
#55359=ORIENTED_EDGE('',*,*,#40856,.T.) ;
#55360=ORIENTED_EDGE('',*,*,#40857,.T.) ;
#55361=ORIENTED_EDGE('',*,*,#40858,.T.) ;
#55362=ORIENTED_EDGE('',*,*,#40857,.F.) ;
#55363=ORIENTED_EDGE('',*,*,#40859,.T.) ;
#55364=ORIENTED_EDGE('',*,*,#40860,.T.) ;
#55365=ORIENTED_EDGE('',*,*,#40861,.T.) ;
#55366=ORIENTED_EDGE('',*,*,#40860,.F.) ;
#55367=ORIENTED_EDGE('',*,*,#40862,.T.) ;
#55368=ORIENTED_EDGE('',*,*,#40863,.T.) ;
#55369=ORIENTED_EDGE('',*,*,#40864,.T.) ;
#55370=ORIENTED_EDGE('',*,*,#40863,.F.) ;
#55371=ORIENTED_EDGE('',*,*,#40865,.T.) ;
#55372=ORIENTED_EDGE('',*,*,#40866,.T.) ;
#55373=ORIENTED_EDGE('',*,*,#40867,.T.) ;
#55374=ORIENTED_EDGE('',*,*,#40866,.F.) ;
#55375=ORIENTED_EDGE('',*,*,#40868,.T.) ;
#55376=ORIENTED_EDGE('',*,*,#40869,.T.) ;
#55377=ORIENTED_EDGE('',*,*,#40870,.T.) ;
#55378=ORIENTED_EDGE('',*,*,#40869,.F.) ;
#55379=ORIENTED_EDGE('',*,*,#40871,.T.) ;
#55380=ORIENTED_EDGE('',*,*,#40872,.T.) ;
#55381=ORIENTED_EDGE('',*,*,#40873,.T.) ;
#55382=ORIENTED_EDGE('',*,*,#40872,.F.) ;
#55383=ORIENTED_EDGE('',*,*,#39129,.T.) ;
#55384=ORIENTED_EDGE('',*,*,#40874,.T.) ;
#55385=ORIENTED_EDGE('',*,*,#40875,.T.) ;
#55386=ORIENTED_EDGE('',*,*,#40874,.F.) ;
#55387=ORIENTED_EDGE('',*,*,#40876,.T.) ;
#55388=ORIENTED_EDGE('',*,*,#39306,.T.) ;
#55389=ORIENTED_EDGE('',*,*,#40877,.T.) ;
#55390=ORIENTED_EDGE('',*,*,#39305,.F.) ;
#55391=ORIENTED_EDGE('',*,*,#40878,.T.) ;
#55392=ORIENTED_EDGE('',*,*,#40879,.T.) ;
#55393=ORIENTED_EDGE('',*,*,#40880,.T.) ;
#55394=ORIENTED_EDGE('',*,*,#40879,.F.) ;
#55395=ORIENTED_EDGE('',*,*,#40881,.T.) ;
#55396=ORIENTED_EDGE('',*,*,#40882,.T.) ;
#55397=ORIENTED_EDGE('',*,*,#40883,.T.) ;
#55398=ORIENTED_EDGE('',*,*,#40882,.F.) ;
#55399=ORIENTED_EDGE('',*,*,#40884,.T.) ;
#55400=ORIENTED_EDGE('',*,*,#40885,.T.) ;
#55401=ORIENTED_EDGE('',*,*,#40886,.T.) ;
#55402=ORIENTED_EDGE('',*,*,#40885,.F.) ;
#55403=ORIENTED_EDGE('',*,*,#40887,.T.) ;
#55404=ORIENTED_EDGE('',*,*,#40888,.T.) ;
#55405=ORIENTED_EDGE('',*,*,#40889,.T.) ;
#55406=ORIENTED_EDGE('',*,*,#40888,.F.) ;
#55407=ORIENTED_EDGE('',*,*,#40890,.T.) ;
#55408=ORIENTED_EDGE('',*,*,#40891,.T.) ;
#55409=ORIENTED_EDGE('',*,*,#40892,.T.) ;
#55410=ORIENTED_EDGE('',*,*,#40891,.F.) ;
#55411=ORIENTED_EDGE('',*,*,#40893,.T.) ;
#55412=ORIENTED_EDGE('',*,*,#40894,.T.) ;
#55413=ORIENTED_EDGE('',*,*,#40895,.T.) ;
#55414=ORIENTED_EDGE('',*,*,#40894,.F.) ;
#55415=ORIENTED_EDGE('',*,*,#40896,.T.) ;
#55416=ORIENTED_EDGE('',*,*,#40897,.T.) ;
#55417=ORIENTED_EDGE('',*,*,#40898,.T.) ;
#55418=ORIENTED_EDGE('',*,*,#40897,.F.) ;
#55419=ORIENTED_EDGE('',*,*,#40899,.T.) ;
#55420=ORIENTED_EDGE('',*,*,#40900,.T.) ;
#55421=ORIENTED_EDGE('',*,*,#40901,.T.) ;
#55422=ORIENTED_EDGE('',*,*,#40900,.F.) ;
#55423=ORIENTED_EDGE('',*,*,#40902,.T.) ;
#55424=ORIENTED_EDGE('',*,*,#40903,.T.) ;
#55425=ORIENTED_EDGE('',*,*,#40904,.T.) ;
#55426=ORIENTED_EDGE('',*,*,#40903,.F.) ;
#55427=ORIENTED_EDGE('',*,*,#40905,.T.) ;
#55428=ORIENTED_EDGE('',*,*,#40906,.T.) ;
#55429=ORIENTED_EDGE('',*,*,#40907,.T.) ;
#55430=ORIENTED_EDGE('',*,*,#40906,.F.) ;
#55431=ORIENTED_EDGE('',*,*,#40908,.T.) ;
#55432=ORIENTED_EDGE('',*,*,#40909,.T.) ;
#55433=ORIENTED_EDGE('',*,*,#40910,.T.) ;
#55434=ORIENTED_EDGE('',*,*,#40909,.F.) ;
#55435=ORIENTED_EDGE('',*,*,#40911,.T.) ;
#55436=ORIENTED_EDGE('',*,*,#40912,.T.) ;
#55437=ORIENTED_EDGE('',*,*,#40913,.T.) ;
#55438=ORIENTED_EDGE('',*,*,#40912,.F.) ;
#55439=ORIENTED_EDGE('',*,*,#40914,.T.) ;
#55440=ORIENTED_EDGE('',*,*,#40915,.T.) ;
#55441=ORIENTED_EDGE('',*,*,#40916,.T.) ;
#55442=ORIENTED_EDGE('',*,*,#40915,.F.) ;
#55443=ORIENTED_EDGE('',*,*,#40917,.T.) ;
#55444=ORIENTED_EDGE('',*,*,#40918,.T.) ;
#55445=ORIENTED_EDGE('',*,*,#40919,.T.) ;
#55446=ORIENTED_EDGE('',*,*,#40918,.F.) ;
#55447=ORIENTED_EDGE('',*,*,#40920,.T.) ;
#55448=ORIENTED_EDGE('',*,*,#40921,.T.) ;
#55449=ORIENTED_EDGE('',*,*,#40922,.T.) ;
#55450=ORIENTED_EDGE('',*,*,#40921,.F.) ;
#55451=ORIENTED_EDGE('',*,*,#40923,.T.) ;
#55452=ORIENTED_EDGE('',*,*,#40924,.T.) ;
#55453=ORIENTED_EDGE('',*,*,#40925,.T.) ;
#55454=ORIENTED_EDGE('',*,*,#40924,.F.) ;
#55455=ORIENTED_EDGE('',*,*,#40926,.T.) ;
#55456=ORIENTED_EDGE('',*,*,#40927,.T.) ;
#55457=ORIENTED_EDGE('',*,*,#40928,.T.) ;
#55458=ORIENTED_EDGE('',*,*,#40927,.F.) ;
#55459=ORIENTED_EDGE('',*,*,#40929,.T.) ;
#55460=ORIENTED_EDGE('',*,*,#40930,.T.) ;
#55461=ORIENTED_EDGE('',*,*,#40931,.T.) ;
#55462=ORIENTED_EDGE('',*,*,#40930,.F.) ;
#55463=ORIENTED_EDGE('',*,*,#40932,.T.) ;
#55464=ORIENTED_EDGE('',*,*,#40855,.T.) ;
#55465=ORIENTED_EDGE('',*,*,#40933,.T.) ;
#55466=ORIENTED_EDGE('',*,*,#40934,.T.) ;
#55467=ORIENTED_EDGE('',*,*,#40935,.T.) ;
#55468=ORIENTED_EDGE('',*,*,#40936,.T.) ;
#55469=ORIENTED_EDGE('',*,*,#40937,.T.) ;
#55470=ORIENTED_EDGE('',*,*,#40938,.T.) ;
#55471=ORIENTED_EDGE('',*,*,#40939,.T.) ;
#55472=ORIENTED_EDGE('',*,*,#40940,.T.) ;
#55473=ORIENTED_EDGE('',*,*,#40941,.T.) ;
#55474=ORIENTED_EDGE('',*,*,#40942,.T.) ;
#55475=ORIENTED_EDGE('',*,*,#40943,.T.) ;
#55476=ORIENTED_EDGE('',*,*,#40944,.T.) ;
#55477=ORIENTED_EDGE('',*,*,#40945,.T.) ;
#55478=ORIENTED_EDGE('',*,*,#40946,.T.) ;
#55479=ORIENTED_EDGE('',*,*,#40947,.T.) ;
#55480=ORIENTED_EDGE('',*,*,#40948,.T.) ;
#55481=ORIENTED_EDGE('',*,*,#40949,.T.) ;
#55482=ORIENTED_EDGE('',*,*,#40950,.T.) ;
#55483=ORIENTED_EDGE('',*,*,#40951,.T.) ;
#55484=ORIENTED_EDGE('',*,*,#39126,.T.) ;
#55485=ORIENTED_EDGE('',*,*,#40952,.F.) ;
#55486=ORIENTED_EDGE('',*,*,#40953,.T.) ;
#55487=ORIENTED_EDGE('',*,*,#40954,.T.) ;
#55488=ORIENTED_EDGE('',*,*,#40955,.T.) ;
#55489=ORIENTED_EDGE('',*,*,#40954,.F.) ;
#55490=ORIENTED_EDGE('',*,*,#40956,.T.) ;
#55491=ORIENTED_EDGE('',*,*,#40957,.T.) ;
#55492=ORIENTED_EDGE('',*,*,#40958,.T.) ;
#55493=ORIENTED_EDGE('',*,*,#40957,.F.) ;
#55494=ORIENTED_EDGE('',*,*,#40959,.T.) ;
#55495=ORIENTED_EDGE('',*,*,#40960,.T.) ;
#55496=ORIENTED_EDGE('',*,*,#40961,.T.) ;
#55497=ORIENTED_EDGE('',*,*,#40960,.F.) ;
#55498=ORIENTED_EDGE('',*,*,#40962,.T.) ;
#55499=ORIENTED_EDGE('',*,*,#40963,.T.) ;
#55500=ORIENTED_EDGE('',*,*,#40964,.T.) ;
#55501=ORIENTED_EDGE('',*,*,#40963,.F.) ;
#55502=ORIENTED_EDGE('',*,*,#40965,.T.) ;
#55503=ORIENTED_EDGE('',*,*,#40966,.T.) ;
#55504=ORIENTED_EDGE('',*,*,#40967,.T.) ;
#55505=ORIENTED_EDGE('',*,*,#40966,.F.) ;
#55506=ORIENTED_EDGE('',*,*,#40968,.T.) ;
#55507=ORIENTED_EDGE('',*,*,#40969,.T.) ;
#55508=ORIENTED_EDGE('',*,*,#40970,.T.) ;
#55509=ORIENTED_EDGE('',*,*,#40969,.F.) ;
#55510=ORIENTED_EDGE('',*,*,#39146,.T.) ;
#55511=ORIENTED_EDGE('',*,*,#40971,.T.) ;
#55512=ORIENTED_EDGE('',*,*,#40972,.T.) ;
#55513=ORIENTED_EDGE('',*,*,#40971,.F.) ;
#55514=ORIENTED_EDGE('',*,*,#40973,.T.) ;
#55515=ORIENTED_EDGE('',*,*,#39303,.T.) ;
#55516=ORIENTED_EDGE('',*,*,#40974,.T.) ;
#55517=ORIENTED_EDGE('',*,*,#39302,.F.) ;
#55518=ORIENTED_EDGE('',*,*,#40975,.T.) ;
#55519=ORIENTED_EDGE('',*,*,#40976,.T.) ;
#55520=ORIENTED_EDGE('',*,*,#40977,.T.) ;
#55521=ORIENTED_EDGE('',*,*,#40976,.F.) ;
#55522=ORIENTED_EDGE('',*,*,#40978,.T.) ;
#55523=ORIENTED_EDGE('',*,*,#40979,.T.) ;
#55524=ORIENTED_EDGE('',*,*,#40980,.T.) ;
#55525=ORIENTED_EDGE('',*,*,#40979,.F.) ;
#55526=ORIENTED_EDGE('',*,*,#40981,.T.) ;
#55527=ORIENTED_EDGE('',*,*,#40982,.T.) ;
#55528=ORIENTED_EDGE('',*,*,#40983,.T.) ;
#55529=ORIENTED_EDGE('',*,*,#40982,.F.) ;
#55530=ORIENTED_EDGE('',*,*,#40984,.T.) ;
#55531=ORIENTED_EDGE('',*,*,#40985,.T.) ;
#55532=ORIENTED_EDGE('',*,*,#40986,.T.) ;
#55533=ORIENTED_EDGE('',*,*,#40985,.F.) ;
#55534=ORIENTED_EDGE('',*,*,#40987,.T.) ;
#55535=ORIENTED_EDGE('',*,*,#40988,.T.) ;
#55536=ORIENTED_EDGE('',*,*,#40989,.T.) ;
#55537=ORIENTED_EDGE('',*,*,#40988,.F.) ;
#55538=ORIENTED_EDGE('',*,*,#40990,.T.) ;
#55539=ORIENTED_EDGE('',*,*,#40991,.T.) ;
#55540=ORIENTED_EDGE('',*,*,#40992,.T.) ;
#55541=ORIENTED_EDGE('',*,*,#40991,.F.) ;
#55542=ORIENTED_EDGE('',*,*,#40993,.T.) ;
#55543=ORIENTED_EDGE('',*,*,#40994,.T.) ;
#55544=ORIENTED_EDGE('',*,*,#40995,.T.) ;
#55545=ORIENTED_EDGE('',*,*,#40994,.F.) ;
#55546=ORIENTED_EDGE('',*,*,#40996,.T.) ;
#55547=ORIENTED_EDGE('',*,*,#40997,.T.) ;
#55548=ORIENTED_EDGE('',*,*,#40998,.T.) ;
#55549=ORIENTED_EDGE('',*,*,#40997,.F.) ;
#55550=ORIENTED_EDGE('',*,*,#40999,.T.) ;
#55551=ORIENTED_EDGE('',*,*,#41000,.T.) ;
#55552=ORIENTED_EDGE('',*,*,#41001,.T.) ;
#55553=ORIENTED_EDGE('',*,*,#41000,.F.) ;
#55554=ORIENTED_EDGE('',*,*,#41002,.T.) ;
#55555=ORIENTED_EDGE('',*,*,#41003,.T.) ;
#55556=ORIENTED_EDGE('',*,*,#41004,.T.) ;
#55557=ORIENTED_EDGE('',*,*,#41003,.F.) ;
#55558=ORIENTED_EDGE('',*,*,#41005,.T.) ;
#55559=ORIENTED_EDGE('',*,*,#41006,.T.) ;
#55560=ORIENTED_EDGE('',*,*,#41007,.T.) ;
#55561=ORIENTED_EDGE('',*,*,#41006,.F.) ;
#55562=ORIENTED_EDGE('',*,*,#41008,.T.) ;
#55563=ORIENTED_EDGE('',*,*,#41009,.T.) ;
#55564=ORIENTED_EDGE('',*,*,#41010,.T.) ;
#55565=ORIENTED_EDGE('',*,*,#41009,.F.) ;
#55566=ORIENTED_EDGE('',*,*,#41011,.T.) ;
#55567=ORIENTED_EDGE('',*,*,#41012,.T.) ;
#55568=ORIENTED_EDGE('',*,*,#41013,.T.) ;
#55569=ORIENTED_EDGE('',*,*,#41012,.F.) ;
#55570=ORIENTED_EDGE('',*,*,#41014,.T.) ;
#55571=ORIENTED_EDGE('',*,*,#41015,.T.) ;
#55572=ORIENTED_EDGE('',*,*,#41016,.T.) ;
#55573=ORIENTED_EDGE('',*,*,#41015,.F.) ;
#55574=ORIENTED_EDGE('',*,*,#41017,.T.) ;
#55575=ORIENTED_EDGE('',*,*,#41018,.T.) ;
#55576=ORIENTED_EDGE('',*,*,#41019,.T.) ;
#55577=ORIENTED_EDGE('',*,*,#41018,.F.) ;
#55578=ORIENTED_EDGE('',*,*,#41020,.T.) ;
#55579=ORIENTED_EDGE('',*,*,#41021,.T.) ;
#55580=ORIENTED_EDGE('',*,*,#41022,.T.) ;
#55581=ORIENTED_EDGE('',*,*,#41021,.F.) ;
#55582=ORIENTED_EDGE('',*,*,#41023,.T.) ;
#55583=ORIENTED_EDGE('',*,*,#41024,.T.) ;
#55584=ORIENTED_EDGE('',*,*,#41025,.T.) ;
#55585=ORIENTED_EDGE('',*,*,#41024,.F.) ;
#55586=ORIENTED_EDGE('',*,*,#41026,.T.) ;
#55587=ORIENTED_EDGE('',*,*,#41027,.T.) ;
#55588=ORIENTED_EDGE('',*,*,#41028,.T.) ;
#55589=ORIENTED_EDGE('',*,*,#41027,.F.) ;
#55590=ORIENTED_EDGE('',*,*,#41029,.T.) ;
#55591=ORIENTED_EDGE('',*,*,#40952,.T.) ;
#55592=ORIENTED_EDGE('',*,*,#41030,.T.) ;
#55593=ORIENTED_EDGE('',*,*,#41031,.T.) ;
#55594=ORIENTED_EDGE('',*,*,#41032,.T.) ;
#55595=ORIENTED_EDGE('',*,*,#41033,.T.) ;
#55596=ORIENTED_EDGE('',*,*,#41034,.T.) ;
#55597=ORIENTED_EDGE('',*,*,#41035,.T.) ;
#55598=ORIENTED_EDGE('',*,*,#41036,.T.) ;
#55599=ORIENTED_EDGE('',*,*,#41037,.T.) ;
#55600=ORIENTED_EDGE('',*,*,#41038,.T.) ;
#55601=ORIENTED_EDGE('',*,*,#41039,.T.) ;
#55602=ORIENTED_EDGE('',*,*,#41040,.T.) ;
#55603=ORIENTED_EDGE('',*,*,#41041,.T.) ;
#55604=ORIENTED_EDGE('',*,*,#41042,.T.) ;
#55605=ORIENTED_EDGE('',*,*,#41043,.T.) ;
#55606=ORIENTED_EDGE('',*,*,#41044,.T.) ;
#55607=ORIENTED_EDGE('',*,*,#41045,.T.) ;
#55608=ORIENTED_EDGE('',*,*,#41046,.T.) ;
#55609=ORIENTED_EDGE('',*,*,#41047,.T.) ;
#55610=ORIENTED_EDGE('',*,*,#41048,.T.) ;
#55611=ORIENTED_EDGE('',*,*,#39143,.T.) ;
#55612=ORIENTED_EDGE('',*,*,#41049,.F.) ;
#55613=ORIENTED_EDGE('',*,*,#41050,.T.) ;
#55614=ORIENTED_EDGE('',*,*,#41051,.T.) ;
#55615=ORIENTED_EDGE('',*,*,#41052,.T.) ;
#55616=ORIENTED_EDGE('',*,*,#41051,.F.) ;
#55617=ORIENTED_EDGE('',*,*,#41053,.T.) ;
#55618=ORIENTED_EDGE('',*,*,#41054,.T.) ;
#55619=ORIENTED_EDGE('',*,*,#41055,.T.) ;
#55620=ORIENTED_EDGE('',*,*,#41054,.F.) ;
#55621=ORIENTED_EDGE('',*,*,#41056,.T.) ;
#55622=ORIENTED_EDGE('',*,*,#41057,.T.) ;
#55623=ORIENTED_EDGE('',*,*,#41058,.T.) ;
#55624=ORIENTED_EDGE('',*,*,#41057,.F.) ;
#55625=ORIENTED_EDGE('',*,*,#41059,.T.) ;
#55626=ORIENTED_EDGE('',*,*,#41060,.T.) ;
#55627=ORIENTED_EDGE('',*,*,#41061,.T.) ;
#55628=ORIENTED_EDGE('',*,*,#41060,.F.) ;
#55629=ORIENTED_EDGE('',*,*,#41062,.T.) ;
#55630=ORIENTED_EDGE('',*,*,#41063,.T.) ;
#55631=ORIENTED_EDGE('',*,*,#41064,.T.) ;
#55632=ORIENTED_EDGE('',*,*,#41063,.F.) ;
#55633=ORIENTED_EDGE('',*,*,#41065,.T.) ;
#55634=ORIENTED_EDGE('',*,*,#41066,.T.) ;
#55635=ORIENTED_EDGE('',*,*,#41067,.T.) ;
#55636=ORIENTED_EDGE('',*,*,#41066,.F.) ;
#55637=ORIENTED_EDGE('',*,*,#39163,.T.) ;
#55638=ORIENTED_EDGE('',*,*,#41068,.T.) ;
#55639=ORIENTED_EDGE('',*,*,#41069,.T.) ;
#55640=ORIENTED_EDGE('',*,*,#41068,.F.) ;
#55641=ORIENTED_EDGE('',*,*,#41070,.T.) ;
#55642=ORIENTED_EDGE('',*,*,#39300,.T.) ;
#55643=ORIENTED_EDGE('',*,*,#41071,.T.) ;
#55644=ORIENTED_EDGE('',*,*,#39299,.F.) ;
#55645=ORIENTED_EDGE('',*,*,#41072,.T.) ;
#55646=ORIENTED_EDGE('',*,*,#41073,.T.) ;
#55647=ORIENTED_EDGE('',*,*,#41074,.T.) ;
#55648=ORIENTED_EDGE('',*,*,#41073,.F.) ;
#55649=ORIENTED_EDGE('',*,*,#41075,.T.) ;
#55650=ORIENTED_EDGE('',*,*,#41076,.T.) ;
#55651=ORIENTED_EDGE('',*,*,#41077,.T.) ;
#55652=ORIENTED_EDGE('',*,*,#41076,.F.) ;
#55653=ORIENTED_EDGE('',*,*,#41078,.T.) ;
#55654=ORIENTED_EDGE('',*,*,#41079,.T.) ;
#55655=ORIENTED_EDGE('',*,*,#41080,.T.) ;
#55656=ORIENTED_EDGE('',*,*,#41079,.F.) ;
#55657=ORIENTED_EDGE('',*,*,#41081,.T.) ;
#55658=ORIENTED_EDGE('',*,*,#41082,.T.) ;
#55659=ORIENTED_EDGE('',*,*,#41083,.T.) ;
#55660=ORIENTED_EDGE('',*,*,#41082,.F.) ;
#55661=ORIENTED_EDGE('',*,*,#41084,.T.) ;
#55662=ORIENTED_EDGE('',*,*,#41085,.T.) ;
#55663=ORIENTED_EDGE('',*,*,#41086,.T.) ;
#55664=ORIENTED_EDGE('',*,*,#41085,.F.) ;
#55665=ORIENTED_EDGE('',*,*,#41087,.T.) ;
#55666=ORIENTED_EDGE('',*,*,#41088,.T.) ;
#55667=ORIENTED_EDGE('',*,*,#41089,.T.) ;
#55668=ORIENTED_EDGE('',*,*,#41088,.F.) ;
#55669=ORIENTED_EDGE('',*,*,#41090,.T.) ;
#55670=ORIENTED_EDGE('',*,*,#41091,.T.) ;
#55671=ORIENTED_EDGE('',*,*,#41092,.T.) ;
#55672=ORIENTED_EDGE('',*,*,#41091,.F.) ;
#55673=ORIENTED_EDGE('',*,*,#41093,.T.) ;
#55674=ORIENTED_EDGE('',*,*,#41094,.T.) ;
#55675=ORIENTED_EDGE('',*,*,#41095,.T.) ;
#55676=ORIENTED_EDGE('',*,*,#41094,.F.) ;
#55677=ORIENTED_EDGE('',*,*,#41096,.T.) ;
#55678=ORIENTED_EDGE('',*,*,#41097,.T.) ;
#55679=ORIENTED_EDGE('',*,*,#41098,.T.) ;
#55680=ORIENTED_EDGE('',*,*,#41097,.F.) ;
#55681=ORIENTED_EDGE('',*,*,#41099,.T.) ;
#55682=ORIENTED_EDGE('',*,*,#41100,.T.) ;
#55683=ORIENTED_EDGE('',*,*,#41101,.T.) ;
#55684=ORIENTED_EDGE('',*,*,#41100,.F.) ;
#55685=ORIENTED_EDGE('',*,*,#41102,.T.) ;
#55686=ORIENTED_EDGE('',*,*,#41103,.T.) ;
#55687=ORIENTED_EDGE('',*,*,#41104,.T.) ;
#55688=ORIENTED_EDGE('',*,*,#41103,.F.) ;
#55689=ORIENTED_EDGE('',*,*,#41105,.T.) ;
#55690=ORIENTED_EDGE('',*,*,#41106,.T.) ;
#55691=ORIENTED_EDGE('',*,*,#41107,.T.) ;
#55692=ORIENTED_EDGE('',*,*,#41106,.F.) ;
#55693=ORIENTED_EDGE('',*,*,#41108,.T.) ;
#55694=ORIENTED_EDGE('',*,*,#41109,.T.) ;
#55695=ORIENTED_EDGE('',*,*,#41110,.T.) ;
#55696=ORIENTED_EDGE('',*,*,#41109,.F.) ;
#55697=ORIENTED_EDGE('',*,*,#41111,.T.) ;
#55698=ORIENTED_EDGE('',*,*,#41112,.T.) ;
#55699=ORIENTED_EDGE('',*,*,#41113,.T.) ;
#55700=ORIENTED_EDGE('',*,*,#41112,.F.) ;
#55701=ORIENTED_EDGE('',*,*,#41114,.T.) ;
#55702=ORIENTED_EDGE('',*,*,#41115,.T.) ;
#55703=ORIENTED_EDGE('',*,*,#41116,.T.) ;
#55704=ORIENTED_EDGE('',*,*,#41115,.F.) ;
#55705=ORIENTED_EDGE('',*,*,#41117,.T.) ;
#55706=ORIENTED_EDGE('',*,*,#41118,.T.) ;
#55707=ORIENTED_EDGE('',*,*,#41119,.T.) ;
#55708=ORIENTED_EDGE('',*,*,#41118,.F.) ;
#55709=ORIENTED_EDGE('',*,*,#41120,.T.) ;
#55710=ORIENTED_EDGE('',*,*,#41121,.T.) ;
#55711=ORIENTED_EDGE('',*,*,#41122,.T.) ;
#55712=ORIENTED_EDGE('',*,*,#41121,.F.) ;
#55713=ORIENTED_EDGE('',*,*,#41123,.T.) ;
#55714=ORIENTED_EDGE('',*,*,#41124,.T.) ;
#55715=ORIENTED_EDGE('',*,*,#41125,.T.) ;
#55716=ORIENTED_EDGE('',*,*,#41124,.F.) ;
#55717=ORIENTED_EDGE('',*,*,#41126,.T.) ;
#55718=ORIENTED_EDGE('',*,*,#41049,.T.) ;
#55719=ORIENTED_EDGE('',*,*,#41127,.T.) ;
#55720=ORIENTED_EDGE('',*,*,#41128,.T.) ;
#55721=ORIENTED_EDGE('',*,*,#41129,.T.) ;
#55722=ORIENTED_EDGE('',*,*,#41130,.T.) ;
#55723=ORIENTED_EDGE('',*,*,#41131,.T.) ;
#55724=ORIENTED_EDGE('',*,*,#41132,.T.) ;
#55725=ORIENTED_EDGE('',*,*,#41133,.T.) ;
#55726=ORIENTED_EDGE('',*,*,#41134,.T.) ;
#55727=ORIENTED_EDGE('',*,*,#41135,.T.) ;
#55728=ORIENTED_EDGE('',*,*,#41136,.T.) ;
#55729=ORIENTED_EDGE('',*,*,#41137,.T.) ;
#55730=ORIENTED_EDGE('',*,*,#41138,.T.) ;
#55731=ORIENTED_EDGE('',*,*,#41139,.T.) ;
#55732=ORIENTED_EDGE('',*,*,#41140,.T.) ;
#55733=ORIENTED_EDGE('',*,*,#41141,.T.) ;
#55734=ORIENTED_EDGE('',*,*,#41142,.T.) ;
#55735=ORIENTED_EDGE('',*,*,#41143,.T.) ;
#55736=ORIENTED_EDGE('',*,*,#41144,.T.) ;
#55737=ORIENTED_EDGE('',*,*,#41145,.T.) ;
#55738=ORIENTED_EDGE('',*,*,#39160,.T.) ;
#55739=ORIENTED_EDGE('',*,*,#41146,.F.) ;
#55740=ORIENTED_EDGE('',*,*,#41147,.T.) ;
#55741=ORIENTED_EDGE('',*,*,#41148,.T.) ;
#55742=ORIENTED_EDGE('',*,*,#41149,.T.) ;
#55743=ORIENTED_EDGE('',*,*,#41148,.F.) ;
#55744=ORIENTED_EDGE('',*,*,#41150,.T.) ;
#55745=ORIENTED_EDGE('',*,*,#41151,.T.) ;
#55746=ORIENTED_EDGE('',*,*,#41152,.T.) ;
#55747=ORIENTED_EDGE('',*,*,#41151,.F.) ;
#55748=ORIENTED_EDGE('',*,*,#41153,.T.) ;
#55749=ORIENTED_EDGE('',*,*,#41154,.T.) ;
#55750=ORIENTED_EDGE('',*,*,#41155,.T.) ;
#55751=ORIENTED_EDGE('',*,*,#41154,.F.) ;
#55752=ORIENTED_EDGE('',*,*,#41156,.T.) ;
#55753=ORIENTED_EDGE('',*,*,#41157,.T.) ;
#55754=ORIENTED_EDGE('',*,*,#41158,.T.) ;
#55755=ORIENTED_EDGE('',*,*,#41157,.F.) ;
#55756=ORIENTED_EDGE('',*,*,#41159,.T.) ;
#55757=ORIENTED_EDGE('',*,*,#41160,.T.) ;
#55758=ORIENTED_EDGE('',*,*,#41161,.T.) ;
#55759=ORIENTED_EDGE('',*,*,#41160,.F.) ;
#55760=ORIENTED_EDGE('',*,*,#41162,.T.) ;
#55761=ORIENTED_EDGE('',*,*,#41163,.T.) ;
#55762=ORIENTED_EDGE('',*,*,#41164,.T.) ;
#55763=ORIENTED_EDGE('',*,*,#41163,.F.) ;
#55764=ORIENTED_EDGE('',*,*,#39180,.T.) ;
#55765=ORIENTED_EDGE('',*,*,#41165,.T.) ;
#55766=ORIENTED_EDGE('',*,*,#41166,.T.) ;
#55767=ORIENTED_EDGE('',*,*,#41165,.F.) ;
#55768=ORIENTED_EDGE('',*,*,#41167,.T.) ;
#55769=ORIENTED_EDGE('',*,*,#39297,.T.) ;
#55770=ORIENTED_EDGE('',*,*,#41168,.T.) ;
#55771=ORIENTED_EDGE('',*,*,#39296,.F.) ;
#55772=ORIENTED_EDGE('',*,*,#41169,.T.) ;
#55773=ORIENTED_EDGE('',*,*,#41170,.T.) ;
#55774=ORIENTED_EDGE('',*,*,#41171,.T.) ;
#55775=ORIENTED_EDGE('',*,*,#41170,.F.) ;
#55776=ORIENTED_EDGE('',*,*,#41172,.T.) ;
#55777=ORIENTED_EDGE('',*,*,#41173,.T.) ;
#55778=ORIENTED_EDGE('',*,*,#41174,.T.) ;
#55779=ORIENTED_EDGE('',*,*,#41173,.F.) ;
#55780=ORIENTED_EDGE('',*,*,#41175,.T.) ;
#55781=ORIENTED_EDGE('',*,*,#41176,.T.) ;
#55782=ORIENTED_EDGE('',*,*,#41177,.T.) ;
#55783=ORIENTED_EDGE('',*,*,#41176,.F.) ;
#55784=ORIENTED_EDGE('',*,*,#41178,.T.) ;
#55785=ORIENTED_EDGE('',*,*,#41179,.T.) ;
#55786=ORIENTED_EDGE('',*,*,#41180,.T.) ;
#55787=ORIENTED_EDGE('',*,*,#41179,.F.) ;
#55788=ORIENTED_EDGE('',*,*,#41181,.T.) ;
#55789=ORIENTED_EDGE('',*,*,#41182,.T.) ;
#55790=ORIENTED_EDGE('',*,*,#41183,.T.) ;
#55791=ORIENTED_EDGE('',*,*,#41182,.F.) ;
#55792=ORIENTED_EDGE('',*,*,#41184,.T.) ;
#55793=ORIENTED_EDGE('',*,*,#41185,.T.) ;
#55794=ORIENTED_EDGE('',*,*,#41186,.T.) ;
#55795=ORIENTED_EDGE('',*,*,#41185,.F.) ;
#55796=ORIENTED_EDGE('',*,*,#41187,.T.) ;
#55797=ORIENTED_EDGE('',*,*,#41188,.T.) ;
#55798=ORIENTED_EDGE('',*,*,#41189,.T.) ;
#55799=ORIENTED_EDGE('',*,*,#41188,.F.) ;
#55800=ORIENTED_EDGE('',*,*,#41190,.T.) ;
#55801=ORIENTED_EDGE('',*,*,#41191,.T.) ;
#55802=ORIENTED_EDGE('',*,*,#41192,.T.) ;
#55803=ORIENTED_EDGE('',*,*,#41191,.F.) ;
#55804=ORIENTED_EDGE('',*,*,#41193,.T.) ;
#55805=ORIENTED_EDGE('',*,*,#41194,.T.) ;
#55806=ORIENTED_EDGE('',*,*,#41195,.T.) ;
#55807=ORIENTED_EDGE('',*,*,#41194,.F.) ;
#55808=ORIENTED_EDGE('',*,*,#41196,.T.) ;
#55809=ORIENTED_EDGE('',*,*,#41197,.T.) ;
#55810=ORIENTED_EDGE('',*,*,#41198,.T.) ;
#55811=ORIENTED_EDGE('',*,*,#41197,.F.) ;
#55812=ORIENTED_EDGE('',*,*,#41199,.T.) ;
#55813=ORIENTED_EDGE('',*,*,#41200,.T.) ;
#55814=ORIENTED_EDGE('',*,*,#41201,.T.) ;
#55815=ORIENTED_EDGE('',*,*,#41200,.F.) ;
#55816=ORIENTED_EDGE('',*,*,#41202,.T.) ;
#55817=ORIENTED_EDGE('',*,*,#41203,.T.) ;
#55818=ORIENTED_EDGE('',*,*,#41204,.T.) ;
#55819=ORIENTED_EDGE('',*,*,#41203,.F.) ;
#55820=ORIENTED_EDGE('',*,*,#41205,.T.) ;
#55821=ORIENTED_EDGE('',*,*,#41206,.T.) ;
#55822=ORIENTED_EDGE('',*,*,#41207,.T.) ;
#55823=ORIENTED_EDGE('',*,*,#41206,.F.) ;
#55824=ORIENTED_EDGE('',*,*,#41208,.T.) ;
#55825=ORIENTED_EDGE('',*,*,#41209,.T.) ;
#55826=ORIENTED_EDGE('',*,*,#41210,.T.) ;
#55827=ORIENTED_EDGE('',*,*,#41209,.F.) ;
#55828=ORIENTED_EDGE('',*,*,#41211,.T.) ;
#55829=ORIENTED_EDGE('',*,*,#41212,.T.) ;
#55830=ORIENTED_EDGE('',*,*,#41213,.T.) ;
#55831=ORIENTED_EDGE('',*,*,#41212,.F.) ;
#55832=ORIENTED_EDGE('',*,*,#41214,.T.) ;
#55833=ORIENTED_EDGE('',*,*,#41215,.T.) ;
#55834=ORIENTED_EDGE('',*,*,#41216,.T.) ;
#55835=ORIENTED_EDGE('',*,*,#41215,.F.) ;
#55836=ORIENTED_EDGE('',*,*,#41217,.T.) ;
#55837=ORIENTED_EDGE('',*,*,#41218,.T.) ;
#55838=ORIENTED_EDGE('',*,*,#41219,.T.) ;
#55839=ORIENTED_EDGE('',*,*,#41218,.F.) ;
#55840=ORIENTED_EDGE('',*,*,#41220,.T.) ;
#55841=ORIENTED_EDGE('',*,*,#41221,.T.) ;
#55842=ORIENTED_EDGE('',*,*,#41222,.T.) ;
#55843=ORIENTED_EDGE('',*,*,#41221,.F.) ;
#55844=ORIENTED_EDGE('',*,*,#41223,.T.) ;
#55845=ORIENTED_EDGE('',*,*,#41146,.T.) ;
#55846=ORIENTED_EDGE('',*,*,#41224,.T.) ;
#55847=ORIENTED_EDGE('',*,*,#41225,.T.) ;
#55848=ORIENTED_EDGE('',*,*,#41226,.T.) ;
#55849=ORIENTED_EDGE('',*,*,#41227,.T.) ;
#55850=ORIENTED_EDGE('',*,*,#41228,.T.) ;
#55851=ORIENTED_EDGE('',*,*,#41229,.T.) ;
#55852=ORIENTED_EDGE('',*,*,#41230,.T.) ;
#55853=ORIENTED_EDGE('',*,*,#41231,.T.) ;
#55854=ORIENTED_EDGE('',*,*,#41232,.T.) ;
#55855=ORIENTED_EDGE('',*,*,#41233,.T.) ;
#55856=ORIENTED_EDGE('',*,*,#41234,.T.) ;
#55857=ORIENTED_EDGE('',*,*,#41235,.T.) ;
#55858=ORIENTED_EDGE('',*,*,#41236,.T.) ;
#55859=ORIENTED_EDGE('',*,*,#41237,.T.) ;
#55860=ORIENTED_EDGE('',*,*,#41238,.T.) ;
#55861=ORIENTED_EDGE('',*,*,#41239,.T.) ;
#55862=ORIENTED_EDGE('',*,*,#41240,.T.) ;
#55863=ORIENTED_EDGE('',*,*,#41241,.T.) ;
#55864=ORIENTED_EDGE('',*,*,#41242,.T.) ;
#55865=ORIENTED_EDGE('',*,*,#39177,.T.) ;
#55866=ORIENTED_EDGE('',*,*,#41243,.F.) ;
#55867=ORIENTED_EDGE('',*,*,#41244,.T.) ;
#55868=ORIENTED_EDGE('',*,*,#41245,.T.) ;
#55869=ORIENTED_EDGE('',*,*,#41246,.T.) ;
#55870=ORIENTED_EDGE('',*,*,#41245,.F.) ;
#55871=ORIENTED_EDGE('',*,*,#41247,.T.) ;
#55872=ORIENTED_EDGE('',*,*,#41248,.T.) ;
#55873=ORIENTED_EDGE('',*,*,#41249,.T.) ;
#55874=ORIENTED_EDGE('',*,*,#41248,.F.) ;
#55875=ORIENTED_EDGE('',*,*,#41250,.T.) ;
#55876=ORIENTED_EDGE('',*,*,#41251,.T.) ;
#55877=ORIENTED_EDGE('',*,*,#41252,.T.) ;
#55878=ORIENTED_EDGE('',*,*,#41251,.F.) ;
#55879=ORIENTED_EDGE('',*,*,#41253,.T.) ;
#55880=ORIENTED_EDGE('',*,*,#41254,.T.) ;
#55881=ORIENTED_EDGE('',*,*,#41255,.T.) ;
#55882=ORIENTED_EDGE('',*,*,#41254,.F.) ;
#55883=ORIENTED_EDGE('',*,*,#41256,.T.) ;
#55884=ORIENTED_EDGE('',*,*,#41257,.T.) ;
#55885=ORIENTED_EDGE('',*,*,#41258,.T.) ;
#55886=ORIENTED_EDGE('',*,*,#41257,.F.) ;
#55887=ORIENTED_EDGE('',*,*,#41259,.T.) ;
#55888=ORIENTED_EDGE('',*,*,#41260,.T.) ;
#55889=ORIENTED_EDGE('',*,*,#41261,.T.) ;
#55890=ORIENTED_EDGE('',*,*,#41260,.F.) ;
#55891=ORIENTED_EDGE('',*,*,#39197,.T.) ;
#55892=ORIENTED_EDGE('',*,*,#41262,.T.) ;
#55893=ORIENTED_EDGE('',*,*,#41263,.T.) ;
#55894=ORIENTED_EDGE('',*,*,#41262,.F.) ;
#55895=ORIENTED_EDGE('',*,*,#41264,.T.) ;
#55896=ORIENTED_EDGE('',*,*,#39294,.T.) ;
#55897=ORIENTED_EDGE('',*,*,#41265,.T.) ;
#55898=ORIENTED_EDGE('',*,*,#39293,.F.) ;
#55899=ORIENTED_EDGE('',*,*,#41266,.T.) ;
#55900=ORIENTED_EDGE('',*,*,#41267,.T.) ;
#55901=ORIENTED_EDGE('',*,*,#41268,.T.) ;
#55902=ORIENTED_EDGE('',*,*,#41267,.F.) ;
#55903=ORIENTED_EDGE('',*,*,#41269,.T.) ;
#55904=ORIENTED_EDGE('',*,*,#41270,.T.) ;
#55905=ORIENTED_EDGE('',*,*,#41271,.T.) ;
#55906=ORIENTED_EDGE('',*,*,#41270,.F.) ;
#55907=ORIENTED_EDGE('',*,*,#41272,.T.) ;
#55908=ORIENTED_EDGE('',*,*,#41273,.T.) ;
#55909=ORIENTED_EDGE('',*,*,#41274,.T.) ;
#55910=ORIENTED_EDGE('',*,*,#41273,.F.) ;
#55911=ORIENTED_EDGE('',*,*,#41275,.T.) ;
#55912=ORIENTED_EDGE('',*,*,#41276,.T.) ;
#55913=ORIENTED_EDGE('',*,*,#41277,.T.) ;
#55914=ORIENTED_EDGE('',*,*,#41276,.F.) ;
#55915=ORIENTED_EDGE('',*,*,#41278,.T.) ;
#55916=ORIENTED_EDGE('',*,*,#41279,.T.) ;
#55917=ORIENTED_EDGE('',*,*,#41280,.T.) ;
#55918=ORIENTED_EDGE('',*,*,#41279,.F.) ;
#55919=ORIENTED_EDGE('',*,*,#41281,.T.) ;
#55920=ORIENTED_EDGE('',*,*,#41282,.T.) ;
#55921=ORIENTED_EDGE('',*,*,#41283,.T.) ;
#55922=ORIENTED_EDGE('',*,*,#41282,.F.) ;
#55923=ORIENTED_EDGE('',*,*,#41284,.T.) ;
#55924=ORIENTED_EDGE('',*,*,#41285,.T.) ;
#55925=ORIENTED_EDGE('',*,*,#41286,.T.) ;
#55926=ORIENTED_EDGE('',*,*,#41285,.F.) ;
#55927=ORIENTED_EDGE('',*,*,#41287,.T.) ;
#55928=ORIENTED_EDGE('',*,*,#41288,.T.) ;
#55929=ORIENTED_EDGE('',*,*,#41289,.T.) ;
#55930=ORIENTED_EDGE('',*,*,#41288,.F.) ;
#55931=ORIENTED_EDGE('',*,*,#41290,.T.) ;
#55932=ORIENTED_EDGE('',*,*,#41291,.T.) ;
#55933=ORIENTED_EDGE('',*,*,#41292,.T.) ;
#55934=ORIENTED_EDGE('',*,*,#41291,.F.) ;
#55935=ORIENTED_EDGE('',*,*,#41293,.T.) ;
#55936=ORIENTED_EDGE('',*,*,#41294,.T.) ;
#55937=ORIENTED_EDGE('',*,*,#41295,.T.) ;
#55938=ORIENTED_EDGE('',*,*,#41294,.F.) ;
#55939=ORIENTED_EDGE('',*,*,#41296,.T.) ;
#55940=ORIENTED_EDGE('',*,*,#41297,.T.) ;
#55941=ORIENTED_EDGE('',*,*,#41298,.T.) ;
#55942=ORIENTED_EDGE('',*,*,#41297,.F.) ;
#55943=ORIENTED_EDGE('',*,*,#41299,.T.) ;
#55944=ORIENTED_EDGE('',*,*,#41300,.T.) ;
#55945=ORIENTED_EDGE('',*,*,#41301,.T.) ;
#55946=ORIENTED_EDGE('',*,*,#41300,.F.) ;
#55947=ORIENTED_EDGE('',*,*,#41302,.T.) ;
#55948=ORIENTED_EDGE('',*,*,#41303,.T.) ;
#55949=ORIENTED_EDGE('',*,*,#41304,.T.) ;
#55950=ORIENTED_EDGE('',*,*,#41303,.F.) ;
#55951=ORIENTED_EDGE('',*,*,#41305,.T.) ;
#55952=ORIENTED_EDGE('',*,*,#41306,.T.) ;
#55953=ORIENTED_EDGE('',*,*,#41307,.T.) ;
#55954=ORIENTED_EDGE('',*,*,#41306,.F.) ;
#55955=ORIENTED_EDGE('',*,*,#41308,.T.) ;
#55956=ORIENTED_EDGE('',*,*,#41309,.T.) ;
#55957=ORIENTED_EDGE('',*,*,#41310,.T.) ;
#55958=ORIENTED_EDGE('',*,*,#41309,.F.) ;
#55959=ORIENTED_EDGE('',*,*,#41311,.T.) ;
#55960=ORIENTED_EDGE('',*,*,#41312,.T.) ;
#55961=ORIENTED_EDGE('',*,*,#41313,.T.) ;
#55962=ORIENTED_EDGE('',*,*,#41312,.F.) ;
#55963=ORIENTED_EDGE('',*,*,#41314,.T.) ;
#55964=ORIENTED_EDGE('',*,*,#41315,.T.) ;
#55965=ORIENTED_EDGE('',*,*,#41316,.T.) ;
#55966=ORIENTED_EDGE('',*,*,#41315,.F.) ;
#55967=ORIENTED_EDGE('',*,*,#41317,.T.) ;
#55968=ORIENTED_EDGE('',*,*,#41318,.T.) ;
#55969=ORIENTED_EDGE('',*,*,#41319,.T.) ;
#55970=ORIENTED_EDGE('',*,*,#41318,.F.) ;
#55971=ORIENTED_EDGE('',*,*,#41320,.T.) ;
#55972=ORIENTED_EDGE('',*,*,#41243,.T.) ;
#55973=ORIENTED_EDGE('',*,*,#41321,.T.) ;
#55974=ORIENTED_EDGE('',*,*,#41322,.T.) ;
#55975=ORIENTED_EDGE('',*,*,#41323,.T.) ;
#55976=ORIENTED_EDGE('',*,*,#41324,.T.) ;
#55977=ORIENTED_EDGE('',*,*,#41325,.T.) ;
#55978=ORIENTED_EDGE('',*,*,#41326,.T.) ;
#55979=ORIENTED_EDGE('',*,*,#41327,.T.) ;
#55980=ORIENTED_EDGE('',*,*,#41328,.T.) ;
#55981=ORIENTED_EDGE('',*,*,#41329,.T.) ;
#55982=ORIENTED_EDGE('',*,*,#41330,.T.) ;
#55983=ORIENTED_EDGE('',*,*,#41331,.T.) ;
#55984=ORIENTED_EDGE('',*,*,#41332,.T.) ;
#55985=ORIENTED_EDGE('',*,*,#41333,.T.) ;
#55986=ORIENTED_EDGE('',*,*,#41334,.T.) ;
#55987=ORIENTED_EDGE('',*,*,#41335,.T.) ;
#55988=ORIENTED_EDGE('',*,*,#41336,.T.) ;
#55989=ORIENTED_EDGE('',*,*,#41337,.T.) ;
#55990=ORIENTED_EDGE('',*,*,#41338,.T.) ;
#55991=ORIENTED_EDGE('',*,*,#41339,.T.) ;
#55992=ORIENTED_EDGE('',*,*,#39194,.T.) ;
#55993=ORIENTED_EDGE('',*,*,#41340,.F.) ;
#55994=ORIENTED_EDGE('',*,*,#41341,.T.) ;
#55995=ORIENTED_EDGE('',*,*,#41342,.T.) ;
#55996=ORIENTED_EDGE('',*,*,#41343,.T.) ;
#55997=ORIENTED_EDGE('',*,*,#41342,.F.) ;
#55998=ORIENTED_EDGE('',*,*,#41344,.T.) ;
#55999=ORIENTED_EDGE('',*,*,#41345,.T.) ;
#56000=ORIENTED_EDGE('',*,*,#41346,.T.) ;
#56001=ORIENTED_EDGE('',*,*,#41345,.F.) ;
#56002=ORIENTED_EDGE('',*,*,#41347,.T.) ;
#56003=ORIENTED_EDGE('',*,*,#41348,.T.) ;
#56004=ORIENTED_EDGE('',*,*,#41349,.T.) ;
#56005=ORIENTED_EDGE('',*,*,#41348,.F.) ;
#56006=ORIENTED_EDGE('',*,*,#41350,.T.) ;
#56007=ORIENTED_EDGE('',*,*,#41351,.T.) ;
#56008=ORIENTED_EDGE('',*,*,#41352,.T.) ;
#56009=ORIENTED_EDGE('',*,*,#41351,.F.) ;
#56010=ORIENTED_EDGE('',*,*,#41353,.T.) ;
#56011=ORIENTED_EDGE('',*,*,#41354,.T.) ;
#56012=ORIENTED_EDGE('',*,*,#41355,.T.) ;
#56013=ORIENTED_EDGE('',*,*,#41354,.F.) ;
#56014=ORIENTED_EDGE('',*,*,#41356,.T.) ;
#56015=ORIENTED_EDGE('',*,*,#41357,.T.) ;
#56016=ORIENTED_EDGE('',*,*,#41358,.T.) ;
#56017=ORIENTED_EDGE('',*,*,#41357,.F.) ;
#56018=ORIENTED_EDGE('',*,*,#39214,.T.) ;
#56019=ORIENTED_EDGE('',*,*,#41359,.T.) ;
#56020=ORIENTED_EDGE('',*,*,#41360,.T.) ;
#56021=ORIENTED_EDGE('',*,*,#41359,.F.) ;
#56022=ORIENTED_EDGE('',*,*,#41361,.T.) ;
#56023=ORIENTED_EDGE('',*,*,#39291,.T.) ;
#56024=ORIENTED_EDGE('',*,*,#41362,.T.) ;
#56025=ORIENTED_EDGE('',*,*,#39290,.F.) ;
#56026=ORIENTED_EDGE('',*,*,#41363,.T.) ;
#56027=ORIENTED_EDGE('',*,*,#41364,.T.) ;
#56028=ORIENTED_EDGE('',*,*,#41365,.T.) ;
#56029=ORIENTED_EDGE('',*,*,#41364,.F.) ;
#56030=ORIENTED_EDGE('',*,*,#41366,.T.) ;
#56031=ORIENTED_EDGE('',*,*,#41367,.T.) ;
#56032=ORIENTED_EDGE('',*,*,#41368,.T.) ;
#56033=ORIENTED_EDGE('',*,*,#41367,.F.) ;
#56034=ORIENTED_EDGE('',*,*,#41369,.T.) ;
#56035=ORIENTED_EDGE('',*,*,#41370,.T.) ;
#56036=ORIENTED_EDGE('',*,*,#41371,.T.) ;
#56037=ORIENTED_EDGE('',*,*,#41370,.F.) ;
#56038=ORIENTED_EDGE('',*,*,#41372,.T.) ;
#56039=ORIENTED_EDGE('',*,*,#41373,.T.) ;
#56040=ORIENTED_EDGE('',*,*,#41374,.T.) ;
#56041=ORIENTED_EDGE('',*,*,#41373,.F.) ;
#56042=ORIENTED_EDGE('',*,*,#41375,.T.) ;
#56043=ORIENTED_EDGE('',*,*,#41376,.T.) ;
#56044=ORIENTED_EDGE('',*,*,#41377,.T.) ;
#56045=ORIENTED_EDGE('',*,*,#41376,.F.) ;
#56046=ORIENTED_EDGE('',*,*,#41378,.T.) ;
#56047=ORIENTED_EDGE('',*,*,#41379,.T.) ;
#56048=ORIENTED_EDGE('',*,*,#41380,.T.) ;
#56049=ORIENTED_EDGE('',*,*,#41379,.F.) ;
#56050=ORIENTED_EDGE('',*,*,#41381,.T.) ;
#56051=ORIENTED_EDGE('',*,*,#41382,.T.) ;
#56052=ORIENTED_EDGE('',*,*,#41383,.T.) ;
#56053=ORIENTED_EDGE('',*,*,#41382,.F.) ;
#56054=ORIENTED_EDGE('',*,*,#41384,.T.) ;
#56055=ORIENTED_EDGE('',*,*,#41385,.T.) ;
#56056=ORIENTED_EDGE('',*,*,#41386,.T.) ;
#56057=ORIENTED_EDGE('',*,*,#41385,.F.) ;
#56058=ORIENTED_EDGE('',*,*,#41387,.T.) ;
#56059=ORIENTED_EDGE('',*,*,#41388,.T.) ;
#56060=ORIENTED_EDGE('',*,*,#41389,.T.) ;
#56061=ORIENTED_EDGE('',*,*,#41388,.F.) ;
#56062=ORIENTED_EDGE('',*,*,#41390,.T.) ;
#56063=ORIENTED_EDGE('',*,*,#41391,.T.) ;
#56064=ORIENTED_EDGE('',*,*,#41392,.T.) ;
#56065=ORIENTED_EDGE('',*,*,#41391,.F.) ;
#56066=ORIENTED_EDGE('',*,*,#41393,.T.) ;
#56067=ORIENTED_EDGE('',*,*,#41394,.T.) ;
#56068=ORIENTED_EDGE('',*,*,#41395,.T.) ;
#56069=ORIENTED_EDGE('',*,*,#41394,.F.) ;
#56070=ORIENTED_EDGE('',*,*,#41396,.T.) ;
#56071=ORIENTED_EDGE('',*,*,#41397,.T.) ;
#56072=ORIENTED_EDGE('',*,*,#41398,.T.) ;
#56073=ORIENTED_EDGE('',*,*,#41397,.F.) ;
#56074=ORIENTED_EDGE('',*,*,#41399,.T.) ;
#56075=ORIENTED_EDGE('',*,*,#41400,.T.) ;
#56076=ORIENTED_EDGE('',*,*,#41401,.T.) ;
#56077=ORIENTED_EDGE('',*,*,#41400,.F.) ;
#56078=ORIENTED_EDGE('',*,*,#41402,.T.) ;
#56079=ORIENTED_EDGE('',*,*,#41403,.T.) ;
#56080=ORIENTED_EDGE('',*,*,#41404,.T.) ;
#56081=ORIENTED_EDGE('',*,*,#41403,.F.) ;
#56082=ORIENTED_EDGE('',*,*,#41405,.T.) ;
#56083=ORIENTED_EDGE('',*,*,#41406,.T.) ;
#56084=ORIENTED_EDGE('',*,*,#41407,.T.) ;
#56085=ORIENTED_EDGE('',*,*,#41406,.F.) ;
#56086=ORIENTED_EDGE('',*,*,#41408,.T.) ;
#56087=ORIENTED_EDGE('',*,*,#41409,.T.) ;
#56088=ORIENTED_EDGE('',*,*,#41410,.T.) ;
#56089=ORIENTED_EDGE('',*,*,#41409,.F.) ;
#56090=ORIENTED_EDGE('',*,*,#41411,.T.) ;
#56091=ORIENTED_EDGE('',*,*,#41412,.T.) ;
#56092=ORIENTED_EDGE('',*,*,#41413,.T.) ;
#56093=ORIENTED_EDGE('',*,*,#41412,.F.) ;
#56094=ORIENTED_EDGE('',*,*,#41414,.T.) ;
#56095=ORIENTED_EDGE('',*,*,#41415,.T.) ;
#56096=ORIENTED_EDGE('',*,*,#41416,.T.) ;
#56097=ORIENTED_EDGE('',*,*,#41415,.F.) ;
#56098=ORIENTED_EDGE('',*,*,#41417,.T.) ;
#56099=ORIENTED_EDGE('',*,*,#41340,.T.) ;
#56100=ORIENTED_EDGE('',*,*,#41418,.T.) ;
#56101=ORIENTED_EDGE('',*,*,#41419,.T.) ;
#56102=ORIENTED_EDGE('',*,*,#41420,.T.) ;
#56103=ORIENTED_EDGE('',*,*,#41421,.T.) ;
#56104=ORIENTED_EDGE('',*,*,#41422,.T.) ;
#56105=ORIENTED_EDGE('',*,*,#41423,.T.) ;
#56106=ORIENTED_EDGE('',*,*,#41424,.T.) ;
#56107=ORIENTED_EDGE('',*,*,#41425,.T.) ;
#56108=ORIENTED_EDGE('',*,*,#41426,.T.) ;
#56109=ORIENTED_EDGE('',*,*,#41427,.T.) ;
#56110=ORIENTED_EDGE('',*,*,#41428,.T.) ;
#56111=ORIENTED_EDGE('',*,*,#41429,.T.) ;
#56112=ORIENTED_EDGE('',*,*,#41430,.T.) ;
#56113=ORIENTED_EDGE('',*,*,#41431,.T.) ;
#56114=ORIENTED_EDGE('',*,*,#41432,.T.) ;
#56115=ORIENTED_EDGE('',*,*,#41433,.T.) ;
#56116=ORIENTED_EDGE('',*,*,#41434,.T.) ;
#56117=ORIENTED_EDGE('',*,*,#41435,.T.) ;
#56118=ORIENTED_EDGE('',*,*,#41436,.T.) ;
#56119=ORIENTED_EDGE('',*,*,#39211,.T.) ;
#56120=ORIENTED_EDGE('',*,*,#41437,.F.) ;
#56121=ORIENTED_EDGE('',*,*,#41438,.T.) ;
#56122=ORIENTED_EDGE('',*,*,#41439,.T.) ;
#56123=ORIENTED_EDGE('',*,*,#41440,.T.) ;
#56124=ORIENTED_EDGE('',*,*,#41439,.F.) ;
#56125=ORIENTED_EDGE('',*,*,#41441,.T.) ;
#56126=ORIENTED_EDGE('',*,*,#41442,.T.) ;
#56127=ORIENTED_EDGE('',*,*,#41443,.T.) ;
#56128=ORIENTED_EDGE('',*,*,#41442,.F.) ;
#56129=ORIENTED_EDGE('',*,*,#41444,.T.) ;
#56130=ORIENTED_EDGE('',*,*,#41445,.T.) ;
#56131=ORIENTED_EDGE('',*,*,#41446,.T.) ;
#56132=ORIENTED_EDGE('',*,*,#41445,.F.) ;
#56133=ORIENTED_EDGE('',*,*,#41447,.T.) ;
#56134=ORIENTED_EDGE('',*,*,#41448,.T.) ;
#56135=ORIENTED_EDGE('',*,*,#41449,.T.) ;
#56136=ORIENTED_EDGE('',*,*,#41448,.F.) ;
#56137=ORIENTED_EDGE('',*,*,#41450,.T.) ;
#56138=ORIENTED_EDGE('',*,*,#41451,.T.) ;
#56139=ORIENTED_EDGE('',*,*,#41452,.T.) ;
#56140=ORIENTED_EDGE('',*,*,#41451,.F.) ;
#56141=ORIENTED_EDGE('',*,*,#41453,.T.) ;
#56142=ORIENTED_EDGE('',*,*,#41454,.T.) ;
#56143=ORIENTED_EDGE('',*,*,#41455,.T.) ;
#56144=ORIENTED_EDGE('',*,*,#41454,.F.) ;
#56145=ORIENTED_EDGE('',*,*,#39267,.T.) ;
#56146=ORIENTED_EDGE('',*,*,#41456,.T.) ;
#56147=ORIENTED_EDGE('',*,*,#41457,.T.) ;
#56148=ORIENTED_EDGE('',*,*,#41456,.F.) ;
#56149=ORIENTED_EDGE('',*,*,#41458,.T.) ;
#56150=ORIENTED_EDGE('',*,*,#39288,.T.) ;
#56151=ORIENTED_EDGE('',*,*,#41459,.T.) ;
#56152=ORIENTED_EDGE('',*,*,#39287,.F.) ;
#56153=ORIENTED_EDGE('',*,*,#41460,.T.) ;
#56154=ORIENTED_EDGE('',*,*,#41461,.T.) ;
#56155=ORIENTED_EDGE('',*,*,#41462,.T.) ;
#56156=ORIENTED_EDGE('',*,*,#41461,.F.) ;
#56157=ORIENTED_EDGE('',*,*,#41463,.T.) ;
#56158=ORIENTED_EDGE('',*,*,#41464,.T.) ;
#56159=ORIENTED_EDGE('',*,*,#41465,.T.) ;
#56160=ORIENTED_EDGE('',*,*,#41464,.F.) ;
#56161=ORIENTED_EDGE('',*,*,#41466,.T.) ;
#56162=ORIENTED_EDGE('',*,*,#41467,.T.) ;
#56163=ORIENTED_EDGE('',*,*,#41468,.T.) ;
#56164=ORIENTED_EDGE('',*,*,#41467,.F.) ;
#56165=ORIENTED_EDGE('',*,*,#41469,.T.) ;
#56166=ORIENTED_EDGE('',*,*,#41470,.T.) ;
#56167=ORIENTED_EDGE('',*,*,#41471,.T.) ;
#56168=ORIENTED_EDGE('',*,*,#41470,.F.) ;
#56169=ORIENTED_EDGE('',*,*,#41472,.T.) ;
#56170=ORIENTED_EDGE('',*,*,#41473,.T.) ;
#56171=ORIENTED_EDGE('',*,*,#41474,.T.) ;
#56172=ORIENTED_EDGE('',*,*,#41473,.F.) ;
#56173=ORIENTED_EDGE('',*,*,#41475,.T.) ;
#56174=ORIENTED_EDGE('',*,*,#41476,.T.) ;
#56175=ORIENTED_EDGE('',*,*,#41477,.T.) ;
#56176=ORIENTED_EDGE('',*,*,#41476,.F.) ;
#56177=ORIENTED_EDGE('',*,*,#41478,.T.) ;
#56178=ORIENTED_EDGE('',*,*,#41479,.T.) ;
#56179=ORIENTED_EDGE('',*,*,#41480,.T.) ;
#56180=ORIENTED_EDGE('',*,*,#41479,.F.) ;
#56181=ORIENTED_EDGE('',*,*,#41481,.T.) ;
#56182=ORIENTED_EDGE('',*,*,#41482,.T.) ;
#56183=ORIENTED_EDGE('',*,*,#41483,.T.) ;
#56184=ORIENTED_EDGE('',*,*,#41482,.F.) ;
#56185=ORIENTED_EDGE('',*,*,#41484,.T.) ;
#56186=ORIENTED_EDGE('',*,*,#41485,.T.) ;
#56187=ORIENTED_EDGE('',*,*,#41486,.T.) ;
#56188=ORIENTED_EDGE('',*,*,#41485,.F.) ;
#56189=ORIENTED_EDGE('',*,*,#41487,.T.) ;
#56190=ORIENTED_EDGE('',*,*,#41488,.T.) ;
#56191=ORIENTED_EDGE('',*,*,#41489,.T.) ;
#56192=ORIENTED_EDGE('',*,*,#41488,.F.) ;
#56193=ORIENTED_EDGE('',*,*,#41490,.T.) ;
#56194=ORIENTED_EDGE('',*,*,#41491,.T.) ;
#56195=ORIENTED_EDGE('',*,*,#41492,.T.) ;
#56196=ORIENTED_EDGE('',*,*,#41491,.F.) ;
#56197=ORIENTED_EDGE('',*,*,#41493,.T.) ;
#56198=ORIENTED_EDGE('',*,*,#41494,.T.) ;
#56199=ORIENTED_EDGE('',*,*,#41495,.T.) ;
#56200=ORIENTED_EDGE('',*,*,#41494,.F.) ;
#56201=ORIENTED_EDGE('',*,*,#41496,.T.) ;
#56202=ORIENTED_EDGE('',*,*,#41497,.T.) ;
#56203=ORIENTED_EDGE('',*,*,#41498,.T.) ;
#56204=ORIENTED_EDGE('',*,*,#41497,.F.) ;
#56205=ORIENTED_EDGE('',*,*,#41499,.T.) ;
#56206=ORIENTED_EDGE('',*,*,#41500,.T.) ;
#56207=ORIENTED_EDGE('',*,*,#41501,.T.) ;
#56208=ORIENTED_EDGE('',*,*,#41500,.F.) ;
#56209=ORIENTED_EDGE('',*,*,#41502,.T.) ;
#56210=ORIENTED_EDGE('',*,*,#41503,.T.) ;
#56211=ORIENTED_EDGE('',*,*,#41504,.T.) ;
#56212=ORIENTED_EDGE('',*,*,#41503,.F.) ;
#56213=ORIENTED_EDGE('',*,*,#41505,.T.) ;
#56214=ORIENTED_EDGE('',*,*,#41506,.T.) ;
#56215=ORIENTED_EDGE('',*,*,#41507,.T.) ;
#56216=ORIENTED_EDGE('',*,*,#41506,.F.) ;
#56217=ORIENTED_EDGE('',*,*,#41508,.T.) ;
#56218=ORIENTED_EDGE('',*,*,#41509,.T.) ;
#56219=ORIENTED_EDGE('',*,*,#41510,.T.) ;
#56220=ORIENTED_EDGE('',*,*,#41509,.F.) ;
#56221=ORIENTED_EDGE('',*,*,#41511,.T.) ;
#56222=ORIENTED_EDGE('',*,*,#41512,.T.) ;
#56223=ORIENTED_EDGE('',*,*,#41513,.T.) ;
#56224=ORIENTED_EDGE('',*,*,#41512,.F.) ;
#56225=ORIENTED_EDGE('',*,*,#41514,.T.) ;
#56226=ORIENTED_EDGE('',*,*,#41437,.T.) ;
#56227=ORIENTED_EDGE('',*,*,#41515,.T.) ;
#56228=ORIENTED_EDGE('',*,*,#41516,.T.) ;
#56229=ORIENTED_EDGE('',*,*,#41517,.T.) ;
#56230=ORIENTED_EDGE('',*,*,#41518,.T.) ;
#56231=ORIENTED_EDGE('',*,*,#41519,.T.) ;
#56232=ORIENTED_EDGE('',*,*,#41520,.T.) ;
#56233=ORIENTED_EDGE('',*,*,#41521,.T.) ;
#56234=ORIENTED_EDGE('',*,*,#41522,.T.) ;
#56235=ORIENTED_EDGE('',*,*,#41523,.T.) ;
#56236=ORIENTED_EDGE('',*,*,#41524,.T.) ;
#56237=ORIENTED_EDGE('',*,*,#41525,.T.) ;
#56238=ORIENTED_EDGE('',*,*,#41526,.T.) ;
#56239=ORIENTED_EDGE('',*,*,#41527,.T.) ;
#56240=ORIENTED_EDGE('',*,*,#41528,.T.) ;
#56241=ORIENTED_EDGE('',*,*,#41529,.T.) ;
#56242=ORIENTED_EDGE('',*,*,#41530,.T.) ;
#56243=ORIENTED_EDGE('',*,*,#41531,.T.) ;
#56244=ORIENTED_EDGE('',*,*,#41532,.T.) ;
#56245=ORIENTED_EDGE('',*,*,#41533,.T.) ;
#56246=ORIENTED_EDGE('',*,*,#39264,.T.) ;
#56247=ORIENTED_EDGE('',*,*,#39224,.T.) ;
#56248=ORIENTED_EDGE('',*,*,#41534,.F.) ;
#56249=ORIENTED_EDGE('',*,*,#41535,.T.) ;
#56250=ORIENTED_EDGE('',*,*,#41536,.T.) ;
#56251=ORIENTED_EDGE('',*,*,#41537,.T.) ;
#56252=ORIENTED_EDGE('',*,*,#41538,.T.) ;
#56253=ORIENTED_EDGE('',*,*,#41539,.T.) ;
#56254=ORIENTED_EDGE('',*,*,#41540,.T.) ;
#56255=ORIENTED_EDGE('',*,*,#41541,.T.) ;
#56256=ORIENTED_EDGE('',*,*,#39207,.T.) ;
#56257=ORIENTED_EDGE('',*,*,#41542,.F.) ;
#56258=ORIENTED_EDGE('',*,*,#41543,.T.) ;
#56259=ORIENTED_EDGE('',*,*,#41544,.T.) ;
#56260=ORIENTED_EDGE('',*,*,#41545,.T.) ;
#56261=ORIENTED_EDGE('',*,*,#41546,.T.) ;
#56262=ORIENTED_EDGE('',*,*,#41547,.T.) ;
#56263=ORIENTED_EDGE('',*,*,#41548,.T.) ;
#56264=ORIENTED_EDGE('',*,*,#41549,.T.) ;
#56265=ORIENTED_EDGE('',*,*,#39190,.T.) ;
#56266=ORIENTED_EDGE('',*,*,#41550,.F.) ;
#56267=ORIENTED_EDGE('',*,*,#41551,.T.) ;
#56268=ORIENTED_EDGE('',*,*,#41552,.T.) ;
#56269=ORIENTED_EDGE('',*,*,#41553,.T.) ;
#56270=ORIENTED_EDGE('',*,*,#41554,.T.) ;
#56271=ORIENTED_EDGE('',*,*,#41555,.T.) ;
#56272=ORIENTED_EDGE('',*,*,#41556,.T.) ;
#56273=ORIENTED_EDGE('',*,*,#41557,.T.) ;
#56274=ORIENTED_EDGE('',*,*,#39173,.T.) ;
#56275=ORIENTED_EDGE('',*,*,#41558,.F.) ;
#56276=ORIENTED_EDGE('',*,*,#41559,.T.) ;
#56277=ORIENTED_EDGE('',*,*,#41560,.T.) ;
#56278=ORIENTED_EDGE('',*,*,#41561,.T.) ;
#56279=ORIENTED_EDGE('',*,*,#41562,.T.) ;
#56280=ORIENTED_EDGE('',*,*,#41563,.T.) ;
#56281=ORIENTED_EDGE('',*,*,#41564,.T.) ;
#56282=ORIENTED_EDGE('',*,*,#41565,.T.) ;
#56283=ORIENTED_EDGE('',*,*,#39156,.T.) ;
#56284=ORIENTED_EDGE('',*,*,#41566,.F.) ;
#56285=ORIENTED_EDGE('',*,*,#41567,.T.) ;
#56286=ORIENTED_EDGE('',*,*,#41568,.T.) ;
#56287=ORIENTED_EDGE('',*,*,#41569,.T.) ;
#56288=ORIENTED_EDGE('',*,*,#41570,.T.) ;
#56289=ORIENTED_EDGE('',*,*,#41571,.T.) ;
#56290=ORIENTED_EDGE('',*,*,#41572,.T.) ;
#56291=ORIENTED_EDGE('',*,*,#41573,.T.) ;
#56292=ORIENTED_EDGE('',*,*,#39139,.T.) ;
#56293=ORIENTED_EDGE('',*,*,#41574,.F.) ;
#56294=ORIENTED_EDGE('',*,*,#41575,.T.) ;
#56295=ORIENTED_EDGE('',*,*,#41576,.T.) ;
#56296=ORIENTED_EDGE('',*,*,#41577,.T.) ;
#56297=ORIENTED_EDGE('',*,*,#41578,.T.) ;
#56298=ORIENTED_EDGE('',*,*,#41579,.T.) ;
#56299=ORIENTED_EDGE('',*,*,#41580,.T.) ;
#56300=ORIENTED_EDGE('',*,*,#41581,.T.) ;
#56301=ORIENTED_EDGE('',*,*,#39122,.T.) ;
#56302=ORIENTED_EDGE('',*,*,#41582,.F.) ;
#56303=ORIENTED_EDGE('',*,*,#41583,.T.) ;
#56304=ORIENTED_EDGE('',*,*,#41584,.T.) ;
#56305=ORIENTED_EDGE('',*,*,#41585,.T.) ;
#56306=ORIENTED_EDGE('',*,*,#41586,.T.) ;
#56307=ORIENTED_EDGE('',*,*,#41587,.T.) ;
#56308=ORIENTED_EDGE('',*,*,#41588,.T.) ;
#56309=ORIENTED_EDGE('',*,*,#41589,.T.) ;
#56310=ORIENTED_EDGE('',*,*,#39105,.T.) ;
#56311=ORIENTED_EDGE('',*,*,#41590,.F.) ;
#56312=ORIENTED_EDGE('',*,*,#41591,.T.) ;
#56313=ORIENTED_EDGE('',*,*,#41592,.T.) ;
#56314=ORIENTED_EDGE('',*,*,#41593,.T.) ;
#56315=ORIENTED_EDGE('',*,*,#41594,.T.) ;
#56316=ORIENTED_EDGE('',*,*,#41595,.T.) ;
#56317=ORIENTED_EDGE('',*,*,#41596,.T.) ;
#56318=ORIENTED_EDGE('',*,*,#41597,.T.) ;
#56319=ORIENTED_EDGE('',*,*,#39088,.T.) ;
#56320=ORIENTED_EDGE('',*,*,#41598,.F.) ;
#56321=ORIENTED_EDGE('',*,*,#41599,.T.) ;
#56322=ORIENTED_EDGE('',*,*,#41600,.T.) ;
#56323=ORIENTED_EDGE('',*,*,#41601,.T.) ;
#56324=ORIENTED_EDGE('',*,*,#41602,.T.) ;
#56325=ORIENTED_EDGE('',*,*,#41603,.T.) ;
#56326=ORIENTED_EDGE('',*,*,#41604,.T.) ;
#56327=ORIENTED_EDGE('',*,*,#41605,.T.) ;
#56328=ORIENTED_EDGE('',*,*,#41606,.F.) ;
#56329=ORIENTED_EDGE('',*,*,#40502,.F.) ;
#56330=ORIENTED_EDGE('',*,*,#41607,.F.) ;
#56331=ORIENTED_EDGE('',*,*,#40489,.F.) ;
#56332=ORIENTED_EDGE('',*,*,#41608,.F.) ;
#56333=ORIENTED_EDGE('',*,*,#40503,.F.) ;
#56334=ORIENTED_EDGE('',*,*,#41609,.F.) ;
#56335=ORIENTED_EDGE('',*,*,#40497,.F.) ;
#56336=ORIENTED_EDGE('',*,*,#41610,.F.) ;
#56337=ORIENTED_EDGE('',*,*,#41608,.T.) ;
#56338=ORIENTED_EDGE('',*,*,#41611,.F.) ;
#56339=ORIENTED_EDGE('',*,*,#41612,.F.) ;
#56340=ORIENTED_EDGE('',*,*,#41607,.T.) ;
#56341=ORIENTED_EDGE('',*,*,#41613,.F.) ;
#56342=ORIENTED_EDGE('',*,*,#41606,.T.) ;
#56343=ORIENTED_EDGE('',*,*,#40488,.T.) ;
#56344=ORIENTED_EDGE('',*,*,#41614,.F.) ;
#56345=ORIENTED_EDGE('',*,*,#41609,.T.) ;
#56346=ORIENTED_EDGE('',*,*,#41611,.T.) ;
#56347=ORIENTED_EDGE('',*,*,#40500,.F.) ;
#56348=ORIENTED_EDGE('',*,*,#41615,.F.) ;
#56349=ORIENTED_EDGE('',*,*,#39270,.T.) ;
#56350=ORIENTED_EDGE('',*,*,#41616,.T.) ;
#56351=ORIENTED_EDGE('',*,*,#41617,.F.) ;
#56352=ORIENTED_EDGE('',*,*,#41610,.T.) ;
#56353=ORIENTED_EDGE('',*,*,#41618,.F.) ;
#56354=ORIENTED_EDGE('',*,*,#41619,.T.) ;
#56355=ORIENTED_EDGE('',*,*,#41620,.F.) ;
#56356=ORIENTED_EDGE('',*,*,#39426,.F.) ;
#56357=ORIENTED_EDGE('',*,*,#41621,.F.) ;
#56358=ORIENTED_EDGE('',*,*,#40504,.F.) ;
#56359=ORIENTED_EDGE('',*,*,#41613,.T.) ;
#56360=ORIENTED_EDGE('',*,*,#40501,.F.) ;
#56361=ORIENTED_EDGE('',*,*,#41622,.F.) ;
#56362=ORIENTED_EDGE('',*,*,#40507,.F.) ;
#56363=ORIENTED_EDGE('',*,*,#41612,.T.) ;
#56364=ORIENTED_EDGE('',*,*,#40506,.F.) ;
#56365=ORIENTED_EDGE('',*,*,#41623,.F.) ;
#56366=ORIENTED_EDGE('',*,*,#40480,.F.) ;
#56367=ORIENTED_EDGE('',*,*,#41614,.T.) ;
#56368=ORIENTED_EDGE('',*,*,#40487,.F.) ;
#56369=ORIENTED_EDGE('',*,*,#41624,.F.) ;
#56370=ORIENTED_EDGE('',*,*,#40498,.F.) ;
#56371=ORIENTED_EDGE('',*,*,#41625,.F.) ;
#56372=ORIENTED_EDGE('',*,*,#40499,.F.) ;
#56373=ORIENTED_EDGE('',*,*,#41626,.F.) ;
#56374=ORIENTED_EDGE('',*,*,#40494,.F.) ;
#56375=ORIENTED_EDGE('',*,*,#41615,.T.) ;
#56376=ORIENTED_EDGE('',*,*,#41625,.T.) ;
#56377=ORIENTED_EDGE('',*,*,#39271,.F.) ;
#56378=ORIENTED_EDGE('',*,*,#41621,.T.) ;
#56379=ORIENTED_EDGE('',*,*,#39436,.T.) ;
#56380=ORIENTED_EDGE('',*,*,#41627,.F.) ;
#56381=ORIENTED_EDGE('',*,*,#41622,.T.) ;
#56382=ORIENTED_EDGE('',*,*,#41628,.F.) ;
#56383=ORIENTED_EDGE('',*,*,#41623,.T.) ;
#56384=ORIENTED_EDGE('',*,*,#41629,.F.) ;
#56385=ORIENTED_EDGE('',*,*,#39522,.T.) ;
#56386=ORIENTED_EDGE('',*,*,#41624,.T.) ;
#56387=ORIENTED_EDGE('',*,*,#40486,.T.) ;
#56388=ORIENTED_EDGE('',*,*,#41630,.F.) ;
#56389=ORIENTED_EDGE('',*,*,#41626,.T.) ;
#56390=ORIENTED_EDGE('',*,*,#41627,.T.) ;
#56391=ORIENTED_EDGE('',*,*,#39435,.F.) ;
#56392=ORIENTED_EDGE('',*,*,#41631,.F.) ;
#56393=ORIENTED_EDGE('',*,*,#40508,.F.) ;
#56394=ORIENTED_EDGE('',*,*,#41629,.T.) ;
#56395=ORIENTED_EDGE('',*,*,#40505,.F.) ;
#56396=ORIENTED_EDGE('',*,*,#41632,.F.) ;
#56397=ORIENTED_EDGE('',*,*,#39523,.F.) ;
#56398=ORIENTED_EDGE('',*,*,#40481,.F.) ;
#56399=ORIENTED_EDGE('',*,*,#41628,.T.) ;
#56400=ORIENTED_EDGE('',*,*,#41633,.F.) ;
#56401=ORIENTED_EDGE('',*,*,#41634,.F.) ;
#56402=ORIENTED_EDGE('',*,*,#41630,.T.) ;
#56403=ORIENTED_EDGE('',*,*,#40485,.F.) ;
#56404=ORIENTED_EDGE('',*,*,#41635,.F.) ;
#56405=ORIENTED_EDGE('',*,*,#40495,.F.) ;
#56406=ORIENTED_EDGE('',*,*,#41636,.F.) ;
#56407=ORIENTED_EDGE('',*,*,#40496,.F.) ;
#56408=ORIENTED_EDGE('',*,*,#41637,.F.) ;
#56409=ORIENTED_EDGE('',*,*,#40490,.F.) ;
#56410=ORIENTED_EDGE('',*,*,#39273,.T.) ;
#56411=ORIENTED_EDGE('',*,*,#41636,.T.) ;
#56412=ORIENTED_EDGE('',*,*,#41638,.F.) ;
#56413=ORIENTED_EDGE('',*,*,#39430,.T.) ;
#56414=ORIENTED_EDGE('',*,*,#41632,.T.) ;
#56415=ORIENTED_EDGE('',*,*,#41631,.T.) ;
#56416=ORIENTED_EDGE('',*,*,#41639,.F.) ;
#56417=ORIENTED_EDGE('',*,*,#41640,.F.) ;
#56418=ORIENTED_EDGE('',*,*,#39528,.F.) ;
#56419=ORIENTED_EDGE('',*,*,#41641,.F.) ;
#56420=ORIENTED_EDGE('',*,*,#41642,.F.) ;
#56421=ORIENTED_EDGE('',*,*,#41633,.T.) ;
#56422=ORIENTED_EDGE('',*,*,#39526,.F.) ;
#56423=ORIENTED_EDGE('',*,*,#41641,.T.) ;
#56424=ORIENTED_EDGE('',*,*,#39689,.F.) ;
#56425=ORIENTED_EDGE('',*,*,#41634,.T.) ;
#56426=ORIENTED_EDGE('',*,*,#41643,.F.) ;
#56427=ORIENTED_EDGE('',*,*,#41644,.F.) ;
#56428=ORIENTED_EDGE('',*,*,#41637,.T.) ;
#56429=ORIENTED_EDGE('',*,*,#41635,.T.) ;
#56430=ORIENTED_EDGE('',*,*,#41645,.F.) ;
#56431=ORIENTED_EDGE('',*,*,#41638,.T.) ;
#56432=ORIENTED_EDGE('',*,*,#40493,.F.) ;
#56433=ORIENTED_EDGE('',*,*,#41646,.F.) ;
#56434=ORIENTED_EDGE('',*,*,#39431,.F.) ;
#56435=ORIENTED_EDGE('',*,*,#41639,.T.) ;
#56436=ORIENTED_EDGE('',*,*,#39434,.F.) ;
#56437=ORIENTED_EDGE('',*,*,#41647,.F.) ;
#56438=ORIENTED_EDGE('',*,*,#39524,.F.) ;
#56439=ORIENTED_EDGE('',*,*,#41640,.T.) ;
#56440=ORIENTED_EDGE('',*,*,#39525,.F.) ;
#56441=ORIENTED_EDGE('',*,*,#41648,.F.) ;
#56442=ORIENTED_EDGE('',*,*,#39602,.F.) ;
#56443=ORIENTED_EDGE('',*,*,#41642,.T.) ;
#56444=ORIENTED_EDGE('',*,*,#39688,.T.) ;
#56445=ORIENTED_EDGE('',*,*,#41649,.F.) ;
#56446=ORIENTED_EDGE('',*,*,#41643,.T.) ;
#56447=ORIENTED_EDGE('',*,*,#40482,.F.) ;
#56448=ORIENTED_EDGE('',*,*,#41644,.T.) ;
#56449=ORIENTED_EDGE('',*,*,#41650,.F.) ;
#56450=ORIENTED_EDGE('',*,*,#41651,.F.) ;
#56451=ORIENTED_EDGE('',*,*,#41645,.T.) ;
#56452=ORIENTED_EDGE('',*,*,#40484,.F.) ;
#56453=ORIENTED_EDGE('',*,*,#41652,.F.) ;
#56454=ORIENTED_EDGE('',*,*,#40491,.F.) ;
#56455=ORIENTED_EDGE('',*,*,#41653,.F.) ;
#56456=ORIENTED_EDGE('',*,*,#40492,.F.) ;
#56457=ORIENTED_EDGE('',*,*,#41654,.F.) ;
#56458=ORIENTED_EDGE('',*,*,#39521,.F.) ;
#56459=ORIENTED_EDGE('',*,*,#41646,.T.) ;
#56460=ORIENTED_EDGE('',*,*,#41653,.T.) ;
#56461=ORIENTED_EDGE('',*,*,#41655,.F.) ;
#56462=ORIENTED_EDGE('',*,*,#41648,.T.) ;
#56463=ORIENTED_EDGE('',*,*,#41647,.T.) ;
#56464=ORIENTED_EDGE('',*,*,#41656,.F.) ;
#56465=ORIENTED_EDGE('',*,*,#39603,.T.) ;
#56466=ORIENTED_EDGE('',*,*,#41657,.F.) ;
#56467=ORIENTED_EDGE('',*,*,#41650,.T.) ;
#56468=ORIENTED_EDGE('',*,*,#41649,.T.) ;
#56469=ORIENTED_EDGE('',*,*,#39687,.F.) ;
#56470=ORIENTED_EDGE('',*,*,#41651,.T.) ;
#56471=ORIENTED_EDGE('',*,*,#41658,.F.) ;
#56472=ORIENTED_EDGE('',*,*,#41659,.F.) ;
#56473=ORIENTED_EDGE('',*,*,#41654,.T.) ;
#56474=ORIENTED_EDGE('',*,*,#41652,.T.) ;
#56475=ORIENTED_EDGE('',*,*,#41660,.F.) ;
#56476=ORIENTED_EDGE('',*,*,#39517,.T.) ;
#56477=ORIENTED_EDGE('',*,*,#41655,.T.) ;
#56478=ORIENTED_EDGE('',*,*,#39520,.F.) ;
#56479=ORIENTED_EDGE('',*,*,#41661,.F.) ;
#56480=ORIENTED_EDGE('',*,*,#39432,.F.) ;
#56481=ORIENTED_EDGE('',*,*,#41656,.T.) ;
#56482=ORIENTED_EDGE('',*,*,#39433,.F.) ;
#56483=ORIENTED_EDGE('',*,*,#41662,.F.) ;
#56484=ORIENTED_EDGE('',*,*,#39604,.F.) ;
#56485=ORIENTED_EDGE('',*,*,#41657,.T.) ;
#56486=ORIENTED_EDGE('',*,*,#39686,.T.) ;
#56487=ORIENTED_EDGE('',*,*,#41663,.F.) ;
#56488=ORIENTED_EDGE('',*,*,#41658,.T.) ;
#56489=ORIENTED_EDGE('',*,*,#40483,.F.) ;
#56490=ORIENTED_EDGE('',*,*,#41659,.T.) ;
#56491=ORIENTED_EDGE('',*,*,#41664,.F.) ;
#56492=ORIENTED_EDGE('',*,*,#41660,.T.) ;
#56493=ORIENTED_EDGE('',*,*,#41662,.T.) ;
#56494=ORIENTED_EDGE('',*,*,#41661,.T.) ;
#56495=ORIENTED_EDGE('',*,*,#41665,.F.) ;
#56496=ORIENTED_EDGE('',*,*,#39605,.T.) ;
#56497=ORIENTED_EDGE('',*,*,#41663,.T.) ;
#56498=ORIENTED_EDGE('',*,*,#39685,.F.) ;
#56499=ORIENTED_EDGE('',*,*,#41666,.F.) ;
#56500=ORIENTED_EDGE('',*,*,#39518,.F.) ;
#56501=ORIENTED_EDGE('',*,*,#41664,.T.) ;
#56502=ORIENTED_EDGE('',*,*,#41665,.T.) ;
#56503=ORIENTED_EDGE('',*,*,#39519,.F.) ;
#56504=ORIENTED_EDGE('',*,*,#41667,.F.) ;
#56505=ORIENTED_EDGE('',*,*,#39606,.F.) ;
#56506=ORIENTED_EDGE('',*,*,#41666,.T.) ;
#56507=ORIENTED_EDGE('',*,*,#39534,.F.) ;
#56508=ORIENTED_EDGE('',*,*,#41667,.T.) ;
#56509=ORIENTED_EDGE('',*,*,#41668,.F.) ;
#56510=ORIENTED_EDGE('',*,*,#41478,.F.) ;
#56511=ORIENTED_EDGE('',*,*,#41669,.F.) ;
#56512=ORIENTED_EDGE('',*,*,#41525,.F.) ;
#56513=ORIENTED_EDGE('',*,*,#41669,.T.) ;
#56514=ORIENTED_EDGE('',*,*,#41475,.F.) ;
#56515=ORIENTED_EDGE('',*,*,#41670,.F.) ;
#56516=ORIENTED_EDGE('',*,*,#41526,.F.) ;
#56517=ORIENTED_EDGE('',*,*,#41481,.F.) ;
#56518=ORIENTED_EDGE('',*,*,#41668,.T.) ;
#56519=ORIENTED_EDGE('',*,*,#41671,.F.) ;
#56520=ORIENTED_EDGE('',*,*,#41670,.T.) ;
#56521=ORIENTED_EDGE('',*,*,#41472,.F.) ;
#56522=ORIENTED_EDGE('',*,*,#41672,.F.) ;
#56523=ORIENTED_EDGE('',*,*,#41527,.F.) ;
#56524=ORIENTED_EDGE('',*,*,#41671,.T.) ;
#56525=ORIENTED_EDGE('',*,*,#41524,.F.) ;
#56526=ORIENTED_EDGE('',*,*,#41673,.F.) ;
#56527=ORIENTED_EDGE('',*,*,#41484,.F.) ;
#56528=ORIENTED_EDGE('',*,*,#41672,.T.) ;
#56529=ORIENTED_EDGE('',*,*,#41469,.F.) ;
#56530=ORIENTED_EDGE('',*,*,#41674,.F.) ;
#56531=ORIENTED_EDGE('',*,*,#41528,.F.) ;
#56532=ORIENTED_EDGE('',*,*,#41487,.F.) ;
#56533=ORIENTED_EDGE('',*,*,#41673,.T.) ;
#56534=ORIENTED_EDGE('',*,*,#41675,.F.) ;
#56535=ORIENTED_EDGE('',*,*,#41674,.T.) ;
#56536=ORIENTED_EDGE('',*,*,#41466,.F.) ;
#56537=ORIENTED_EDGE('',*,*,#41676,.F.) ;
#56538=ORIENTED_EDGE('',*,*,#41529,.F.) ;
#56539=ORIENTED_EDGE('',*,*,#41675,.T.) ;
#56540=ORIENTED_EDGE('',*,*,#41523,.F.) ;
#56541=ORIENTED_EDGE('',*,*,#41677,.F.) ;
#56542=ORIENTED_EDGE('',*,*,#41490,.F.) ;
#56543=ORIENTED_EDGE('',*,*,#41676,.T.) ;
#56544=ORIENTED_EDGE('',*,*,#41463,.F.) ;
#56545=ORIENTED_EDGE('',*,*,#41678,.F.) ;
#56546=ORIENTED_EDGE('',*,*,#41493,.F.) ;
#56547=ORIENTED_EDGE('',*,*,#41677,.T.) ;
#56548=ORIENTED_EDGE('',*,*,#41679,.F.) ;
#56549=ORIENTED_EDGE('',*,*,#41678,.T.) ;
#56550=ORIENTED_EDGE('',*,*,#41460,.F.) ;
#56551=ORIENTED_EDGE('',*,*,#41680,.F.) ;
#56552=ORIENTED_EDGE('',*,*,#41530,.F.) ;
#56553=ORIENTED_EDGE('',*,*,#41679,.T.) ;
#56554=ORIENTED_EDGE('',*,*,#41522,.F.) ;
#56555=ORIENTED_EDGE('',*,*,#41681,.F.) ;
#56556=ORIENTED_EDGE('',*,*,#41496,.F.) ;
#56557=ORIENTED_EDGE('',*,*,#41680,.T.) ;
#56558=ORIENTED_EDGE('',*,*,#39286,.F.) ;
#56559=ORIENTED_EDGE('',*,*,#41682,.F.) ;
#56560=ORIENTED_EDGE('',*,*,#41499,.F.) ;
#56561=ORIENTED_EDGE('',*,*,#41681,.T.) ;
#56562=ORIENTED_EDGE('',*,*,#41683,.F.) ;
#56563=ORIENTED_EDGE('',*,*,#41682,.T.) ;
#56564=ORIENTED_EDGE('',*,*,#41458,.F.) ;
#56565=ORIENTED_EDGE('',*,*,#39269,.F.) ;
#56566=ORIENTED_EDGE('',*,*,#41531,.F.) ;
#56567=ORIENTED_EDGE('',*,*,#41683,.T.) ;
#56568=ORIENTED_EDGE('',*,*,#41521,.F.) ;
#56569=ORIENTED_EDGE('',*,*,#41684,.F.) ;
#56570=ORIENTED_EDGE('',*,*,#41502,.F.) ;
#56571=ORIENTED_EDGE('',*,*,#41505,.F.) ;
#56572=ORIENTED_EDGE('',*,*,#41684,.T.) ;
#56573=ORIENTED_EDGE('',*,*,#41685,.F.) ;
#56574=ORIENTED_EDGE('',*,*,#39268,.T.) ;
#56575=ORIENTED_EDGE('',*,*,#41453,.F.) ;
#56576=ORIENTED_EDGE('',*,*,#41686,.F.) ;
#56577=ORIENTED_EDGE('',*,*,#41532,.F.) ;
#56578=ORIENTED_EDGE('',*,*,#41685,.T.) ;
#56579=ORIENTED_EDGE('',*,*,#41520,.F.) ;
#56580=ORIENTED_EDGE('',*,*,#41687,.F.) ;
#56581=ORIENTED_EDGE('',*,*,#41508,.F.) ;
#56582=ORIENTED_EDGE('',*,*,#41686,.T.) ;
#56583=ORIENTED_EDGE('',*,*,#41450,.F.) ;
#56584=ORIENTED_EDGE('',*,*,#41688,.F.) ;
#56585=ORIENTED_EDGE('',*,*,#41511,.F.) ;
#56586=ORIENTED_EDGE('',*,*,#41687,.T.) ;
#56587=ORIENTED_EDGE('',*,*,#41689,.F.) ;
#56588=ORIENTED_EDGE('',*,*,#41688,.T.) ;
#56589=ORIENTED_EDGE('',*,*,#41447,.F.) ;
#56590=ORIENTED_EDGE('',*,*,#41690,.F.) ;
#56591=ORIENTED_EDGE('',*,*,#41533,.F.) ;
#56592=ORIENTED_EDGE('',*,*,#41689,.T.) ;
#56593=ORIENTED_EDGE('',*,*,#41519,.F.) ;
#56594=ORIENTED_EDGE('',*,*,#41691,.F.) ;
#56595=ORIENTED_EDGE('',*,*,#41514,.F.) ;
#56596=ORIENTED_EDGE('',*,*,#41690,.T.) ;
#56597=ORIENTED_EDGE('',*,*,#41444,.F.) ;
#56598=ORIENTED_EDGE('',*,*,#41692,.F.) ;
#56599=ORIENTED_EDGE('',*,*,#41516,.F.) ;
#56600=ORIENTED_EDGE('',*,*,#41691,.T.) ;
#56601=ORIENTED_EDGE('',*,*,#41518,.F.) ;
#56602=ORIENTED_EDGE('',*,*,#41693,.F.) ;
#56603=ORIENTED_EDGE('',*,*,#41438,.F.) ;
#56604=ORIENTED_EDGE('',*,*,#41692,.T.) ;
#56605=ORIENTED_EDGE('',*,*,#41441,.F.) ;
#56606=ORIENTED_EDGE('',*,*,#41693,.T.) ;
#56607=ORIENTED_EDGE('',*,*,#41517,.F.) ;
#56608=ORIENTED_EDGE('',*,*,#41694,.F.) ;
#56609=ORIENTED_EDGE('',*,*,#40698,.F.) ;
#56610=ORIENTED_EDGE('',*,*,#41695,.F.) ;
#56611=ORIENTED_EDGE('',*,*,#39747,.F.) ;
#56612=ORIENTED_EDGE('',*,*,#40695,.F.) ;
#56613=ORIENTED_EDGE('',*,*,#41694,.T.) ;
#56614=ORIENTED_EDGE('',*,*,#41696,.F.) ;
#56615=ORIENTED_EDGE('',*,*,#41695,.T.) ;
#56616=ORIENTED_EDGE('',*,*,#40701,.F.) ;
#56617=ORIENTED_EDGE('',*,*,#41697,.F.) ;
#56618=ORIENTED_EDGE('',*,*,#41696,.T.) ;
#56619=ORIENTED_EDGE('',*,*,#39746,.F.) ;
#56620=ORIENTED_EDGE('',*,*,#41698,.F.) ;
#56621=ORIENTED_EDGE('',*,*,#40692,.F.) ;
#56622=ORIENTED_EDGE('',*,*,#41697,.T.) ;
#56623=ORIENTED_EDGE('',*,*,#40704,.F.) ;
#56624=ORIENTED_EDGE('',*,*,#41699,.F.) ;
#56625=ORIENTED_EDGE('',*,*,#39748,.F.) ;
#56626=ORIENTED_EDGE('',*,*,#41698,.T.) ;
#56627=ORIENTED_EDGE('',*,*,#39745,.F.) ;
#56628=ORIENTED_EDGE('',*,*,#41700,.F.) ;
#56629=ORIENTED_EDGE('',*,*,#40689,.F.) ;
#56630=ORIENTED_EDGE('',*,*,#41699,.T.) ;
#56631=ORIENTED_EDGE('',*,*,#40707,.F.) ;
#56632=ORIENTED_EDGE('',*,*,#41701,.F.) ;
#56633=ORIENTED_EDGE('',*,*,#39749,.F.) ;
#56634=ORIENTED_EDGE('',*,*,#41700,.T.) ;
#56635=ORIENTED_EDGE('',*,*,#39744,.F.) ;
#56636=ORIENTED_EDGE('',*,*,#39263,.F.) ;
#56637=ORIENTED_EDGE('',*,*,#40686,.F.) ;
#56638=ORIENTED_EDGE('',*,*,#41701,.T.) ;
#56639=ORIENTED_EDGE('',*,*,#40710,.F.) ;
#56640=ORIENTED_EDGE('',*,*,#41702,.F.) ;
#56641=ORIENTED_EDGE('',*,*,#39750,.F.) ;
#56642=ORIENTED_EDGE('',*,*,#41702,.T.) ;
#56643=ORIENTED_EDGE('',*,*,#40713,.F.) ;
#56644=ORIENTED_EDGE('',*,*,#41703,.F.) ;
#56645=ORIENTED_EDGE('',*,*,#39751,.F.) ;
#56646=ORIENTED_EDGE('',*,*,#39261,.T.) ;
#56647=ORIENTED_EDGE('',*,*,#39743,.F.) ;
#56648=ORIENTED_EDGE('',*,*,#41704,.F.) ;
#56649=ORIENTED_EDGE('',*,*,#40683,.F.) ;
#56650=ORIENTED_EDGE('',*,*,#41703,.T.) ;
#56651=ORIENTED_EDGE('',*,*,#40716,.F.) ;
#56652=ORIENTED_EDGE('',*,*,#41705,.F.) ;
#56653=ORIENTED_EDGE('',*,*,#39752,.F.) ;
#56654=ORIENTED_EDGE('',*,*,#41704,.T.) ;
#56655=ORIENTED_EDGE('',*,*,#39742,.F.) ;
#56656=ORIENTED_EDGE('',*,*,#41706,.F.) ;
#56657=ORIENTED_EDGE('',*,*,#40681,.F.) ;
#56658=ORIENTED_EDGE('',*,*,#41705,.T.) ;
#56659=ORIENTED_EDGE('',*,*,#40719,.F.) ;
#56660=ORIENTED_EDGE('',*,*,#41707,.F.) ;
#56661=ORIENTED_EDGE('',*,*,#39753,.F.) ;
#56662=ORIENTED_EDGE('',*,*,#41706,.T.) ;
#56663=ORIENTED_EDGE('',*,*,#39741,.F.) ;
#56664=ORIENTED_EDGE('',*,*,#41708,.F.) ;
#56665=ORIENTED_EDGE('',*,*,#40679,.F.) ;
#56666=ORIENTED_EDGE('',*,*,#41707,.T.) ;
#56667=ORIENTED_EDGE('',*,*,#40722,.F.) ;
#56668=ORIENTED_EDGE('',*,*,#41709,.F.) ;
#56669=ORIENTED_EDGE('',*,*,#39754,.F.) ;
#56670=ORIENTED_EDGE('',*,*,#41708,.T.) ;
#56671=ORIENTED_EDGE('',*,*,#39740,.F.) ;
#56672=ORIENTED_EDGE('',*,*,#41710,.F.) ;
#56673=ORIENTED_EDGE('',*,*,#40676,.F.) ;
#56674=ORIENTED_EDGE('',*,*,#41709,.T.) ;
#56675=ORIENTED_EDGE('',*,*,#40725,.F.) ;
#56676=ORIENTED_EDGE('',*,*,#41711,.F.) ;
#56677=ORIENTED_EDGE('',*,*,#39755,.F.) ;
#56678=ORIENTED_EDGE('',*,*,#41710,.T.) ;
#56679=ORIENTED_EDGE('',*,*,#39739,.F.) ;
#56680=ORIENTED_EDGE('',*,*,#41712,.F.) ;
#56681=ORIENTED_EDGE('',*,*,#40673,.F.) ;
#56682=ORIENTED_EDGE('',*,*,#41711,.T.) ;
#56683=ORIENTED_EDGE('',*,*,#40728,.F.) ;
#56684=ORIENTED_EDGE('',*,*,#41713,.F.) ;
#56685=ORIENTED_EDGE('',*,*,#39756,.F.) ;
#56686=ORIENTED_EDGE('',*,*,#40670,.F.) ;
#56687=ORIENTED_EDGE('',*,*,#41712,.T.) ;
#56688=ORIENTED_EDGE('',*,*,#41714,.F.) ;
#56689=ORIENTED_EDGE('',*,*,#41713,.T.) ;
#56690=ORIENTED_EDGE('',*,*,#40731,.F.) ;
#56691=ORIENTED_EDGE('',*,*,#41715,.F.) ;
#56692=ORIENTED_EDGE('',*,*,#39757,.F.) ;
#56693=ORIENTED_EDGE('',*,*,#41714,.T.) ;
#56694=ORIENTED_EDGE('',*,*,#39738,.F.) ;
#56695=ORIENTED_EDGE('',*,*,#41716,.F.) ;
#56696=ORIENTED_EDGE('',*,*,#40667,.F.) ;
#56697=ORIENTED_EDGE('',*,*,#41715,.T.) ;
#56698=ORIENTED_EDGE('',*,*,#40734,.F.) ;
#56699=ORIENTED_EDGE('',*,*,#41717,.F.) ;
#56700=ORIENTED_EDGE('',*,*,#39758,.F.) ;
#56701=ORIENTED_EDGE('',*,*,#40664,.F.) ;
#56702=ORIENTED_EDGE('',*,*,#41716,.T.) ;
#56703=ORIENTED_EDGE('',*,*,#41718,.F.) ;
#56704=ORIENTED_EDGE('',*,*,#41717,.T.) ;
#56705=ORIENTED_EDGE('',*,*,#40737,.F.) ;
#56706=ORIENTED_EDGE('',*,*,#41719,.F.) ;
#56707=ORIENTED_EDGE('',*,*,#39736,.F.) ;
#56708=ORIENTED_EDGE('',*,*,#41718,.T.) ;
#56709=ORIENTED_EDGE('',*,*,#39737,.F.) ;
#56710=ORIENTED_EDGE('',*,*,#41719,.T.) ;
#56711=ORIENTED_EDGE('',*,*,#40739,.F.) ;
#56712=ORIENTED_EDGE('',*,*,#41720,.F.) ;
#56713=ORIENTED_EDGE('',*,*,#40795,.F.) ;
#56714=ORIENTED_EDGE('',*,*,#41721,.F.) ;
#56715=ORIENTED_EDGE('',*,*,#39770,.F.) ;
#56716=ORIENTED_EDGE('',*,*,#40792,.F.) ;
#56717=ORIENTED_EDGE('',*,*,#41720,.T.) ;
#56718=ORIENTED_EDGE('',*,*,#41722,.F.) ;
#56719=ORIENTED_EDGE('',*,*,#41721,.T.) ;
#56720=ORIENTED_EDGE('',*,*,#40798,.F.) ;
#56721=ORIENTED_EDGE('',*,*,#41723,.F.) ;
#56722=ORIENTED_EDGE('',*,*,#41722,.T.) ;
#56723=ORIENTED_EDGE('',*,*,#39769,.F.) ;
#56724=ORIENTED_EDGE('',*,*,#41724,.F.) ;
#56725=ORIENTED_EDGE('',*,*,#40789,.F.) ;
#56726=ORIENTED_EDGE('',*,*,#41723,.T.) ;
#56727=ORIENTED_EDGE('',*,*,#40801,.F.) ;
#56728=ORIENTED_EDGE('',*,*,#41725,.F.) ;
#56729=ORIENTED_EDGE('',*,*,#39771,.F.) ;
#56730=ORIENTED_EDGE('',*,*,#41724,.T.) ;
#56731=ORIENTED_EDGE('',*,*,#39768,.F.) ;
#56732=ORIENTED_EDGE('',*,*,#41726,.F.) ;
#56733=ORIENTED_EDGE('',*,*,#40786,.F.) ;
#56734=ORIENTED_EDGE('',*,*,#41725,.T.) ;
#56735=ORIENTED_EDGE('',*,*,#40804,.F.) ;
#56736=ORIENTED_EDGE('',*,*,#41727,.F.) ;
#56737=ORIENTED_EDGE('',*,*,#39772,.F.) ;
#56738=ORIENTED_EDGE('',*,*,#41726,.T.) ;
#56739=ORIENTED_EDGE('',*,*,#39767,.F.) ;
#56740=ORIENTED_EDGE('',*,*,#39259,.F.) ;
#56741=ORIENTED_EDGE('',*,*,#40783,.F.) ;
#56742=ORIENTED_EDGE('',*,*,#41727,.T.) ;
#56743=ORIENTED_EDGE('',*,*,#40807,.F.) ;
#56744=ORIENTED_EDGE('',*,*,#41728,.F.) ;
#56745=ORIENTED_EDGE('',*,*,#39773,.F.) ;
#56746=ORIENTED_EDGE('',*,*,#41728,.T.) ;
#56747=ORIENTED_EDGE('',*,*,#40810,.F.) ;
#56748=ORIENTED_EDGE('',*,*,#41729,.F.) ;
#56749=ORIENTED_EDGE('',*,*,#39774,.F.) ;
#56750=ORIENTED_EDGE('',*,*,#39257,.T.) ;
#56751=ORIENTED_EDGE('',*,*,#39766,.F.) ;
#56752=ORIENTED_EDGE('',*,*,#41730,.F.) ;
#56753=ORIENTED_EDGE('',*,*,#40780,.F.) ;
#56754=ORIENTED_EDGE('',*,*,#41729,.T.) ;
#56755=ORIENTED_EDGE('',*,*,#40813,.F.) ;
#56756=ORIENTED_EDGE('',*,*,#41731,.F.) ;
#56757=ORIENTED_EDGE('',*,*,#39775,.F.) ;
#56758=ORIENTED_EDGE('',*,*,#41730,.T.) ;
#56759=ORIENTED_EDGE('',*,*,#39765,.F.) ;
#56760=ORIENTED_EDGE('',*,*,#41732,.F.) ;
#56761=ORIENTED_EDGE('',*,*,#40778,.F.) ;
#56762=ORIENTED_EDGE('',*,*,#41731,.T.) ;
#56763=ORIENTED_EDGE('',*,*,#40816,.F.) ;
#56764=ORIENTED_EDGE('',*,*,#41733,.F.) ;
#56765=ORIENTED_EDGE('',*,*,#39776,.F.) ;
#56766=ORIENTED_EDGE('',*,*,#41732,.T.) ;
#56767=ORIENTED_EDGE('',*,*,#39764,.F.) ;
#56768=ORIENTED_EDGE('',*,*,#41734,.F.) ;
#56769=ORIENTED_EDGE('',*,*,#40776,.F.) ;
#56770=ORIENTED_EDGE('',*,*,#41733,.T.) ;
#56771=ORIENTED_EDGE('',*,*,#40819,.F.) ;
#56772=ORIENTED_EDGE('',*,*,#41735,.F.) ;
#56773=ORIENTED_EDGE('',*,*,#39777,.F.) ;
#56774=ORIENTED_EDGE('',*,*,#41734,.T.) ;
#56775=ORIENTED_EDGE('',*,*,#39763,.F.) ;
#56776=ORIENTED_EDGE('',*,*,#41736,.F.) ;
#56777=ORIENTED_EDGE('',*,*,#40773,.F.) ;
#56778=ORIENTED_EDGE('',*,*,#41735,.T.) ;
#56779=ORIENTED_EDGE('',*,*,#40822,.F.) ;
#56780=ORIENTED_EDGE('',*,*,#41737,.F.) ;
#56781=ORIENTED_EDGE('',*,*,#39778,.F.) ;
#56782=ORIENTED_EDGE('',*,*,#41736,.T.) ;
#56783=ORIENTED_EDGE('',*,*,#39762,.F.) ;
#56784=ORIENTED_EDGE('',*,*,#41738,.F.) ;
#56785=ORIENTED_EDGE('',*,*,#40770,.F.) ;
#56786=ORIENTED_EDGE('',*,*,#41737,.T.) ;
#56787=ORIENTED_EDGE('',*,*,#40825,.F.) ;
#56788=ORIENTED_EDGE('',*,*,#41739,.F.) ;
#56789=ORIENTED_EDGE('',*,*,#39779,.F.) ;
#56790=ORIENTED_EDGE('',*,*,#40767,.F.) ;
#56791=ORIENTED_EDGE('',*,*,#41738,.T.) ;
#56792=ORIENTED_EDGE('',*,*,#41740,.F.) ;
#56793=ORIENTED_EDGE('',*,*,#41739,.T.) ;
#56794=ORIENTED_EDGE('',*,*,#40828,.F.) ;
#56795=ORIENTED_EDGE('',*,*,#41741,.F.) ;
#56796=ORIENTED_EDGE('',*,*,#39780,.F.) ;
#56797=ORIENTED_EDGE('',*,*,#41740,.T.) ;
#56798=ORIENTED_EDGE('',*,*,#39761,.F.) ;
#56799=ORIENTED_EDGE('',*,*,#41742,.F.) ;
#56800=ORIENTED_EDGE('',*,*,#40764,.F.) ;
#56801=ORIENTED_EDGE('',*,*,#41741,.T.) ;
#56802=ORIENTED_EDGE('',*,*,#40831,.F.) ;
#56803=ORIENTED_EDGE('',*,*,#41743,.F.) ;
#56804=ORIENTED_EDGE('',*,*,#39781,.F.) ;
#56805=ORIENTED_EDGE('',*,*,#40761,.F.) ;
#56806=ORIENTED_EDGE('',*,*,#41742,.T.) ;
#56807=ORIENTED_EDGE('',*,*,#41744,.F.) ;
#56808=ORIENTED_EDGE('',*,*,#41743,.T.) ;
#56809=ORIENTED_EDGE('',*,*,#40834,.F.) ;
#56810=ORIENTED_EDGE('',*,*,#41745,.F.) ;
#56811=ORIENTED_EDGE('',*,*,#39759,.F.) ;
#56812=ORIENTED_EDGE('',*,*,#41744,.T.) ;
#56813=ORIENTED_EDGE('',*,*,#39760,.F.) ;
#56814=ORIENTED_EDGE('',*,*,#41745,.T.) ;
#56815=ORIENTED_EDGE('',*,*,#40836,.F.) ;
#56816=ORIENTED_EDGE('',*,*,#41746,.F.) ;
#56817=ORIENTED_EDGE('',*,*,#40892,.F.) ;
#56818=ORIENTED_EDGE('',*,*,#41747,.F.) ;
#56819=ORIENTED_EDGE('',*,*,#39793,.F.) ;
#56820=ORIENTED_EDGE('',*,*,#40889,.F.) ;
#56821=ORIENTED_EDGE('',*,*,#41746,.T.) ;
#56822=ORIENTED_EDGE('',*,*,#41748,.F.) ;
#56823=ORIENTED_EDGE('',*,*,#41747,.T.) ;
#56824=ORIENTED_EDGE('',*,*,#40895,.F.) ;
#56825=ORIENTED_EDGE('',*,*,#41749,.F.) ;
#56826=ORIENTED_EDGE('',*,*,#41748,.T.) ;
#56827=ORIENTED_EDGE('',*,*,#39792,.F.) ;
#56828=ORIENTED_EDGE('',*,*,#41750,.F.) ;
#56829=ORIENTED_EDGE('',*,*,#40886,.F.) ;
#56830=ORIENTED_EDGE('',*,*,#41749,.T.) ;
#56831=ORIENTED_EDGE('',*,*,#40898,.F.) ;
#56832=ORIENTED_EDGE('',*,*,#41751,.F.) ;
#56833=ORIENTED_EDGE('',*,*,#39794,.F.) ;
#56834=ORIENTED_EDGE('',*,*,#41750,.T.) ;
#56835=ORIENTED_EDGE('',*,*,#39791,.F.) ;
#56836=ORIENTED_EDGE('',*,*,#41752,.F.) ;
#56837=ORIENTED_EDGE('',*,*,#40883,.F.) ;
#56838=ORIENTED_EDGE('',*,*,#41751,.T.) ;
#56839=ORIENTED_EDGE('',*,*,#40901,.F.) ;
#56840=ORIENTED_EDGE('',*,*,#41753,.F.) ;
#56841=ORIENTED_EDGE('',*,*,#39795,.F.) ;
#56842=ORIENTED_EDGE('',*,*,#41752,.T.) ;
#56843=ORIENTED_EDGE('',*,*,#39790,.F.) ;
#56844=ORIENTED_EDGE('',*,*,#39255,.F.) ;
#56845=ORIENTED_EDGE('',*,*,#40880,.F.) ;
#56846=ORIENTED_EDGE('',*,*,#41753,.T.) ;
#56847=ORIENTED_EDGE('',*,*,#40904,.F.) ;
#56848=ORIENTED_EDGE('',*,*,#41754,.F.) ;
#56849=ORIENTED_EDGE('',*,*,#39796,.F.) ;
#56850=ORIENTED_EDGE('',*,*,#41754,.T.) ;
#56851=ORIENTED_EDGE('',*,*,#40907,.F.) ;
#56852=ORIENTED_EDGE('',*,*,#41755,.F.) ;
#56853=ORIENTED_EDGE('',*,*,#39797,.F.) ;
#56854=ORIENTED_EDGE('',*,*,#39253,.T.) ;
#56855=ORIENTED_EDGE('',*,*,#39789,.F.) ;
#56856=ORIENTED_EDGE('',*,*,#41756,.F.) ;
#56857=ORIENTED_EDGE('',*,*,#40877,.F.) ;
#56858=ORIENTED_EDGE('',*,*,#41755,.T.) ;
#56859=ORIENTED_EDGE('',*,*,#40910,.F.) ;
#56860=ORIENTED_EDGE('',*,*,#41757,.F.) ;
#56861=ORIENTED_EDGE('',*,*,#39798,.F.) ;
#56862=ORIENTED_EDGE('',*,*,#41756,.T.) ;
#56863=ORIENTED_EDGE('',*,*,#39788,.F.) ;
#56864=ORIENTED_EDGE('',*,*,#41758,.F.) ;
#56865=ORIENTED_EDGE('',*,*,#40875,.F.) ;
#56866=ORIENTED_EDGE('',*,*,#41757,.T.) ;
#56867=ORIENTED_EDGE('',*,*,#40913,.F.) ;
#56868=ORIENTED_EDGE('',*,*,#41759,.F.) ;
#56869=ORIENTED_EDGE('',*,*,#39799,.F.) ;
#56870=ORIENTED_EDGE('',*,*,#41758,.T.) ;
#56871=ORIENTED_EDGE('',*,*,#39787,.F.) ;
#56872=ORIENTED_EDGE('',*,*,#41760,.F.) ;
#56873=ORIENTED_EDGE('',*,*,#40873,.F.) ;
#56874=ORIENTED_EDGE('',*,*,#41759,.T.) ;
#56875=ORIENTED_EDGE('',*,*,#40916,.F.) ;
#56876=ORIENTED_EDGE('',*,*,#41761,.F.) ;
#56877=ORIENTED_EDGE('',*,*,#39800,.F.) ;
#56878=ORIENTED_EDGE('',*,*,#41760,.T.) ;
#56879=ORIENTED_EDGE('',*,*,#39786,.F.) ;
#56880=ORIENTED_EDGE('',*,*,#41762,.F.) ;
#56881=ORIENTED_EDGE('',*,*,#40870,.F.) ;
#56882=ORIENTED_EDGE('',*,*,#41761,.T.) ;
#56883=ORIENTED_EDGE('',*,*,#40919,.F.) ;
#56884=ORIENTED_EDGE('',*,*,#41763,.F.) ;
#56885=ORIENTED_EDGE('',*,*,#39801,.F.) ;
#56886=ORIENTED_EDGE('',*,*,#41762,.T.) ;
#56887=ORIENTED_EDGE('',*,*,#39785,.F.) ;
#56888=ORIENTED_EDGE('',*,*,#41764,.F.) ;
#56889=ORIENTED_EDGE('',*,*,#40867,.F.) ;
#56890=ORIENTED_EDGE('',*,*,#41763,.T.) ;
#56891=ORIENTED_EDGE('',*,*,#40922,.F.) ;
#56892=ORIENTED_EDGE('',*,*,#41765,.F.) ;
#56893=ORIENTED_EDGE('',*,*,#39802,.F.) ;
#56894=ORIENTED_EDGE('',*,*,#40864,.F.) ;
#56895=ORIENTED_EDGE('',*,*,#41764,.T.) ;
#56896=ORIENTED_EDGE('',*,*,#41766,.F.) ;
#56897=ORIENTED_EDGE('',*,*,#41765,.T.) ;
#56898=ORIENTED_EDGE('',*,*,#40925,.F.) ;
#56899=ORIENTED_EDGE('',*,*,#41767,.F.) ;
#56900=ORIENTED_EDGE('',*,*,#39803,.F.) ;
#56901=ORIENTED_EDGE('',*,*,#41766,.T.) ;
#56902=ORIENTED_EDGE('',*,*,#39784,.F.) ;
#56903=ORIENTED_EDGE('',*,*,#41768,.F.) ;
#56904=ORIENTED_EDGE('',*,*,#40861,.F.) ;
#56905=ORIENTED_EDGE('',*,*,#41767,.T.) ;
#56906=ORIENTED_EDGE('',*,*,#40928,.F.) ;
#56907=ORIENTED_EDGE('',*,*,#41769,.F.) ;
#56908=ORIENTED_EDGE('',*,*,#39804,.F.) ;
#56909=ORIENTED_EDGE('',*,*,#40858,.F.) ;
#56910=ORIENTED_EDGE('',*,*,#41768,.T.) ;
#56911=ORIENTED_EDGE('',*,*,#41770,.F.) ;
#56912=ORIENTED_EDGE('',*,*,#41769,.T.) ;
#56913=ORIENTED_EDGE('',*,*,#40931,.F.) ;
#56914=ORIENTED_EDGE('',*,*,#41771,.F.) ;
#56915=ORIENTED_EDGE('',*,*,#39782,.F.) ;
#56916=ORIENTED_EDGE('',*,*,#41770,.T.) ;
#56917=ORIENTED_EDGE('',*,*,#39783,.F.) ;
#56918=ORIENTED_EDGE('',*,*,#41771,.T.) ;
#56919=ORIENTED_EDGE('',*,*,#40933,.F.) ;
#56920=ORIENTED_EDGE('',*,*,#41772,.F.) ;
#56921=ORIENTED_EDGE('',*,*,#40989,.F.) ;
#56922=ORIENTED_EDGE('',*,*,#41773,.F.) ;
#56923=ORIENTED_EDGE('',*,*,#39816,.F.) ;
#56924=ORIENTED_EDGE('',*,*,#40986,.F.) ;
#56925=ORIENTED_EDGE('',*,*,#41772,.T.) ;
#56926=ORIENTED_EDGE('',*,*,#41774,.F.) ;
#56927=ORIENTED_EDGE('',*,*,#41773,.T.) ;
#56928=ORIENTED_EDGE('',*,*,#40992,.F.) ;
#56929=ORIENTED_EDGE('',*,*,#41775,.F.) ;
#56930=ORIENTED_EDGE('',*,*,#41774,.T.) ;
#56931=ORIENTED_EDGE('',*,*,#39815,.F.) ;
#56932=ORIENTED_EDGE('',*,*,#41776,.F.) ;
#56933=ORIENTED_EDGE('',*,*,#40983,.F.) ;
#56934=ORIENTED_EDGE('',*,*,#41775,.T.) ;
#56935=ORIENTED_EDGE('',*,*,#40995,.F.) ;
#56936=ORIENTED_EDGE('',*,*,#41777,.F.) ;
#56937=ORIENTED_EDGE('',*,*,#39817,.F.) ;
#56938=ORIENTED_EDGE('',*,*,#41776,.T.) ;
#56939=ORIENTED_EDGE('',*,*,#39814,.F.) ;
#56940=ORIENTED_EDGE('',*,*,#41778,.F.) ;
#56941=ORIENTED_EDGE('',*,*,#40980,.F.) ;
#56942=ORIENTED_EDGE('',*,*,#41777,.T.) ;
#56943=ORIENTED_EDGE('',*,*,#40998,.F.) ;
#56944=ORIENTED_EDGE('',*,*,#41779,.F.) ;
#56945=ORIENTED_EDGE('',*,*,#39818,.F.) ;
#56946=ORIENTED_EDGE('',*,*,#41778,.T.) ;
#56947=ORIENTED_EDGE('',*,*,#39813,.F.) ;
#56948=ORIENTED_EDGE('',*,*,#39251,.F.) ;
#56949=ORIENTED_EDGE('',*,*,#40977,.F.) ;
#56950=ORIENTED_EDGE('',*,*,#41779,.T.) ;
#56951=ORIENTED_EDGE('',*,*,#41001,.F.) ;
#56952=ORIENTED_EDGE('',*,*,#41780,.F.) ;
#56953=ORIENTED_EDGE('',*,*,#39819,.F.) ;
#56954=ORIENTED_EDGE('',*,*,#41780,.T.) ;
#56955=ORIENTED_EDGE('',*,*,#41004,.F.) ;
#56956=ORIENTED_EDGE('',*,*,#41781,.F.) ;
#56957=ORIENTED_EDGE('',*,*,#39820,.F.) ;
#56958=ORIENTED_EDGE('',*,*,#39249,.T.) ;
#56959=ORIENTED_EDGE('',*,*,#39812,.F.) ;
#56960=ORIENTED_EDGE('',*,*,#41782,.F.) ;
#56961=ORIENTED_EDGE('',*,*,#40974,.F.) ;
#56962=ORIENTED_EDGE('',*,*,#41781,.T.) ;
#56963=ORIENTED_EDGE('',*,*,#41007,.F.) ;
#56964=ORIENTED_EDGE('',*,*,#41783,.F.) ;
#56965=ORIENTED_EDGE('',*,*,#39821,.F.) ;
#56966=ORIENTED_EDGE('',*,*,#41782,.T.) ;
#56967=ORIENTED_EDGE('',*,*,#39811,.F.) ;
#56968=ORIENTED_EDGE('',*,*,#41784,.F.) ;
#56969=ORIENTED_EDGE('',*,*,#40972,.F.) ;
#56970=ORIENTED_EDGE('',*,*,#41783,.T.) ;
#56971=ORIENTED_EDGE('',*,*,#41010,.F.) ;
#56972=ORIENTED_EDGE('',*,*,#41785,.F.) ;
#56973=ORIENTED_EDGE('',*,*,#39822,.F.) ;
#56974=ORIENTED_EDGE('',*,*,#41784,.T.) ;
#56975=ORIENTED_EDGE('',*,*,#39810,.F.) ;
#56976=ORIENTED_EDGE('',*,*,#41786,.F.) ;
#56977=ORIENTED_EDGE('',*,*,#40970,.F.) ;
#56978=ORIENTED_EDGE('',*,*,#41785,.T.) ;
#56979=ORIENTED_EDGE('',*,*,#41013,.F.) ;
#56980=ORIENTED_EDGE('',*,*,#41787,.F.) ;
#56981=ORIENTED_EDGE('',*,*,#39823,.F.) ;
#56982=ORIENTED_EDGE('',*,*,#41786,.T.) ;
#56983=ORIENTED_EDGE('',*,*,#39809,.F.) ;
#56984=ORIENTED_EDGE('',*,*,#41788,.F.) ;
#56985=ORIENTED_EDGE('',*,*,#40967,.F.) ;
#56986=ORIENTED_EDGE('',*,*,#41787,.T.) ;
#56987=ORIENTED_EDGE('',*,*,#41016,.F.) ;
#56988=ORIENTED_EDGE('',*,*,#41789,.F.) ;
#56989=ORIENTED_EDGE('',*,*,#39824,.F.) ;
#56990=ORIENTED_EDGE('',*,*,#41788,.T.) ;
#56991=ORIENTED_EDGE('',*,*,#39808,.F.) ;
#56992=ORIENTED_EDGE('',*,*,#41790,.F.) ;
#56993=ORIENTED_EDGE('',*,*,#40964,.F.) ;
#56994=ORIENTED_EDGE('',*,*,#41789,.T.) ;
#56995=ORIENTED_EDGE('',*,*,#41019,.F.) ;
#56996=ORIENTED_EDGE('',*,*,#41791,.F.) ;
#56997=ORIENTED_EDGE('',*,*,#39825,.F.) ;
#56998=ORIENTED_EDGE('',*,*,#40961,.F.) ;
#56999=ORIENTED_EDGE('',*,*,#41790,.T.) ;
#57000=ORIENTED_EDGE('',*,*,#41792,.F.) ;
#57001=ORIENTED_EDGE('',*,*,#41791,.T.) ;
#57002=ORIENTED_EDGE('',*,*,#41022,.F.) ;
#57003=ORIENTED_EDGE('',*,*,#41793,.F.) ;
#57004=ORIENTED_EDGE('',*,*,#39826,.F.) ;
#57005=ORIENTED_EDGE('',*,*,#41792,.T.) ;
#57006=ORIENTED_EDGE('',*,*,#39807,.F.) ;
#57007=ORIENTED_EDGE('',*,*,#41794,.F.) ;
#57008=ORIENTED_EDGE('',*,*,#40958,.F.) ;
#57009=ORIENTED_EDGE('',*,*,#41793,.T.) ;
#57010=ORIENTED_EDGE('',*,*,#41025,.F.) ;
#57011=ORIENTED_EDGE('',*,*,#41795,.F.) ;
#57012=ORIENTED_EDGE('',*,*,#39827,.F.) ;
#57013=ORIENTED_EDGE('',*,*,#40955,.F.) ;
#57014=ORIENTED_EDGE('',*,*,#41794,.T.) ;
#57015=ORIENTED_EDGE('',*,*,#41796,.F.) ;
#57016=ORIENTED_EDGE('',*,*,#41795,.T.) ;
#57017=ORIENTED_EDGE('',*,*,#41028,.F.) ;
#57018=ORIENTED_EDGE('',*,*,#41797,.F.) ;
#57019=ORIENTED_EDGE('',*,*,#39805,.F.) ;
#57020=ORIENTED_EDGE('',*,*,#41796,.T.) ;
#57021=ORIENTED_EDGE('',*,*,#39806,.F.) ;
#57022=ORIENTED_EDGE('',*,*,#41797,.T.) ;
#57023=ORIENTED_EDGE('',*,*,#41030,.F.) ;
#57024=ORIENTED_EDGE('',*,*,#41798,.F.) ;
#57025=ORIENTED_EDGE('',*,*,#41086,.F.) ;
#57026=ORIENTED_EDGE('',*,*,#41799,.F.) ;
#57027=ORIENTED_EDGE('',*,*,#39839,.F.) ;
#57028=ORIENTED_EDGE('',*,*,#41083,.F.) ;
#57029=ORIENTED_EDGE('',*,*,#41798,.T.) ;
#57030=ORIENTED_EDGE('',*,*,#41800,.F.) ;
#57031=ORIENTED_EDGE('',*,*,#41799,.T.) ;
#57032=ORIENTED_EDGE('',*,*,#41089,.F.) ;
#57033=ORIENTED_EDGE('',*,*,#41801,.F.) ;
#57034=ORIENTED_EDGE('',*,*,#41800,.T.) ;
#57035=ORIENTED_EDGE('',*,*,#39838,.F.) ;
#57036=ORIENTED_EDGE('',*,*,#41802,.F.) ;
#57037=ORIENTED_EDGE('',*,*,#41080,.F.) ;
#57038=ORIENTED_EDGE('',*,*,#41801,.T.) ;
#57039=ORIENTED_EDGE('',*,*,#41092,.F.) ;
#57040=ORIENTED_EDGE('',*,*,#41803,.F.) ;
#57041=ORIENTED_EDGE('',*,*,#39840,.F.) ;
#57042=ORIENTED_EDGE('',*,*,#41802,.T.) ;
#57043=ORIENTED_EDGE('',*,*,#39837,.F.) ;
#57044=ORIENTED_EDGE('',*,*,#41804,.F.) ;
#57045=ORIENTED_EDGE('',*,*,#41077,.F.) ;
#57046=ORIENTED_EDGE('',*,*,#41803,.T.) ;
#57047=ORIENTED_EDGE('',*,*,#41095,.F.) ;
#57048=ORIENTED_EDGE('',*,*,#41805,.F.) ;
#57049=ORIENTED_EDGE('',*,*,#39841,.F.) ;
#57050=ORIENTED_EDGE('',*,*,#41804,.T.) ;
#57051=ORIENTED_EDGE('',*,*,#39836,.F.) ;
#57052=ORIENTED_EDGE('',*,*,#39247,.F.) ;
#57053=ORIENTED_EDGE('',*,*,#41074,.F.) ;
#57054=ORIENTED_EDGE('',*,*,#41805,.T.) ;
#57055=ORIENTED_EDGE('',*,*,#41098,.F.) ;
#57056=ORIENTED_EDGE('',*,*,#41806,.F.) ;
#57057=ORIENTED_EDGE('',*,*,#39842,.F.) ;
#57058=ORIENTED_EDGE('',*,*,#41806,.T.) ;
#57059=ORIENTED_EDGE('',*,*,#41101,.F.) ;
#57060=ORIENTED_EDGE('',*,*,#41807,.F.) ;
#57061=ORIENTED_EDGE('',*,*,#39843,.F.) ;
#57062=ORIENTED_EDGE('',*,*,#39245,.T.) ;
#57063=ORIENTED_EDGE('',*,*,#39835,.F.) ;
#57064=ORIENTED_EDGE('',*,*,#41808,.F.) ;
#57065=ORIENTED_EDGE('',*,*,#41071,.F.) ;
#57066=ORIENTED_EDGE('',*,*,#41807,.T.) ;
#57067=ORIENTED_EDGE('',*,*,#41104,.F.) ;
#57068=ORIENTED_EDGE('',*,*,#41809,.F.) ;
#57069=ORIENTED_EDGE('',*,*,#39844,.F.) ;
#57070=ORIENTED_EDGE('',*,*,#41808,.T.) ;
#57071=ORIENTED_EDGE('',*,*,#39834,.F.) ;
#57072=ORIENTED_EDGE('',*,*,#41810,.F.) ;
#57073=ORIENTED_EDGE('',*,*,#41069,.F.) ;
#57074=ORIENTED_EDGE('',*,*,#41809,.T.) ;
#57075=ORIENTED_EDGE('',*,*,#41107,.F.) ;
#57076=ORIENTED_EDGE('',*,*,#41811,.F.) ;
#57077=ORIENTED_EDGE('',*,*,#39845,.F.) ;
#57078=ORIENTED_EDGE('',*,*,#41810,.T.) ;
#57079=ORIENTED_EDGE('',*,*,#39833,.F.) ;
#57080=ORIENTED_EDGE('',*,*,#41812,.F.) ;
#57081=ORIENTED_EDGE('',*,*,#41067,.F.) ;
#57082=ORIENTED_EDGE('',*,*,#41811,.T.) ;
#57083=ORIENTED_EDGE('',*,*,#41110,.F.) ;
#57084=ORIENTED_EDGE('',*,*,#41813,.F.) ;
#57085=ORIENTED_EDGE('',*,*,#39846,.F.) ;
#57086=ORIENTED_EDGE('',*,*,#41812,.T.) ;
#57087=ORIENTED_EDGE('',*,*,#39832,.F.) ;
#57088=ORIENTED_EDGE('',*,*,#41814,.F.) ;
#57089=ORIENTED_EDGE('',*,*,#41064,.F.) ;
#57090=ORIENTED_EDGE('',*,*,#41813,.T.) ;
#57091=ORIENTED_EDGE('',*,*,#41113,.F.) ;
#57092=ORIENTED_EDGE('',*,*,#41815,.F.) ;
#57093=ORIENTED_EDGE('',*,*,#39847,.F.) ;
#57094=ORIENTED_EDGE('',*,*,#41814,.T.) ;
#57095=ORIENTED_EDGE('',*,*,#39831,.F.) ;
#57096=ORIENTED_EDGE('',*,*,#41816,.F.) ;
#57097=ORIENTED_EDGE('',*,*,#41061,.F.) ;
#57098=ORIENTED_EDGE('',*,*,#41815,.T.) ;
#57099=ORIENTED_EDGE('',*,*,#41116,.F.) ;
#57100=ORIENTED_EDGE('',*,*,#41817,.F.) ;
#57101=ORIENTED_EDGE('',*,*,#39848,.F.) ;
#57102=ORIENTED_EDGE('',*,*,#41058,.F.) ;
#57103=ORIENTED_EDGE('',*,*,#41816,.T.) ;
#57104=ORIENTED_EDGE('',*,*,#41818,.F.) ;
#57105=ORIENTED_EDGE('',*,*,#41817,.T.) ;
#57106=ORIENTED_EDGE('',*,*,#41119,.F.) ;
#57107=ORIENTED_EDGE('',*,*,#41819,.F.) ;
#57108=ORIENTED_EDGE('',*,*,#39849,.F.) ;
#57109=ORIENTED_EDGE('',*,*,#41818,.T.) ;
#57110=ORIENTED_EDGE('',*,*,#39830,.F.) ;
#57111=ORIENTED_EDGE('',*,*,#41820,.F.) ;
#57112=ORIENTED_EDGE('',*,*,#41055,.F.) ;
#57113=ORIENTED_EDGE('',*,*,#41819,.T.) ;
#57114=ORIENTED_EDGE('',*,*,#41122,.F.) ;
#57115=ORIENTED_EDGE('',*,*,#41821,.F.) ;
#57116=ORIENTED_EDGE('',*,*,#39850,.F.) ;
#57117=ORIENTED_EDGE('',*,*,#41052,.F.) ;
#57118=ORIENTED_EDGE('',*,*,#41820,.T.) ;
#57119=ORIENTED_EDGE('',*,*,#41822,.F.) ;
#57120=ORIENTED_EDGE('',*,*,#41821,.T.) ;
#57121=ORIENTED_EDGE('',*,*,#41125,.F.) ;
#57122=ORIENTED_EDGE('',*,*,#41823,.F.) ;
#57123=ORIENTED_EDGE('',*,*,#39828,.F.) ;
#57124=ORIENTED_EDGE('',*,*,#41822,.T.) ;
#57125=ORIENTED_EDGE('',*,*,#39829,.F.) ;
#57126=ORIENTED_EDGE('',*,*,#41823,.T.) ;
#57127=ORIENTED_EDGE('',*,*,#41127,.F.) ;
#57128=ORIENTED_EDGE('',*,*,#41824,.F.) ;
#57129=ORIENTED_EDGE('',*,*,#41183,.F.) ;
#57130=ORIENTED_EDGE('',*,*,#41825,.F.) ;
#57131=ORIENTED_EDGE('',*,*,#39862,.F.) ;
#57132=ORIENTED_EDGE('',*,*,#41180,.F.) ;
#57133=ORIENTED_EDGE('',*,*,#41824,.T.) ;
#57134=ORIENTED_EDGE('',*,*,#41826,.F.) ;
#57135=ORIENTED_EDGE('',*,*,#41825,.T.) ;
#57136=ORIENTED_EDGE('',*,*,#41186,.F.) ;
#57137=ORIENTED_EDGE('',*,*,#41827,.F.) ;
#57138=ORIENTED_EDGE('',*,*,#41826,.T.) ;
#57139=ORIENTED_EDGE('',*,*,#39861,.F.) ;
#57140=ORIENTED_EDGE('',*,*,#41828,.F.) ;
#57141=ORIENTED_EDGE('',*,*,#41177,.F.) ;
#57142=ORIENTED_EDGE('',*,*,#41827,.T.) ;
#57143=ORIENTED_EDGE('',*,*,#41189,.F.) ;
#57144=ORIENTED_EDGE('',*,*,#41829,.F.) ;
#57145=ORIENTED_EDGE('',*,*,#39863,.F.) ;
#57146=ORIENTED_EDGE('',*,*,#41828,.T.) ;
#57147=ORIENTED_EDGE('',*,*,#39860,.F.) ;
#57148=ORIENTED_EDGE('',*,*,#41830,.F.) ;
#57149=ORIENTED_EDGE('',*,*,#41174,.F.) ;
#57150=ORIENTED_EDGE('',*,*,#41829,.T.) ;
#57151=ORIENTED_EDGE('',*,*,#41192,.F.) ;
#57152=ORIENTED_EDGE('',*,*,#41831,.F.) ;
#57153=ORIENTED_EDGE('',*,*,#39864,.F.) ;
#57154=ORIENTED_EDGE('',*,*,#41830,.T.) ;
#57155=ORIENTED_EDGE('',*,*,#39859,.F.) ;
#57156=ORIENTED_EDGE('',*,*,#39243,.F.) ;
#57157=ORIENTED_EDGE('',*,*,#41171,.F.) ;
#57158=ORIENTED_EDGE('',*,*,#41831,.T.) ;
#57159=ORIENTED_EDGE('',*,*,#41195,.F.) ;
#57160=ORIENTED_EDGE('',*,*,#41832,.F.) ;
#57161=ORIENTED_EDGE('',*,*,#39865,.F.) ;
#57162=ORIENTED_EDGE('',*,*,#41832,.T.) ;
#57163=ORIENTED_EDGE('',*,*,#41198,.F.) ;
#57164=ORIENTED_EDGE('',*,*,#41833,.F.) ;
#57165=ORIENTED_EDGE('',*,*,#39866,.F.) ;
#57166=ORIENTED_EDGE('',*,*,#39241,.T.) ;
#57167=ORIENTED_EDGE('',*,*,#39858,.F.) ;
#57168=ORIENTED_EDGE('',*,*,#41834,.F.) ;
#57169=ORIENTED_EDGE('',*,*,#41168,.F.) ;
#57170=ORIENTED_EDGE('',*,*,#41833,.T.) ;
#57171=ORIENTED_EDGE('',*,*,#41201,.F.) ;
#57172=ORIENTED_EDGE('',*,*,#41835,.F.) ;
#57173=ORIENTED_EDGE('',*,*,#39867,.F.) ;
#57174=ORIENTED_EDGE('',*,*,#41834,.T.) ;
#57175=ORIENTED_EDGE('',*,*,#39857,.F.) ;
#57176=ORIENTED_EDGE('',*,*,#41836,.F.) ;
#57177=ORIENTED_EDGE('',*,*,#41166,.F.) ;
#57178=ORIENTED_EDGE('',*,*,#41835,.T.) ;
#57179=ORIENTED_EDGE('',*,*,#41204,.F.) ;
#57180=ORIENTED_EDGE('',*,*,#41837,.F.) ;
#57181=ORIENTED_EDGE('',*,*,#39868,.F.) ;
#57182=ORIENTED_EDGE('',*,*,#41836,.T.) ;
#57183=ORIENTED_EDGE('',*,*,#39856,.F.) ;
#57184=ORIENTED_EDGE('',*,*,#41838,.F.) ;
#57185=ORIENTED_EDGE('',*,*,#41164,.F.) ;
#57186=ORIENTED_EDGE('',*,*,#41837,.T.) ;
#57187=ORIENTED_EDGE('',*,*,#41207,.F.) ;
#57188=ORIENTED_EDGE('',*,*,#41839,.F.) ;
#57189=ORIENTED_EDGE('',*,*,#39869,.F.) ;
#57190=ORIENTED_EDGE('',*,*,#41838,.T.) ;
#57191=ORIENTED_EDGE('',*,*,#39855,.F.) ;
#57192=ORIENTED_EDGE('',*,*,#41840,.F.) ;
#57193=ORIENTED_EDGE('',*,*,#41161,.F.) ;
#57194=ORIENTED_EDGE('',*,*,#41839,.T.) ;
#57195=ORIENTED_EDGE('',*,*,#41210,.F.) ;
#57196=ORIENTED_EDGE('',*,*,#41841,.F.) ;
#57197=ORIENTED_EDGE('',*,*,#39870,.F.) ;
#57198=ORIENTED_EDGE('',*,*,#41840,.T.) ;
#57199=ORIENTED_EDGE('',*,*,#39854,.F.) ;
#57200=ORIENTED_EDGE('',*,*,#41842,.F.) ;
#57201=ORIENTED_EDGE('',*,*,#41158,.F.) ;
#57202=ORIENTED_EDGE('',*,*,#41841,.T.) ;
#57203=ORIENTED_EDGE('',*,*,#41213,.F.) ;
#57204=ORIENTED_EDGE('',*,*,#41843,.F.) ;
#57205=ORIENTED_EDGE('',*,*,#39871,.F.) ;
#57206=ORIENTED_EDGE('',*,*,#41155,.F.) ;
#57207=ORIENTED_EDGE('',*,*,#41842,.T.) ;
#57208=ORIENTED_EDGE('',*,*,#41844,.F.) ;
#57209=ORIENTED_EDGE('',*,*,#41843,.T.) ;
#57210=ORIENTED_EDGE('',*,*,#41216,.F.) ;
#57211=ORIENTED_EDGE('',*,*,#41845,.F.) ;
#57212=ORIENTED_EDGE('',*,*,#39872,.F.) ;
#57213=ORIENTED_EDGE('',*,*,#41844,.T.) ;
#57214=ORIENTED_EDGE('',*,*,#39853,.F.) ;
#57215=ORIENTED_EDGE('',*,*,#41846,.F.) ;
#57216=ORIENTED_EDGE('',*,*,#41152,.F.) ;
#57217=ORIENTED_EDGE('',*,*,#41845,.T.) ;
#57218=ORIENTED_EDGE('',*,*,#41219,.F.) ;
#57219=ORIENTED_EDGE('',*,*,#41847,.F.) ;
#57220=ORIENTED_EDGE('',*,*,#39873,.F.) ;
#57221=ORIENTED_EDGE('',*,*,#41149,.F.) ;
#57222=ORIENTED_EDGE('',*,*,#41846,.T.) ;
#57223=ORIENTED_EDGE('',*,*,#41848,.F.) ;
#57224=ORIENTED_EDGE('',*,*,#41847,.T.) ;
#57225=ORIENTED_EDGE('',*,*,#41222,.F.) ;
#57226=ORIENTED_EDGE('',*,*,#41849,.F.) ;
#57227=ORIENTED_EDGE('',*,*,#39851,.F.) ;
#57228=ORIENTED_EDGE('',*,*,#41848,.T.) ;
#57229=ORIENTED_EDGE('',*,*,#39852,.F.) ;
#57230=ORIENTED_EDGE('',*,*,#41849,.T.) ;
#57231=ORIENTED_EDGE('',*,*,#41224,.F.) ;
#57232=ORIENTED_EDGE('',*,*,#41850,.F.) ;
#57233=ORIENTED_EDGE('',*,*,#41280,.F.) ;
#57234=ORIENTED_EDGE('',*,*,#41851,.F.) ;
#57235=ORIENTED_EDGE('',*,*,#39885,.F.) ;
#57236=ORIENTED_EDGE('',*,*,#41277,.F.) ;
#57237=ORIENTED_EDGE('',*,*,#41850,.T.) ;
#57238=ORIENTED_EDGE('',*,*,#41852,.F.) ;
#57239=ORIENTED_EDGE('',*,*,#41851,.T.) ;
#57240=ORIENTED_EDGE('',*,*,#41283,.F.) ;
#57241=ORIENTED_EDGE('',*,*,#41853,.F.) ;
#57242=ORIENTED_EDGE('',*,*,#41852,.T.) ;
#57243=ORIENTED_EDGE('',*,*,#39884,.F.) ;
#57244=ORIENTED_EDGE('',*,*,#41854,.F.) ;
#57245=ORIENTED_EDGE('',*,*,#41274,.F.) ;
#57246=ORIENTED_EDGE('',*,*,#41853,.T.) ;
#57247=ORIENTED_EDGE('',*,*,#41286,.F.) ;
#57248=ORIENTED_EDGE('',*,*,#41855,.F.) ;
#57249=ORIENTED_EDGE('',*,*,#39886,.F.) ;
#57250=ORIENTED_EDGE('',*,*,#41854,.T.) ;
#57251=ORIENTED_EDGE('',*,*,#39883,.F.) ;
#57252=ORIENTED_EDGE('',*,*,#41856,.F.) ;
#57253=ORIENTED_EDGE('',*,*,#41271,.F.) ;
#57254=ORIENTED_EDGE('',*,*,#41855,.T.) ;
#57255=ORIENTED_EDGE('',*,*,#41289,.F.) ;
#57256=ORIENTED_EDGE('',*,*,#41857,.F.) ;
#57257=ORIENTED_EDGE('',*,*,#39887,.F.) ;
#57258=ORIENTED_EDGE('',*,*,#41856,.T.) ;
#57259=ORIENTED_EDGE('',*,*,#39882,.F.) ;
#57260=ORIENTED_EDGE('',*,*,#39239,.F.) ;
#57261=ORIENTED_EDGE('',*,*,#41268,.F.) ;
#57262=ORIENTED_EDGE('',*,*,#41857,.T.) ;
#57263=ORIENTED_EDGE('',*,*,#41292,.F.) ;
#57264=ORIENTED_EDGE('',*,*,#41858,.F.) ;
#57265=ORIENTED_EDGE('',*,*,#39888,.F.) ;
#57266=ORIENTED_EDGE('',*,*,#41858,.T.) ;
#57267=ORIENTED_EDGE('',*,*,#41295,.F.) ;
#57268=ORIENTED_EDGE('',*,*,#41859,.F.) ;
#57269=ORIENTED_EDGE('',*,*,#39889,.F.) ;
#57270=ORIENTED_EDGE('',*,*,#39237,.T.) ;
#57271=ORIENTED_EDGE('',*,*,#39881,.F.) ;
#57272=ORIENTED_EDGE('',*,*,#41860,.F.) ;
#57273=ORIENTED_EDGE('',*,*,#41265,.F.) ;
#57274=ORIENTED_EDGE('',*,*,#41859,.T.) ;
#57275=ORIENTED_EDGE('',*,*,#41298,.F.) ;
#57276=ORIENTED_EDGE('',*,*,#41861,.F.) ;
#57277=ORIENTED_EDGE('',*,*,#39890,.F.) ;
#57278=ORIENTED_EDGE('',*,*,#41860,.T.) ;
#57279=ORIENTED_EDGE('',*,*,#39880,.F.) ;
#57280=ORIENTED_EDGE('',*,*,#41862,.F.) ;
#57281=ORIENTED_EDGE('',*,*,#41263,.F.) ;
#57282=ORIENTED_EDGE('',*,*,#41861,.T.) ;
#57283=ORIENTED_EDGE('',*,*,#41301,.F.) ;
#57284=ORIENTED_EDGE('',*,*,#41863,.F.) ;
#57285=ORIENTED_EDGE('',*,*,#39891,.F.) ;
#57286=ORIENTED_EDGE('',*,*,#41862,.T.) ;
#57287=ORIENTED_EDGE('',*,*,#39879,.F.) ;
#57288=ORIENTED_EDGE('',*,*,#41864,.F.) ;
#57289=ORIENTED_EDGE('',*,*,#41261,.F.) ;
#57290=ORIENTED_EDGE('',*,*,#41863,.T.) ;
#57291=ORIENTED_EDGE('',*,*,#41304,.F.) ;
#57292=ORIENTED_EDGE('',*,*,#41865,.F.) ;
#57293=ORIENTED_EDGE('',*,*,#39892,.F.) ;
#57294=ORIENTED_EDGE('',*,*,#41864,.T.) ;
#57295=ORIENTED_EDGE('',*,*,#39878,.F.) ;
#57296=ORIENTED_EDGE('',*,*,#41866,.F.) ;
#57297=ORIENTED_EDGE('',*,*,#41258,.F.) ;
#57298=ORIENTED_EDGE('',*,*,#41865,.T.) ;
#57299=ORIENTED_EDGE('',*,*,#41307,.F.) ;
#57300=ORIENTED_EDGE('',*,*,#41867,.F.) ;
#57301=ORIENTED_EDGE('',*,*,#39893,.F.) ;
#57302=ORIENTED_EDGE('',*,*,#41866,.T.) ;
#57303=ORIENTED_EDGE('',*,*,#39877,.F.) ;
#57304=ORIENTED_EDGE('',*,*,#41868,.F.) ;
#57305=ORIENTED_EDGE('',*,*,#41255,.F.) ;
#57306=ORIENTED_EDGE('',*,*,#41867,.T.) ;
#57307=ORIENTED_EDGE('',*,*,#41310,.F.) ;
#57308=ORIENTED_EDGE('',*,*,#41869,.F.) ;
#57309=ORIENTED_EDGE('',*,*,#39894,.F.) ;
#57310=ORIENTED_EDGE('',*,*,#41252,.F.) ;
#57311=ORIENTED_EDGE('',*,*,#41868,.T.) ;
#57312=ORIENTED_EDGE('',*,*,#41870,.F.) ;
#57313=ORIENTED_EDGE('',*,*,#41869,.T.) ;
#57314=ORIENTED_EDGE('',*,*,#41313,.F.) ;
#57315=ORIENTED_EDGE('',*,*,#41871,.F.) ;
#57316=ORIENTED_EDGE('',*,*,#39895,.F.) ;
#57317=ORIENTED_EDGE('',*,*,#41870,.T.) ;
#57318=ORIENTED_EDGE('',*,*,#39876,.F.) ;
#57319=ORIENTED_EDGE('',*,*,#41872,.F.) ;
#57320=ORIENTED_EDGE('',*,*,#41249,.F.) ;
#57321=ORIENTED_EDGE('',*,*,#41871,.T.) ;
#57322=ORIENTED_EDGE('',*,*,#41316,.F.) ;
#57323=ORIENTED_EDGE('',*,*,#41873,.F.) ;
#57324=ORIENTED_EDGE('',*,*,#39896,.F.) ;
#57325=ORIENTED_EDGE('',*,*,#41246,.F.) ;
#57326=ORIENTED_EDGE('',*,*,#41872,.T.) ;
#57327=ORIENTED_EDGE('',*,*,#41874,.F.) ;
#57328=ORIENTED_EDGE('',*,*,#41873,.T.) ;
#57329=ORIENTED_EDGE('',*,*,#41319,.F.) ;
#57330=ORIENTED_EDGE('',*,*,#41875,.F.) ;
#57331=ORIENTED_EDGE('',*,*,#39874,.F.) ;
#57332=ORIENTED_EDGE('',*,*,#41874,.T.) ;
#57333=ORIENTED_EDGE('',*,*,#39875,.F.) ;
#57334=ORIENTED_EDGE('',*,*,#41875,.T.) ;
#57335=ORIENTED_EDGE('',*,*,#41321,.F.) ;
#57336=ORIENTED_EDGE('',*,*,#41876,.F.) ;
#57337=ORIENTED_EDGE('',*,*,#41377,.F.) ;
#57338=ORIENTED_EDGE('',*,*,#41877,.F.) ;
#57339=ORIENTED_EDGE('',*,*,#39908,.F.) ;
#57340=ORIENTED_EDGE('',*,*,#41374,.F.) ;
#57341=ORIENTED_EDGE('',*,*,#41876,.T.) ;
#57342=ORIENTED_EDGE('',*,*,#41878,.F.) ;
#57343=ORIENTED_EDGE('',*,*,#41877,.T.) ;
#57344=ORIENTED_EDGE('',*,*,#41380,.F.) ;
#57345=ORIENTED_EDGE('',*,*,#41879,.F.) ;
#57346=ORIENTED_EDGE('',*,*,#41878,.T.) ;
#57347=ORIENTED_EDGE('',*,*,#39907,.F.) ;
#57348=ORIENTED_EDGE('',*,*,#41880,.F.) ;
#57349=ORIENTED_EDGE('',*,*,#41371,.F.) ;
#57350=ORIENTED_EDGE('',*,*,#41879,.T.) ;
#57351=ORIENTED_EDGE('',*,*,#41383,.F.) ;
#57352=ORIENTED_EDGE('',*,*,#41881,.F.) ;
#57353=ORIENTED_EDGE('',*,*,#39909,.F.) ;
#57354=ORIENTED_EDGE('',*,*,#41880,.T.) ;
#57355=ORIENTED_EDGE('',*,*,#39906,.F.) ;
#57356=ORIENTED_EDGE('',*,*,#41882,.F.) ;
#57357=ORIENTED_EDGE('',*,*,#41368,.F.) ;
#57358=ORIENTED_EDGE('',*,*,#41881,.T.) ;
#57359=ORIENTED_EDGE('',*,*,#41386,.F.) ;
#57360=ORIENTED_EDGE('',*,*,#41883,.F.) ;
#57361=ORIENTED_EDGE('',*,*,#39910,.F.) ;
#57362=ORIENTED_EDGE('',*,*,#41882,.T.) ;
#57363=ORIENTED_EDGE('',*,*,#39905,.F.) ;
#57364=ORIENTED_EDGE('',*,*,#39235,.F.) ;
#57365=ORIENTED_EDGE('',*,*,#41365,.F.) ;
#57366=ORIENTED_EDGE('',*,*,#41883,.T.) ;
#57367=ORIENTED_EDGE('',*,*,#41389,.F.) ;
#57368=ORIENTED_EDGE('',*,*,#41884,.F.) ;
#57369=ORIENTED_EDGE('',*,*,#39911,.F.) ;
#57370=ORIENTED_EDGE('',*,*,#41884,.T.) ;
#57371=ORIENTED_EDGE('',*,*,#41392,.F.) ;
#57372=ORIENTED_EDGE('',*,*,#41885,.F.) ;
#57373=ORIENTED_EDGE('',*,*,#39912,.F.) ;
#57374=ORIENTED_EDGE('',*,*,#39233,.T.) ;
#57375=ORIENTED_EDGE('',*,*,#39904,.F.) ;
#57376=ORIENTED_EDGE('',*,*,#41886,.F.) ;
#57377=ORIENTED_EDGE('',*,*,#41362,.F.) ;
#57378=ORIENTED_EDGE('',*,*,#41885,.T.) ;
#57379=ORIENTED_EDGE('',*,*,#41395,.F.) ;
#57380=ORIENTED_EDGE('',*,*,#41887,.F.) ;
#57381=ORIENTED_EDGE('',*,*,#39913,.F.) ;
#57382=ORIENTED_EDGE('',*,*,#41886,.T.) ;
#57383=ORIENTED_EDGE('',*,*,#39903,.F.) ;
#57384=ORIENTED_EDGE('',*,*,#41888,.F.) ;
#57385=ORIENTED_EDGE('',*,*,#41360,.F.) ;
#57386=ORIENTED_EDGE('',*,*,#41887,.T.) ;
#57387=ORIENTED_EDGE('',*,*,#41398,.F.) ;
#57388=ORIENTED_EDGE('',*,*,#41889,.F.) ;
#57389=ORIENTED_EDGE('',*,*,#39914,.F.) ;
#57390=ORIENTED_EDGE('',*,*,#41888,.T.) ;
#57391=ORIENTED_EDGE('',*,*,#39902,.F.) ;
#57392=ORIENTED_EDGE('',*,*,#41890,.F.) ;
#57393=ORIENTED_EDGE('',*,*,#41358,.F.) ;
#57394=ORIENTED_EDGE('',*,*,#41889,.T.) ;
#57395=ORIENTED_EDGE('',*,*,#41401,.F.) ;
#57396=ORIENTED_EDGE('',*,*,#41891,.F.) ;
#57397=ORIENTED_EDGE('',*,*,#39915,.F.) ;
#57398=ORIENTED_EDGE('',*,*,#41890,.T.) ;
#57399=ORIENTED_EDGE('',*,*,#39901,.F.) ;
#57400=ORIENTED_EDGE('',*,*,#41892,.F.) ;
#57401=ORIENTED_EDGE('',*,*,#41355,.F.) ;
#57402=ORIENTED_EDGE('',*,*,#41891,.T.) ;
#57403=ORIENTED_EDGE('',*,*,#41404,.F.) ;
#57404=ORIENTED_EDGE('',*,*,#41893,.F.) ;
#57405=ORIENTED_EDGE('',*,*,#39916,.F.) ;
#57406=ORIENTED_EDGE('',*,*,#41892,.T.) ;
#57407=ORIENTED_EDGE('',*,*,#39900,.F.) ;
#57408=ORIENTED_EDGE('',*,*,#41894,.F.) ;
#57409=ORIENTED_EDGE('',*,*,#41352,.F.) ;
#57410=ORIENTED_EDGE('',*,*,#41893,.T.) ;
#57411=ORIENTED_EDGE('',*,*,#41407,.F.) ;
#57412=ORIENTED_EDGE('',*,*,#41895,.F.) ;
#57413=ORIENTED_EDGE('',*,*,#39917,.F.) ;
#57414=ORIENTED_EDGE('',*,*,#41349,.F.) ;
#57415=ORIENTED_EDGE('',*,*,#41894,.T.) ;
#57416=ORIENTED_EDGE('',*,*,#41896,.F.) ;
#57417=ORIENTED_EDGE('',*,*,#41895,.T.) ;
#57418=ORIENTED_EDGE('',*,*,#41410,.F.) ;
#57419=ORIENTED_EDGE('',*,*,#41897,.F.) ;
#57420=ORIENTED_EDGE('',*,*,#39918,.F.) ;
#57421=ORIENTED_EDGE('',*,*,#41896,.T.) ;
#57422=ORIENTED_EDGE('',*,*,#39899,.F.) ;
#57423=ORIENTED_EDGE('',*,*,#41898,.F.) ;
#57424=ORIENTED_EDGE('',*,*,#41346,.F.) ;
#57425=ORIENTED_EDGE('',*,*,#41897,.T.) ;
#57426=ORIENTED_EDGE('',*,*,#41413,.F.) ;
#57427=ORIENTED_EDGE('',*,*,#41899,.F.) ;
#57428=ORIENTED_EDGE('',*,*,#39919,.F.) ;
#57429=ORIENTED_EDGE('',*,*,#41343,.F.) ;
#57430=ORIENTED_EDGE('',*,*,#41898,.T.) ;
#57431=ORIENTED_EDGE('',*,*,#41900,.F.) ;
#57432=ORIENTED_EDGE('',*,*,#41899,.T.) ;
#57433=ORIENTED_EDGE('',*,*,#41416,.F.) ;
#57434=ORIENTED_EDGE('',*,*,#41901,.F.) ;
#57435=ORIENTED_EDGE('',*,*,#39897,.F.) ;
#57436=ORIENTED_EDGE('',*,*,#41900,.T.) ;
#57437=ORIENTED_EDGE('',*,*,#39898,.F.) ;
#57438=ORIENTED_EDGE('',*,*,#41901,.T.) ;
#57439=ORIENTED_EDGE('',*,*,#41418,.F.) ;
#57440=ORIENTED_EDGE('',*,*,#41902,.F.) ;
#57441=ORIENTED_EDGE('',*,*,#41474,.F.) ;
#57442=ORIENTED_EDGE('',*,*,#41903,.F.) ;
#57443=ORIENTED_EDGE('',*,*,#39931,.F.) ;
#57444=ORIENTED_EDGE('',*,*,#41471,.F.) ;
#57445=ORIENTED_EDGE('',*,*,#41902,.T.) ;
#57446=ORIENTED_EDGE('',*,*,#41904,.F.) ;
#57447=ORIENTED_EDGE('',*,*,#41903,.T.) ;
#57448=ORIENTED_EDGE('',*,*,#41477,.F.) ;
#57449=ORIENTED_EDGE('',*,*,#41905,.F.) ;
#57450=ORIENTED_EDGE('',*,*,#41904,.T.) ;
#57451=ORIENTED_EDGE('',*,*,#39930,.F.) ;
#57452=ORIENTED_EDGE('',*,*,#41906,.F.) ;
#57453=ORIENTED_EDGE('',*,*,#41468,.F.) ;
#57454=ORIENTED_EDGE('',*,*,#41905,.T.) ;
#57455=ORIENTED_EDGE('',*,*,#41480,.F.) ;
#57456=ORIENTED_EDGE('',*,*,#41907,.F.) ;
#57457=ORIENTED_EDGE('',*,*,#39932,.F.) ;
#57458=ORIENTED_EDGE('',*,*,#41906,.T.) ;
#57459=ORIENTED_EDGE('',*,*,#39929,.F.) ;
#57460=ORIENTED_EDGE('',*,*,#41908,.F.) ;
#57461=ORIENTED_EDGE('',*,*,#41465,.F.) ;
#57462=ORIENTED_EDGE('',*,*,#41907,.T.) ;
#57463=ORIENTED_EDGE('',*,*,#41483,.F.) ;
#57464=ORIENTED_EDGE('',*,*,#41909,.F.) ;
#57465=ORIENTED_EDGE('',*,*,#39933,.F.) ;
#57466=ORIENTED_EDGE('',*,*,#41908,.T.) ;
#57467=ORIENTED_EDGE('',*,*,#39928,.F.) ;
#57468=ORIENTED_EDGE('',*,*,#39231,.F.) ;
#57469=ORIENTED_EDGE('',*,*,#41462,.F.) ;
#57470=ORIENTED_EDGE('',*,*,#41909,.T.) ;
#57471=ORIENTED_EDGE('',*,*,#41486,.F.) ;
#57472=ORIENTED_EDGE('',*,*,#41910,.F.) ;
#57473=ORIENTED_EDGE('',*,*,#39934,.F.) ;
#57474=ORIENTED_EDGE('',*,*,#41910,.T.) ;
#57475=ORIENTED_EDGE('',*,*,#41489,.F.) ;
#57476=ORIENTED_EDGE('',*,*,#41911,.F.) ;
#57477=ORIENTED_EDGE('',*,*,#39935,.F.) ;
#57478=ORIENTED_EDGE('',*,*,#39229,.T.) ;
#57479=ORIENTED_EDGE('',*,*,#39927,.F.) ;
#57480=ORIENTED_EDGE('',*,*,#41912,.F.) ;
#57481=ORIENTED_EDGE('',*,*,#41459,.F.) ;
#57482=ORIENTED_EDGE('',*,*,#41911,.T.) ;
#57483=ORIENTED_EDGE('',*,*,#41492,.F.) ;
#57484=ORIENTED_EDGE('',*,*,#41913,.F.) ;
#57485=ORIENTED_EDGE('',*,*,#39936,.F.) ;
#57486=ORIENTED_EDGE('',*,*,#41912,.T.) ;
#57487=ORIENTED_EDGE('',*,*,#39926,.F.) ;
#57488=ORIENTED_EDGE('',*,*,#41914,.F.) ;
#57489=ORIENTED_EDGE('',*,*,#41457,.F.) ;
#57490=ORIENTED_EDGE('',*,*,#41913,.T.) ;
#57491=ORIENTED_EDGE('',*,*,#41495,.F.) ;
#57492=ORIENTED_EDGE('',*,*,#41915,.F.) ;
#57493=ORIENTED_EDGE('',*,*,#39937,.F.) ;
#57494=ORIENTED_EDGE('',*,*,#41914,.T.) ;
#57495=ORIENTED_EDGE('',*,*,#39925,.F.) ;
#57496=ORIENTED_EDGE('',*,*,#41916,.F.) ;
#57497=ORIENTED_EDGE('',*,*,#41455,.F.) ;
#57498=ORIENTED_EDGE('',*,*,#41915,.T.) ;
#57499=ORIENTED_EDGE('',*,*,#41498,.F.) ;
#57500=ORIENTED_EDGE('',*,*,#41917,.F.) ;
#57501=ORIENTED_EDGE('',*,*,#39938,.F.) ;
#57502=ORIENTED_EDGE('',*,*,#41916,.T.) ;
#57503=ORIENTED_EDGE('',*,*,#39924,.F.) ;
#57504=ORIENTED_EDGE('',*,*,#41918,.F.) ;
#57505=ORIENTED_EDGE('',*,*,#41452,.F.) ;
#57506=ORIENTED_EDGE('',*,*,#41917,.T.) ;
#57507=ORIENTED_EDGE('',*,*,#41501,.F.) ;
#57508=ORIENTED_EDGE('',*,*,#41919,.F.) ;
#57509=ORIENTED_EDGE('',*,*,#39939,.F.) ;
#57510=ORIENTED_EDGE('',*,*,#41918,.T.) ;
#57511=ORIENTED_EDGE('',*,*,#39923,.F.) ;
#57512=ORIENTED_EDGE('',*,*,#41920,.F.) ;
#57513=ORIENTED_EDGE('',*,*,#41449,.F.) ;
#57514=ORIENTED_EDGE('',*,*,#41919,.T.) ;
#57515=ORIENTED_EDGE('',*,*,#41504,.F.) ;
#57516=ORIENTED_EDGE('',*,*,#41921,.F.) ;
#57517=ORIENTED_EDGE('',*,*,#39940,.F.) ;
#57518=ORIENTED_EDGE('',*,*,#41446,.F.) ;
#57519=ORIENTED_EDGE('',*,*,#41920,.T.) ;
#57520=ORIENTED_EDGE('',*,*,#41922,.F.) ;
#57521=ORIENTED_EDGE('',*,*,#41921,.T.) ;
#57522=ORIENTED_EDGE('',*,*,#41507,.F.) ;
#57523=ORIENTED_EDGE('',*,*,#41923,.F.) ;
#57524=ORIENTED_EDGE('',*,*,#39941,.F.) ;
#57525=ORIENTED_EDGE('',*,*,#41922,.T.) ;
#57526=ORIENTED_EDGE('',*,*,#39922,.F.) ;
#57527=ORIENTED_EDGE('',*,*,#41924,.F.) ;
#57528=ORIENTED_EDGE('',*,*,#41443,.F.) ;
#57529=ORIENTED_EDGE('',*,*,#41923,.T.) ;
#57530=ORIENTED_EDGE('',*,*,#41510,.F.) ;
#57531=ORIENTED_EDGE('',*,*,#41925,.F.) ;
#57532=ORIENTED_EDGE('',*,*,#39942,.F.) ;
#57533=ORIENTED_EDGE('',*,*,#41440,.F.) ;
#57534=ORIENTED_EDGE('',*,*,#41924,.T.) ;
#57535=ORIENTED_EDGE('',*,*,#41926,.F.) ;
#57536=ORIENTED_EDGE('',*,*,#41925,.T.) ;
#57537=ORIENTED_EDGE('',*,*,#41513,.F.) ;
#57538=ORIENTED_EDGE('',*,*,#41927,.F.) ;
#57539=ORIENTED_EDGE('',*,*,#39920,.F.) ;
#57540=ORIENTED_EDGE('',*,*,#41926,.T.) ;
#57541=ORIENTED_EDGE('',*,*,#39921,.F.) ;
#57542=ORIENTED_EDGE('',*,*,#41927,.T.) ;
#57543=ORIENTED_EDGE('',*,*,#41515,.F.) ;
#57544=ORIENTED_EDGE('',*,*,#41928,.F.) ;
#57545=ORIENTED_EDGE('',*,*,#40521,.F.) ;
#57546=ORIENTED_EDGE('',*,*,#41929,.F.) ;
#57547=ORIENTED_EDGE('',*,*,#40479,.F.) ;
#57548=ORIENTED_EDGE('',*,*,#41930,.F.) ;
#57549=ORIENTED_EDGE('',*,*,#40522,.F.) ;
#57550=ORIENTED_EDGE('',*,*,#41931,.F.) ;
#57551=ORIENTED_EDGE('',*,*,#40516,.F.) ;
#57552=ORIENTED_EDGE('',*,*,#41932,.F.) ;
#57553=ORIENTED_EDGE('',*,*,#41930,.T.) ;
#57554=ORIENTED_EDGE('',*,*,#41933,.F.) ;
#57555=ORIENTED_EDGE('',*,*,#41934,.F.) ;
#57556=ORIENTED_EDGE('',*,*,#41929,.T.) ;
#57557=ORIENTED_EDGE('',*,*,#41935,.F.) ;
#57558=ORIENTED_EDGE('',*,*,#41928,.T.) ;
#57559=ORIENTED_EDGE('',*,*,#40478,.T.) ;
#57560=ORIENTED_EDGE('',*,*,#41936,.F.) ;
#57561=ORIENTED_EDGE('',*,*,#41931,.T.) ;
#57562=ORIENTED_EDGE('',*,*,#41933,.T.) ;
#57563=ORIENTED_EDGE('',*,*,#40519,.F.) ;
#57564=ORIENTED_EDGE('',*,*,#41937,.F.) ;
#57565=ORIENTED_EDGE('',*,*,#39217,.T.) ;
#57566=ORIENTED_EDGE('',*,*,#41938,.T.) ;
#57567=ORIENTED_EDGE('',*,*,#41939,.F.) ;
#57568=ORIENTED_EDGE('',*,*,#41932,.T.) ;
#57569=ORIENTED_EDGE('',*,*,#41940,.F.) ;
#57570=ORIENTED_EDGE('',*,*,#41941,.T.) ;
#57571=ORIENTED_EDGE('',*,*,#41942,.F.) ;
#57572=ORIENTED_EDGE('',*,*,#39415,.F.) ;
#57573=ORIENTED_EDGE('',*,*,#41943,.F.) ;
#57574=ORIENTED_EDGE('',*,*,#40523,.F.) ;
#57575=ORIENTED_EDGE('',*,*,#41935,.T.) ;
#57576=ORIENTED_EDGE('',*,*,#40520,.F.) ;
#57577=ORIENTED_EDGE('',*,*,#41944,.F.) ;
#57578=ORIENTED_EDGE('',*,*,#40526,.F.) ;
#57579=ORIENTED_EDGE('',*,*,#41934,.T.) ;
#57580=ORIENTED_EDGE('',*,*,#40525,.F.) ;
#57581=ORIENTED_EDGE('',*,*,#41945,.F.) ;
#57582=ORIENTED_EDGE('',*,*,#40470,.F.) ;
#57583=ORIENTED_EDGE('',*,*,#41936,.T.) ;
#57584=ORIENTED_EDGE('',*,*,#40477,.F.) ;
#57585=ORIENTED_EDGE('',*,*,#41946,.F.) ;
#57586=ORIENTED_EDGE('',*,*,#40517,.F.) ;
#57587=ORIENTED_EDGE('',*,*,#41947,.F.) ;
#57588=ORIENTED_EDGE('',*,*,#40518,.F.) ;
#57589=ORIENTED_EDGE('',*,*,#41948,.F.) ;
#57590=ORIENTED_EDGE('',*,*,#40513,.F.) ;
#57591=ORIENTED_EDGE('',*,*,#41937,.T.) ;
#57592=ORIENTED_EDGE('',*,*,#41947,.T.) ;
#57593=ORIENTED_EDGE('',*,*,#39218,.F.) ;
#57594=ORIENTED_EDGE('',*,*,#41943,.T.) ;
#57595=ORIENTED_EDGE('',*,*,#39425,.T.) ;
#57596=ORIENTED_EDGE('',*,*,#41949,.F.) ;
#57597=ORIENTED_EDGE('',*,*,#41944,.T.) ;
#57598=ORIENTED_EDGE('',*,*,#41950,.F.) ;
#57599=ORIENTED_EDGE('',*,*,#41945,.T.) ;
#57600=ORIENTED_EDGE('',*,*,#41951,.F.) ;
#57601=ORIENTED_EDGE('',*,*,#39512,.T.) ;
#57602=ORIENTED_EDGE('',*,*,#41946,.T.) ;
#57603=ORIENTED_EDGE('',*,*,#40476,.T.) ;
#57604=ORIENTED_EDGE('',*,*,#41952,.F.) ;
#57605=ORIENTED_EDGE('',*,*,#41948,.T.) ;
#57606=ORIENTED_EDGE('',*,*,#41949,.T.) ;
#57607=ORIENTED_EDGE('',*,*,#39424,.F.) ;
#57608=ORIENTED_EDGE('',*,*,#41953,.F.) ;
#57609=ORIENTED_EDGE('',*,*,#40527,.F.) ;
#57610=ORIENTED_EDGE('',*,*,#41951,.T.) ;
#57611=ORIENTED_EDGE('',*,*,#40524,.F.) ;
#57612=ORIENTED_EDGE('',*,*,#41954,.F.) ;
#57613=ORIENTED_EDGE('',*,*,#39513,.F.) ;
#57614=ORIENTED_EDGE('',*,*,#40471,.F.) ;
#57615=ORIENTED_EDGE('',*,*,#41950,.T.) ;
#57616=ORIENTED_EDGE('',*,*,#41955,.F.) ;
#57617=ORIENTED_EDGE('',*,*,#41956,.F.) ;
#57618=ORIENTED_EDGE('',*,*,#41952,.T.) ;
#57619=ORIENTED_EDGE('',*,*,#40475,.F.) ;
#57620=ORIENTED_EDGE('',*,*,#41957,.F.) ;
#57621=ORIENTED_EDGE('',*,*,#40514,.F.) ;
#57622=ORIENTED_EDGE('',*,*,#41958,.F.) ;
#57623=ORIENTED_EDGE('',*,*,#40515,.F.) ;
#57624=ORIENTED_EDGE('',*,*,#41959,.F.) ;
#57625=ORIENTED_EDGE('',*,*,#40509,.F.) ;
#57626=ORIENTED_EDGE('',*,*,#39220,.T.) ;
#57627=ORIENTED_EDGE('',*,*,#41958,.T.) ;
#57628=ORIENTED_EDGE('',*,*,#41960,.F.) ;
#57629=ORIENTED_EDGE('',*,*,#39419,.T.) ;
#57630=ORIENTED_EDGE('',*,*,#41954,.T.) ;
#57631=ORIENTED_EDGE('',*,*,#41953,.T.) ;
#57632=ORIENTED_EDGE('',*,*,#41961,.F.) ;
#57633=ORIENTED_EDGE('',*,*,#41962,.F.) ;
#57634=ORIENTED_EDGE('',*,*,#39532,.F.) ;
#57635=ORIENTED_EDGE('',*,*,#41963,.F.) ;
#57636=ORIENTED_EDGE('',*,*,#41964,.F.) ;
#57637=ORIENTED_EDGE('',*,*,#41955,.T.) ;
#57638=ORIENTED_EDGE('',*,*,#39516,.F.) ;
#57639=ORIENTED_EDGE('',*,*,#41963,.T.) ;
#57640=ORIENTED_EDGE('',*,*,#39684,.F.) ;
#57641=ORIENTED_EDGE('',*,*,#41956,.T.) ;
#57642=ORIENTED_EDGE('',*,*,#41965,.F.) ;
#57643=ORIENTED_EDGE('',*,*,#41966,.F.) ;
#57644=ORIENTED_EDGE('',*,*,#41959,.T.) ;
#57645=ORIENTED_EDGE('',*,*,#41957,.T.) ;
#57646=ORIENTED_EDGE('',*,*,#41967,.F.) ;
#57647=ORIENTED_EDGE('',*,*,#41960,.T.) ;
#57648=ORIENTED_EDGE('',*,*,#40512,.F.) ;
#57649=ORIENTED_EDGE('',*,*,#41968,.F.) ;
#57650=ORIENTED_EDGE('',*,*,#39420,.F.) ;
#57651=ORIENTED_EDGE('',*,*,#41961,.T.) ;
#57652=ORIENTED_EDGE('',*,*,#39423,.F.) ;
#57653=ORIENTED_EDGE('',*,*,#41969,.F.) ;
#57654=ORIENTED_EDGE('',*,*,#39514,.F.) ;
#57655=ORIENTED_EDGE('',*,*,#41962,.T.) ;
#57656=ORIENTED_EDGE('',*,*,#39515,.F.) ;
#57657=ORIENTED_EDGE('',*,*,#41970,.F.) ;
#57658=ORIENTED_EDGE('',*,*,#39607,.F.) ;
#57659=ORIENTED_EDGE('',*,*,#41964,.T.) ;
#57660=ORIENTED_EDGE('',*,*,#39683,.T.) ;
#57661=ORIENTED_EDGE('',*,*,#41971,.F.) ;
#57662=ORIENTED_EDGE('',*,*,#41965,.T.) ;
#57663=ORIENTED_EDGE('',*,*,#40472,.F.) ;
#57664=ORIENTED_EDGE('',*,*,#41966,.T.) ;
#57665=ORIENTED_EDGE('',*,*,#41972,.F.) ;
#57666=ORIENTED_EDGE('',*,*,#41973,.F.) ;
#57667=ORIENTED_EDGE('',*,*,#41967,.T.) ;
#57668=ORIENTED_EDGE('',*,*,#40474,.F.) ;
#57669=ORIENTED_EDGE('',*,*,#41974,.F.) ;
#57670=ORIENTED_EDGE('',*,*,#40510,.F.) ;
#57671=ORIENTED_EDGE('',*,*,#41975,.F.) ;
#57672=ORIENTED_EDGE('',*,*,#40511,.F.) ;
#57673=ORIENTED_EDGE('',*,*,#41976,.F.) ;
#57674=ORIENTED_EDGE('',*,*,#39511,.F.) ;
#57675=ORIENTED_EDGE('',*,*,#41968,.T.) ;
#57676=ORIENTED_EDGE('',*,*,#41975,.T.) ;
#57677=ORIENTED_EDGE('',*,*,#41977,.F.) ;
#57678=ORIENTED_EDGE('',*,*,#41970,.T.) ;
#57679=ORIENTED_EDGE('',*,*,#41969,.T.) ;
#57680=ORIENTED_EDGE('',*,*,#41978,.F.) ;
#57681=ORIENTED_EDGE('',*,*,#39608,.T.) ;
#57682=ORIENTED_EDGE('',*,*,#41979,.F.) ;
#57683=ORIENTED_EDGE('',*,*,#41972,.T.) ;
#57684=ORIENTED_EDGE('',*,*,#41971,.T.) ;
#57685=ORIENTED_EDGE('',*,*,#39682,.F.) ;
#57686=ORIENTED_EDGE('',*,*,#41973,.T.) ;
#57687=ORIENTED_EDGE('',*,*,#41980,.F.) ;
#57688=ORIENTED_EDGE('',*,*,#41981,.F.) ;
#57689=ORIENTED_EDGE('',*,*,#41976,.T.) ;
#57690=ORIENTED_EDGE('',*,*,#41974,.T.) ;
#57691=ORIENTED_EDGE('',*,*,#41982,.F.) ;
#57692=ORIENTED_EDGE('',*,*,#39507,.T.) ;
#57693=ORIENTED_EDGE('',*,*,#41977,.T.) ;
#57694=ORIENTED_EDGE('',*,*,#39510,.F.) ;
#57695=ORIENTED_EDGE('',*,*,#41983,.F.) ;
#57696=ORIENTED_EDGE('',*,*,#39421,.F.) ;
#57697=ORIENTED_EDGE('',*,*,#41978,.T.) ;
#57698=ORIENTED_EDGE('',*,*,#39422,.F.) ;
#57699=ORIENTED_EDGE('',*,*,#41984,.F.) ;
#57700=ORIENTED_EDGE('',*,*,#39609,.F.) ;
#57701=ORIENTED_EDGE('',*,*,#41979,.T.) ;
#57702=ORIENTED_EDGE('',*,*,#39681,.T.) ;
#57703=ORIENTED_EDGE('',*,*,#41985,.F.) ;
#57704=ORIENTED_EDGE('',*,*,#41980,.T.) ;
#57705=ORIENTED_EDGE('',*,*,#40473,.F.) ;
#57706=ORIENTED_EDGE('',*,*,#41981,.T.) ;
#57707=ORIENTED_EDGE('',*,*,#41986,.F.) ;
#57708=ORIENTED_EDGE('',*,*,#41982,.T.) ;
#57709=ORIENTED_EDGE('',*,*,#41984,.T.) ;
#57710=ORIENTED_EDGE('',*,*,#41983,.T.) ;
#57711=ORIENTED_EDGE('',*,*,#41987,.F.) ;
#57712=ORIENTED_EDGE('',*,*,#39610,.T.) ;
#57713=ORIENTED_EDGE('',*,*,#41985,.T.) ;
#57714=ORIENTED_EDGE('',*,*,#39680,.F.) ;
#57715=ORIENTED_EDGE('',*,*,#41988,.F.) ;
#57716=ORIENTED_EDGE('',*,*,#39508,.F.) ;
#57717=ORIENTED_EDGE('',*,*,#41986,.T.) ;
#57718=ORIENTED_EDGE('',*,*,#41987,.T.) ;
#57719=ORIENTED_EDGE('',*,*,#39509,.F.) ;
#57720=ORIENTED_EDGE('',*,*,#41989,.F.) ;
#57721=ORIENTED_EDGE('',*,*,#39611,.F.) ;
#57722=ORIENTED_EDGE('',*,*,#41988,.T.) ;
#57723=ORIENTED_EDGE('',*,*,#39538,.F.) ;
#57724=ORIENTED_EDGE('',*,*,#41989,.T.) ;
#57725=ORIENTED_EDGE('',*,*,#41990,.F.) ;
#57726=ORIENTED_EDGE('',*,*,#41381,.F.) ;
#57727=ORIENTED_EDGE('',*,*,#41991,.F.) ;
#57728=ORIENTED_EDGE('',*,*,#41428,.F.) ;
#57729=ORIENTED_EDGE('',*,*,#41991,.T.) ;
#57730=ORIENTED_EDGE('',*,*,#41378,.F.) ;
#57731=ORIENTED_EDGE('',*,*,#41992,.F.) ;
#57732=ORIENTED_EDGE('',*,*,#41429,.F.) ;
#57733=ORIENTED_EDGE('',*,*,#41384,.F.) ;
#57734=ORIENTED_EDGE('',*,*,#41990,.T.) ;
#57735=ORIENTED_EDGE('',*,*,#41993,.F.) ;
#57736=ORIENTED_EDGE('',*,*,#41992,.T.) ;
#57737=ORIENTED_EDGE('',*,*,#41375,.F.) ;
#57738=ORIENTED_EDGE('',*,*,#41994,.F.) ;
#57739=ORIENTED_EDGE('',*,*,#41430,.F.) ;
#57740=ORIENTED_EDGE('',*,*,#41993,.T.) ;
#57741=ORIENTED_EDGE('',*,*,#41427,.F.) ;
#57742=ORIENTED_EDGE('',*,*,#41995,.F.) ;
#57743=ORIENTED_EDGE('',*,*,#41387,.F.) ;
#57744=ORIENTED_EDGE('',*,*,#41994,.T.) ;
#57745=ORIENTED_EDGE('',*,*,#41372,.F.) ;
#57746=ORIENTED_EDGE('',*,*,#41996,.F.) ;
#57747=ORIENTED_EDGE('',*,*,#41431,.F.) ;
#57748=ORIENTED_EDGE('',*,*,#41390,.F.) ;
#57749=ORIENTED_EDGE('',*,*,#41995,.T.) ;
#57750=ORIENTED_EDGE('',*,*,#41997,.F.) ;
#57751=ORIENTED_EDGE('',*,*,#41996,.T.) ;
#57752=ORIENTED_EDGE('',*,*,#41369,.F.) ;
#57753=ORIENTED_EDGE('',*,*,#41998,.F.) ;
#57754=ORIENTED_EDGE('',*,*,#41432,.F.) ;
#57755=ORIENTED_EDGE('',*,*,#41997,.T.) ;
#57756=ORIENTED_EDGE('',*,*,#41426,.F.) ;
#57757=ORIENTED_EDGE('',*,*,#41999,.F.) ;
#57758=ORIENTED_EDGE('',*,*,#41393,.F.) ;
#57759=ORIENTED_EDGE('',*,*,#41998,.T.) ;
#57760=ORIENTED_EDGE('',*,*,#41366,.F.) ;
#57761=ORIENTED_EDGE('',*,*,#42000,.F.) ;
#57762=ORIENTED_EDGE('',*,*,#41396,.F.) ;
#57763=ORIENTED_EDGE('',*,*,#41999,.T.) ;
#57764=ORIENTED_EDGE('',*,*,#42001,.F.) ;
#57765=ORIENTED_EDGE('',*,*,#42000,.T.) ;
#57766=ORIENTED_EDGE('',*,*,#41363,.F.) ;
#57767=ORIENTED_EDGE('',*,*,#42002,.F.) ;
#57768=ORIENTED_EDGE('',*,*,#41433,.F.) ;
#57769=ORIENTED_EDGE('',*,*,#42001,.T.) ;
#57770=ORIENTED_EDGE('',*,*,#41425,.F.) ;
#57771=ORIENTED_EDGE('',*,*,#42003,.F.) ;
#57772=ORIENTED_EDGE('',*,*,#41399,.F.) ;
#57773=ORIENTED_EDGE('',*,*,#42002,.T.) ;
#57774=ORIENTED_EDGE('',*,*,#39289,.F.) ;
#57775=ORIENTED_EDGE('',*,*,#42004,.F.) ;
#57776=ORIENTED_EDGE('',*,*,#41402,.F.) ;
#57777=ORIENTED_EDGE('',*,*,#42003,.T.) ;
#57778=ORIENTED_EDGE('',*,*,#42005,.F.) ;
#57779=ORIENTED_EDGE('',*,*,#42004,.T.) ;
#57780=ORIENTED_EDGE('',*,*,#41361,.F.) ;
#57781=ORIENTED_EDGE('',*,*,#39216,.F.) ;
#57782=ORIENTED_EDGE('',*,*,#41434,.F.) ;
#57783=ORIENTED_EDGE('',*,*,#42005,.T.) ;
#57784=ORIENTED_EDGE('',*,*,#41424,.F.) ;
#57785=ORIENTED_EDGE('',*,*,#42006,.F.) ;
#57786=ORIENTED_EDGE('',*,*,#41405,.F.) ;
#57787=ORIENTED_EDGE('',*,*,#41408,.F.) ;
#57788=ORIENTED_EDGE('',*,*,#42006,.T.) ;
#57789=ORIENTED_EDGE('',*,*,#42007,.F.) ;
#57790=ORIENTED_EDGE('',*,*,#39215,.T.) ;
#57791=ORIENTED_EDGE('',*,*,#41356,.F.) ;
#57792=ORIENTED_EDGE('',*,*,#42008,.F.) ;
#57793=ORIENTED_EDGE('',*,*,#41435,.F.) ;
#57794=ORIENTED_EDGE('',*,*,#42007,.T.) ;
#57795=ORIENTED_EDGE('',*,*,#41423,.F.) ;
#57796=ORIENTED_EDGE('',*,*,#42009,.F.) ;
#57797=ORIENTED_EDGE('',*,*,#41411,.F.) ;
#57798=ORIENTED_EDGE('',*,*,#42008,.T.) ;
#57799=ORIENTED_EDGE('',*,*,#41353,.F.) ;
#57800=ORIENTED_EDGE('',*,*,#42010,.F.) ;
#57801=ORIENTED_EDGE('',*,*,#41414,.F.) ;
#57802=ORIENTED_EDGE('',*,*,#42009,.T.) ;
#57803=ORIENTED_EDGE('',*,*,#42011,.F.) ;
#57804=ORIENTED_EDGE('',*,*,#42010,.T.) ;
#57805=ORIENTED_EDGE('',*,*,#41350,.F.) ;
#57806=ORIENTED_EDGE('',*,*,#42012,.F.) ;
#57807=ORIENTED_EDGE('',*,*,#41436,.F.) ;
#57808=ORIENTED_EDGE('',*,*,#42011,.T.) ;
#57809=ORIENTED_EDGE('',*,*,#41422,.F.) ;
#57810=ORIENTED_EDGE('',*,*,#42013,.F.) ;
#57811=ORIENTED_EDGE('',*,*,#41417,.F.) ;
#57812=ORIENTED_EDGE('',*,*,#42012,.T.) ;
#57813=ORIENTED_EDGE('',*,*,#41347,.F.) ;
#57814=ORIENTED_EDGE('',*,*,#42014,.F.) ;
#57815=ORIENTED_EDGE('',*,*,#41419,.F.) ;
#57816=ORIENTED_EDGE('',*,*,#42013,.T.) ;
#57817=ORIENTED_EDGE('',*,*,#41421,.F.) ;
#57818=ORIENTED_EDGE('',*,*,#42015,.F.) ;
#57819=ORIENTED_EDGE('',*,*,#41341,.F.) ;
#57820=ORIENTED_EDGE('',*,*,#42014,.T.) ;
#57821=ORIENTED_EDGE('',*,*,#41344,.F.) ;
#57822=ORIENTED_EDGE('',*,*,#42015,.T.) ;
#57823=ORIENTED_EDGE('',*,*,#41420,.F.) ;
#57824=ORIENTED_EDGE('',*,*,#42016,.F.) ;
#57825=ORIENTED_EDGE('',*,*,#40540,.F.) ;
#57826=ORIENTED_EDGE('',*,*,#42017,.F.) ;
#57827=ORIENTED_EDGE('',*,*,#40469,.F.) ;
#57828=ORIENTED_EDGE('',*,*,#42018,.F.) ;
#57829=ORIENTED_EDGE('',*,*,#40541,.F.) ;
#57830=ORIENTED_EDGE('',*,*,#42019,.F.) ;
#57831=ORIENTED_EDGE('',*,*,#40535,.F.) ;
#57832=ORIENTED_EDGE('',*,*,#42020,.F.) ;
#57833=ORIENTED_EDGE('',*,*,#42018,.T.) ;
#57834=ORIENTED_EDGE('',*,*,#42021,.F.) ;
#57835=ORIENTED_EDGE('',*,*,#42022,.F.) ;
#57836=ORIENTED_EDGE('',*,*,#42017,.T.) ;
#57837=ORIENTED_EDGE('',*,*,#42023,.F.) ;
#57838=ORIENTED_EDGE('',*,*,#42016,.T.) ;
#57839=ORIENTED_EDGE('',*,*,#40468,.T.) ;
#57840=ORIENTED_EDGE('',*,*,#42024,.F.) ;
#57841=ORIENTED_EDGE('',*,*,#42019,.T.) ;
#57842=ORIENTED_EDGE('',*,*,#42021,.T.) ;
#57843=ORIENTED_EDGE('',*,*,#40538,.F.) ;
#57844=ORIENTED_EDGE('',*,*,#42025,.F.) ;
#57845=ORIENTED_EDGE('',*,*,#39200,.T.) ;
#57846=ORIENTED_EDGE('',*,*,#42026,.T.) ;
#57847=ORIENTED_EDGE('',*,*,#42027,.F.) ;
#57848=ORIENTED_EDGE('',*,*,#42020,.T.) ;
#57849=ORIENTED_EDGE('',*,*,#42028,.F.) ;
#57850=ORIENTED_EDGE('',*,*,#42029,.T.) ;
#57851=ORIENTED_EDGE('',*,*,#42030,.F.) ;
#57852=ORIENTED_EDGE('',*,*,#39404,.F.) ;
#57853=ORIENTED_EDGE('',*,*,#42031,.F.) ;
#57854=ORIENTED_EDGE('',*,*,#40542,.F.) ;
#57855=ORIENTED_EDGE('',*,*,#42023,.T.) ;
#57856=ORIENTED_EDGE('',*,*,#40539,.F.) ;
#57857=ORIENTED_EDGE('',*,*,#42032,.F.) ;
#57858=ORIENTED_EDGE('',*,*,#40545,.F.) ;
#57859=ORIENTED_EDGE('',*,*,#42022,.T.) ;
#57860=ORIENTED_EDGE('',*,*,#40544,.F.) ;
#57861=ORIENTED_EDGE('',*,*,#42033,.F.) ;
#57862=ORIENTED_EDGE('',*,*,#40460,.F.) ;
#57863=ORIENTED_EDGE('',*,*,#42024,.T.) ;
#57864=ORIENTED_EDGE('',*,*,#40467,.F.) ;
#57865=ORIENTED_EDGE('',*,*,#42034,.F.) ;
#57866=ORIENTED_EDGE('',*,*,#40536,.F.) ;
#57867=ORIENTED_EDGE('',*,*,#42035,.F.) ;
#57868=ORIENTED_EDGE('',*,*,#40537,.F.) ;
#57869=ORIENTED_EDGE('',*,*,#42036,.F.) ;
#57870=ORIENTED_EDGE('',*,*,#40532,.F.) ;
#57871=ORIENTED_EDGE('',*,*,#42025,.T.) ;
#57872=ORIENTED_EDGE('',*,*,#42035,.T.) ;
#57873=ORIENTED_EDGE('',*,*,#39201,.F.) ;
#57874=ORIENTED_EDGE('',*,*,#42031,.T.) ;
#57875=ORIENTED_EDGE('',*,*,#39414,.T.) ;
#57876=ORIENTED_EDGE('',*,*,#42037,.F.) ;
#57877=ORIENTED_EDGE('',*,*,#42032,.T.) ;
#57878=ORIENTED_EDGE('',*,*,#42038,.F.) ;
#57879=ORIENTED_EDGE('',*,*,#42033,.T.) ;
#57880=ORIENTED_EDGE('',*,*,#42039,.F.) ;
#57881=ORIENTED_EDGE('',*,*,#39502,.T.) ;
#57882=ORIENTED_EDGE('',*,*,#42034,.T.) ;
#57883=ORIENTED_EDGE('',*,*,#40466,.T.) ;
#57884=ORIENTED_EDGE('',*,*,#42040,.F.) ;
#57885=ORIENTED_EDGE('',*,*,#42036,.T.) ;
#57886=ORIENTED_EDGE('',*,*,#42037,.T.) ;
#57887=ORIENTED_EDGE('',*,*,#39413,.F.) ;
#57888=ORIENTED_EDGE('',*,*,#42041,.F.) ;
#57889=ORIENTED_EDGE('',*,*,#40546,.F.) ;
#57890=ORIENTED_EDGE('',*,*,#42039,.T.) ;
#57891=ORIENTED_EDGE('',*,*,#40543,.F.) ;
#57892=ORIENTED_EDGE('',*,*,#42042,.F.) ;
#57893=ORIENTED_EDGE('',*,*,#39503,.F.) ;
#57894=ORIENTED_EDGE('',*,*,#40461,.F.) ;
#57895=ORIENTED_EDGE('',*,*,#42038,.T.) ;
#57896=ORIENTED_EDGE('',*,*,#42043,.F.) ;
#57897=ORIENTED_EDGE('',*,*,#42044,.F.) ;
#57898=ORIENTED_EDGE('',*,*,#42040,.T.) ;
#57899=ORIENTED_EDGE('',*,*,#40465,.F.) ;
#57900=ORIENTED_EDGE('',*,*,#42045,.F.) ;
#57901=ORIENTED_EDGE('',*,*,#40533,.F.) ;
#57902=ORIENTED_EDGE('',*,*,#42046,.F.) ;
#57903=ORIENTED_EDGE('',*,*,#40534,.F.) ;
#57904=ORIENTED_EDGE('',*,*,#42047,.F.) ;
#57905=ORIENTED_EDGE('',*,*,#40528,.F.) ;
#57906=ORIENTED_EDGE('',*,*,#39203,.T.) ;
#57907=ORIENTED_EDGE('',*,*,#42046,.T.) ;
#57908=ORIENTED_EDGE('',*,*,#42048,.F.) ;
#57909=ORIENTED_EDGE('',*,*,#39408,.T.) ;
#57910=ORIENTED_EDGE('',*,*,#42042,.T.) ;
#57911=ORIENTED_EDGE('',*,*,#42041,.T.) ;
#57912=ORIENTED_EDGE('',*,*,#42049,.F.) ;
#57913=ORIENTED_EDGE('',*,*,#42050,.F.) ;
#57914=ORIENTED_EDGE('',*,*,#39536,.F.) ;
#57915=ORIENTED_EDGE('',*,*,#42051,.F.) ;
#57916=ORIENTED_EDGE('',*,*,#42052,.F.) ;
#57917=ORIENTED_EDGE('',*,*,#42043,.T.) ;
#57918=ORIENTED_EDGE('',*,*,#39506,.F.) ;
#57919=ORIENTED_EDGE('',*,*,#42051,.T.) ;
#57920=ORIENTED_EDGE('',*,*,#39679,.F.) ;
#57921=ORIENTED_EDGE('',*,*,#42044,.T.) ;
#57922=ORIENTED_EDGE('',*,*,#42053,.F.) ;
#57923=ORIENTED_EDGE('',*,*,#42054,.F.) ;
#57924=ORIENTED_EDGE('',*,*,#42047,.T.) ;
#57925=ORIENTED_EDGE('',*,*,#42045,.T.) ;
#57926=ORIENTED_EDGE('',*,*,#42055,.F.) ;
#57927=ORIENTED_EDGE('',*,*,#42048,.T.) ;
#57928=ORIENTED_EDGE('',*,*,#40531,.F.) ;
#57929=ORIENTED_EDGE('',*,*,#42056,.F.) ;
#57930=ORIENTED_EDGE('',*,*,#39409,.F.) ;
#57931=ORIENTED_EDGE('',*,*,#42049,.T.) ;
#57932=ORIENTED_EDGE('',*,*,#39412,.F.) ;
#57933=ORIENTED_EDGE('',*,*,#42057,.F.) ;
#57934=ORIENTED_EDGE('',*,*,#39504,.F.) ;
#57935=ORIENTED_EDGE('',*,*,#42050,.T.) ;
#57936=ORIENTED_EDGE('',*,*,#39505,.F.) ;
#57937=ORIENTED_EDGE('',*,*,#42058,.F.) ;
#57938=ORIENTED_EDGE('',*,*,#39612,.F.) ;
#57939=ORIENTED_EDGE('',*,*,#42052,.T.) ;
#57940=ORIENTED_EDGE('',*,*,#39678,.T.) ;
#57941=ORIENTED_EDGE('',*,*,#42059,.F.) ;
#57942=ORIENTED_EDGE('',*,*,#42053,.T.) ;
#57943=ORIENTED_EDGE('',*,*,#40462,.F.) ;
#57944=ORIENTED_EDGE('',*,*,#42054,.T.) ;
#57945=ORIENTED_EDGE('',*,*,#42060,.F.) ;
#57946=ORIENTED_EDGE('',*,*,#42061,.F.) ;
#57947=ORIENTED_EDGE('',*,*,#42055,.T.) ;
#57948=ORIENTED_EDGE('',*,*,#40464,.F.) ;
#57949=ORIENTED_EDGE('',*,*,#42062,.F.) ;
#57950=ORIENTED_EDGE('',*,*,#40529,.F.) ;
#57951=ORIENTED_EDGE('',*,*,#42063,.F.) ;
#57952=ORIENTED_EDGE('',*,*,#40530,.F.) ;
#57953=ORIENTED_EDGE('',*,*,#42064,.F.) ;
#57954=ORIENTED_EDGE('',*,*,#39501,.F.) ;
#57955=ORIENTED_EDGE('',*,*,#42056,.T.) ;
#57956=ORIENTED_EDGE('',*,*,#42063,.T.) ;
#57957=ORIENTED_EDGE('',*,*,#42065,.F.) ;
#57958=ORIENTED_EDGE('',*,*,#42058,.T.) ;
#57959=ORIENTED_EDGE('',*,*,#42057,.T.) ;
#57960=ORIENTED_EDGE('',*,*,#42066,.F.) ;
#57961=ORIENTED_EDGE('',*,*,#39613,.T.) ;
#57962=ORIENTED_EDGE('',*,*,#42067,.F.) ;
#57963=ORIENTED_EDGE('',*,*,#42060,.T.) ;
#57964=ORIENTED_EDGE('',*,*,#42059,.T.) ;
#57965=ORIENTED_EDGE('',*,*,#39677,.F.) ;
#57966=ORIENTED_EDGE('',*,*,#42061,.T.) ;
#57967=ORIENTED_EDGE('',*,*,#42068,.F.) ;
#57968=ORIENTED_EDGE('',*,*,#42069,.F.) ;
#57969=ORIENTED_EDGE('',*,*,#42064,.T.) ;
#57970=ORIENTED_EDGE('',*,*,#42062,.T.) ;
#57971=ORIENTED_EDGE('',*,*,#42070,.F.) ;
#57972=ORIENTED_EDGE('',*,*,#39497,.T.) ;
#57973=ORIENTED_EDGE('',*,*,#42065,.T.) ;
#57974=ORIENTED_EDGE('',*,*,#39500,.F.) ;
#57975=ORIENTED_EDGE('',*,*,#42071,.F.) ;
#57976=ORIENTED_EDGE('',*,*,#39410,.F.) ;
#57977=ORIENTED_EDGE('',*,*,#42066,.T.) ;
#57978=ORIENTED_EDGE('',*,*,#39411,.F.) ;
#57979=ORIENTED_EDGE('',*,*,#42072,.F.) ;
#57980=ORIENTED_EDGE('',*,*,#39614,.F.) ;
#57981=ORIENTED_EDGE('',*,*,#42067,.T.) ;
#57982=ORIENTED_EDGE('',*,*,#39676,.T.) ;
#57983=ORIENTED_EDGE('',*,*,#42073,.F.) ;
#57984=ORIENTED_EDGE('',*,*,#42068,.T.) ;
#57985=ORIENTED_EDGE('',*,*,#40463,.F.) ;
#57986=ORIENTED_EDGE('',*,*,#42069,.T.) ;
#57987=ORIENTED_EDGE('',*,*,#42074,.F.) ;
#57988=ORIENTED_EDGE('',*,*,#42070,.T.) ;
#57989=ORIENTED_EDGE('',*,*,#42072,.T.) ;
#57990=ORIENTED_EDGE('',*,*,#42071,.T.) ;
#57991=ORIENTED_EDGE('',*,*,#42075,.F.) ;
#57992=ORIENTED_EDGE('',*,*,#39615,.T.) ;
#57993=ORIENTED_EDGE('',*,*,#42073,.T.) ;
#57994=ORIENTED_EDGE('',*,*,#39675,.F.) ;
#57995=ORIENTED_EDGE('',*,*,#42076,.F.) ;
#57996=ORIENTED_EDGE('',*,*,#39498,.F.) ;
#57997=ORIENTED_EDGE('',*,*,#42074,.T.) ;
#57998=ORIENTED_EDGE('',*,*,#42075,.T.) ;
#57999=ORIENTED_EDGE('',*,*,#39499,.F.) ;
#58000=ORIENTED_EDGE('',*,*,#42077,.F.) ;
#58001=ORIENTED_EDGE('',*,*,#39616,.F.) ;
#58002=ORIENTED_EDGE('',*,*,#42076,.T.) ;
#58003=ORIENTED_EDGE('',*,*,#39542,.F.) ;
#58004=ORIENTED_EDGE('',*,*,#42077,.T.) ;
#58005=ORIENTED_EDGE('',*,*,#42078,.F.) ;
#58006=ORIENTED_EDGE('',*,*,#41284,.F.) ;
#58007=ORIENTED_EDGE('',*,*,#42079,.F.) ;
#58008=ORIENTED_EDGE('',*,*,#41331,.F.) ;
#58009=ORIENTED_EDGE('',*,*,#42079,.T.) ;
#58010=ORIENTED_EDGE('',*,*,#41281,.F.) ;
#58011=ORIENTED_EDGE('',*,*,#42080,.F.) ;
#58012=ORIENTED_EDGE('',*,*,#41332,.F.) ;
#58013=ORIENTED_EDGE('',*,*,#41287,.F.) ;
#58014=ORIENTED_EDGE('',*,*,#42078,.T.) ;
#58015=ORIENTED_EDGE('',*,*,#42081,.F.) ;
#58016=ORIENTED_EDGE('',*,*,#42080,.T.) ;
#58017=ORIENTED_EDGE('',*,*,#41278,.F.) ;
#58018=ORIENTED_EDGE('',*,*,#42082,.F.) ;
#58019=ORIENTED_EDGE('',*,*,#41333,.F.) ;
#58020=ORIENTED_EDGE('',*,*,#42081,.T.) ;
#58021=ORIENTED_EDGE('',*,*,#41330,.F.) ;
#58022=ORIENTED_EDGE('',*,*,#42083,.F.) ;
#58023=ORIENTED_EDGE('',*,*,#41290,.F.) ;
#58024=ORIENTED_EDGE('',*,*,#42082,.T.) ;
#58025=ORIENTED_EDGE('',*,*,#41275,.F.) ;
#58026=ORIENTED_EDGE('',*,*,#42084,.F.) ;
#58027=ORIENTED_EDGE('',*,*,#41334,.F.) ;
#58028=ORIENTED_EDGE('',*,*,#41293,.F.) ;
#58029=ORIENTED_EDGE('',*,*,#42083,.T.) ;
#58030=ORIENTED_EDGE('',*,*,#42085,.F.) ;
#58031=ORIENTED_EDGE('',*,*,#42084,.T.) ;
#58032=ORIENTED_EDGE('',*,*,#41272,.F.) ;
#58033=ORIENTED_EDGE('',*,*,#42086,.F.) ;
#58034=ORIENTED_EDGE('',*,*,#41335,.F.) ;
#58035=ORIENTED_EDGE('',*,*,#42085,.T.) ;
#58036=ORIENTED_EDGE('',*,*,#41329,.F.) ;
#58037=ORIENTED_EDGE('',*,*,#42087,.F.) ;
#58038=ORIENTED_EDGE('',*,*,#41296,.F.) ;
#58039=ORIENTED_EDGE('',*,*,#42086,.T.) ;
#58040=ORIENTED_EDGE('',*,*,#41269,.F.) ;
#58041=ORIENTED_EDGE('',*,*,#42088,.F.) ;
#58042=ORIENTED_EDGE('',*,*,#41299,.F.) ;
#58043=ORIENTED_EDGE('',*,*,#42087,.T.) ;
#58044=ORIENTED_EDGE('',*,*,#42089,.F.) ;
#58045=ORIENTED_EDGE('',*,*,#42088,.T.) ;
#58046=ORIENTED_EDGE('',*,*,#41266,.F.) ;
#58047=ORIENTED_EDGE('',*,*,#42090,.F.) ;
#58048=ORIENTED_EDGE('',*,*,#41336,.F.) ;
#58049=ORIENTED_EDGE('',*,*,#42089,.T.) ;
#58050=ORIENTED_EDGE('',*,*,#41328,.F.) ;
#58051=ORIENTED_EDGE('',*,*,#42091,.F.) ;
#58052=ORIENTED_EDGE('',*,*,#41302,.F.) ;
#58053=ORIENTED_EDGE('',*,*,#42090,.T.) ;
#58054=ORIENTED_EDGE('',*,*,#39292,.F.) ;
#58055=ORIENTED_EDGE('',*,*,#42092,.F.) ;
#58056=ORIENTED_EDGE('',*,*,#41305,.F.) ;
#58057=ORIENTED_EDGE('',*,*,#42091,.T.) ;
#58058=ORIENTED_EDGE('',*,*,#42093,.F.) ;
#58059=ORIENTED_EDGE('',*,*,#42092,.T.) ;
#58060=ORIENTED_EDGE('',*,*,#41264,.F.) ;
#58061=ORIENTED_EDGE('',*,*,#39199,.F.) ;
#58062=ORIENTED_EDGE('',*,*,#41337,.F.) ;
#58063=ORIENTED_EDGE('',*,*,#42093,.T.) ;
#58064=ORIENTED_EDGE('',*,*,#41327,.F.) ;
#58065=ORIENTED_EDGE('',*,*,#42094,.F.) ;
#58066=ORIENTED_EDGE('',*,*,#41308,.F.) ;
#58067=ORIENTED_EDGE('',*,*,#41311,.F.) ;
#58068=ORIENTED_EDGE('',*,*,#42094,.T.) ;
#58069=ORIENTED_EDGE('',*,*,#42095,.F.) ;
#58070=ORIENTED_EDGE('',*,*,#39198,.T.) ;
#58071=ORIENTED_EDGE('',*,*,#41259,.F.) ;
#58072=ORIENTED_EDGE('',*,*,#42096,.F.) ;
#58073=ORIENTED_EDGE('',*,*,#41338,.F.) ;
#58074=ORIENTED_EDGE('',*,*,#42095,.T.) ;
#58075=ORIENTED_EDGE('',*,*,#41326,.F.) ;
#58076=ORIENTED_EDGE('',*,*,#42097,.F.) ;
#58077=ORIENTED_EDGE('',*,*,#41314,.F.) ;
#58078=ORIENTED_EDGE('',*,*,#42096,.T.) ;
#58079=ORIENTED_EDGE('',*,*,#41256,.F.) ;
#58080=ORIENTED_EDGE('',*,*,#42098,.F.) ;
#58081=ORIENTED_EDGE('',*,*,#41317,.F.) ;
#58082=ORIENTED_EDGE('',*,*,#42097,.T.) ;
#58083=ORIENTED_EDGE('',*,*,#42099,.F.) ;
#58084=ORIENTED_EDGE('',*,*,#42098,.T.) ;
#58085=ORIENTED_EDGE('',*,*,#41253,.F.) ;
#58086=ORIENTED_EDGE('',*,*,#42100,.F.) ;
#58087=ORIENTED_EDGE('',*,*,#41339,.F.) ;
#58088=ORIENTED_EDGE('',*,*,#42099,.T.) ;
#58089=ORIENTED_EDGE('',*,*,#41325,.F.) ;
#58090=ORIENTED_EDGE('',*,*,#42101,.F.) ;
#58091=ORIENTED_EDGE('',*,*,#41320,.F.) ;
#58092=ORIENTED_EDGE('',*,*,#42100,.T.) ;
#58093=ORIENTED_EDGE('',*,*,#41250,.F.) ;
#58094=ORIENTED_EDGE('',*,*,#42102,.F.) ;
#58095=ORIENTED_EDGE('',*,*,#41322,.F.) ;
#58096=ORIENTED_EDGE('',*,*,#42101,.T.) ;
#58097=ORIENTED_EDGE('',*,*,#41324,.F.) ;
#58098=ORIENTED_EDGE('',*,*,#42103,.F.) ;
#58099=ORIENTED_EDGE('',*,*,#41244,.F.) ;
#58100=ORIENTED_EDGE('',*,*,#42102,.T.) ;
#58101=ORIENTED_EDGE('',*,*,#41247,.F.) ;
#58102=ORIENTED_EDGE('',*,*,#42103,.T.) ;
#58103=ORIENTED_EDGE('',*,*,#41323,.F.) ;
#58104=ORIENTED_EDGE('',*,*,#42104,.F.) ;
#58105=ORIENTED_EDGE('',*,*,#40559,.F.) ;
#58106=ORIENTED_EDGE('',*,*,#42105,.F.) ;
#58107=ORIENTED_EDGE('',*,*,#40459,.F.) ;
#58108=ORIENTED_EDGE('',*,*,#42106,.F.) ;
#58109=ORIENTED_EDGE('',*,*,#40560,.F.) ;
#58110=ORIENTED_EDGE('',*,*,#42107,.F.) ;
#58111=ORIENTED_EDGE('',*,*,#40554,.F.) ;
#58112=ORIENTED_EDGE('',*,*,#42108,.F.) ;
#58113=ORIENTED_EDGE('',*,*,#42106,.T.) ;
#58114=ORIENTED_EDGE('',*,*,#42109,.F.) ;
#58115=ORIENTED_EDGE('',*,*,#42110,.F.) ;
#58116=ORIENTED_EDGE('',*,*,#42105,.T.) ;
#58117=ORIENTED_EDGE('',*,*,#42111,.F.) ;
#58118=ORIENTED_EDGE('',*,*,#42104,.T.) ;
#58119=ORIENTED_EDGE('',*,*,#40458,.T.) ;
#58120=ORIENTED_EDGE('',*,*,#42112,.F.) ;
#58121=ORIENTED_EDGE('',*,*,#42107,.T.) ;
#58122=ORIENTED_EDGE('',*,*,#42109,.T.) ;
#58123=ORIENTED_EDGE('',*,*,#40557,.F.) ;
#58124=ORIENTED_EDGE('',*,*,#42113,.F.) ;
#58125=ORIENTED_EDGE('',*,*,#39183,.T.) ;
#58126=ORIENTED_EDGE('',*,*,#42114,.T.) ;
#58127=ORIENTED_EDGE('',*,*,#42115,.F.) ;
#58128=ORIENTED_EDGE('',*,*,#42108,.T.) ;
#58129=ORIENTED_EDGE('',*,*,#42116,.F.) ;
#58130=ORIENTED_EDGE('',*,*,#42117,.T.) ;
#58131=ORIENTED_EDGE('',*,*,#42118,.F.) ;
#58132=ORIENTED_EDGE('',*,*,#39393,.F.) ;
#58133=ORIENTED_EDGE('',*,*,#42119,.F.) ;
#58134=ORIENTED_EDGE('',*,*,#40561,.F.) ;
#58135=ORIENTED_EDGE('',*,*,#42111,.T.) ;
#58136=ORIENTED_EDGE('',*,*,#40558,.F.) ;
#58137=ORIENTED_EDGE('',*,*,#42120,.F.) ;
#58138=ORIENTED_EDGE('',*,*,#40564,.F.) ;
#58139=ORIENTED_EDGE('',*,*,#42110,.T.) ;
#58140=ORIENTED_EDGE('',*,*,#40563,.F.) ;
#58141=ORIENTED_EDGE('',*,*,#42121,.F.) ;
#58142=ORIENTED_EDGE('',*,*,#40450,.F.) ;
#58143=ORIENTED_EDGE('',*,*,#42112,.T.) ;
#58144=ORIENTED_EDGE('',*,*,#40457,.F.) ;
#58145=ORIENTED_EDGE('',*,*,#42122,.F.) ;
#58146=ORIENTED_EDGE('',*,*,#40555,.F.) ;
#58147=ORIENTED_EDGE('',*,*,#42123,.F.) ;
#58148=ORIENTED_EDGE('',*,*,#40556,.F.) ;
#58149=ORIENTED_EDGE('',*,*,#42124,.F.) ;
#58150=ORIENTED_EDGE('',*,*,#40551,.F.) ;
#58151=ORIENTED_EDGE('',*,*,#42113,.T.) ;
#58152=ORIENTED_EDGE('',*,*,#42123,.T.) ;
#58153=ORIENTED_EDGE('',*,*,#39184,.F.) ;
#58154=ORIENTED_EDGE('',*,*,#42119,.T.) ;
#58155=ORIENTED_EDGE('',*,*,#39403,.T.) ;
#58156=ORIENTED_EDGE('',*,*,#42125,.F.) ;
#58157=ORIENTED_EDGE('',*,*,#42120,.T.) ;
#58158=ORIENTED_EDGE('',*,*,#42126,.F.) ;
#58159=ORIENTED_EDGE('',*,*,#42121,.T.) ;
#58160=ORIENTED_EDGE('',*,*,#42127,.F.) ;
#58161=ORIENTED_EDGE('',*,*,#39492,.T.) ;
#58162=ORIENTED_EDGE('',*,*,#42122,.T.) ;
#58163=ORIENTED_EDGE('',*,*,#40456,.T.) ;
#58164=ORIENTED_EDGE('',*,*,#42128,.F.) ;
#58165=ORIENTED_EDGE('',*,*,#42124,.T.) ;
#58166=ORIENTED_EDGE('',*,*,#42125,.T.) ;
#58167=ORIENTED_EDGE('',*,*,#39402,.F.) ;
#58168=ORIENTED_EDGE('',*,*,#42129,.F.) ;
#58169=ORIENTED_EDGE('',*,*,#40565,.F.) ;
#58170=ORIENTED_EDGE('',*,*,#42127,.T.) ;
#58171=ORIENTED_EDGE('',*,*,#40562,.F.) ;
#58172=ORIENTED_EDGE('',*,*,#42130,.F.) ;
#58173=ORIENTED_EDGE('',*,*,#39493,.F.) ;
#58174=ORIENTED_EDGE('',*,*,#40451,.F.) ;
#58175=ORIENTED_EDGE('',*,*,#42126,.T.) ;
#58176=ORIENTED_EDGE('',*,*,#42131,.F.) ;
#58177=ORIENTED_EDGE('',*,*,#42132,.F.) ;
#58178=ORIENTED_EDGE('',*,*,#42128,.T.) ;
#58179=ORIENTED_EDGE('',*,*,#40455,.F.) ;
#58180=ORIENTED_EDGE('',*,*,#42133,.F.) ;
#58181=ORIENTED_EDGE('',*,*,#40552,.F.) ;
#58182=ORIENTED_EDGE('',*,*,#42134,.F.) ;
#58183=ORIENTED_EDGE('',*,*,#40553,.F.) ;
#58184=ORIENTED_EDGE('',*,*,#42135,.F.) ;
#58185=ORIENTED_EDGE('',*,*,#40547,.F.) ;
#58186=ORIENTED_EDGE('',*,*,#39186,.T.) ;
#58187=ORIENTED_EDGE('',*,*,#42134,.T.) ;
#58188=ORIENTED_EDGE('',*,*,#42136,.F.) ;
#58189=ORIENTED_EDGE('',*,*,#39397,.T.) ;
#58190=ORIENTED_EDGE('',*,*,#42130,.T.) ;
#58191=ORIENTED_EDGE('',*,*,#42129,.T.) ;
#58192=ORIENTED_EDGE('',*,*,#42137,.F.) ;
#58193=ORIENTED_EDGE('',*,*,#42138,.F.) ;
#58194=ORIENTED_EDGE('',*,*,#39540,.F.) ;
#58195=ORIENTED_EDGE('',*,*,#42139,.F.) ;
#58196=ORIENTED_EDGE('',*,*,#42140,.F.) ;
#58197=ORIENTED_EDGE('',*,*,#42131,.T.) ;
#58198=ORIENTED_EDGE('',*,*,#39496,.F.) ;
#58199=ORIENTED_EDGE('',*,*,#42139,.T.) ;
#58200=ORIENTED_EDGE('',*,*,#39674,.F.) ;
#58201=ORIENTED_EDGE('',*,*,#42132,.T.) ;
#58202=ORIENTED_EDGE('',*,*,#42141,.F.) ;
#58203=ORIENTED_EDGE('',*,*,#42142,.F.) ;
#58204=ORIENTED_EDGE('',*,*,#42135,.T.) ;
#58205=ORIENTED_EDGE('',*,*,#42133,.T.) ;
#58206=ORIENTED_EDGE('',*,*,#42143,.F.) ;
#58207=ORIENTED_EDGE('',*,*,#42136,.T.) ;
#58208=ORIENTED_EDGE('',*,*,#40550,.F.) ;
#58209=ORIENTED_EDGE('',*,*,#42144,.F.) ;
#58210=ORIENTED_EDGE('',*,*,#39398,.F.) ;
#58211=ORIENTED_EDGE('',*,*,#42137,.T.) ;
#58212=ORIENTED_EDGE('',*,*,#39401,.F.) ;
#58213=ORIENTED_EDGE('',*,*,#42145,.F.) ;
#58214=ORIENTED_EDGE('',*,*,#39494,.F.) ;
#58215=ORIENTED_EDGE('',*,*,#42138,.T.) ;
#58216=ORIENTED_EDGE('',*,*,#39495,.F.) ;
#58217=ORIENTED_EDGE('',*,*,#42146,.F.) ;
#58218=ORIENTED_EDGE('',*,*,#39617,.F.) ;
#58219=ORIENTED_EDGE('',*,*,#42140,.T.) ;
#58220=ORIENTED_EDGE('',*,*,#39673,.T.) ;
#58221=ORIENTED_EDGE('',*,*,#42147,.F.) ;
#58222=ORIENTED_EDGE('',*,*,#42141,.T.) ;
#58223=ORIENTED_EDGE('',*,*,#40452,.F.) ;
#58224=ORIENTED_EDGE('',*,*,#42142,.T.) ;
#58225=ORIENTED_EDGE('',*,*,#42148,.F.) ;
#58226=ORIENTED_EDGE('',*,*,#42149,.F.) ;
#58227=ORIENTED_EDGE('',*,*,#42143,.T.) ;
#58228=ORIENTED_EDGE('',*,*,#40454,.F.) ;
#58229=ORIENTED_EDGE('',*,*,#42150,.F.) ;
#58230=ORIENTED_EDGE('',*,*,#40548,.F.) ;
#58231=ORIENTED_EDGE('',*,*,#42151,.F.) ;
#58232=ORIENTED_EDGE('',*,*,#40549,.F.) ;
#58233=ORIENTED_EDGE('',*,*,#42152,.F.) ;
#58234=ORIENTED_EDGE('',*,*,#39491,.F.) ;
#58235=ORIENTED_EDGE('',*,*,#42144,.T.) ;
#58236=ORIENTED_EDGE('',*,*,#42151,.T.) ;
#58237=ORIENTED_EDGE('',*,*,#42153,.F.) ;
#58238=ORIENTED_EDGE('',*,*,#42146,.T.) ;
#58239=ORIENTED_EDGE('',*,*,#42145,.T.) ;
#58240=ORIENTED_EDGE('',*,*,#42154,.F.) ;
#58241=ORIENTED_EDGE('',*,*,#39618,.T.) ;
#58242=ORIENTED_EDGE('',*,*,#42155,.F.) ;
#58243=ORIENTED_EDGE('',*,*,#42148,.T.) ;
#58244=ORIENTED_EDGE('',*,*,#42147,.T.) ;
#58245=ORIENTED_EDGE('',*,*,#39672,.F.) ;
#58246=ORIENTED_EDGE('',*,*,#42149,.T.) ;
#58247=ORIENTED_EDGE('',*,*,#42156,.F.) ;
#58248=ORIENTED_EDGE('',*,*,#42157,.F.) ;
#58249=ORIENTED_EDGE('',*,*,#42152,.T.) ;
#58250=ORIENTED_EDGE('',*,*,#42150,.T.) ;
#58251=ORIENTED_EDGE('',*,*,#42158,.F.) ;
#58252=ORIENTED_EDGE('',*,*,#39487,.T.) ;
#58253=ORIENTED_EDGE('',*,*,#42153,.T.) ;
#58254=ORIENTED_EDGE('',*,*,#39490,.F.) ;
#58255=ORIENTED_EDGE('',*,*,#42159,.F.) ;
#58256=ORIENTED_EDGE('',*,*,#39399,.F.) ;
#58257=ORIENTED_EDGE('',*,*,#42154,.T.) ;
#58258=ORIENTED_EDGE('',*,*,#39400,.F.) ;
#58259=ORIENTED_EDGE('',*,*,#42160,.F.) ;
#58260=ORIENTED_EDGE('',*,*,#39619,.F.) ;
#58261=ORIENTED_EDGE('',*,*,#42155,.T.) ;
#58262=ORIENTED_EDGE('',*,*,#39671,.T.) ;
#58263=ORIENTED_EDGE('',*,*,#42161,.F.) ;
#58264=ORIENTED_EDGE('',*,*,#42156,.T.) ;
#58265=ORIENTED_EDGE('',*,*,#40453,.F.) ;
#58266=ORIENTED_EDGE('',*,*,#42157,.T.) ;
#58267=ORIENTED_EDGE('',*,*,#42162,.F.) ;
#58268=ORIENTED_EDGE('',*,*,#42158,.T.) ;
#58269=ORIENTED_EDGE('',*,*,#42160,.T.) ;
#58270=ORIENTED_EDGE('',*,*,#42159,.T.) ;
#58271=ORIENTED_EDGE('',*,*,#42163,.F.) ;
#58272=ORIENTED_EDGE('',*,*,#39620,.T.) ;
#58273=ORIENTED_EDGE('',*,*,#42161,.T.) ;
#58274=ORIENTED_EDGE('',*,*,#39670,.F.) ;
#58275=ORIENTED_EDGE('',*,*,#42164,.F.) ;
#58276=ORIENTED_EDGE('',*,*,#39488,.F.) ;
#58277=ORIENTED_EDGE('',*,*,#42162,.T.) ;
#58278=ORIENTED_EDGE('',*,*,#42163,.T.) ;
#58279=ORIENTED_EDGE('',*,*,#39489,.F.) ;
#58280=ORIENTED_EDGE('',*,*,#42165,.F.) ;
#58281=ORIENTED_EDGE('',*,*,#39621,.F.) ;
#58282=ORIENTED_EDGE('',*,*,#42164,.T.) ;
#58283=ORIENTED_EDGE('',*,*,#39546,.F.) ;
#58284=ORIENTED_EDGE('',*,*,#42165,.T.) ;
#58285=ORIENTED_EDGE('',*,*,#42166,.F.) ;
#58286=ORIENTED_EDGE('',*,*,#41187,.F.) ;
#58287=ORIENTED_EDGE('',*,*,#42167,.F.) ;
#58288=ORIENTED_EDGE('',*,*,#41234,.F.) ;
#58289=ORIENTED_EDGE('',*,*,#42167,.T.) ;
#58290=ORIENTED_EDGE('',*,*,#41184,.F.) ;
#58291=ORIENTED_EDGE('',*,*,#42168,.F.) ;
#58292=ORIENTED_EDGE('',*,*,#41235,.F.) ;
#58293=ORIENTED_EDGE('',*,*,#41190,.F.) ;
#58294=ORIENTED_EDGE('',*,*,#42166,.T.) ;
#58295=ORIENTED_EDGE('',*,*,#42169,.F.) ;
#58296=ORIENTED_EDGE('',*,*,#42168,.T.) ;
#58297=ORIENTED_EDGE('',*,*,#41181,.F.) ;
#58298=ORIENTED_EDGE('',*,*,#42170,.F.) ;
#58299=ORIENTED_EDGE('',*,*,#41236,.F.) ;
#58300=ORIENTED_EDGE('',*,*,#42169,.T.) ;
#58301=ORIENTED_EDGE('',*,*,#41233,.F.) ;
#58302=ORIENTED_EDGE('',*,*,#42171,.F.) ;
#58303=ORIENTED_EDGE('',*,*,#41193,.F.) ;
#58304=ORIENTED_EDGE('',*,*,#42170,.T.) ;
#58305=ORIENTED_EDGE('',*,*,#41178,.F.) ;
#58306=ORIENTED_EDGE('',*,*,#42172,.F.) ;
#58307=ORIENTED_EDGE('',*,*,#41237,.F.) ;
#58308=ORIENTED_EDGE('',*,*,#41196,.F.) ;
#58309=ORIENTED_EDGE('',*,*,#42171,.T.) ;
#58310=ORIENTED_EDGE('',*,*,#42173,.F.) ;
#58311=ORIENTED_EDGE('',*,*,#42172,.T.) ;
#58312=ORIENTED_EDGE('',*,*,#41175,.F.) ;
#58313=ORIENTED_EDGE('',*,*,#42174,.F.) ;
#58314=ORIENTED_EDGE('',*,*,#41238,.F.) ;
#58315=ORIENTED_EDGE('',*,*,#42173,.T.) ;
#58316=ORIENTED_EDGE('',*,*,#41232,.F.) ;
#58317=ORIENTED_EDGE('',*,*,#42175,.F.) ;
#58318=ORIENTED_EDGE('',*,*,#41199,.F.) ;
#58319=ORIENTED_EDGE('',*,*,#42174,.T.) ;
#58320=ORIENTED_EDGE('',*,*,#41172,.F.) ;
#58321=ORIENTED_EDGE('',*,*,#42176,.F.) ;
#58322=ORIENTED_EDGE('',*,*,#41202,.F.) ;
#58323=ORIENTED_EDGE('',*,*,#42175,.T.) ;
#58324=ORIENTED_EDGE('',*,*,#42177,.F.) ;
#58325=ORIENTED_EDGE('',*,*,#42176,.T.) ;
#58326=ORIENTED_EDGE('',*,*,#41169,.F.) ;
#58327=ORIENTED_EDGE('',*,*,#42178,.F.) ;
#58328=ORIENTED_EDGE('',*,*,#41239,.F.) ;
#58329=ORIENTED_EDGE('',*,*,#42177,.T.) ;
#58330=ORIENTED_EDGE('',*,*,#41231,.F.) ;
#58331=ORIENTED_EDGE('',*,*,#42179,.F.) ;
#58332=ORIENTED_EDGE('',*,*,#41205,.F.) ;
#58333=ORIENTED_EDGE('',*,*,#42178,.T.) ;
#58334=ORIENTED_EDGE('',*,*,#39295,.F.) ;
#58335=ORIENTED_EDGE('',*,*,#42180,.F.) ;
#58336=ORIENTED_EDGE('',*,*,#41208,.F.) ;
#58337=ORIENTED_EDGE('',*,*,#42179,.T.) ;
#58338=ORIENTED_EDGE('',*,*,#42181,.F.) ;
#58339=ORIENTED_EDGE('',*,*,#42180,.T.) ;
#58340=ORIENTED_EDGE('',*,*,#41167,.F.) ;
#58341=ORIENTED_EDGE('',*,*,#39182,.F.) ;
#58342=ORIENTED_EDGE('',*,*,#41240,.F.) ;
#58343=ORIENTED_EDGE('',*,*,#42181,.T.) ;
#58344=ORIENTED_EDGE('',*,*,#41230,.F.) ;
#58345=ORIENTED_EDGE('',*,*,#42182,.F.) ;
#58346=ORIENTED_EDGE('',*,*,#41211,.F.) ;
#58347=ORIENTED_EDGE('',*,*,#41214,.F.) ;
#58348=ORIENTED_EDGE('',*,*,#42182,.T.) ;
#58349=ORIENTED_EDGE('',*,*,#42183,.F.) ;
#58350=ORIENTED_EDGE('',*,*,#39181,.T.) ;
#58351=ORIENTED_EDGE('',*,*,#41162,.F.) ;
#58352=ORIENTED_EDGE('',*,*,#42184,.F.) ;
#58353=ORIENTED_EDGE('',*,*,#41241,.F.) ;
#58354=ORIENTED_EDGE('',*,*,#42183,.T.) ;
#58355=ORIENTED_EDGE('',*,*,#41229,.F.) ;
#58356=ORIENTED_EDGE('',*,*,#42185,.F.) ;
#58357=ORIENTED_EDGE('',*,*,#41217,.F.) ;
#58358=ORIENTED_EDGE('',*,*,#42184,.T.) ;
#58359=ORIENTED_EDGE('',*,*,#41159,.F.) ;
#58360=ORIENTED_EDGE('',*,*,#42186,.F.) ;
#58361=ORIENTED_EDGE('',*,*,#41220,.F.) ;
#58362=ORIENTED_EDGE('',*,*,#42185,.T.) ;
#58363=ORIENTED_EDGE('',*,*,#42187,.F.) ;
#58364=ORIENTED_EDGE('',*,*,#42186,.T.) ;
#58365=ORIENTED_EDGE('',*,*,#41156,.F.) ;
#58366=ORIENTED_EDGE('',*,*,#42188,.F.) ;
#58367=ORIENTED_EDGE('',*,*,#41242,.F.) ;
#58368=ORIENTED_EDGE('',*,*,#42187,.T.) ;
#58369=ORIENTED_EDGE('',*,*,#41228,.F.) ;
#58370=ORIENTED_EDGE('',*,*,#42189,.F.) ;
#58371=ORIENTED_EDGE('',*,*,#41223,.F.) ;
#58372=ORIENTED_EDGE('',*,*,#42188,.T.) ;
#58373=ORIENTED_EDGE('',*,*,#41153,.F.) ;
#58374=ORIENTED_EDGE('',*,*,#42190,.F.) ;
#58375=ORIENTED_EDGE('',*,*,#41225,.F.) ;
#58376=ORIENTED_EDGE('',*,*,#42189,.T.) ;
#58377=ORIENTED_EDGE('',*,*,#41227,.F.) ;
#58378=ORIENTED_EDGE('',*,*,#42191,.F.) ;
#58379=ORIENTED_EDGE('',*,*,#41147,.F.) ;
#58380=ORIENTED_EDGE('',*,*,#42190,.T.) ;
#58381=ORIENTED_EDGE('',*,*,#41150,.F.) ;
#58382=ORIENTED_EDGE('',*,*,#42191,.T.) ;
#58383=ORIENTED_EDGE('',*,*,#41226,.F.) ;
#58384=ORIENTED_EDGE('',*,*,#42192,.F.) ;
#58385=ORIENTED_EDGE('',*,*,#40578,.F.) ;
#58386=ORIENTED_EDGE('',*,*,#42193,.F.) ;
#58387=ORIENTED_EDGE('',*,*,#40449,.F.) ;
#58388=ORIENTED_EDGE('',*,*,#42194,.F.) ;
#58389=ORIENTED_EDGE('',*,*,#40579,.F.) ;
#58390=ORIENTED_EDGE('',*,*,#42195,.F.) ;
#58391=ORIENTED_EDGE('',*,*,#40573,.F.) ;
#58392=ORIENTED_EDGE('',*,*,#42196,.F.) ;
#58393=ORIENTED_EDGE('',*,*,#42194,.T.) ;
#58394=ORIENTED_EDGE('',*,*,#42197,.F.) ;
#58395=ORIENTED_EDGE('',*,*,#42198,.F.) ;
#58396=ORIENTED_EDGE('',*,*,#42193,.T.) ;
#58397=ORIENTED_EDGE('',*,*,#42199,.F.) ;
#58398=ORIENTED_EDGE('',*,*,#42192,.T.) ;
#58399=ORIENTED_EDGE('',*,*,#40448,.T.) ;
#58400=ORIENTED_EDGE('',*,*,#42200,.F.) ;
#58401=ORIENTED_EDGE('',*,*,#42195,.T.) ;
#58402=ORIENTED_EDGE('',*,*,#42197,.T.) ;
#58403=ORIENTED_EDGE('',*,*,#40576,.F.) ;
#58404=ORIENTED_EDGE('',*,*,#42201,.F.) ;
#58405=ORIENTED_EDGE('',*,*,#39166,.T.) ;
#58406=ORIENTED_EDGE('',*,*,#42202,.T.) ;
#58407=ORIENTED_EDGE('',*,*,#42203,.F.) ;
#58408=ORIENTED_EDGE('',*,*,#42196,.T.) ;
#58409=ORIENTED_EDGE('',*,*,#42204,.F.) ;
#58410=ORIENTED_EDGE('',*,*,#42205,.T.) ;
#58411=ORIENTED_EDGE('',*,*,#42206,.F.) ;
#58412=ORIENTED_EDGE('',*,*,#39382,.F.) ;
#58413=ORIENTED_EDGE('',*,*,#42207,.F.) ;
#58414=ORIENTED_EDGE('',*,*,#40580,.F.) ;
#58415=ORIENTED_EDGE('',*,*,#42199,.T.) ;
#58416=ORIENTED_EDGE('',*,*,#40577,.F.) ;
#58417=ORIENTED_EDGE('',*,*,#42208,.F.) ;
#58418=ORIENTED_EDGE('',*,*,#40583,.F.) ;
#58419=ORIENTED_EDGE('',*,*,#42198,.T.) ;
#58420=ORIENTED_EDGE('',*,*,#40582,.F.) ;
#58421=ORIENTED_EDGE('',*,*,#42209,.F.) ;
#58422=ORIENTED_EDGE('',*,*,#40440,.F.) ;
#58423=ORIENTED_EDGE('',*,*,#42200,.T.) ;
#58424=ORIENTED_EDGE('',*,*,#40447,.F.) ;
#58425=ORIENTED_EDGE('',*,*,#42210,.F.) ;
#58426=ORIENTED_EDGE('',*,*,#40574,.F.) ;
#58427=ORIENTED_EDGE('',*,*,#42211,.F.) ;
#58428=ORIENTED_EDGE('',*,*,#40575,.F.) ;
#58429=ORIENTED_EDGE('',*,*,#42212,.F.) ;
#58430=ORIENTED_EDGE('',*,*,#40570,.F.) ;
#58431=ORIENTED_EDGE('',*,*,#42201,.T.) ;
#58432=ORIENTED_EDGE('',*,*,#42211,.T.) ;
#58433=ORIENTED_EDGE('',*,*,#39167,.F.) ;
#58434=ORIENTED_EDGE('',*,*,#42207,.T.) ;
#58435=ORIENTED_EDGE('',*,*,#39392,.T.) ;
#58436=ORIENTED_EDGE('',*,*,#42213,.F.) ;
#58437=ORIENTED_EDGE('',*,*,#42208,.T.) ;
#58438=ORIENTED_EDGE('',*,*,#42214,.F.) ;
#58439=ORIENTED_EDGE('',*,*,#42209,.T.) ;
#58440=ORIENTED_EDGE('',*,*,#42215,.F.) ;
#58441=ORIENTED_EDGE('',*,*,#39482,.T.) ;
#58442=ORIENTED_EDGE('',*,*,#42210,.T.) ;
#58443=ORIENTED_EDGE('',*,*,#40446,.T.) ;
#58444=ORIENTED_EDGE('',*,*,#42216,.F.) ;
#58445=ORIENTED_EDGE('',*,*,#42212,.T.) ;
#58446=ORIENTED_EDGE('',*,*,#42213,.T.) ;
#58447=ORIENTED_EDGE('',*,*,#39391,.F.) ;
#58448=ORIENTED_EDGE('',*,*,#42217,.F.) ;
#58449=ORIENTED_EDGE('',*,*,#40584,.F.) ;
#58450=ORIENTED_EDGE('',*,*,#42215,.T.) ;
#58451=ORIENTED_EDGE('',*,*,#40581,.F.) ;
#58452=ORIENTED_EDGE('',*,*,#42218,.F.) ;
#58453=ORIENTED_EDGE('',*,*,#39483,.F.) ;
#58454=ORIENTED_EDGE('',*,*,#40441,.F.) ;
#58455=ORIENTED_EDGE('',*,*,#42214,.T.) ;
#58456=ORIENTED_EDGE('',*,*,#42219,.F.) ;
#58457=ORIENTED_EDGE('',*,*,#42220,.F.) ;
#58458=ORIENTED_EDGE('',*,*,#42216,.T.) ;
#58459=ORIENTED_EDGE('',*,*,#40445,.F.) ;
#58460=ORIENTED_EDGE('',*,*,#42221,.F.) ;
#58461=ORIENTED_EDGE('',*,*,#40571,.F.) ;
#58462=ORIENTED_EDGE('',*,*,#42222,.F.) ;
#58463=ORIENTED_EDGE('',*,*,#40572,.F.) ;
#58464=ORIENTED_EDGE('',*,*,#42223,.F.) ;
#58465=ORIENTED_EDGE('',*,*,#40566,.F.) ;
#58466=ORIENTED_EDGE('',*,*,#39169,.T.) ;
#58467=ORIENTED_EDGE('',*,*,#42222,.T.) ;
#58468=ORIENTED_EDGE('',*,*,#42224,.F.) ;
#58469=ORIENTED_EDGE('',*,*,#39386,.T.) ;
#58470=ORIENTED_EDGE('',*,*,#42218,.T.) ;
#58471=ORIENTED_EDGE('',*,*,#42217,.T.) ;
#58472=ORIENTED_EDGE('',*,*,#42225,.F.) ;
#58473=ORIENTED_EDGE('',*,*,#42226,.F.) ;
#58474=ORIENTED_EDGE('',*,*,#39544,.F.) ;
#58475=ORIENTED_EDGE('',*,*,#42227,.F.) ;
#58476=ORIENTED_EDGE('',*,*,#42228,.F.) ;
#58477=ORIENTED_EDGE('',*,*,#42219,.T.) ;
#58478=ORIENTED_EDGE('',*,*,#39486,.F.) ;
#58479=ORIENTED_EDGE('',*,*,#42227,.T.) ;
#58480=ORIENTED_EDGE('',*,*,#39669,.F.) ;
#58481=ORIENTED_EDGE('',*,*,#42220,.T.) ;
#58482=ORIENTED_EDGE('',*,*,#42229,.F.) ;
#58483=ORIENTED_EDGE('',*,*,#42230,.F.) ;
#58484=ORIENTED_EDGE('',*,*,#42223,.T.) ;
#58485=ORIENTED_EDGE('',*,*,#42221,.T.) ;
#58486=ORIENTED_EDGE('',*,*,#42231,.F.) ;
#58487=ORIENTED_EDGE('',*,*,#42224,.T.) ;
#58488=ORIENTED_EDGE('',*,*,#40569,.F.) ;
#58489=ORIENTED_EDGE('',*,*,#42232,.F.) ;
#58490=ORIENTED_EDGE('',*,*,#39387,.F.) ;
#58491=ORIENTED_EDGE('',*,*,#42225,.T.) ;
#58492=ORIENTED_EDGE('',*,*,#39390,.F.) ;
#58493=ORIENTED_EDGE('',*,*,#42233,.F.) ;
#58494=ORIENTED_EDGE('',*,*,#39484,.F.) ;
#58495=ORIENTED_EDGE('',*,*,#42226,.T.) ;
#58496=ORIENTED_EDGE('',*,*,#39485,.F.) ;
#58497=ORIENTED_EDGE('',*,*,#42234,.F.) ;
#58498=ORIENTED_EDGE('',*,*,#39622,.F.) ;
#58499=ORIENTED_EDGE('',*,*,#42228,.T.) ;
#58500=ORIENTED_EDGE('',*,*,#39668,.T.) ;
#58501=ORIENTED_EDGE('',*,*,#42235,.F.) ;
#58502=ORIENTED_EDGE('',*,*,#42229,.T.) ;
#58503=ORIENTED_EDGE('',*,*,#40442,.F.) ;
#58504=ORIENTED_EDGE('',*,*,#42230,.T.) ;
#58505=ORIENTED_EDGE('',*,*,#42236,.F.) ;
#58506=ORIENTED_EDGE('',*,*,#42237,.F.) ;
#58507=ORIENTED_EDGE('',*,*,#42231,.T.) ;
#58508=ORIENTED_EDGE('',*,*,#40444,.F.) ;
#58509=ORIENTED_EDGE('',*,*,#42238,.F.) ;
#58510=ORIENTED_EDGE('',*,*,#40567,.F.) ;
#58511=ORIENTED_EDGE('',*,*,#42239,.F.) ;
#58512=ORIENTED_EDGE('',*,*,#40568,.F.) ;
#58513=ORIENTED_EDGE('',*,*,#42240,.F.) ;
#58514=ORIENTED_EDGE('',*,*,#39481,.F.) ;
#58515=ORIENTED_EDGE('',*,*,#42232,.T.) ;
#58516=ORIENTED_EDGE('',*,*,#42239,.T.) ;
#58517=ORIENTED_EDGE('',*,*,#42241,.F.) ;
#58518=ORIENTED_EDGE('',*,*,#42234,.T.) ;
#58519=ORIENTED_EDGE('',*,*,#42233,.T.) ;
#58520=ORIENTED_EDGE('',*,*,#42242,.F.) ;
#58521=ORIENTED_EDGE('',*,*,#39623,.T.) ;
#58522=ORIENTED_EDGE('',*,*,#42243,.F.) ;
#58523=ORIENTED_EDGE('',*,*,#42236,.T.) ;
#58524=ORIENTED_EDGE('',*,*,#42235,.T.) ;
#58525=ORIENTED_EDGE('',*,*,#39667,.F.) ;
#58526=ORIENTED_EDGE('',*,*,#42237,.T.) ;
#58527=ORIENTED_EDGE('',*,*,#42244,.F.) ;
#58528=ORIENTED_EDGE('',*,*,#42245,.F.) ;
#58529=ORIENTED_EDGE('',*,*,#42240,.T.) ;
#58530=ORIENTED_EDGE('',*,*,#42238,.T.) ;
#58531=ORIENTED_EDGE('',*,*,#42246,.F.) ;
#58532=ORIENTED_EDGE('',*,*,#39477,.T.) ;
#58533=ORIENTED_EDGE('',*,*,#42241,.T.) ;
#58534=ORIENTED_EDGE('',*,*,#39480,.F.) ;
#58535=ORIENTED_EDGE('',*,*,#42247,.F.) ;
#58536=ORIENTED_EDGE('',*,*,#39388,.F.) ;
#58537=ORIENTED_EDGE('',*,*,#42242,.T.) ;
#58538=ORIENTED_EDGE('',*,*,#39389,.F.) ;
#58539=ORIENTED_EDGE('',*,*,#42248,.F.) ;
#58540=ORIENTED_EDGE('',*,*,#39624,.F.) ;
#58541=ORIENTED_EDGE('',*,*,#42243,.T.) ;
#58542=ORIENTED_EDGE('',*,*,#39666,.T.) ;
#58543=ORIENTED_EDGE('',*,*,#42249,.F.) ;
#58544=ORIENTED_EDGE('',*,*,#42244,.T.) ;
#58545=ORIENTED_EDGE('',*,*,#40443,.F.) ;
#58546=ORIENTED_EDGE('',*,*,#42245,.T.) ;
#58547=ORIENTED_EDGE('',*,*,#42250,.F.) ;
#58548=ORIENTED_EDGE('',*,*,#42246,.T.) ;
#58549=ORIENTED_EDGE('',*,*,#42248,.T.) ;
#58550=ORIENTED_EDGE('',*,*,#42247,.T.) ;
#58551=ORIENTED_EDGE('',*,*,#42251,.F.) ;
#58552=ORIENTED_EDGE('',*,*,#39625,.T.) ;
#58553=ORIENTED_EDGE('',*,*,#42249,.T.) ;
#58554=ORIENTED_EDGE('',*,*,#39665,.F.) ;
#58555=ORIENTED_EDGE('',*,*,#42252,.F.) ;
#58556=ORIENTED_EDGE('',*,*,#39478,.F.) ;
#58557=ORIENTED_EDGE('',*,*,#42250,.T.) ;
#58558=ORIENTED_EDGE('',*,*,#42251,.T.) ;
#58559=ORIENTED_EDGE('',*,*,#39479,.F.) ;
#58560=ORIENTED_EDGE('',*,*,#42253,.F.) ;
#58561=ORIENTED_EDGE('',*,*,#39626,.F.) ;
#58562=ORIENTED_EDGE('',*,*,#42252,.T.) ;
#58563=ORIENTED_EDGE('',*,*,#39550,.F.) ;
#58564=ORIENTED_EDGE('',*,*,#42253,.T.) ;
#58565=ORIENTED_EDGE('',*,*,#42254,.F.) ;
#58566=ORIENTED_EDGE('',*,*,#41090,.F.) ;
#58567=ORIENTED_EDGE('',*,*,#42255,.F.) ;
#58568=ORIENTED_EDGE('',*,*,#41137,.F.) ;
#58569=ORIENTED_EDGE('',*,*,#42255,.T.) ;
#58570=ORIENTED_EDGE('',*,*,#41087,.F.) ;
#58571=ORIENTED_EDGE('',*,*,#42256,.F.) ;
#58572=ORIENTED_EDGE('',*,*,#41138,.F.) ;
#58573=ORIENTED_EDGE('',*,*,#41093,.F.) ;
#58574=ORIENTED_EDGE('',*,*,#42254,.T.) ;
#58575=ORIENTED_EDGE('',*,*,#42257,.F.) ;
#58576=ORIENTED_EDGE('',*,*,#42256,.T.) ;
#58577=ORIENTED_EDGE('',*,*,#41084,.F.) ;
#58578=ORIENTED_EDGE('',*,*,#42258,.F.) ;
#58579=ORIENTED_EDGE('',*,*,#41139,.F.) ;
#58580=ORIENTED_EDGE('',*,*,#42257,.T.) ;
#58581=ORIENTED_EDGE('',*,*,#41136,.F.) ;
#58582=ORIENTED_EDGE('',*,*,#42259,.F.) ;
#58583=ORIENTED_EDGE('',*,*,#41096,.F.) ;
#58584=ORIENTED_EDGE('',*,*,#42258,.T.) ;
#58585=ORIENTED_EDGE('',*,*,#41081,.F.) ;
#58586=ORIENTED_EDGE('',*,*,#42260,.F.) ;
#58587=ORIENTED_EDGE('',*,*,#41140,.F.) ;
#58588=ORIENTED_EDGE('',*,*,#41099,.F.) ;
#58589=ORIENTED_EDGE('',*,*,#42259,.T.) ;
#58590=ORIENTED_EDGE('',*,*,#42261,.F.) ;
#58591=ORIENTED_EDGE('',*,*,#42260,.T.) ;
#58592=ORIENTED_EDGE('',*,*,#41078,.F.) ;
#58593=ORIENTED_EDGE('',*,*,#42262,.F.) ;
#58594=ORIENTED_EDGE('',*,*,#41141,.F.) ;
#58595=ORIENTED_EDGE('',*,*,#42261,.T.) ;
#58596=ORIENTED_EDGE('',*,*,#41135,.F.) ;
#58597=ORIENTED_EDGE('',*,*,#42263,.F.) ;
#58598=ORIENTED_EDGE('',*,*,#41102,.F.) ;
#58599=ORIENTED_EDGE('',*,*,#42262,.T.) ;
#58600=ORIENTED_EDGE('',*,*,#41075,.F.) ;
#58601=ORIENTED_EDGE('',*,*,#42264,.F.) ;
#58602=ORIENTED_EDGE('',*,*,#41105,.F.) ;
#58603=ORIENTED_EDGE('',*,*,#42263,.T.) ;
#58604=ORIENTED_EDGE('',*,*,#42265,.F.) ;
#58605=ORIENTED_EDGE('',*,*,#42264,.T.) ;
#58606=ORIENTED_EDGE('',*,*,#41072,.F.) ;
#58607=ORIENTED_EDGE('',*,*,#42266,.F.) ;
#58608=ORIENTED_EDGE('',*,*,#41142,.F.) ;
#58609=ORIENTED_EDGE('',*,*,#42265,.T.) ;
#58610=ORIENTED_EDGE('',*,*,#41134,.F.) ;
#58611=ORIENTED_EDGE('',*,*,#42267,.F.) ;
#58612=ORIENTED_EDGE('',*,*,#41108,.F.) ;
#58613=ORIENTED_EDGE('',*,*,#42266,.T.) ;
#58614=ORIENTED_EDGE('',*,*,#39298,.F.) ;
#58615=ORIENTED_EDGE('',*,*,#42268,.F.) ;
#58616=ORIENTED_EDGE('',*,*,#41111,.F.) ;
#58617=ORIENTED_EDGE('',*,*,#42267,.T.) ;
#58618=ORIENTED_EDGE('',*,*,#42269,.F.) ;
#58619=ORIENTED_EDGE('',*,*,#42268,.T.) ;
#58620=ORIENTED_EDGE('',*,*,#41070,.F.) ;
#58621=ORIENTED_EDGE('',*,*,#39165,.F.) ;
#58622=ORIENTED_EDGE('',*,*,#41143,.F.) ;
#58623=ORIENTED_EDGE('',*,*,#42269,.T.) ;
#58624=ORIENTED_EDGE('',*,*,#41133,.F.) ;
#58625=ORIENTED_EDGE('',*,*,#42270,.F.) ;
#58626=ORIENTED_EDGE('',*,*,#41114,.F.) ;
#58627=ORIENTED_EDGE('',*,*,#41117,.F.) ;
#58628=ORIENTED_EDGE('',*,*,#42270,.T.) ;
#58629=ORIENTED_EDGE('',*,*,#42271,.F.) ;
#58630=ORIENTED_EDGE('',*,*,#39164,.T.) ;
#58631=ORIENTED_EDGE('',*,*,#41065,.F.) ;
#58632=ORIENTED_EDGE('',*,*,#42272,.F.) ;
#58633=ORIENTED_EDGE('',*,*,#41144,.F.) ;
#58634=ORIENTED_EDGE('',*,*,#42271,.T.) ;
#58635=ORIENTED_EDGE('',*,*,#41132,.F.) ;
#58636=ORIENTED_EDGE('',*,*,#42273,.F.) ;
#58637=ORIENTED_EDGE('',*,*,#41120,.F.) ;
#58638=ORIENTED_EDGE('',*,*,#42272,.T.) ;
#58639=ORIENTED_EDGE('',*,*,#41062,.F.) ;
#58640=ORIENTED_EDGE('',*,*,#42274,.F.) ;
#58641=ORIENTED_EDGE('',*,*,#41123,.F.) ;
#58642=ORIENTED_EDGE('',*,*,#42273,.T.) ;
#58643=ORIENTED_EDGE('',*,*,#42275,.F.) ;
#58644=ORIENTED_EDGE('',*,*,#42274,.T.) ;
#58645=ORIENTED_EDGE('',*,*,#41059,.F.) ;
#58646=ORIENTED_EDGE('',*,*,#42276,.F.) ;
#58647=ORIENTED_EDGE('',*,*,#41145,.F.) ;
#58648=ORIENTED_EDGE('',*,*,#42275,.T.) ;
#58649=ORIENTED_EDGE('',*,*,#41131,.F.) ;
#58650=ORIENTED_EDGE('',*,*,#42277,.F.) ;
#58651=ORIENTED_EDGE('',*,*,#41126,.F.) ;
#58652=ORIENTED_EDGE('',*,*,#42276,.T.) ;
#58653=ORIENTED_EDGE('',*,*,#41056,.F.) ;
#58654=ORIENTED_EDGE('',*,*,#42278,.F.) ;
#58655=ORIENTED_EDGE('',*,*,#41128,.F.) ;
#58656=ORIENTED_EDGE('',*,*,#42277,.T.) ;
#58657=ORIENTED_EDGE('',*,*,#41130,.F.) ;
#58658=ORIENTED_EDGE('',*,*,#42279,.F.) ;
#58659=ORIENTED_EDGE('',*,*,#41050,.F.) ;
#58660=ORIENTED_EDGE('',*,*,#42278,.T.) ;
#58661=ORIENTED_EDGE('',*,*,#41053,.F.) ;
#58662=ORIENTED_EDGE('',*,*,#42279,.T.) ;
#58663=ORIENTED_EDGE('',*,*,#41129,.F.) ;
#58664=ORIENTED_EDGE('',*,*,#42280,.F.) ;
#58665=ORIENTED_EDGE('',*,*,#40597,.F.) ;
#58666=ORIENTED_EDGE('',*,*,#42281,.F.) ;
#58667=ORIENTED_EDGE('',*,*,#40439,.F.) ;
#58668=ORIENTED_EDGE('',*,*,#42282,.F.) ;
#58669=ORIENTED_EDGE('',*,*,#40598,.F.) ;
#58670=ORIENTED_EDGE('',*,*,#42283,.F.) ;
#58671=ORIENTED_EDGE('',*,*,#40592,.F.) ;
#58672=ORIENTED_EDGE('',*,*,#42284,.F.) ;
#58673=ORIENTED_EDGE('',*,*,#42282,.T.) ;
#58674=ORIENTED_EDGE('',*,*,#42285,.F.) ;
#58675=ORIENTED_EDGE('',*,*,#42286,.F.) ;
#58676=ORIENTED_EDGE('',*,*,#42281,.T.) ;
#58677=ORIENTED_EDGE('',*,*,#42287,.F.) ;
#58678=ORIENTED_EDGE('',*,*,#42280,.T.) ;
#58679=ORIENTED_EDGE('',*,*,#40438,.T.) ;
#58680=ORIENTED_EDGE('',*,*,#42288,.F.) ;
#58681=ORIENTED_EDGE('',*,*,#42283,.T.) ;
#58682=ORIENTED_EDGE('',*,*,#42285,.T.) ;
#58683=ORIENTED_EDGE('',*,*,#40595,.F.) ;
#58684=ORIENTED_EDGE('',*,*,#42289,.F.) ;
#58685=ORIENTED_EDGE('',*,*,#39149,.T.) ;
#58686=ORIENTED_EDGE('',*,*,#42290,.T.) ;
#58687=ORIENTED_EDGE('',*,*,#42291,.F.) ;
#58688=ORIENTED_EDGE('',*,*,#42284,.T.) ;
#58689=ORIENTED_EDGE('',*,*,#42292,.F.) ;
#58690=ORIENTED_EDGE('',*,*,#42293,.T.) ;
#58691=ORIENTED_EDGE('',*,*,#42294,.F.) ;
#58692=ORIENTED_EDGE('',*,*,#39371,.F.) ;
#58693=ORIENTED_EDGE('',*,*,#42295,.F.) ;
#58694=ORIENTED_EDGE('',*,*,#40599,.F.) ;
#58695=ORIENTED_EDGE('',*,*,#42287,.T.) ;
#58696=ORIENTED_EDGE('',*,*,#40596,.F.) ;
#58697=ORIENTED_EDGE('',*,*,#42296,.F.) ;
#58698=ORIENTED_EDGE('',*,*,#40602,.F.) ;
#58699=ORIENTED_EDGE('',*,*,#42286,.T.) ;
#58700=ORIENTED_EDGE('',*,*,#40601,.F.) ;
#58701=ORIENTED_EDGE('',*,*,#42297,.F.) ;
#58702=ORIENTED_EDGE('',*,*,#40430,.F.) ;
#58703=ORIENTED_EDGE('',*,*,#42288,.T.) ;
#58704=ORIENTED_EDGE('',*,*,#40437,.F.) ;
#58705=ORIENTED_EDGE('',*,*,#42298,.F.) ;
#58706=ORIENTED_EDGE('',*,*,#40593,.F.) ;
#58707=ORIENTED_EDGE('',*,*,#42299,.F.) ;
#58708=ORIENTED_EDGE('',*,*,#40594,.F.) ;
#58709=ORIENTED_EDGE('',*,*,#42300,.F.) ;
#58710=ORIENTED_EDGE('',*,*,#40589,.F.) ;
#58711=ORIENTED_EDGE('',*,*,#42289,.T.) ;
#58712=ORIENTED_EDGE('',*,*,#42299,.T.) ;
#58713=ORIENTED_EDGE('',*,*,#39150,.F.) ;
#58714=ORIENTED_EDGE('',*,*,#42295,.T.) ;
#58715=ORIENTED_EDGE('',*,*,#39381,.T.) ;
#58716=ORIENTED_EDGE('',*,*,#42301,.F.) ;
#58717=ORIENTED_EDGE('',*,*,#42296,.T.) ;
#58718=ORIENTED_EDGE('',*,*,#42302,.F.) ;
#58719=ORIENTED_EDGE('',*,*,#42297,.T.) ;
#58720=ORIENTED_EDGE('',*,*,#42303,.F.) ;
#58721=ORIENTED_EDGE('',*,*,#39472,.T.) ;
#58722=ORIENTED_EDGE('',*,*,#42298,.T.) ;
#58723=ORIENTED_EDGE('',*,*,#40436,.T.) ;
#58724=ORIENTED_EDGE('',*,*,#42304,.F.) ;
#58725=ORIENTED_EDGE('',*,*,#42300,.T.) ;
#58726=ORIENTED_EDGE('',*,*,#42301,.T.) ;
#58727=ORIENTED_EDGE('',*,*,#39380,.F.) ;
#58728=ORIENTED_EDGE('',*,*,#42305,.F.) ;
#58729=ORIENTED_EDGE('',*,*,#40603,.F.) ;
#58730=ORIENTED_EDGE('',*,*,#42303,.T.) ;
#58731=ORIENTED_EDGE('',*,*,#40600,.F.) ;
#58732=ORIENTED_EDGE('',*,*,#42306,.F.) ;
#58733=ORIENTED_EDGE('',*,*,#39473,.F.) ;
#58734=ORIENTED_EDGE('',*,*,#40431,.F.) ;
#58735=ORIENTED_EDGE('',*,*,#42302,.T.) ;
#58736=ORIENTED_EDGE('',*,*,#42307,.F.) ;
#58737=ORIENTED_EDGE('',*,*,#42308,.F.) ;
#58738=ORIENTED_EDGE('',*,*,#42304,.T.) ;
#58739=ORIENTED_EDGE('',*,*,#40435,.F.) ;
#58740=ORIENTED_EDGE('',*,*,#42309,.F.) ;
#58741=ORIENTED_EDGE('',*,*,#40590,.F.) ;
#58742=ORIENTED_EDGE('',*,*,#42310,.F.) ;
#58743=ORIENTED_EDGE('',*,*,#40591,.F.) ;
#58744=ORIENTED_EDGE('',*,*,#42311,.F.) ;
#58745=ORIENTED_EDGE('',*,*,#40585,.F.) ;
#58746=ORIENTED_EDGE('',*,*,#39152,.T.) ;
#58747=ORIENTED_EDGE('',*,*,#42310,.T.) ;
#58748=ORIENTED_EDGE('',*,*,#42312,.F.) ;
#58749=ORIENTED_EDGE('',*,*,#39375,.T.) ;
#58750=ORIENTED_EDGE('',*,*,#42306,.T.) ;
#58751=ORIENTED_EDGE('',*,*,#42305,.T.) ;
#58752=ORIENTED_EDGE('',*,*,#42313,.F.) ;
#58753=ORIENTED_EDGE('',*,*,#42314,.F.) ;
#58754=ORIENTED_EDGE('',*,*,#39548,.F.) ;
#58755=ORIENTED_EDGE('',*,*,#42315,.F.) ;
#58756=ORIENTED_EDGE('',*,*,#42316,.F.) ;
#58757=ORIENTED_EDGE('',*,*,#42307,.T.) ;
#58758=ORIENTED_EDGE('',*,*,#39476,.F.) ;
#58759=ORIENTED_EDGE('',*,*,#42315,.T.) ;
#58760=ORIENTED_EDGE('',*,*,#39664,.F.) ;
#58761=ORIENTED_EDGE('',*,*,#42308,.T.) ;
#58762=ORIENTED_EDGE('',*,*,#42317,.F.) ;
#58763=ORIENTED_EDGE('',*,*,#42318,.F.) ;
#58764=ORIENTED_EDGE('',*,*,#42311,.T.) ;
#58765=ORIENTED_EDGE('',*,*,#42309,.T.) ;
#58766=ORIENTED_EDGE('',*,*,#42319,.F.) ;
#58767=ORIENTED_EDGE('',*,*,#42312,.T.) ;
#58768=ORIENTED_EDGE('',*,*,#40588,.F.) ;
#58769=ORIENTED_EDGE('',*,*,#42320,.F.) ;
#58770=ORIENTED_EDGE('',*,*,#39376,.F.) ;
#58771=ORIENTED_EDGE('',*,*,#42313,.T.) ;
#58772=ORIENTED_EDGE('',*,*,#39379,.F.) ;
#58773=ORIENTED_EDGE('',*,*,#42321,.F.) ;
#58774=ORIENTED_EDGE('',*,*,#39474,.F.) ;
#58775=ORIENTED_EDGE('',*,*,#42314,.T.) ;
#58776=ORIENTED_EDGE('',*,*,#39475,.F.) ;
#58777=ORIENTED_EDGE('',*,*,#42322,.F.) ;
#58778=ORIENTED_EDGE('',*,*,#39627,.F.) ;
#58779=ORIENTED_EDGE('',*,*,#42316,.T.) ;
#58780=ORIENTED_EDGE('',*,*,#39663,.T.) ;
#58781=ORIENTED_EDGE('',*,*,#42323,.F.) ;
#58782=ORIENTED_EDGE('',*,*,#42317,.T.) ;
#58783=ORIENTED_EDGE('',*,*,#40432,.F.) ;
#58784=ORIENTED_EDGE('',*,*,#42318,.T.) ;
#58785=ORIENTED_EDGE('',*,*,#42324,.F.) ;
#58786=ORIENTED_EDGE('',*,*,#42325,.F.) ;
#58787=ORIENTED_EDGE('',*,*,#42319,.T.) ;
#58788=ORIENTED_EDGE('',*,*,#40434,.F.) ;
#58789=ORIENTED_EDGE('',*,*,#42326,.F.) ;
#58790=ORIENTED_EDGE('',*,*,#40586,.F.) ;
#58791=ORIENTED_EDGE('',*,*,#42327,.F.) ;
#58792=ORIENTED_EDGE('',*,*,#40587,.F.) ;
#58793=ORIENTED_EDGE('',*,*,#42328,.F.) ;
#58794=ORIENTED_EDGE('',*,*,#39471,.F.) ;
#58795=ORIENTED_EDGE('',*,*,#42320,.T.) ;
#58796=ORIENTED_EDGE('',*,*,#42327,.T.) ;
#58797=ORIENTED_EDGE('',*,*,#42329,.F.) ;
#58798=ORIENTED_EDGE('',*,*,#42322,.T.) ;
#58799=ORIENTED_EDGE('',*,*,#42321,.T.) ;
#58800=ORIENTED_EDGE('',*,*,#42330,.F.) ;
#58801=ORIENTED_EDGE('',*,*,#39628,.T.) ;
#58802=ORIENTED_EDGE('',*,*,#42331,.F.) ;
#58803=ORIENTED_EDGE('',*,*,#42324,.T.) ;
#58804=ORIENTED_EDGE('',*,*,#42323,.T.) ;
#58805=ORIENTED_EDGE('',*,*,#39662,.F.) ;
#58806=ORIENTED_EDGE('',*,*,#42325,.T.) ;
#58807=ORIENTED_EDGE('',*,*,#42332,.F.) ;
#58808=ORIENTED_EDGE('',*,*,#42333,.F.) ;
#58809=ORIENTED_EDGE('',*,*,#42328,.T.) ;
#58810=ORIENTED_EDGE('',*,*,#42326,.T.) ;
#58811=ORIENTED_EDGE('',*,*,#42334,.F.) ;
#58812=ORIENTED_EDGE('',*,*,#39467,.T.) ;
#58813=ORIENTED_EDGE('',*,*,#42329,.T.) ;
#58814=ORIENTED_EDGE('',*,*,#39470,.F.) ;
#58815=ORIENTED_EDGE('',*,*,#42335,.F.) ;
#58816=ORIENTED_EDGE('',*,*,#39377,.F.) ;
#58817=ORIENTED_EDGE('',*,*,#42330,.T.) ;
#58818=ORIENTED_EDGE('',*,*,#39378,.F.) ;
#58819=ORIENTED_EDGE('',*,*,#42336,.F.) ;
#58820=ORIENTED_EDGE('',*,*,#39629,.F.) ;
#58821=ORIENTED_EDGE('',*,*,#42331,.T.) ;
#58822=ORIENTED_EDGE('',*,*,#39661,.T.) ;
#58823=ORIENTED_EDGE('',*,*,#42337,.F.) ;
#58824=ORIENTED_EDGE('',*,*,#42332,.T.) ;
#58825=ORIENTED_EDGE('',*,*,#40433,.F.) ;
#58826=ORIENTED_EDGE('',*,*,#42333,.T.) ;
#58827=ORIENTED_EDGE('',*,*,#42338,.F.) ;
#58828=ORIENTED_EDGE('',*,*,#42334,.T.) ;
#58829=ORIENTED_EDGE('',*,*,#42336,.T.) ;
#58830=ORIENTED_EDGE('',*,*,#42335,.T.) ;
#58831=ORIENTED_EDGE('',*,*,#42339,.F.) ;
#58832=ORIENTED_EDGE('',*,*,#39630,.T.) ;
#58833=ORIENTED_EDGE('',*,*,#42337,.T.) ;
#58834=ORIENTED_EDGE('',*,*,#39660,.F.) ;
#58835=ORIENTED_EDGE('',*,*,#42340,.F.) ;
#58836=ORIENTED_EDGE('',*,*,#39468,.F.) ;
#58837=ORIENTED_EDGE('',*,*,#42338,.T.) ;
#58838=ORIENTED_EDGE('',*,*,#42339,.T.) ;
#58839=ORIENTED_EDGE('',*,*,#39469,.F.) ;
#58840=ORIENTED_EDGE('',*,*,#42341,.F.) ;
#58841=ORIENTED_EDGE('',*,*,#39631,.F.) ;
#58842=ORIENTED_EDGE('',*,*,#42340,.T.) ;
#58843=ORIENTED_EDGE('',*,*,#39554,.F.) ;
#58844=ORIENTED_EDGE('',*,*,#42341,.T.) ;
#58845=ORIENTED_EDGE('',*,*,#42342,.F.) ;
#58846=ORIENTED_EDGE('',*,*,#40993,.F.) ;
#58847=ORIENTED_EDGE('',*,*,#42343,.F.) ;
#58848=ORIENTED_EDGE('',*,*,#41040,.F.) ;
#58849=ORIENTED_EDGE('',*,*,#42343,.T.) ;
#58850=ORIENTED_EDGE('',*,*,#40990,.F.) ;
#58851=ORIENTED_EDGE('',*,*,#42344,.F.) ;
#58852=ORIENTED_EDGE('',*,*,#41041,.F.) ;
#58853=ORIENTED_EDGE('',*,*,#40996,.F.) ;
#58854=ORIENTED_EDGE('',*,*,#42342,.T.) ;
#58855=ORIENTED_EDGE('',*,*,#42345,.F.) ;
#58856=ORIENTED_EDGE('',*,*,#42344,.T.) ;
#58857=ORIENTED_EDGE('',*,*,#40987,.F.) ;
#58858=ORIENTED_EDGE('',*,*,#42346,.F.) ;
#58859=ORIENTED_EDGE('',*,*,#41042,.F.) ;
#58860=ORIENTED_EDGE('',*,*,#42345,.T.) ;
#58861=ORIENTED_EDGE('',*,*,#41039,.F.) ;
#58862=ORIENTED_EDGE('',*,*,#42347,.F.) ;
#58863=ORIENTED_EDGE('',*,*,#40999,.F.) ;
#58864=ORIENTED_EDGE('',*,*,#42346,.T.) ;
#58865=ORIENTED_EDGE('',*,*,#40984,.F.) ;
#58866=ORIENTED_EDGE('',*,*,#42348,.F.) ;
#58867=ORIENTED_EDGE('',*,*,#41043,.F.) ;
#58868=ORIENTED_EDGE('',*,*,#41002,.F.) ;
#58869=ORIENTED_EDGE('',*,*,#42347,.T.) ;
#58870=ORIENTED_EDGE('',*,*,#42349,.F.) ;
#58871=ORIENTED_EDGE('',*,*,#42348,.T.) ;
#58872=ORIENTED_EDGE('',*,*,#40981,.F.) ;
#58873=ORIENTED_EDGE('',*,*,#42350,.F.) ;
#58874=ORIENTED_EDGE('',*,*,#41044,.F.) ;
#58875=ORIENTED_EDGE('',*,*,#42349,.T.) ;
#58876=ORIENTED_EDGE('',*,*,#41038,.F.) ;
#58877=ORIENTED_EDGE('',*,*,#42351,.F.) ;
#58878=ORIENTED_EDGE('',*,*,#41005,.F.) ;
#58879=ORIENTED_EDGE('',*,*,#42350,.T.) ;
#58880=ORIENTED_EDGE('',*,*,#40978,.F.) ;
#58881=ORIENTED_EDGE('',*,*,#42352,.F.) ;
#58882=ORIENTED_EDGE('',*,*,#41008,.F.) ;
#58883=ORIENTED_EDGE('',*,*,#42351,.T.) ;
#58884=ORIENTED_EDGE('',*,*,#42353,.F.) ;
#58885=ORIENTED_EDGE('',*,*,#42352,.T.) ;
#58886=ORIENTED_EDGE('',*,*,#40975,.F.) ;
#58887=ORIENTED_EDGE('',*,*,#42354,.F.) ;
#58888=ORIENTED_EDGE('',*,*,#41045,.F.) ;
#58889=ORIENTED_EDGE('',*,*,#42353,.T.) ;
#58890=ORIENTED_EDGE('',*,*,#41037,.F.) ;
#58891=ORIENTED_EDGE('',*,*,#42355,.F.) ;
#58892=ORIENTED_EDGE('',*,*,#41011,.F.) ;
#58893=ORIENTED_EDGE('',*,*,#42354,.T.) ;
#58894=ORIENTED_EDGE('',*,*,#39301,.F.) ;
#58895=ORIENTED_EDGE('',*,*,#42356,.F.) ;
#58896=ORIENTED_EDGE('',*,*,#41014,.F.) ;
#58897=ORIENTED_EDGE('',*,*,#42355,.T.) ;
#58898=ORIENTED_EDGE('',*,*,#42357,.F.) ;
#58899=ORIENTED_EDGE('',*,*,#42356,.T.) ;
#58900=ORIENTED_EDGE('',*,*,#40973,.F.) ;
#58901=ORIENTED_EDGE('',*,*,#39148,.F.) ;
#58902=ORIENTED_EDGE('',*,*,#41046,.F.) ;
#58903=ORIENTED_EDGE('',*,*,#42357,.T.) ;
#58904=ORIENTED_EDGE('',*,*,#41036,.F.) ;
#58905=ORIENTED_EDGE('',*,*,#42358,.F.) ;
#58906=ORIENTED_EDGE('',*,*,#41017,.F.) ;
#58907=ORIENTED_EDGE('',*,*,#41020,.F.) ;
#58908=ORIENTED_EDGE('',*,*,#42358,.T.) ;
#58909=ORIENTED_EDGE('',*,*,#42359,.F.) ;
#58910=ORIENTED_EDGE('',*,*,#39147,.T.) ;
#58911=ORIENTED_EDGE('',*,*,#40968,.F.) ;
#58912=ORIENTED_EDGE('',*,*,#42360,.F.) ;
#58913=ORIENTED_EDGE('',*,*,#41047,.F.) ;
#58914=ORIENTED_EDGE('',*,*,#42359,.T.) ;
#58915=ORIENTED_EDGE('',*,*,#41035,.F.) ;
#58916=ORIENTED_EDGE('',*,*,#42361,.F.) ;
#58917=ORIENTED_EDGE('',*,*,#41023,.F.) ;
#58918=ORIENTED_EDGE('',*,*,#42360,.T.) ;
#58919=ORIENTED_EDGE('',*,*,#40965,.F.) ;
#58920=ORIENTED_EDGE('',*,*,#42362,.F.) ;
#58921=ORIENTED_EDGE('',*,*,#41026,.F.) ;
#58922=ORIENTED_EDGE('',*,*,#42361,.T.) ;
#58923=ORIENTED_EDGE('',*,*,#42363,.F.) ;
#58924=ORIENTED_EDGE('',*,*,#42362,.T.) ;
#58925=ORIENTED_EDGE('',*,*,#40962,.F.) ;
#58926=ORIENTED_EDGE('',*,*,#42364,.F.) ;
#58927=ORIENTED_EDGE('',*,*,#41048,.F.) ;
#58928=ORIENTED_EDGE('',*,*,#42363,.T.) ;
#58929=ORIENTED_EDGE('',*,*,#41034,.F.) ;
#58930=ORIENTED_EDGE('',*,*,#42365,.F.) ;
#58931=ORIENTED_EDGE('',*,*,#41029,.F.) ;
#58932=ORIENTED_EDGE('',*,*,#42364,.T.) ;
#58933=ORIENTED_EDGE('',*,*,#40959,.F.) ;
#58934=ORIENTED_EDGE('',*,*,#42366,.F.) ;
#58935=ORIENTED_EDGE('',*,*,#41031,.F.) ;
#58936=ORIENTED_EDGE('',*,*,#42365,.T.) ;
#58937=ORIENTED_EDGE('',*,*,#41033,.F.) ;
#58938=ORIENTED_EDGE('',*,*,#42367,.F.) ;
#58939=ORIENTED_EDGE('',*,*,#40953,.F.) ;
#58940=ORIENTED_EDGE('',*,*,#42366,.T.) ;
#58941=ORIENTED_EDGE('',*,*,#40956,.F.) ;
#58942=ORIENTED_EDGE('',*,*,#42367,.T.) ;
#58943=ORIENTED_EDGE('',*,*,#41032,.F.) ;
#58944=ORIENTED_EDGE('',*,*,#42368,.F.) ;
#58945=ORIENTED_EDGE('',*,*,#40616,.F.) ;
#58946=ORIENTED_EDGE('',*,*,#42369,.F.) ;
#58947=ORIENTED_EDGE('',*,*,#40429,.F.) ;
#58948=ORIENTED_EDGE('',*,*,#42370,.F.) ;
#58949=ORIENTED_EDGE('',*,*,#40617,.F.) ;
#58950=ORIENTED_EDGE('',*,*,#42371,.F.) ;
#58951=ORIENTED_EDGE('',*,*,#40611,.F.) ;
#58952=ORIENTED_EDGE('',*,*,#42372,.F.) ;
#58953=ORIENTED_EDGE('',*,*,#42370,.T.) ;
#58954=ORIENTED_EDGE('',*,*,#42373,.F.) ;
#58955=ORIENTED_EDGE('',*,*,#42374,.F.) ;
#58956=ORIENTED_EDGE('',*,*,#42369,.T.) ;
#58957=ORIENTED_EDGE('',*,*,#42375,.F.) ;
#58958=ORIENTED_EDGE('',*,*,#42368,.T.) ;
#58959=ORIENTED_EDGE('',*,*,#40428,.T.) ;
#58960=ORIENTED_EDGE('',*,*,#42376,.F.) ;
#58961=ORIENTED_EDGE('',*,*,#42371,.T.) ;
#58962=ORIENTED_EDGE('',*,*,#42373,.T.) ;
#58963=ORIENTED_EDGE('',*,*,#40614,.F.) ;
#58964=ORIENTED_EDGE('',*,*,#42377,.F.) ;
#58965=ORIENTED_EDGE('',*,*,#39132,.T.) ;
#58966=ORIENTED_EDGE('',*,*,#42378,.T.) ;
#58967=ORIENTED_EDGE('',*,*,#42379,.F.) ;
#58968=ORIENTED_EDGE('',*,*,#42372,.T.) ;
#58969=ORIENTED_EDGE('',*,*,#42380,.F.) ;
#58970=ORIENTED_EDGE('',*,*,#42381,.T.) ;
#58971=ORIENTED_EDGE('',*,*,#42382,.F.) ;
#58972=ORIENTED_EDGE('',*,*,#39360,.F.) ;
#58973=ORIENTED_EDGE('',*,*,#42383,.F.) ;
#58974=ORIENTED_EDGE('',*,*,#40618,.F.) ;
#58975=ORIENTED_EDGE('',*,*,#42375,.T.) ;
#58976=ORIENTED_EDGE('',*,*,#40615,.F.) ;
#58977=ORIENTED_EDGE('',*,*,#42384,.F.) ;
#58978=ORIENTED_EDGE('',*,*,#40621,.F.) ;
#58979=ORIENTED_EDGE('',*,*,#42374,.T.) ;
#58980=ORIENTED_EDGE('',*,*,#40620,.F.) ;
#58981=ORIENTED_EDGE('',*,*,#42385,.F.) ;
#58982=ORIENTED_EDGE('',*,*,#40420,.F.) ;
#58983=ORIENTED_EDGE('',*,*,#42376,.T.) ;
#58984=ORIENTED_EDGE('',*,*,#40427,.F.) ;
#58985=ORIENTED_EDGE('',*,*,#42386,.F.) ;
#58986=ORIENTED_EDGE('',*,*,#40612,.F.) ;
#58987=ORIENTED_EDGE('',*,*,#42387,.F.) ;
#58988=ORIENTED_EDGE('',*,*,#40613,.F.) ;
#58989=ORIENTED_EDGE('',*,*,#42388,.F.) ;
#58990=ORIENTED_EDGE('',*,*,#40608,.F.) ;
#58991=ORIENTED_EDGE('',*,*,#42377,.T.) ;
#58992=ORIENTED_EDGE('',*,*,#42387,.T.) ;
#58993=ORIENTED_EDGE('',*,*,#39133,.F.) ;
#58994=ORIENTED_EDGE('',*,*,#42383,.T.) ;
#58995=ORIENTED_EDGE('',*,*,#39370,.T.) ;
#58996=ORIENTED_EDGE('',*,*,#42389,.F.) ;
#58997=ORIENTED_EDGE('',*,*,#42384,.T.) ;
#58998=ORIENTED_EDGE('',*,*,#42390,.F.) ;
#58999=ORIENTED_EDGE('',*,*,#42385,.T.) ;
#59000=ORIENTED_EDGE('',*,*,#42391,.F.) ;
#59001=ORIENTED_EDGE('',*,*,#39462,.T.) ;
#59002=ORIENTED_EDGE('',*,*,#42386,.T.) ;
#59003=ORIENTED_EDGE('',*,*,#40426,.T.) ;
#59004=ORIENTED_EDGE('',*,*,#42392,.F.) ;
#59005=ORIENTED_EDGE('',*,*,#42388,.T.) ;
#59006=ORIENTED_EDGE('',*,*,#42389,.T.) ;
#59007=ORIENTED_EDGE('',*,*,#39369,.F.) ;
#59008=ORIENTED_EDGE('',*,*,#42393,.F.) ;
#59009=ORIENTED_EDGE('',*,*,#40622,.F.) ;
#59010=ORIENTED_EDGE('',*,*,#42391,.T.) ;
#59011=ORIENTED_EDGE('',*,*,#40619,.F.) ;
#59012=ORIENTED_EDGE('',*,*,#42394,.F.) ;
#59013=ORIENTED_EDGE('',*,*,#39463,.F.) ;
#59014=ORIENTED_EDGE('',*,*,#40421,.F.) ;
#59015=ORIENTED_EDGE('',*,*,#42390,.T.) ;
#59016=ORIENTED_EDGE('',*,*,#42395,.F.) ;
#59017=ORIENTED_EDGE('',*,*,#42396,.F.) ;
#59018=ORIENTED_EDGE('',*,*,#42392,.T.) ;
#59019=ORIENTED_EDGE('',*,*,#40425,.F.) ;
#59020=ORIENTED_EDGE('',*,*,#42397,.F.) ;
#59021=ORIENTED_EDGE('',*,*,#40609,.F.) ;
#59022=ORIENTED_EDGE('',*,*,#42398,.F.) ;
#59023=ORIENTED_EDGE('',*,*,#40610,.F.) ;
#59024=ORIENTED_EDGE('',*,*,#42399,.F.) ;
#59025=ORIENTED_EDGE('',*,*,#40604,.F.) ;
#59026=ORIENTED_EDGE('',*,*,#39135,.T.) ;
#59027=ORIENTED_EDGE('',*,*,#42398,.T.) ;
#59028=ORIENTED_EDGE('',*,*,#42400,.F.) ;
#59029=ORIENTED_EDGE('',*,*,#39364,.T.) ;
#59030=ORIENTED_EDGE('',*,*,#42394,.T.) ;
#59031=ORIENTED_EDGE('',*,*,#42393,.T.) ;
#59032=ORIENTED_EDGE('',*,*,#42401,.F.) ;
#59033=ORIENTED_EDGE('',*,*,#42402,.F.) ;
#59034=ORIENTED_EDGE('',*,*,#39552,.F.) ;
#59035=ORIENTED_EDGE('',*,*,#42403,.F.) ;
#59036=ORIENTED_EDGE('',*,*,#42404,.F.) ;
#59037=ORIENTED_EDGE('',*,*,#42395,.T.) ;
#59038=ORIENTED_EDGE('',*,*,#39466,.F.) ;
#59039=ORIENTED_EDGE('',*,*,#42403,.T.) ;
#59040=ORIENTED_EDGE('',*,*,#39659,.F.) ;
#59041=ORIENTED_EDGE('',*,*,#42396,.T.) ;
#59042=ORIENTED_EDGE('',*,*,#42405,.F.) ;
#59043=ORIENTED_EDGE('',*,*,#42406,.F.) ;
#59044=ORIENTED_EDGE('',*,*,#42399,.T.) ;
#59045=ORIENTED_EDGE('',*,*,#42397,.T.) ;
#59046=ORIENTED_EDGE('',*,*,#42407,.F.) ;
#59047=ORIENTED_EDGE('',*,*,#42400,.T.) ;
#59048=ORIENTED_EDGE('',*,*,#40607,.F.) ;
#59049=ORIENTED_EDGE('',*,*,#42408,.F.) ;
#59050=ORIENTED_EDGE('',*,*,#39365,.F.) ;
#59051=ORIENTED_EDGE('',*,*,#42401,.T.) ;
#59052=ORIENTED_EDGE('',*,*,#39368,.F.) ;
#59053=ORIENTED_EDGE('',*,*,#42409,.F.) ;
#59054=ORIENTED_EDGE('',*,*,#39464,.F.) ;
#59055=ORIENTED_EDGE('',*,*,#42402,.T.) ;
#59056=ORIENTED_EDGE('',*,*,#39465,.F.) ;
#59057=ORIENTED_EDGE('',*,*,#42410,.F.) ;
#59058=ORIENTED_EDGE('',*,*,#39632,.F.) ;
#59059=ORIENTED_EDGE('',*,*,#42404,.T.) ;
#59060=ORIENTED_EDGE('',*,*,#39658,.T.) ;
#59061=ORIENTED_EDGE('',*,*,#42411,.F.) ;
#59062=ORIENTED_EDGE('',*,*,#42405,.T.) ;
#59063=ORIENTED_EDGE('',*,*,#40422,.F.) ;
#59064=ORIENTED_EDGE('',*,*,#42406,.T.) ;
#59065=ORIENTED_EDGE('',*,*,#42412,.F.) ;
#59066=ORIENTED_EDGE('',*,*,#42413,.F.) ;
#59067=ORIENTED_EDGE('',*,*,#42407,.T.) ;
#59068=ORIENTED_EDGE('',*,*,#40424,.F.) ;
#59069=ORIENTED_EDGE('',*,*,#42414,.F.) ;
#59070=ORIENTED_EDGE('',*,*,#40605,.F.) ;
#59071=ORIENTED_EDGE('',*,*,#42415,.F.) ;
#59072=ORIENTED_EDGE('',*,*,#40606,.F.) ;
#59073=ORIENTED_EDGE('',*,*,#42416,.F.) ;
#59074=ORIENTED_EDGE('',*,*,#39461,.F.) ;
#59075=ORIENTED_EDGE('',*,*,#42408,.T.) ;
#59076=ORIENTED_EDGE('',*,*,#42415,.T.) ;
#59077=ORIENTED_EDGE('',*,*,#42417,.F.) ;
#59078=ORIENTED_EDGE('',*,*,#42410,.T.) ;
#59079=ORIENTED_EDGE('',*,*,#42409,.T.) ;
#59080=ORIENTED_EDGE('',*,*,#42418,.F.) ;
#59081=ORIENTED_EDGE('',*,*,#39633,.T.) ;
#59082=ORIENTED_EDGE('',*,*,#42419,.F.) ;
#59083=ORIENTED_EDGE('',*,*,#42412,.T.) ;
#59084=ORIENTED_EDGE('',*,*,#42411,.T.) ;
#59085=ORIENTED_EDGE('',*,*,#39657,.F.) ;
#59086=ORIENTED_EDGE('',*,*,#42413,.T.) ;
#59087=ORIENTED_EDGE('',*,*,#42420,.F.) ;
#59088=ORIENTED_EDGE('',*,*,#42421,.F.) ;
#59089=ORIENTED_EDGE('',*,*,#42416,.T.) ;
#59090=ORIENTED_EDGE('',*,*,#42414,.T.) ;
#59091=ORIENTED_EDGE('',*,*,#42422,.F.) ;
#59092=ORIENTED_EDGE('',*,*,#39457,.T.) ;
#59093=ORIENTED_EDGE('',*,*,#42417,.T.) ;
#59094=ORIENTED_EDGE('',*,*,#39460,.F.) ;
#59095=ORIENTED_EDGE('',*,*,#42423,.F.) ;
#59096=ORIENTED_EDGE('',*,*,#39366,.F.) ;
#59097=ORIENTED_EDGE('',*,*,#42418,.T.) ;
#59098=ORIENTED_EDGE('',*,*,#39367,.F.) ;
#59099=ORIENTED_EDGE('',*,*,#42424,.F.) ;
#59100=ORIENTED_EDGE('',*,*,#39634,.F.) ;
#59101=ORIENTED_EDGE('',*,*,#42419,.T.) ;
#59102=ORIENTED_EDGE('',*,*,#39656,.T.) ;
#59103=ORIENTED_EDGE('',*,*,#42425,.F.) ;
#59104=ORIENTED_EDGE('',*,*,#42420,.T.) ;
#59105=ORIENTED_EDGE('',*,*,#40423,.F.) ;
#59106=ORIENTED_EDGE('',*,*,#42421,.T.) ;
#59107=ORIENTED_EDGE('',*,*,#42426,.F.) ;
#59108=ORIENTED_EDGE('',*,*,#42422,.T.) ;
#59109=ORIENTED_EDGE('',*,*,#42424,.T.) ;
#59110=ORIENTED_EDGE('',*,*,#42423,.T.) ;
#59111=ORIENTED_EDGE('',*,*,#42427,.F.) ;
#59112=ORIENTED_EDGE('',*,*,#39635,.T.) ;
#59113=ORIENTED_EDGE('',*,*,#42425,.T.) ;
#59114=ORIENTED_EDGE('',*,*,#39655,.F.) ;
#59115=ORIENTED_EDGE('',*,*,#42428,.F.) ;
#59116=ORIENTED_EDGE('',*,*,#39458,.F.) ;
#59117=ORIENTED_EDGE('',*,*,#42426,.T.) ;
#59118=ORIENTED_EDGE('',*,*,#42427,.T.) ;
#59119=ORIENTED_EDGE('',*,*,#39459,.F.) ;
#59120=ORIENTED_EDGE('',*,*,#42429,.F.) ;
#59121=ORIENTED_EDGE('',*,*,#39636,.F.) ;
#59122=ORIENTED_EDGE('',*,*,#42428,.T.) ;
#59123=ORIENTED_EDGE('',*,*,#39558,.F.) ;
#59124=ORIENTED_EDGE('',*,*,#42429,.T.) ;
#59125=ORIENTED_EDGE('',*,*,#42430,.F.) ;
#59126=ORIENTED_EDGE('',*,*,#40896,.F.) ;
#59127=ORIENTED_EDGE('',*,*,#42431,.F.) ;
#59128=ORIENTED_EDGE('',*,*,#40943,.F.) ;
#59129=ORIENTED_EDGE('',*,*,#42431,.T.) ;
#59130=ORIENTED_EDGE('',*,*,#40893,.F.) ;
#59131=ORIENTED_EDGE('',*,*,#42432,.F.) ;
#59132=ORIENTED_EDGE('',*,*,#40944,.F.) ;
#59133=ORIENTED_EDGE('',*,*,#40899,.F.) ;
#59134=ORIENTED_EDGE('',*,*,#42430,.T.) ;
#59135=ORIENTED_EDGE('',*,*,#42433,.F.) ;
#59136=ORIENTED_EDGE('',*,*,#42432,.T.) ;
#59137=ORIENTED_EDGE('',*,*,#40890,.F.) ;
#59138=ORIENTED_EDGE('',*,*,#42434,.F.) ;
#59139=ORIENTED_EDGE('',*,*,#40945,.F.) ;
#59140=ORIENTED_EDGE('',*,*,#42433,.T.) ;
#59141=ORIENTED_EDGE('',*,*,#40942,.F.) ;
#59142=ORIENTED_EDGE('',*,*,#42435,.F.) ;
#59143=ORIENTED_EDGE('',*,*,#40902,.F.) ;
#59144=ORIENTED_EDGE('',*,*,#42434,.T.) ;
#59145=ORIENTED_EDGE('',*,*,#40887,.F.) ;
#59146=ORIENTED_EDGE('',*,*,#42436,.F.) ;
#59147=ORIENTED_EDGE('',*,*,#40946,.F.) ;
#59148=ORIENTED_EDGE('',*,*,#40905,.F.) ;
#59149=ORIENTED_EDGE('',*,*,#42435,.T.) ;
#59150=ORIENTED_EDGE('',*,*,#42437,.F.) ;
#59151=ORIENTED_EDGE('',*,*,#42436,.T.) ;
#59152=ORIENTED_EDGE('',*,*,#40884,.F.) ;
#59153=ORIENTED_EDGE('',*,*,#42438,.F.) ;
#59154=ORIENTED_EDGE('',*,*,#40947,.F.) ;
#59155=ORIENTED_EDGE('',*,*,#42437,.T.) ;
#59156=ORIENTED_EDGE('',*,*,#40941,.F.) ;
#59157=ORIENTED_EDGE('',*,*,#42439,.F.) ;
#59158=ORIENTED_EDGE('',*,*,#40908,.F.) ;
#59159=ORIENTED_EDGE('',*,*,#42438,.T.) ;
#59160=ORIENTED_EDGE('',*,*,#40881,.F.) ;
#59161=ORIENTED_EDGE('',*,*,#42440,.F.) ;
#59162=ORIENTED_EDGE('',*,*,#40911,.F.) ;
#59163=ORIENTED_EDGE('',*,*,#42439,.T.) ;
#59164=ORIENTED_EDGE('',*,*,#42441,.F.) ;
#59165=ORIENTED_EDGE('',*,*,#42440,.T.) ;
#59166=ORIENTED_EDGE('',*,*,#40878,.F.) ;
#59167=ORIENTED_EDGE('',*,*,#42442,.F.) ;
#59168=ORIENTED_EDGE('',*,*,#40948,.F.) ;
#59169=ORIENTED_EDGE('',*,*,#42441,.T.) ;
#59170=ORIENTED_EDGE('',*,*,#40940,.F.) ;
#59171=ORIENTED_EDGE('',*,*,#42443,.F.) ;
#59172=ORIENTED_EDGE('',*,*,#40914,.F.) ;
#59173=ORIENTED_EDGE('',*,*,#42442,.T.) ;
#59174=ORIENTED_EDGE('',*,*,#39304,.F.) ;
#59175=ORIENTED_EDGE('',*,*,#42444,.F.) ;
#59176=ORIENTED_EDGE('',*,*,#40917,.F.) ;
#59177=ORIENTED_EDGE('',*,*,#42443,.T.) ;
#59178=ORIENTED_EDGE('',*,*,#42445,.F.) ;
#59179=ORIENTED_EDGE('',*,*,#42444,.T.) ;
#59180=ORIENTED_EDGE('',*,*,#40876,.F.) ;
#59181=ORIENTED_EDGE('',*,*,#39131,.F.) ;
#59182=ORIENTED_EDGE('',*,*,#40949,.F.) ;
#59183=ORIENTED_EDGE('',*,*,#42445,.T.) ;
#59184=ORIENTED_EDGE('',*,*,#40939,.F.) ;
#59185=ORIENTED_EDGE('',*,*,#42446,.F.) ;
#59186=ORIENTED_EDGE('',*,*,#40920,.F.) ;
#59187=ORIENTED_EDGE('',*,*,#40923,.F.) ;
#59188=ORIENTED_EDGE('',*,*,#42446,.T.) ;
#59189=ORIENTED_EDGE('',*,*,#42447,.F.) ;
#59190=ORIENTED_EDGE('',*,*,#39130,.T.) ;
#59191=ORIENTED_EDGE('',*,*,#40871,.F.) ;
#59192=ORIENTED_EDGE('',*,*,#42448,.F.) ;
#59193=ORIENTED_EDGE('',*,*,#40950,.F.) ;
#59194=ORIENTED_EDGE('',*,*,#42447,.T.) ;
#59195=ORIENTED_EDGE('',*,*,#40938,.F.) ;
#59196=ORIENTED_EDGE('',*,*,#42449,.F.) ;
#59197=ORIENTED_EDGE('',*,*,#40926,.F.) ;
#59198=ORIENTED_EDGE('',*,*,#42448,.T.) ;
#59199=ORIENTED_EDGE('',*,*,#40868,.F.) ;
#59200=ORIENTED_EDGE('',*,*,#42450,.F.) ;
#59201=ORIENTED_EDGE('',*,*,#40929,.F.) ;
#59202=ORIENTED_EDGE('',*,*,#42449,.T.) ;
#59203=ORIENTED_EDGE('',*,*,#42451,.F.) ;
#59204=ORIENTED_EDGE('',*,*,#42450,.T.) ;
#59205=ORIENTED_EDGE('',*,*,#40865,.F.) ;
#59206=ORIENTED_EDGE('',*,*,#42452,.F.) ;
#59207=ORIENTED_EDGE('',*,*,#40951,.F.) ;
#59208=ORIENTED_EDGE('',*,*,#42451,.T.) ;
#59209=ORIENTED_EDGE('',*,*,#40937,.F.) ;
#59210=ORIENTED_EDGE('',*,*,#42453,.F.) ;
#59211=ORIENTED_EDGE('',*,*,#40932,.F.) ;
#59212=ORIENTED_EDGE('',*,*,#42452,.T.) ;
#59213=ORIENTED_EDGE('',*,*,#40862,.F.) ;
#59214=ORIENTED_EDGE('',*,*,#42454,.F.) ;
#59215=ORIENTED_EDGE('',*,*,#40934,.F.) ;
#59216=ORIENTED_EDGE('',*,*,#42453,.T.) ;
#59217=ORIENTED_EDGE('',*,*,#40936,.F.) ;
#59218=ORIENTED_EDGE('',*,*,#42455,.F.) ;
#59219=ORIENTED_EDGE('',*,*,#40856,.F.) ;
#59220=ORIENTED_EDGE('',*,*,#42454,.T.) ;
#59221=ORIENTED_EDGE('',*,*,#40859,.F.) ;
#59222=ORIENTED_EDGE('',*,*,#42455,.T.) ;
#59223=ORIENTED_EDGE('',*,*,#40935,.F.) ;
#59224=ORIENTED_EDGE('',*,*,#42456,.F.) ;
#59225=ORIENTED_EDGE('',*,*,#40635,.F.) ;
#59226=ORIENTED_EDGE('',*,*,#42457,.F.) ;
#59227=ORIENTED_EDGE('',*,*,#40419,.F.) ;
#59228=ORIENTED_EDGE('',*,*,#42458,.F.) ;
#59229=ORIENTED_EDGE('',*,*,#40636,.F.) ;
#59230=ORIENTED_EDGE('',*,*,#42459,.F.) ;
#59231=ORIENTED_EDGE('',*,*,#40630,.F.) ;
#59232=ORIENTED_EDGE('',*,*,#42460,.F.) ;
#59233=ORIENTED_EDGE('',*,*,#42458,.T.) ;
#59234=ORIENTED_EDGE('',*,*,#42461,.F.) ;
#59235=ORIENTED_EDGE('',*,*,#42462,.F.) ;
#59236=ORIENTED_EDGE('',*,*,#42457,.T.) ;
#59237=ORIENTED_EDGE('',*,*,#42463,.F.) ;
#59238=ORIENTED_EDGE('',*,*,#42456,.T.) ;
#59239=ORIENTED_EDGE('',*,*,#40418,.T.) ;
#59240=ORIENTED_EDGE('',*,*,#42464,.F.) ;
#59241=ORIENTED_EDGE('',*,*,#42459,.T.) ;
#59242=ORIENTED_EDGE('',*,*,#42461,.T.) ;
#59243=ORIENTED_EDGE('',*,*,#40633,.F.) ;
#59244=ORIENTED_EDGE('',*,*,#42465,.F.) ;
#59245=ORIENTED_EDGE('',*,*,#39115,.T.) ;
#59246=ORIENTED_EDGE('',*,*,#42466,.T.) ;
#59247=ORIENTED_EDGE('',*,*,#42467,.F.) ;
#59248=ORIENTED_EDGE('',*,*,#42460,.T.) ;
#59249=ORIENTED_EDGE('',*,*,#42468,.F.) ;
#59250=ORIENTED_EDGE('',*,*,#42469,.T.) ;
#59251=ORIENTED_EDGE('',*,*,#42470,.F.) ;
#59252=ORIENTED_EDGE('',*,*,#39349,.F.) ;
#59253=ORIENTED_EDGE('',*,*,#42471,.F.) ;
#59254=ORIENTED_EDGE('',*,*,#40637,.F.) ;
#59255=ORIENTED_EDGE('',*,*,#42463,.T.) ;
#59256=ORIENTED_EDGE('',*,*,#40634,.F.) ;
#59257=ORIENTED_EDGE('',*,*,#42472,.F.) ;
#59258=ORIENTED_EDGE('',*,*,#40640,.F.) ;
#59259=ORIENTED_EDGE('',*,*,#42462,.T.) ;
#59260=ORIENTED_EDGE('',*,*,#40639,.F.) ;
#59261=ORIENTED_EDGE('',*,*,#42473,.F.) ;
#59262=ORIENTED_EDGE('',*,*,#40410,.F.) ;
#59263=ORIENTED_EDGE('',*,*,#42464,.T.) ;
#59264=ORIENTED_EDGE('',*,*,#40417,.F.) ;
#59265=ORIENTED_EDGE('',*,*,#42474,.F.) ;
#59266=ORIENTED_EDGE('',*,*,#40631,.F.) ;
#59267=ORIENTED_EDGE('',*,*,#42475,.F.) ;
#59268=ORIENTED_EDGE('',*,*,#40632,.F.) ;
#59269=ORIENTED_EDGE('',*,*,#42476,.F.) ;
#59270=ORIENTED_EDGE('',*,*,#40627,.F.) ;
#59271=ORIENTED_EDGE('',*,*,#42465,.T.) ;
#59272=ORIENTED_EDGE('',*,*,#42475,.T.) ;
#59273=ORIENTED_EDGE('',*,*,#39116,.F.) ;
#59274=ORIENTED_EDGE('',*,*,#42471,.T.) ;
#59275=ORIENTED_EDGE('',*,*,#39359,.T.) ;
#59276=ORIENTED_EDGE('',*,*,#42477,.F.) ;
#59277=ORIENTED_EDGE('',*,*,#42472,.T.) ;
#59278=ORIENTED_EDGE('',*,*,#42478,.F.) ;
#59279=ORIENTED_EDGE('',*,*,#42473,.T.) ;
#59280=ORIENTED_EDGE('',*,*,#42479,.F.) ;
#59281=ORIENTED_EDGE('',*,*,#39452,.T.) ;
#59282=ORIENTED_EDGE('',*,*,#42474,.T.) ;
#59283=ORIENTED_EDGE('',*,*,#40416,.T.) ;
#59284=ORIENTED_EDGE('',*,*,#42480,.F.) ;
#59285=ORIENTED_EDGE('',*,*,#42476,.T.) ;
#59286=ORIENTED_EDGE('',*,*,#42477,.T.) ;
#59287=ORIENTED_EDGE('',*,*,#39358,.F.) ;
#59288=ORIENTED_EDGE('',*,*,#42481,.F.) ;
#59289=ORIENTED_EDGE('',*,*,#40641,.F.) ;
#59290=ORIENTED_EDGE('',*,*,#42479,.T.) ;
#59291=ORIENTED_EDGE('',*,*,#40638,.F.) ;
#59292=ORIENTED_EDGE('',*,*,#42482,.F.) ;
#59293=ORIENTED_EDGE('',*,*,#39453,.F.) ;
#59294=ORIENTED_EDGE('',*,*,#40411,.F.) ;
#59295=ORIENTED_EDGE('',*,*,#42478,.T.) ;
#59296=ORIENTED_EDGE('',*,*,#42483,.F.) ;
#59297=ORIENTED_EDGE('',*,*,#42484,.F.) ;
#59298=ORIENTED_EDGE('',*,*,#42480,.T.) ;
#59299=ORIENTED_EDGE('',*,*,#40415,.F.) ;
#59300=ORIENTED_EDGE('',*,*,#42485,.F.) ;
#59301=ORIENTED_EDGE('',*,*,#40628,.F.) ;
#59302=ORIENTED_EDGE('',*,*,#42486,.F.) ;
#59303=ORIENTED_EDGE('',*,*,#40629,.F.) ;
#59304=ORIENTED_EDGE('',*,*,#42487,.F.) ;
#59305=ORIENTED_EDGE('',*,*,#40623,.F.) ;
#59306=ORIENTED_EDGE('',*,*,#39118,.T.) ;
#59307=ORIENTED_EDGE('',*,*,#42486,.T.) ;
#59308=ORIENTED_EDGE('',*,*,#42488,.F.) ;
#59309=ORIENTED_EDGE('',*,*,#39353,.T.) ;
#59310=ORIENTED_EDGE('',*,*,#42482,.T.) ;
#59311=ORIENTED_EDGE('',*,*,#42481,.T.) ;
#59312=ORIENTED_EDGE('',*,*,#42489,.F.) ;
#59313=ORIENTED_EDGE('',*,*,#42490,.F.) ;
#59314=ORIENTED_EDGE('',*,*,#39556,.F.) ;
#59315=ORIENTED_EDGE('',*,*,#42491,.F.) ;
#59316=ORIENTED_EDGE('',*,*,#42492,.F.) ;
#59317=ORIENTED_EDGE('',*,*,#42483,.T.) ;
#59318=ORIENTED_EDGE('',*,*,#39456,.F.) ;
#59319=ORIENTED_EDGE('',*,*,#42491,.T.) ;
#59320=ORIENTED_EDGE('',*,*,#39654,.F.) ;
#59321=ORIENTED_EDGE('',*,*,#42484,.T.) ;
#59322=ORIENTED_EDGE('',*,*,#42493,.F.) ;
#59323=ORIENTED_EDGE('',*,*,#42494,.F.) ;
#59324=ORIENTED_EDGE('',*,*,#42487,.T.) ;
#59325=ORIENTED_EDGE('',*,*,#42485,.T.) ;
#59326=ORIENTED_EDGE('',*,*,#42495,.F.) ;
#59327=ORIENTED_EDGE('',*,*,#42488,.T.) ;
#59328=ORIENTED_EDGE('',*,*,#40626,.F.) ;
#59329=ORIENTED_EDGE('',*,*,#42496,.F.) ;
#59330=ORIENTED_EDGE('',*,*,#39354,.F.) ;
#59331=ORIENTED_EDGE('',*,*,#42489,.T.) ;
#59332=ORIENTED_EDGE('',*,*,#39357,.F.) ;
#59333=ORIENTED_EDGE('',*,*,#42497,.F.) ;
#59334=ORIENTED_EDGE('',*,*,#39454,.F.) ;
#59335=ORIENTED_EDGE('',*,*,#42490,.T.) ;
#59336=ORIENTED_EDGE('',*,*,#39455,.F.) ;
#59337=ORIENTED_EDGE('',*,*,#42498,.F.) ;
#59338=ORIENTED_EDGE('',*,*,#39637,.F.) ;
#59339=ORIENTED_EDGE('',*,*,#42492,.T.) ;
#59340=ORIENTED_EDGE('',*,*,#39653,.T.) ;
#59341=ORIENTED_EDGE('',*,*,#42499,.F.) ;
#59342=ORIENTED_EDGE('',*,*,#42493,.T.) ;
#59343=ORIENTED_EDGE('',*,*,#40412,.F.) ;
#59344=ORIENTED_EDGE('',*,*,#42494,.T.) ;
#59345=ORIENTED_EDGE('',*,*,#42500,.F.) ;
#59346=ORIENTED_EDGE('',*,*,#42501,.F.) ;
#59347=ORIENTED_EDGE('',*,*,#42495,.T.) ;
#59348=ORIENTED_EDGE('',*,*,#40414,.F.) ;
#59349=ORIENTED_EDGE('',*,*,#42502,.F.) ;
#59350=ORIENTED_EDGE('',*,*,#40624,.F.) ;
#59351=ORIENTED_EDGE('',*,*,#42503,.F.) ;
#59352=ORIENTED_EDGE('',*,*,#40625,.F.) ;
#59353=ORIENTED_EDGE('',*,*,#42504,.F.) ;
#59354=ORIENTED_EDGE('',*,*,#39451,.F.) ;
#59355=ORIENTED_EDGE('',*,*,#42496,.T.) ;
#59356=ORIENTED_EDGE('',*,*,#42503,.T.) ;
#59357=ORIENTED_EDGE('',*,*,#42505,.F.) ;
#59358=ORIENTED_EDGE('',*,*,#42498,.T.) ;
#59359=ORIENTED_EDGE('',*,*,#42497,.T.) ;
#59360=ORIENTED_EDGE('',*,*,#42506,.F.) ;
#59361=ORIENTED_EDGE('',*,*,#39638,.T.) ;
#59362=ORIENTED_EDGE('',*,*,#42507,.F.) ;
#59363=ORIENTED_EDGE('',*,*,#42500,.T.) ;
#59364=ORIENTED_EDGE('',*,*,#42499,.T.) ;
#59365=ORIENTED_EDGE('',*,*,#39652,.F.) ;
#59366=ORIENTED_EDGE('',*,*,#42501,.T.) ;
#59367=ORIENTED_EDGE('',*,*,#42508,.F.) ;
#59368=ORIENTED_EDGE('',*,*,#42509,.F.) ;
#59369=ORIENTED_EDGE('',*,*,#42504,.T.) ;
#59370=ORIENTED_EDGE('',*,*,#42502,.T.) ;
#59371=ORIENTED_EDGE('',*,*,#42510,.F.) ;
#59372=ORIENTED_EDGE('',*,*,#39447,.T.) ;
#59373=ORIENTED_EDGE('',*,*,#42505,.T.) ;
#59374=ORIENTED_EDGE('',*,*,#39450,.F.) ;
#59375=ORIENTED_EDGE('',*,*,#42511,.F.) ;
#59376=ORIENTED_EDGE('',*,*,#39355,.F.) ;
#59377=ORIENTED_EDGE('',*,*,#42506,.T.) ;
#59378=ORIENTED_EDGE('',*,*,#39356,.F.) ;
#59379=ORIENTED_EDGE('',*,*,#42512,.F.) ;
#59380=ORIENTED_EDGE('',*,*,#39639,.F.) ;
#59381=ORIENTED_EDGE('',*,*,#42507,.T.) ;
#59382=ORIENTED_EDGE('',*,*,#39651,.T.) ;
#59383=ORIENTED_EDGE('',*,*,#42513,.F.) ;
#59384=ORIENTED_EDGE('',*,*,#42508,.T.) ;
#59385=ORIENTED_EDGE('',*,*,#40413,.F.) ;
#59386=ORIENTED_EDGE('',*,*,#42509,.T.) ;
#59387=ORIENTED_EDGE('',*,*,#42514,.F.) ;
#59388=ORIENTED_EDGE('',*,*,#42510,.T.) ;
#59389=ORIENTED_EDGE('',*,*,#42512,.T.) ;
#59390=ORIENTED_EDGE('',*,*,#42511,.T.) ;
#59391=ORIENTED_EDGE('',*,*,#42515,.F.) ;
#59392=ORIENTED_EDGE('',*,*,#39640,.T.) ;
#59393=ORIENTED_EDGE('',*,*,#42513,.T.) ;
#59394=ORIENTED_EDGE('',*,*,#39650,.F.) ;
#59395=ORIENTED_EDGE('',*,*,#42516,.F.) ;
#59396=ORIENTED_EDGE('',*,*,#39448,.F.) ;
#59397=ORIENTED_EDGE('',*,*,#42514,.T.) ;
#59398=ORIENTED_EDGE('',*,*,#42515,.T.) ;
#59399=ORIENTED_EDGE('',*,*,#39449,.F.) ;
#59400=ORIENTED_EDGE('',*,*,#42517,.F.) ;
#59401=ORIENTED_EDGE('',*,*,#39641,.F.) ;
#59402=ORIENTED_EDGE('',*,*,#42516,.T.) ;
#59403=ORIENTED_EDGE('',*,*,#39562,.F.) ;
#59404=ORIENTED_EDGE('',*,*,#42517,.T.) ;
#59405=ORIENTED_EDGE('',*,*,#42518,.F.) ;
#59406=ORIENTED_EDGE('',*,*,#40799,.F.) ;
#59407=ORIENTED_EDGE('',*,*,#42519,.F.) ;
#59408=ORIENTED_EDGE('',*,*,#40846,.F.) ;
#59409=ORIENTED_EDGE('',*,*,#42519,.T.) ;
#59410=ORIENTED_EDGE('',*,*,#40796,.F.) ;
#59411=ORIENTED_EDGE('',*,*,#42520,.F.) ;
#59412=ORIENTED_EDGE('',*,*,#40847,.F.) ;
#59413=ORIENTED_EDGE('',*,*,#40802,.F.) ;
#59414=ORIENTED_EDGE('',*,*,#42518,.T.) ;
#59415=ORIENTED_EDGE('',*,*,#42521,.F.) ;
#59416=ORIENTED_EDGE('',*,*,#42520,.T.) ;
#59417=ORIENTED_EDGE('',*,*,#40793,.F.) ;
#59418=ORIENTED_EDGE('',*,*,#42522,.F.) ;
#59419=ORIENTED_EDGE('',*,*,#40848,.F.) ;
#59420=ORIENTED_EDGE('',*,*,#42521,.T.) ;
#59421=ORIENTED_EDGE('',*,*,#40845,.F.) ;
#59422=ORIENTED_EDGE('',*,*,#42523,.F.) ;
#59423=ORIENTED_EDGE('',*,*,#40805,.F.) ;
#59424=ORIENTED_EDGE('',*,*,#42522,.T.) ;
#59425=ORIENTED_EDGE('',*,*,#40790,.F.) ;
#59426=ORIENTED_EDGE('',*,*,#42524,.F.) ;
#59427=ORIENTED_EDGE('',*,*,#40849,.F.) ;
#59428=ORIENTED_EDGE('',*,*,#40808,.F.) ;
#59429=ORIENTED_EDGE('',*,*,#42523,.T.) ;
#59430=ORIENTED_EDGE('',*,*,#42525,.F.) ;
#59431=ORIENTED_EDGE('',*,*,#42524,.T.) ;
#59432=ORIENTED_EDGE('',*,*,#40787,.F.) ;
#59433=ORIENTED_EDGE('',*,*,#42526,.F.) ;
#59434=ORIENTED_EDGE('',*,*,#40850,.F.) ;
#59435=ORIENTED_EDGE('',*,*,#42525,.T.) ;
#59436=ORIENTED_EDGE('',*,*,#40844,.F.) ;
#59437=ORIENTED_EDGE('',*,*,#42527,.F.) ;
#59438=ORIENTED_EDGE('',*,*,#40811,.F.) ;
#59439=ORIENTED_EDGE('',*,*,#42526,.T.) ;
#59440=ORIENTED_EDGE('',*,*,#40784,.F.) ;
#59441=ORIENTED_EDGE('',*,*,#42528,.F.) ;
#59442=ORIENTED_EDGE('',*,*,#40814,.F.) ;
#59443=ORIENTED_EDGE('',*,*,#42527,.T.) ;
#59444=ORIENTED_EDGE('',*,*,#42529,.F.) ;
#59445=ORIENTED_EDGE('',*,*,#42528,.T.) ;
#59446=ORIENTED_EDGE('',*,*,#40781,.F.) ;
#59447=ORIENTED_EDGE('',*,*,#42530,.F.) ;
#59448=ORIENTED_EDGE('',*,*,#40851,.F.) ;
#59449=ORIENTED_EDGE('',*,*,#42529,.T.) ;
#59450=ORIENTED_EDGE('',*,*,#40843,.F.) ;
#59451=ORIENTED_EDGE('',*,*,#42531,.F.) ;
#59452=ORIENTED_EDGE('',*,*,#40817,.F.) ;
#59453=ORIENTED_EDGE('',*,*,#42530,.T.) ;
#59454=ORIENTED_EDGE('',*,*,#39307,.F.) ;
#59455=ORIENTED_EDGE('',*,*,#42532,.F.) ;
#59456=ORIENTED_EDGE('',*,*,#40820,.F.) ;
#59457=ORIENTED_EDGE('',*,*,#42531,.T.) ;
#59458=ORIENTED_EDGE('',*,*,#42533,.F.) ;
#59459=ORIENTED_EDGE('',*,*,#42532,.T.) ;
#59460=ORIENTED_EDGE('',*,*,#40779,.F.) ;
#59461=ORIENTED_EDGE('',*,*,#39114,.F.) ;
#59462=ORIENTED_EDGE('',*,*,#40852,.F.) ;
#59463=ORIENTED_EDGE('',*,*,#42533,.T.) ;
#59464=ORIENTED_EDGE('',*,*,#40842,.F.) ;
#59465=ORIENTED_EDGE('',*,*,#42534,.F.) ;
#59466=ORIENTED_EDGE('',*,*,#40823,.F.) ;
#59467=ORIENTED_EDGE('',*,*,#40826,.F.) ;
#59468=ORIENTED_EDGE('',*,*,#42534,.T.) ;
#59469=ORIENTED_EDGE('',*,*,#42535,.F.) ;
#59470=ORIENTED_EDGE('',*,*,#39113,.T.) ;
#59471=ORIENTED_EDGE('',*,*,#40774,.F.) ;
#59472=ORIENTED_EDGE('',*,*,#42536,.F.) ;
#59473=ORIENTED_EDGE('',*,*,#40853,.F.) ;
#59474=ORIENTED_EDGE('',*,*,#42535,.T.) ;
#59475=ORIENTED_EDGE('',*,*,#40841,.F.) ;
#59476=ORIENTED_EDGE('',*,*,#42537,.F.) ;
#59477=ORIENTED_EDGE('',*,*,#40829,.F.) ;
#59478=ORIENTED_EDGE('',*,*,#42536,.T.) ;
#59479=ORIENTED_EDGE('',*,*,#40771,.F.) ;
#59480=ORIENTED_EDGE('',*,*,#42538,.F.) ;
#59481=ORIENTED_EDGE('',*,*,#40832,.F.) ;
#59482=ORIENTED_EDGE('',*,*,#42537,.T.) ;
#59483=ORIENTED_EDGE('',*,*,#42539,.F.) ;
#59484=ORIENTED_EDGE('',*,*,#42538,.T.) ;
#59485=ORIENTED_EDGE('',*,*,#40768,.F.) ;
#59486=ORIENTED_EDGE('',*,*,#42540,.F.) ;
#59487=ORIENTED_EDGE('',*,*,#40854,.F.) ;
#59488=ORIENTED_EDGE('',*,*,#42539,.T.) ;
#59489=ORIENTED_EDGE('',*,*,#40840,.F.) ;
#59490=ORIENTED_EDGE('',*,*,#42541,.F.) ;
#59491=ORIENTED_EDGE('',*,*,#40835,.F.) ;
#59492=ORIENTED_EDGE('',*,*,#42540,.T.) ;
#59493=ORIENTED_EDGE('',*,*,#40765,.F.) ;
#59494=ORIENTED_EDGE('',*,*,#42542,.F.) ;
#59495=ORIENTED_EDGE('',*,*,#40837,.F.) ;
#59496=ORIENTED_EDGE('',*,*,#42541,.T.) ;
#59497=ORIENTED_EDGE('',*,*,#40839,.F.) ;
#59498=ORIENTED_EDGE('',*,*,#42543,.F.) ;
#59499=ORIENTED_EDGE('',*,*,#40759,.F.) ;
#59500=ORIENTED_EDGE('',*,*,#42542,.T.) ;
#59501=ORIENTED_EDGE('',*,*,#40762,.F.) ;
#59502=ORIENTED_EDGE('',*,*,#42543,.T.) ;
#59503=ORIENTED_EDGE('',*,*,#40838,.F.) ;
#59504=ORIENTED_EDGE('',*,*,#42544,.F.) ;
#59505=ORIENTED_EDGE('',*,*,#40654,.F.) ;
#59506=ORIENTED_EDGE('',*,*,#42545,.F.) ;
#59507=ORIENTED_EDGE('',*,*,#40409,.F.) ;
#59508=ORIENTED_EDGE('',*,*,#42546,.F.) ;
#59509=ORIENTED_EDGE('',*,*,#40655,.F.) ;
#59510=ORIENTED_EDGE('',*,*,#42547,.F.) ;
#59511=ORIENTED_EDGE('',*,*,#40649,.F.) ;
#59512=ORIENTED_EDGE('',*,*,#42548,.F.) ;
#59513=ORIENTED_EDGE('',*,*,#42546,.T.) ;
#59514=ORIENTED_EDGE('',*,*,#42549,.F.) ;
#59515=ORIENTED_EDGE('',*,*,#42550,.F.) ;
#59516=ORIENTED_EDGE('',*,*,#42545,.T.) ;
#59517=ORIENTED_EDGE('',*,*,#42551,.F.) ;
#59518=ORIENTED_EDGE('',*,*,#42544,.T.) ;
#59519=ORIENTED_EDGE('',*,*,#40408,.T.) ;
#59520=ORIENTED_EDGE('',*,*,#42552,.F.) ;
#59521=ORIENTED_EDGE('',*,*,#42547,.T.) ;
#59522=ORIENTED_EDGE('',*,*,#42549,.T.) ;
#59523=ORIENTED_EDGE('',*,*,#40652,.F.) ;
#59524=ORIENTED_EDGE('',*,*,#42553,.F.) ;
#59525=ORIENTED_EDGE('',*,*,#39098,.T.) ;
#59526=ORIENTED_EDGE('',*,*,#42554,.T.) ;
#59527=ORIENTED_EDGE('',*,*,#42555,.F.) ;
#59528=ORIENTED_EDGE('',*,*,#42548,.T.) ;
#59529=ORIENTED_EDGE('',*,*,#42556,.F.) ;
#59530=ORIENTED_EDGE('',*,*,#42557,.T.) ;
#59531=ORIENTED_EDGE('',*,*,#42558,.F.) ;
#59532=ORIENTED_EDGE('',*,*,#39338,.F.) ;
#59533=ORIENTED_EDGE('',*,*,#42559,.F.) ;
#59534=ORIENTED_EDGE('',*,*,#40656,.F.) ;
#59535=ORIENTED_EDGE('',*,*,#42551,.T.) ;
#59536=ORIENTED_EDGE('',*,*,#40653,.F.) ;
#59537=ORIENTED_EDGE('',*,*,#42560,.F.) ;
#59538=ORIENTED_EDGE('',*,*,#40659,.F.) ;
#59539=ORIENTED_EDGE('',*,*,#42550,.T.) ;
#59540=ORIENTED_EDGE('',*,*,#40658,.F.) ;
#59541=ORIENTED_EDGE('',*,*,#42561,.F.) ;
#59542=ORIENTED_EDGE('',*,*,#40400,.F.) ;
#59543=ORIENTED_EDGE('',*,*,#42552,.T.) ;
#59544=ORIENTED_EDGE('',*,*,#40407,.F.) ;
#59545=ORIENTED_EDGE('',*,*,#42562,.F.) ;
#59546=ORIENTED_EDGE('',*,*,#40650,.F.) ;
#59547=ORIENTED_EDGE('',*,*,#42563,.F.) ;
#59548=ORIENTED_EDGE('',*,*,#40651,.F.) ;
#59549=ORIENTED_EDGE('',*,*,#42564,.F.) ;
#59550=ORIENTED_EDGE('',*,*,#40646,.F.) ;
#59551=ORIENTED_EDGE('',*,*,#42553,.T.) ;
#59552=ORIENTED_EDGE('',*,*,#42563,.T.) ;
#59553=ORIENTED_EDGE('',*,*,#39099,.F.) ;
#59554=ORIENTED_EDGE('',*,*,#42559,.T.) ;
#59555=ORIENTED_EDGE('',*,*,#39348,.T.) ;
#59556=ORIENTED_EDGE('',*,*,#42565,.F.) ;
#59557=ORIENTED_EDGE('',*,*,#42560,.T.) ;
#59558=ORIENTED_EDGE('',*,*,#42566,.F.) ;
#59559=ORIENTED_EDGE('',*,*,#42561,.T.) ;
#59560=ORIENTED_EDGE('',*,*,#42567,.F.) ;
#59561=ORIENTED_EDGE('',*,*,#39442,.T.) ;
#59562=ORIENTED_EDGE('',*,*,#42562,.T.) ;
#59563=ORIENTED_EDGE('',*,*,#40406,.T.) ;
#59564=ORIENTED_EDGE('',*,*,#42568,.F.) ;
#59565=ORIENTED_EDGE('',*,*,#42564,.T.) ;
#59566=ORIENTED_EDGE('',*,*,#42565,.T.) ;
#59567=ORIENTED_EDGE('',*,*,#39347,.F.) ;
#59568=ORIENTED_EDGE('',*,*,#42569,.F.) ;
#59569=ORIENTED_EDGE('',*,*,#40660,.F.) ;
#59570=ORIENTED_EDGE('',*,*,#42567,.T.) ;
#59571=ORIENTED_EDGE('',*,*,#40657,.F.) ;
#59572=ORIENTED_EDGE('',*,*,#42570,.F.) ;
#59573=ORIENTED_EDGE('',*,*,#39443,.F.) ;
#59574=ORIENTED_EDGE('',*,*,#40401,.F.) ;
#59575=ORIENTED_EDGE('',*,*,#42566,.T.) ;
#59576=ORIENTED_EDGE('',*,*,#42571,.F.) ;
#59577=ORIENTED_EDGE('',*,*,#42572,.F.) ;
#59578=ORIENTED_EDGE('',*,*,#42568,.T.) ;
#59579=ORIENTED_EDGE('',*,*,#40405,.F.) ;
#59580=ORIENTED_EDGE('',*,*,#42573,.F.) ;
#59581=ORIENTED_EDGE('',*,*,#40647,.F.) ;
#59582=ORIENTED_EDGE('',*,*,#42574,.F.) ;
#59583=ORIENTED_EDGE('',*,*,#40648,.F.) ;
#59584=ORIENTED_EDGE('',*,*,#42575,.F.) ;
#59585=ORIENTED_EDGE('',*,*,#40642,.F.) ;
#59586=ORIENTED_EDGE('',*,*,#39101,.T.) ;
#59587=ORIENTED_EDGE('',*,*,#42574,.T.) ;
#59588=ORIENTED_EDGE('',*,*,#42576,.F.) ;
#59589=ORIENTED_EDGE('',*,*,#39342,.T.) ;
#59590=ORIENTED_EDGE('',*,*,#42570,.T.) ;
#59591=ORIENTED_EDGE('',*,*,#42569,.T.) ;
#59592=ORIENTED_EDGE('',*,*,#42577,.F.) ;
#59593=ORIENTED_EDGE('',*,*,#42578,.F.) ;
#59594=ORIENTED_EDGE('',*,*,#39560,.F.) ;
#59595=ORIENTED_EDGE('',*,*,#42579,.F.) ;
#59596=ORIENTED_EDGE('',*,*,#42580,.F.) ;
#59597=ORIENTED_EDGE('',*,*,#42571,.T.) ;
#59598=ORIENTED_EDGE('',*,*,#39446,.F.) ;
#59599=ORIENTED_EDGE('',*,*,#42579,.T.) ;
#59600=ORIENTED_EDGE('',*,*,#39649,.F.) ;
#59601=ORIENTED_EDGE('',*,*,#42572,.T.) ;
#59602=ORIENTED_EDGE('',*,*,#42581,.F.) ;
#59603=ORIENTED_EDGE('',*,*,#42582,.F.) ;
#59604=ORIENTED_EDGE('',*,*,#42575,.T.) ;
#59605=ORIENTED_EDGE('',*,*,#42573,.T.) ;
#59606=ORIENTED_EDGE('',*,*,#42583,.F.) ;
#59607=ORIENTED_EDGE('',*,*,#42576,.T.) ;
#59608=ORIENTED_EDGE('',*,*,#40645,.F.) ;
#59609=ORIENTED_EDGE('',*,*,#42584,.F.) ;
#59610=ORIENTED_EDGE('',*,*,#39343,.F.) ;
#59611=ORIENTED_EDGE('',*,*,#42577,.T.) ;
#59612=ORIENTED_EDGE('',*,*,#39346,.F.) ;
#59613=ORIENTED_EDGE('',*,*,#42585,.F.) ;
#59614=ORIENTED_EDGE('',*,*,#39444,.F.) ;
#59615=ORIENTED_EDGE('',*,*,#42578,.T.) ;
#59616=ORIENTED_EDGE('',*,*,#39445,.F.) ;
#59617=ORIENTED_EDGE('',*,*,#42586,.F.) ;
#59618=ORIENTED_EDGE('',*,*,#39642,.F.) ;
#59619=ORIENTED_EDGE('',*,*,#42580,.T.) ;
#59620=ORIENTED_EDGE('',*,*,#39648,.T.) ;
#59621=ORIENTED_EDGE('',*,*,#42587,.F.) ;
#59622=ORIENTED_EDGE('',*,*,#42581,.T.) ;
#59623=ORIENTED_EDGE('',*,*,#40402,.F.) ;
#59624=ORIENTED_EDGE('',*,*,#42582,.T.) ;
#59625=ORIENTED_EDGE('',*,*,#42588,.F.) ;
#59626=ORIENTED_EDGE('',*,*,#42589,.F.) ;
#59627=ORIENTED_EDGE('',*,*,#42583,.T.) ;
#59628=ORIENTED_EDGE('',*,*,#40404,.F.) ;
#59629=ORIENTED_EDGE('',*,*,#42590,.F.) ;
#59630=ORIENTED_EDGE('',*,*,#40643,.F.) ;
#59631=ORIENTED_EDGE('',*,*,#42591,.F.) ;
#59632=ORIENTED_EDGE('',*,*,#40644,.F.) ;
#59633=ORIENTED_EDGE('',*,*,#42592,.F.) ;
#59634=ORIENTED_EDGE('',*,*,#39441,.F.) ;
#59635=ORIENTED_EDGE('',*,*,#42584,.T.) ;
#59636=ORIENTED_EDGE('',*,*,#42591,.T.) ;
#59637=ORIENTED_EDGE('',*,*,#42593,.F.) ;
#59638=ORIENTED_EDGE('',*,*,#42586,.T.) ;
#59639=ORIENTED_EDGE('',*,*,#42585,.T.) ;
#59640=ORIENTED_EDGE('',*,*,#42594,.F.) ;
#59641=ORIENTED_EDGE('',*,*,#39643,.T.) ;
#59642=ORIENTED_EDGE('',*,*,#42595,.F.) ;
#59643=ORIENTED_EDGE('',*,*,#42588,.T.) ;
#59644=ORIENTED_EDGE('',*,*,#42587,.T.) ;
#59645=ORIENTED_EDGE('',*,*,#39700,.F.) ;
#59646=ORIENTED_EDGE('',*,*,#42589,.T.) ;
#59647=ORIENTED_EDGE('',*,*,#42596,.F.) ;
#59648=ORIENTED_EDGE('',*,*,#42597,.F.) ;
#59649=ORIENTED_EDGE('',*,*,#42592,.T.) ;
#59650=ORIENTED_EDGE('',*,*,#42590,.T.) ;
#59651=ORIENTED_EDGE('',*,*,#42598,.F.) ;
#59652=ORIENTED_EDGE('',*,*,#39437,.T.) ;
#59653=ORIENTED_EDGE('',*,*,#42593,.T.) ;
#59654=ORIENTED_EDGE('',*,*,#39440,.F.) ;
#59655=ORIENTED_EDGE('',*,*,#42599,.F.) ;
#59656=ORIENTED_EDGE('',*,*,#39344,.F.) ;
#59657=ORIENTED_EDGE('',*,*,#42594,.T.) ;
#59658=ORIENTED_EDGE('',*,*,#39345,.F.) ;
#59659=ORIENTED_EDGE('',*,*,#42600,.F.) ;
#59660=ORIENTED_EDGE('',*,*,#39644,.F.) ;
#59661=ORIENTED_EDGE('',*,*,#42595,.T.) ;
#59662=ORIENTED_EDGE('',*,*,#39699,.T.) ;
#59663=ORIENTED_EDGE('',*,*,#42601,.F.) ;
#59664=ORIENTED_EDGE('',*,*,#42596,.T.) ;
#59665=ORIENTED_EDGE('',*,*,#40403,.F.) ;
#59666=ORIENTED_EDGE('',*,*,#42597,.T.) ;
#59667=ORIENTED_EDGE('',*,*,#42602,.F.) ;
#59668=ORIENTED_EDGE('',*,*,#42598,.T.) ;
#59669=ORIENTED_EDGE('',*,*,#42600,.T.) ;
#59670=ORIENTED_EDGE('',*,*,#42599,.T.) ;
#59671=ORIENTED_EDGE('',*,*,#42603,.F.) ;
#59672=ORIENTED_EDGE('',*,*,#39592,.T.) ;
#59673=ORIENTED_EDGE('',*,*,#42601,.T.) ;
#59674=ORIENTED_EDGE('',*,*,#39698,.F.) ;
#59675=ORIENTED_EDGE('',*,*,#42604,.F.) ;
#59676=ORIENTED_EDGE('',*,*,#39438,.F.) ;
#59677=ORIENTED_EDGE('',*,*,#42602,.T.) ;
#59678=ORIENTED_EDGE('',*,*,#42603,.T.) ;
#59679=ORIENTED_EDGE('',*,*,#39439,.F.) ;
#59680=ORIENTED_EDGE('',*,*,#42605,.F.) ;
#59681=ORIENTED_EDGE('',*,*,#39593,.F.) ;
#59682=ORIENTED_EDGE('',*,*,#42604,.T.) ;
#59683=ORIENTED_EDGE('',*,*,#39645,.F.) ;
#59684=ORIENTED_EDGE('',*,*,#42605,.T.) ;
#59685=ORIENTED_EDGE('',*,*,#42606,.F.) ;
#59686=ORIENTED_EDGE('',*,*,#40702,.F.) ;
#59687=ORIENTED_EDGE('',*,*,#42607,.F.) ;
#59688=ORIENTED_EDGE('',*,*,#40749,.F.) ;
#59689=ORIENTED_EDGE('',*,*,#42607,.T.) ;
#59690=ORIENTED_EDGE('',*,*,#40699,.F.) ;
#59691=ORIENTED_EDGE('',*,*,#42608,.F.) ;
#59692=ORIENTED_EDGE('',*,*,#40750,.F.) ;
#59693=ORIENTED_EDGE('',*,*,#40705,.F.) ;
#59694=ORIENTED_EDGE('',*,*,#42606,.T.) ;
#59695=ORIENTED_EDGE('',*,*,#42609,.F.) ;
#59696=ORIENTED_EDGE('',*,*,#42608,.T.) ;
#59697=ORIENTED_EDGE('',*,*,#40696,.F.) ;
#59698=ORIENTED_EDGE('',*,*,#42610,.F.) ;
#59699=ORIENTED_EDGE('',*,*,#40751,.F.) ;
#59700=ORIENTED_EDGE('',*,*,#42609,.T.) ;
#59701=ORIENTED_EDGE('',*,*,#40748,.F.) ;
#59702=ORIENTED_EDGE('',*,*,#42611,.F.) ;
#59703=ORIENTED_EDGE('',*,*,#40708,.F.) ;
#59704=ORIENTED_EDGE('',*,*,#42610,.T.) ;
#59705=ORIENTED_EDGE('',*,*,#40693,.F.) ;
#59706=ORIENTED_EDGE('',*,*,#42612,.F.) ;
#59707=ORIENTED_EDGE('',*,*,#40752,.F.) ;
#59708=ORIENTED_EDGE('',*,*,#40711,.F.) ;
#59709=ORIENTED_EDGE('',*,*,#42611,.T.) ;
#59710=ORIENTED_EDGE('',*,*,#42613,.F.) ;
#59711=ORIENTED_EDGE('',*,*,#42612,.T.) ;
#59712=ORIENTED_EDGE('',*,*,#40690,.F.) ;
#59713=ORIENTED_EDGE('',*,*,#42614,.F.) ;
#59714=ORIENTED_EDGE('',*,*,#40753,.F.) ;
#59715=ORIENTED_EDGE('',*,*,#42613,.T.) ;
#59716=ORIENTED_EDGE('',*,*,#40747,.F.) ;
#59717=ORIENTED_EDGE('',*,*,#42615,.F.) ;
#59718=ORIENTED_EDGE('',*,*,#40714,.F.) ;
#59719=ORIENTED_EDGE('',*,*,#42614,.T.) ;
#59720=ORIENTED_EDGE('',*,*,#40687,.F.) ;
#59721=ORIENTED_EDGE('',*,*,#42616,.F.) ;
#59722=ORIENTED_EDGE('',*,*,#40717,.F.) ;
#59723=ORIENTED_EDGE('',*,*,#42615,.T.) ;
#59724=ORIENTED_EDGE('',*,*,#42617,.F.) ;
#59725=ORIENTED_EDGE('',*,*,#42616,.T.) ;
#59726=ORIENTED_EDGE('',*,*,#40684,.F.) ;
#59727=ORIENTED_EDGE('',*,*,#42618,.F.) ;
#59728=ORIENTED_EDGE('',*,*,#40754,.F.) ;
#59729=ORIENTED_EDGE('',*,*,#42617,.T.) ;
#59730=ORIENTED_EDGE('',*,*,#40746,.F.) ;
#59731=ORIENTED_EDGE('',*,*,#42619,.F.) ;
#59732=ORIENTED_EDGE('',*,*,#40720,.F.) ;
#59733=ORIENTED_EDGE('',*,*,#42618,.T.) ;
#59734=ORIENTED_EDGE('',*,*,#39310,.F.) ;
#59735=ORIENTED_EDGE('',*,*,#42620,.F.) ;
#59736=ORIENTED_EDGE('',*,*,#40723,.F.) ;
#59737=ORIENTED_EDGE('',*,*,#42619,.T.) ;
#59738=ORIENTED_EDGE('',*,*,#42621,.F.) ;
#59739=ORIENTED_EDGE('',*,*,#42620,.T.) ;
#59740=ORIENTED_EDGE('',*,*,#40682,.F.) ;
#59741=ORIENTED_EDGE('',*,*,#39097,.F.) ;
#59742=ORIENTED_EDGE('',*,*,#40755,.F.) ;
#59743=ORIENTED_EDGE('',*,*,#42621,.T.) ;
#59744=ORIENTED_EDGE('',*,*,#40745,.F.) ;
#59745=ORIENTED_EDGE('',*,*,#42622,.F.) ;
#59746=ORIENTED_EDGE('',*,*,#40726,.F.) ;
#59747=ORIENTED_EDGE('',*,*,#40729,.F.) ;
#59748=ORIENTED_EDGE('',*,*,#42622,.T.) ;
#59749=ORIENTED_EDGE('',*,*,#42623,.F.) ;
#59750=ORIENTED_EDGE('',*,*,#39096,.T.) ;
#59751=ORIENTED_EDGE('',*,*,#40677,.F.) ;
#59752=ORIENTED_EDGE('',*,*,#42624,.F.) ;
#59753=ORIENTED_EDGE('',*,*,#40756,.F.) ;
#59754=ORIENTED_EDGE('',*,*,#42623,.T.) ;
#59755=ORIENTED_EDGE('',*,*,#40744,.F.) ;
#59756=ORIENTED_EDGE('',*,*,#42625,.F.) ;
#59757=ORIENTED_EDGE('',*,*,#40732,.F.) ;
#59758=ORIENTED_EDGE('',*,*,#42624,.T.) ;
#59759=ORIENTED_EDGE('',*,*,#40674,.F.) ;
#59760=ORIENTED_EDGE('',*,*,#42626,.F.) ;
#59761=ORIENTED_EDGE('',*,*,#40735,.F.) ;
#59762=ORIENTED_EDGE('',*,*,#42625,.T.) ;
#59763=ORIENTED_EDGE('',*,*,#42627,.F.) ;
#59764=ORIENTED_EDGE('',*,*,#42626,.T.) ;
#59765=ORIENTED_EDGE('',*,*,#40671,.F.) ;
#59766=ORIENTED_EDGE('',*,*,#42628,.F.) ;
#59767=ORIENTED_EDGE('',*,*,#40757,.F.) ;
#59768=ORIENTED_EDGE('',*,*,#42627,.T.) ;
#59769=ORIENTED_EDGE('',*,*,#40743,.F.) ;
#59770=ORIENTED_EDGE('',*,*,#42629,.F.) ;
#59771=ORIENTED_EDGE('',*,*,#40738,.F.) ;
#59772=ORIENTED_EDGE('',*,*,#42628,.T.) ;
#59773=ORIENTED_EDGE('',*,*,#40668,.F.) ;
#59774=ORIENTED_EDGE('',*,*,#42630,.F.) ;
#59775=ORIENTED_EDGE('',*,*,#40740,.F.) ;
#59776=ORIENTED_EDGE('',*,*,#42629,.T.) ;
#59777=ORIENTED_EDGE('',*,*,#40742,.F.) ;
#59778=ORIENTED_EDGE('',*,*,#42631,.F.) ;
#59779=ORIENTED_EDGE('',*,*,#40662,.F.) ;
#59780=ORIENTED_EDGE('',*,*,#42630,.T.) ;
#59781=ORIENTED_EDGE('',*,*,#40665,.F.) ;
#59782=ORIENTED_EDGE('',*,*,#42631,.T.) ;
#59783=ORIENTED_EDGE('',*,*,#40741,.F.) ;
#59784=ORIENTED_EDGE('',*,*,#42632,.T.) ;
#59785=ORIENTED_EDGE('',*,*,#42633,.T.) ;
#59786=ORIENTED_EDGE('',*,*,#42634,.T.) ;
#59787=ORIENTED_EDGE('',*,*,#42635,.T.) ;
#59788=ORIENTED_EDGE('',*,*,#42636,.T.) ;
#59789=ORIENTED_EDGE('',*,*,#42637,.T.) ;
#59790=ORIENTED_EDGE('',*,*,#42638,.T.) ;
#59791=ORIENTED_EDGE('',*,*,#42639,.T.) ;
#59792=ORIENTED_EDGE('',*,*,#42640,.T.) ;
#59793=ORIENTED_EDGE('',*,*,#42641,.T.) ;
#59794=ORIENTED_EDGE('',*,*,#42642,.T.) ;
#59795=ORIENTED_EDGE('',*,*,#42643,.T.) ;
#59796=ORIENTED_EDGE('',*,*,#42644,.T.) ;
#59797=ORIENTED_EDGE('',*,*,#42645,.T.) ;
#59798=ORIENTED_EDGE('',*,*,#42646,.T.) ;
#59799=ORIENTED_EDGE('',*,*,#42647,.T.) ;
#59800=ORIENTED_EDGE('',*,*,#42648,.T.) ;
#59801=ORIENTED_EDGE('',*,*,#42649,.T.) ;
#59802=ORIENTED_EDGE('',*,*,#42650,.F.) ;
#59803=ORIENTED_EDGE('',*,*,#42651,.T.) ;
#59804=ORIENTED_EDGE('',*,*,#42652,.T.) ;
#59805=ORIENTED_EDGE('',*,*,#42653,.T.) ;
#59806=ORIENTED_EDGE('',*,*,#41620,.T.) ;
#59807=ORIENTED_EDGE('',*,*,#42654,.T.) ;
#59808=ORIENTED_EDGE('',*,*,#42655,.T.) ;
#59809=ORIENTED_EDGE('',*,*,#42656,.T.) ;
#59810=ORIENTED_EDGE('',*,*,#42657,.T.) ;
#59811=ORIENTED_EDGE('',*,*,#42658,.T.) ;
#59812=ORIENTED_EDGE('',*,*,#39275,.T.) ;
#59813=ORIENTED_EDGE('',*,*,#42659,.T.) ;
#59814=ORIENTED_EDGE('',*,*,#42660,.T.) ;
#59815=ORIENTED_EDGE('',*,*,#42661,.T.) ;
#59816=ORIENTED_EDGE('',*,*,#41617,.T.) ;
#59817=ORIENTED_EDGE('',*,*,#42662,.T.) ;
#59818=ORIENTED_EDGE('',*,*,#42632,.F.) ;
#59819=ORIENTED_EDGE('',*,*,#42663,.T.) ;
#59820=ORIENTED_EDGE('',*,*,#41618,.T.) ;
#59821=ORIENTED_EDGE('',*,*,#42650,.T.) ;
#59822=ORIENTED_EDGE('',*,*,#42664,.T.) ;
#59823=ORIENTED_EDGE('',*,*,#39428,.F.) ;
#59824=ORIENTED_EDGE('',*,*,#42665,.T.) ;
#59825=ORIENTED_EDGE('',*,*,#42666,.T.) ;
#59826=ORIENTED_EDGE('',*,*,#42667,.T.) ;
#59827=ORIENTED_EDGE('',*,*,#42668,.T.) ;
#59828=ORIENTED_EDGE('',*,*,#42669,.T.) ;
#59829=ORIENTED_EDGE('',*,*,#42670,.T.) ;
#59830=ORIENTED_EDGE('',*,*,#42671,.T.) ;
#59831=ORIENTED_EDGE('',*,*,#41536,.F.) ;
#59832=ORIENTED_EDGE('',*,*,#42672,.T.) ;
#59833=ORIENTED_EDGE('',*,*,#41540,.F.) ;
#59834=ORIENTED_EDGE('',*,*,#42673,.T.) ;
#59835=ORIENTED_EDGE('',*,*,#42674,.T.) ;
#59836=ORIENTED_EDGE('',*,*,#42675,.T.) ;
#59837=ORIENTED_EDGE('',*,*,#42676,.T.) ;
#59838=ORIENTED_EDGE('',*,*,#42677,.T.) ;
#59839=ORIENTED_EDGE('',*,*,#42678,.T.) ;
#59840=ORIENTED_EDGE('',*,*,#42679,.T.) ;
#59841=ORIENTED_EDGE('',*,*,#42680,.T.) ;
#59842=ORIENTED_EDGE('',*,*,#42681,.T.) ;
#59843=ORIENTED_EDGE('',*,*,#42682,.T.) ;
#59844=ORIENTED_EDGE('',*,*,#42683,.T.) ;
#59845=ORIENTED_EDGE('',*,*,#42684,.T.) ;
#59846=ORIENTED_EDGE('',*,*,#42685,.T.) ;
#59847=ORIENTED_EDGE('',*,*,#41534,.T.) ;
#59848=ORIENTED_EDGE('',*,*,#42686,.T.) ;
#59849=ORIENTED_EDGE('',*,*,#41538,.F.) ;
#59850=ORIENTED_EDGE('',*,*,#42687,.T.) ;
#59851=ORIENTED_EDGE('',*,*,#42688,.T.) ;
#59852=ORIENTED_EDGE('',*,*,#42689,.T.) ;
#59853=ORIENTED_EDGE('',*,*,#42690,.T.) ;
#59854=ORIENTED_EDGE('',*,*,#42691,.T.) ;
#59855=ORIENTED_EDGE('',*,*,#42692,.T.) ;
#59856=ORIENTED_EDGE('',*,*,#42693,.T.) ;
#59857=ORIENTED_EDGE('',*,*,#42694,.T.) ;
#59858=ORIENTED_EDGE('',*,*,#42695,.T.) ;
#59859=ORIENTED_EDGE('',*,*,#42696,.T.) ;
#59860=ORIENTED_EDGE('',*,*,#42697,.T.) ;
#59861=ORIENTED_EDGE('',*,*,#42698,.T.) ;
#59862=ORIENTED_EDGE('',*,*,#42699,.T.) ;
#59863=ORIENTED_EDGE('',*,*,#42700,.T.) ;
#59864=ORIENTED_EDGE('',*,*,#42701,.T.) ;
#59865=ORIENTED_EDGE('',*,*,#42702,.T.) ;
#59866=ORIENTED_EDGE('',*,*,#42703,.T.) ;
#59867=ORIENTED_EDGE('',*,*,#42704,.T.) ;
#59868=ORIENTED_EDGE('',*,*,#42705,.T.) ;
#59869=ORIENTED_EDGE('',*,*,#42706,.T.) ;
#59870=ORIENTED_EDGE('',*,*,#42707,.T.) ;
#59871=ORIENTED_EDGE('',*,*,#42708,.F.) ;
#59872=ORIENTED_EDGE('',*,*,#42709,.T.) ;
#59873=ORIENTED_EDGE('',*,*,#42710,.T.) ;
#59874=ORIENTED_EDGE('',*,*,#42711,.T.) ;
#59875=ORIENTED_EDGE('',*,*,#41942,.T.) ;
#59876=ORIENTED_EDGE('',*,*,#42712,.T.) ;
#59877=ORIENTED_EDGE('',*,*,#42713,.T.) ;
#59878=ORIENTED_EDGE('',*,*,#42714,.T.) ;
#59879=ORIENTED_EDGE('',*,*,#42715,.T.) ;
#59880=ORIENTED_EDGE('',*,*,#42716,.T.) ;
#59881=ORIENTED_EDGE('',*,*,#39222,.T.) ;
#59882=ORIENTED_EDGE('',*,*,#42717,.T.) ;
#59883=ORIENTED_EDGE('',*,*,#42718,.T.) ;
#59884=ORIENTED_EDGE('',*,*,#42719,.T.) ;
#59885=ORIENTED_EDGE('',*,*,#41939,.T.) ;
#59886=ORIENTED_EDGE('',*,*,#42720,.T.) ;
#59887=ORIENTED_EDGE('',*,*,#42690,.F.) ;
#59888=ORIENTED_EDGE('',*,*,#42721,.T.) ;
#59889=ORIENTED_EDGE('',*,*,#41940,.T.) ;
#59890=ORIENTED_EDGE('',*,*,#42708,.T.) ;
#59891=ORIENTED_EDGE('',*,*,#42722,.T.) ;
#59892=ORIENTED_EDGE('',*,*,#39417,.F.) ;
#59893=ORIENTED_EDGE('',*,*,#42723,.T.) ;
#59894=ORIENTED_EDGE('',*,*,#42724,.T.) ;
#59895=ORIENTED_EDGE('',*,*,#42725,.T.) ;
#59896=ORIENTED_EDGE('',*,*,#42726,.T.) ;
#59897=ORIENTED_EDGE('',*,*,#42727,.T.) ;
#59898=ORIENTED_EDGE('',*,*,#42728,.T.) ;
#59899=ORIENTED_EDGE('',*,*,#42729,.T.) ;
#59900=ORIENTED_EDGE('',*,*,#41544,.F.) ;
#59901=ORIENTED_EDGE('',*,*,#42730,.T.) ;
#59902=ORIENTED_EDGE('',*,*,#41548,.F.) ;
#59903=ORIENTED_EDGE('',*,*,#42731,.T.) ;
#59904=ORIENTED_EDGE('',*,*,#42732,.T.) ;
#59905=ORIENTED_EDGE('',*,*,#42733,.T.) ;
#59906=ORIENTED_EDGE('',*,*,#42734,.T.) ;
#59907=ORIENTED_EDGE('',*,*,#42735,.T.) ;
#59908=ORIENTED_EDGE('',*,*,#42736,.T.) ;
#59909=ORIENTED_EDGE('',*,*,#42737,.T.) ;
#59910=ORIENTED_EDGE('',*,*,#42738,.T.) ;
#59911=ORIENTED_EDGE('',*,*,#42739,.T.) ;
#59912=ORIENTED_EDGE('',*,*,#42740,.T.) ;
#59913=ORIENTED_EDGE('',*,*,#42741,.T.) ;
#59914=ORIENTED_EDGE('',*,*,#42742,.T.) ;
#59915=ORIENTED_EDGE('',*,*,#42743,.T.) ;
#59916=ORIENTED_EDGE('',*,*,#41542,.T.) ;
#59917=ORIENTED_EDGE('',*,*,#42744,.T.) ;
#59918=ORIENTED_EDGE('',*,*,#41546,.F.) ;
#59919=ORIENTED_EDGE('',*,*,#42745,.T.) ;
#59920=ORIENTED_EDGE('',*,*,#42746,.T.) ;
#59921=ORIENTED_EDGE('',*,*,#42747,.T.) ;
#59922=ORIENTED_EDGE('',*,*,#42748,.T.) ;
#59923=ORIENTED_EDGE('',*,*,#42749,.T.) ;
#59924=ORIENTED_EDGE('',*,*,#42750,.T.) ;
#59925=ORIENTED_EDGE('',*,*,#42751,.T.) ;
#59926=ORIENTED_EDGE('',*,*,#42752,.T.) ;
#59927=ORIENTED_EDGE('',*,*,#42753,.T.) ;
#59928=ORIENTED_EDGE('',*,*,#42754,.T.) ;
#59929=ORIENTED_EDGE('',*,*,#42755,.T.) ;
#59930=ORIENTED_EDGE('',*,*,#42756,.T.) ;
#59931=ORIENTED_EDGE('',*,*,#42757,.T.) ;
#59932=ORIENTED_EDGE('',*,*,#42758,.T.) ;
#59933=ORIENTED_EDGE('',*,*,#42759,.T.) ;
#59934=ORIENTED_EDGE('',*,*,#42760,.T.) ;
#59935=ORIENTED_EDGE('',*,*,#42761,.T.) ;
#59936=ORIENTED_EDGE('',*,*,#42762,.T.) ;
#59937=ORIENTED_EDGE('',*,*,#42763,.T.) ;
#59938=ORIENTED_EDGE('',*,*,#42764,.T.) ;
#59939=ORIENTED_EDGE('',*,*,#42765,.T.) ;
#59940=ORIENTED_EDGE('',*,*,#42766,.F.) ;
#59941=ORIENTED_EDGE('',*,*,#42767,.T.) ;
#59942=ORIENTED_EDGE('',*,*,#42768,.T.) ;
#59943=ORIENTED_EDGE('',*,*,#42769,.T.) ;
#59944=ORIENTED_EDGE('',*,*,#42030,.T.) ;
#59945=ORIENTED_EDGE('',*,*,#42770,.T.) ;
#59946=ORIENTED_EDGE('',*,*,#42771,.T.) ;
#59947=ORIENTED_EDGE('',*,*,#42772,.T.) ;
#59948=ORIENTED_EDGE('',*,*,#42773,.T.) ;
#59949=ORIENTED_EDGE('',*,*,#42774,.T.) ;
#59950=ORIENTED_EDGE('',*,*,#39205,.T.) ;
#59951=ORIENTED_EDGE('',*,*,#42775,.T.) ;
#59952=ORIENTED_EDGE('',*,*,#42776,.T.) ;
#59953=ORIENTED_EDGE('',*,*,#42777,.T.) ;
#59954=ORIENTED_EDGE('',*,*,#42027,.T.) ;
#59955=ORIENTED_EDGE('',*,*,#42778,.T.) ;
#59956=ORIENTED_EDGE('',*,*,#42748,.F.) ;
#59957=ORIENTED_EDGE('',*,*,#42779,.T.) ;
#59958=ORIENTED_EDGE('',*,*,#42028,.T.) ;
#59959=ORIENTED_EDGE('',*,*,#42766,.T.) ;
#59960=ORIENTED_EDGE('',*,*,#42780,.T.) ;
#59961=ORIENTED_EDGE('',*,*,#39406,.F.) ;
#59962=ORIENTED_EDGE('',*,*,#42781,.T.) ;
#59963=ORIENTED_EDGE('',*,*,#42782,.T.) ;
#59964=ORIENTED_EDGE('',*,*,#42783,.T.) ;
#59965=ORIENTED_EDGE('',*,*,#42784,.T.) ;
#59966=ORIENTED_EDGE('',*,*,#42785,.T.) ;
#59967=ORIENTED_EDGE('',*,*,#42786,.T.) ;
#59968=ORIENTED_EDGE('',*,*,#42787,.T.) ;
#59969=ORIENTED_EDGE('',*,*,#41552,.F.) ;
#59970=ORIENTED_EDGE('',*,*,#42788,.T.) ;
#59971=ORIENTED_EDGE('',*,*,#41556,.F.) ;
#59972=ORIENTED_EDGE('',*,*,#42789,.T.) ;
#59973=ORIENTED_EDGE('',*,*,#42790,.T.) ;
#59974=ORIENTED_EDGE('',*,*,#42791,.T.) ;
#59975=ORIENTED_EDGE('',*,*,#42792,.T.) ;
#59976=ORIENTED_EDGE('',*,*,#42793,.T.) ;
#59977=ORIENTED_EDGE('',*,*,#42794,.T.) ;
#59978=ORIENTED_EDGE('',*,*,#42795,.T.) ;
#59979=ORIENTED_EDGE('',*,*,#42796,.T.) ;
#59980=ORIENTED_EDGE('',*,*,#42797,.T.) ;
#59981=ORIENTED_EDGE('',*,*,#42798,.T.) ;
#59982=ORIENTED_EDGE('',*,*,#42799,.T.) ;
#59983=ORIENTED_EDGE('',*,*,#42800,.T.) ;
#59984=ORIENTED_EDGE('',*,*,#42801,.T.) ;
#59985=ORIENTED_EDGE('',*,*,#41550,.T.) ;
#59986=ORIENTED_EDGE('',*,*,#42802,.T.) ;
#59987=ORIENTED_EDGE('',*,*,#41554,.F.) ;
#59988=ORIENTED_EDGE('',*,*,#42803,.T.) ;
#59989=ORIENTED_EDGE('',*,*,#42804,.T.) ;
#59990=ORIENTED_EDGE('',*,*,#42805,.T.) ;
#59991=ORIENTED_EDGE('',*,*,#42806,.T.) ;
#59992=ORIENTED_EDGE('',*,*,#42807,.T.) ;
#59993=ORIENTED_EDGE('',*,*,#42808,.T.) ;
#59994=ORIENTED_EDGE('',*,*,#42809,.T.) ;
#59995=ORIENTED_EDGE('',*,*,#42810,.T.) ;
#59996=ORIENTED_EDGE('',*,*,#42811,.T.) ;
#59997=ORIENTED_EDGE('',*,*,#42812,.T.) ;
#59998=ORIENTED_EDGE('',*,*,#42813,.T.) ;
#59999=ORIENTED_EDGE('',*,*,#42814,.T.) ;
#60000=ORIENTED_EDGE('',*,*,#42815,.T.) ;
#60001=ORIENTED_EDGE('',*,*,#42816,.T.) ;
#60002=ORIENTED_EDGE('',*,*,#42817,.T.) ;
#60003=ORIENTED_EDGE('',*,*,#42818,.T.) ;
#60004=ORIENTED_EDGE('',*,*,#42819,.T.) ;
#60005=ORIENTED_EDGE('',*,*,#42820,.T.) ;
#60006=ORIENTED_EDGE('',*,*,#42821,.T.) ;
#60007=ORIENTED_EDGE('',*,*,#42822,.T.) ;
#60008=ORIENTED_EDGE('',*,*,#42823,.T.) ;
#60009=ORIENTED_EDGE('',*,*,#42824,.F.) ;
#60010=ORIENTED_EDGE('',*,*,#42825,.T.) ;
#60011=ORIENTED_EDGE('',*,*,#42826,.T.) ;
#60012=ORIENTED_EDGE('',*,*,#42827,.T.) ;
#60013=ORIENTED_EDGE('',*,*,#42118,.T.) ;
#60014=ORIENTED_EDGE('',*,*,#42828,.T.) ;
#60015=ORIENTED_EDGE('',*,*,#42829,.T.) ;
#60016=ORIENTED_EDGE('',*,*,#42830,.T.) ;
#60017=ORIENTED_EDGE('',*,*,#42831,.T.) ;
#60018=ORIENTED_EDGE('',*,*,#42832,.T.) ;
#60019=ORIENTED_EDGE('',*,*,#39188,.T.) ;
#60020=ORIENTED_EDGE('',*,*,#42833,.T.) ;
#60021=ORIENTED_EDGE('',*,*,#42834,.T.) ;
#60022=ORIENTED_EDGE('',*,*,#42835,.T.) ;
#60023=ORIENTED_EDGE('',*,*,#42115,.T.) ;
#60024=ORIENTED_EDGE('',*,*,#42836,.T.) ;
#60025=ORIENTED_EDGE('',*,*,#42806,.F.) ;
#60026=ORIENTED_EDGE('',*,*,#42837,.T.) ;
#60027=ORIENTED_EDGE('',*,*,#42116,.T.) ;
#60028=ORIENTED_EDGE('',*,*,#42824,.T.) ;
#60029=ORIENTED_EDGE('',*,*,#42838,.T.) ;
#60030=ORIENTED_EDGE('',*,*,#39395,.F.) ;
#60031=ORIENTED_EDGE('',*,*,#42839,.T.) ;
#60032=ORIENTED_EDGE('',*,*,#42840,.T.) ;
#60033=ORIENTED_EDGE('',*,*,#42841,.T.) ;
#60034=ORIENTED_EDGE('',*,*,#42842,.T.) ;
#60035=ORIENTED_EDGE('',*,*,#42843,.T.) ;
#60036=ORIENTED_EDGE('',*,*,#42844,.T.) ;
#60037=ORIENTED_EDGE('',*,*,#42845,.T.) ;
#60038=ORIENTED_EDGE('',*,*,#41560,.F.) ;
#60039=ORIENTED_EDGE('',*,*,#42846,.T.) ;
#60040=ORIENTED_EDGE('',*,*,#41564,.F.) ;
#60041=ORIENTED_EDGE('',*,*,#42847,.T.) ;
#60042=ORIENTED_EDGE('',*,*,#42848,.T.) ;
#60043=ORIENTED_EDGE('',*,*,#42849,.T.) ;
#60044=ORIENTED_EDGE('',*,*,#42850,.T.) ;
#60045=ORIENTED_EDGE('',*,*,#42851,.T.) ;
#60046=ORIENTED_EDGE('',*,*,#42852,.T.) ;
#60047=ORIENTED_EDGE('',*,*,#42853,.T.) ;
#60048=ORIENTED_EDGE('',*,*,#42854,.T.) ;
#60049=ORIENTED_EDGE('',*,*,#42855,.T.) ;
#60050=ORIENTED_EDGE('',*,*,#42856,.T.) ;
#60051=ORIENTED_EDGE('',*,*,#42857,.T.) ;
#60052=ORIENTED_EDGE('',*,*,#42858,.T.) ;
#60053=ORIENTED_EDGE('',*,*,#42859,.T.) ;
#60054=ORIENTED_EDGE('',*,*,#41558,.T.) ;
#60055=ORIENTED_EDGE('',*,*,#42860,.T.) ;
#60056=ORIENTED_EDGE('',*,*,#41562,.F.) ;
#60057=ORIENTED_EDGE('',*,*,#42861,.T.) ;
#60058=ORIENTED_EDGE('',*,*,#42862,.T.) ;
#60059=ORIENTED_EDGE('',*,*,#42863,.T.) ;
#60060=ORIENTED_EDGE('',*,*,#42864,.T.) ;
#60061=ORIENTED_EDGE('',*,*,#42865,.T.) ;
#60062=ORIENTED_EDGE('',*,*,#42866,.T.) ;
#60063=ORIENTED_EDGE('',*,*,#42867,.T.) ;
#60064=ORIENTED_EDGE('',*,*,#42868,.T.) ;
#60065=ORIENTED_EDGE('',*,*,#42869,.T.) ;
#60066=ORIENTED_EDGE('',*,*,#42870,.T.) ;
#60067=ORIENTED_EDGE('',*,*,#42871,.T.) ;
#60068=ORIENTED_EDGE('',*,*,#42872,.T.) ;
#60069=ORIENTED_EDGE('',*,*,#42873,.T.) ;
#60070=ORIENTED_EDGE('',*,*,#42874,.T.) ;
#60071=ORIENTED_EDGE('',*,*,#42875,.T.) ;
#60072=ORIENTED_EDGE('',*,*,#42876,.T.) ;
#60073=ORIENTED_EDGE('',*,*,#42877,.T.) ;
#60074=ORIENTED_EDGE('',*,*,#42878,.T.) ;
#60075=ORIENTED_EDGE('',*,*,#42879,.T.) ;
#60076=ORIENTED_EDGE('',*,*,#42880,.T.) ;
#60077=ORIENTED_EDGE('',*,*,#42881,.T.) ;
#60078=ORIENTED_EDGE('',*,*,#42882,.F.) ;
#60079=ORIENTED_EDGE('',*,*,#42883,.T.) ;
#60080=ORIENTED_EDGE('',*,*,#42884,.T.) ;
#60081=ORIENTED_EDGE('',*,*,#42885,.T.) ;
#60082=ORIENTED_EDGE('',*,*,#42206,.T.) ;
#60083=ORIENTED_EDGE('',*,*,#42886,.T.) ;
#60084=ORIENTED_EDGE('',*,*,#42887,.T.) ;
#60085=ORIENTED_EDGE('',*,*,#42888,.T.) ;
#60086=ORIENTED_EDGE('',*,*,#42889,.T.) ;
#60087=ORIENTED_EDGE('',*,*,#42890,.T.) ;
#60088=ORIENTED_EDGE('',*,*,#39171,.T.) ;
#60089=ORIENTED_EDGE('',*,*,#42891,.T.) ;
#60090=ORIENTED_EDGE('',*,*,#42892,.T.) ;
#60091=ORIENTED_EDGE('',*,*,#42893,.T.) ;
#60092=ORIENTED_EDGE('',*,*,#42203,.T.) ;
#60093=ORIENTED_EDGE('',*,*,#42894,.T.) ;
#60094=ORIENTED_EDGE('',*,*,#42864,.F.) ;
#60095=ORIENTED_EDGE('',*,*,#42895,.T.) ;
#60096=ORIENTED_EDGE('',*,*,#42204,.T.) ;
#60097=ORIENTED_EDGE('',*,*,#42882,.T.) ;
#60098=ORIENTED_EDGE('',*,*,#42896,.T.) ;
#60099=ORIENTED_EDGE('',*,*,#39384,.F.) ;
#60100=ORIENTED_EDGE('',*,*,#42897,.T.) ;
#60101=ORIENTED_EDGE('',*,*,#42898,.T.) ;
#60102=ORIENTED_EDGE('',*,*,#42899,.T.) ;
#60103=ORIENTED_EDGE('',*,*,#42900,.T.) ;
#60104=ORIENTED_EDGE('',*,*,#42901,.T.) ;
#60105=ORIENTED_EDGE('',*,*,#42902,.T.) ;
#60106=ORIENTED_EDGE('',*,*,#42903,.T.) ;
#60107=ORIENTED_EDGE('',*,*,#41568,.F.) ;
#60108=ORIENTED_EDGE('',*,*,#42904,.T.) ;
#60109=ORIENTED_EDGE('',*,*,#41572,.F.) ;
#60110=ORIENTED_EDGE('',*,*,#42905,.T.) ;
#60111=ORIENTED_EDGE('',*,*,#42906,.T.) ;
#60112=ORIENTED_EDGE('',*,*,#42907,.T.) ;
#60113=ORIENTED_EDGE('',*,*,#42908,.T.) ;
#60114=ORIENTED_EDGE('',*,*,#42909,.T.) ;
#60115=ORIENTED_EDGE('',*,*,#42910,.T.) ;
#60116=ORIENTED_EDGE('',*,*,#42911,.T.) ;
#60117=ORIENTED_EDGE('',*,*,#42912,.T.) ;
#60118=ORIENTED_EDGE('',*,*,#42913,.T.) ;
#60119=ORIENTED_EDGE('',*,*,#42914,.T.) ;
#60120=ORIENTED_EDGE('',*,*,#42915,.T.) ;
#60121=ORIENTED_EDGE('',*,*,#42916,.T.) ;
#60122=ORIENTED_EDGE('',*,*,#42917,.T.) ;
#60123=ORIENTED_EDGE('',*,*,#41566,.T.) ;
#60124=ORIENTED_EDGE('',*,*,#42918,.T.) ;
#60125=ORIENTED_EDGE('',*,*,#41570,.F.) ;
#60126=ORIENTED_EDGE('',*,*,#42919,.T.) ;
#60127=ORIENTED_EDGE('',*,*,#42920,.T.) ;
#60128=ORIENTED_EDGE('',*,*,#42921,.T.) ;
#60129=ORIENTED_EDGE('',*,*,#42922,.T.) ;
#60130=ORIENTED_EDGE('',*,*,#42923,.T.) ;
#60131=ORIENTED_EDGE('',*,*,#42924,.T.) ;
#60132=ORIENTED_EDGE('',*,*,#42925,.T.) ;
#60133=ORIENTED_EDGE('',*,*,#42926,.T.) ;
#60134=ORIENTED_EDGE('',*,*,#42927,.T.) ;
#60135=ORIENTED_EDGE('',*,*,#42928,.T.) ;
#60136=ORIENTED_EDGE('',*,*,#42929,.T.) ;
#60137=ORIENTED_EDGE('',*,*,#42930,.T.) ;
#60138=ORIENTED_EDGE('',*,*,#42931,.T.) ;
#60139=ORIENTED_EDGE('',*,*,#42932,.T.) ;
#60140=ORIENTED_EDGE('',*,*,#42933,.T.) ;
#60141=ORIENTED_EDGE('',*,*,#42934,.T.) ;
#60142=ORIENTED_EDGE('',*,*,#42935,.T.) ;
#60143=ORIENTED_EDGE('',*,*,#42936,.T.) ;
#60144=ORIENTED_EDGE('',*,*,#42937,.T.) ;
#60145=ORIENTED_EDGE('',*,*,#42938,.T.) ;
#60146=ORIENTED_EDGE('',*,*,#42939,.T.) ;
#60147=ORIENTED_EDGE('',*,*,#42940,.F.) ;
#60148=ORIENTED_EDGE('',*,*,#42941,.T.) ;
#60149=ORIENTED_EDGE('',*,*,#42942,.T.) ;
#60150=ORIENTED_EDGE('',*,*,#42943,.T.) ;
#60151=ORIENTED_EDGE('',*,*,#42294,.T.) ;
#60152=ORIENTED_EDGE('',*,*,#42944,.T.) ;
#60153=ORIENTED_EDGE('',*,*,#42945,.T.) ;
#60154=ORIENTED_EDGE('',*,*,#42946,.T.) ;
#60155=ORIENTED_EDGE('',*,*,#42947,.T.) ;
#60156=ORIENTED_EDGE('',*,*,#42948,.T.) ;
#60157=ORIENTED_EDGE('',*,*,#39154,.T.) ;
#60158=ORIENTED_EDGE('',*,*,#42949,.T.) ;
#60159=ORIENTED_EDGE('',*,*,#42950,.T.) ;
#60160=ORIENTED_EDGE('',*,*,#42951,.T.) ;
#60161=ORIENTED_EDGE('',*,*,#42291,.T.) ;
#60162=ORIENTED_EDGE('',*,*,#42952,.T.) ;
#60163=ORIENTED_EDGE('',*,*,#42922,.F.) ;
#60164=ORIENTED_EDGE('',*,*,#42953,.T.) ;
#60165=ORIENTED_EDGE('',*,*,#42292,.T.) ;
#60166=ORIENTED_EDGE('',*,*,#42940,.T.) ;
#60167=ORIENTED_EDGE('',*,*,#42954,.T.) ;
#60168=ORIENTED_EDGE('',*,*,#39373,.F.) ;
#60169=ORIENTED_EDGE('',*,*,#42955,.T.) ;
#60170=ORIENTED_EDGE('',*,*,#42956,.T.) ;
#60171=ORIENTED_EDGE('',*,*,#42957,.T.) ;
#60172=ORIENTED_EDGE('',*,*,#42958,.T.) ;
#60173=ORIENTED_EDGE('',*,*,#42959,.T.) ;
#60174=ORIENTED_EDGE('',*,*,#42960,.T.) ;
#60175=ORIENTED_EDGE('',*,*,#42961,.T.) ;
#60176=ORIENTED_EDGE('',*,*,#41576,.F.) ;
#60177=ORIENTED_EDGE('',*,*,#42962,.T.) ;
#60178=ORIENTED_EDGE('',*,*,#41580,.F.) ;
#60179=ORIENTED_EDGE('',*,*,#42963,.T.) ;
#60180=ORIENTED_EDGE('',*,*,#42964,.T.) ;
#60181=ORIENTED_EDGE('',*,*,#42965,.T.) ;
#60182=ORIENTED_EDGE('',*,*,#42966,.T.) ;
#60183=ORIENTED_EDGE('',*,*,#42967,.T.) ;
#60184=ORIENTED_EDGE('',*,*,#42968,.T.) ;
#60185=ORIENTED_EDGE('',*,*,#42969,.T.) ;
#60186=ORIENTED_EDGE('',*,*,#42970,.T.) ;
#60187=ORIENTED_EDGE('',*,*,#42971,.T.) ;
#60188=ORIENTED_EDGE('',*,*,#42972,.T.) ;
#60189=ORIENTED_EDGE('',*,*,#42973,.T.) ;
#60190=ORIENTED_EDGE('',*,*,#42974,.T.) ;
#60191=ORIENTED_EDGE('',*,*,#42975,.T.) ;
#60192=ORIENTED_EDGE('',*,*,#41574,.T.) ;
#60193=ORIENTED_EDGE('',*,*,#42976,.T.) ;
#60194=ORIENTED_EDGE('',*,*,#41578,.F.) ;
#60195=ORIENTED_EDGE('',*,*,#42977,.T.) ;
#60196=ORIENTED_EDGE('',*,*,#42978,.T.) ;
#60197=ORIENTED_EDGE('',*,*,#42979,.T.) ;
#60198=ORIENTED_EDGE('',*,*,#42980,.T.) ;
#60199=ORIENTED_EDGE('',*,*,#42981,.T.) ;
#60200=ORIENTED_EDGE('',*,*,#42982,.T.) ;
#60201=ORIENTED_EDGE('',*,*,#42983,.T.) ;
#60202=ORIENTED_EDGE('',*,*,#42984,.T.) ;
#60203=ORIENTED_EDGE('',*,*,#42985,.T.) ;
#60204=ORIENTED_EDGE('',*,*,#42986,.T.) ;
#60205=ORIENTED_EDGE('',*,*,#42987,.T.) ;
#60206=ORIENTED_EDGE('',*,*,#42988,.T.) ;
#60207=ORIENTED_EDGE('',*,*,#42989,.T.) ;
#60208=ORIENTED_EDGE('',*,*,#42990,.T.) ;
#60209=ORIENTED_EDGE('',*,*,#42991,.T.) ;
#60210=ORIENTED_EDGE('',*,*,#42992,.T.) ;
#60211=ORIENTED_EDGE('',*,*,#42993,.T.) ;
#60212=ORIENTED_EDGE('',*,*,#42994,.T.) ;
#60213=ORIENTED_EDGE('',*,*,#42995,.T.) ;
#60214=ORIENTED_EDGE('',*,*,#42996,.T.) ;
#60215=ORIENTED_EDGE('',*,*,#42997,.T.) ;
#60216=ORIENTED_EDGE('',*,*,#42998,.F.) ;
#60217=ORIENTED_EDGE('',*,*,#42999,.T.) ;
#60218=ORIENTED_EDGE('',*,*,#43000,.T.) ;
#60219=ORIENTED_EDGE('',*,*,#43001,.T.) ;
#60220=ORIENTED_EDGE('',*,*,#42382,.T.) ;
#60221=ORIENTED_EDGE('',*,*,#43002,.T.) ;
#60222=ORIENTED_EDGE('',*,*,#43003,.T.) ;
#60223=ORIENTED_EDGE('',*,*,#43004,.T.) ;
#60224=ORIENTED_EDGE('',*,*,#43005,.T.) ;
#60225=ORIENTED_EDGE('',*,*,#43006,.T.) ;
#60226=ORIENTED_EDGE('',*,*,#39137,.T.) ;
#60227=ORIENTED_EDGE('',*,*,#43007,.T.) ;
#60228=ORIENTED_EDGE('',*,*,#43008,.T.) ;
#60229=ORIENTED_EDGE('',*,*,#43009,.T.) ;
#60230=ORIENTED_EDGE('',*,*,#42379,.T.) ;
#60231=ORIENTED_EDGE('',*,*,#43010,.T.) ;
#60232=ORIENTED_EDGE('',*,*,#42980,.F.) ;
#60233=ORIENTED_EDGE('',*,*,#43011,.T.) ;
#60234=ORIENTED_EDGE('',*,*,#42380,.T.) ;
#60235=ORIENTED_EDGE('',*,*,#42998,.T.) ;
#60236=ORIENTED_EDGE('',*,*,#43012,.T.) ;
#60237=ORIENTED_EDGE('',*,*,#39362,.F.) ;
#60238=ORIENTED_EDGE('',*,*,#43013,.T.) ;
#60239=ORIENTED_EDGE('',*,*,#43014,.T.) ;
#60240=ORIENTED_EDGE('',*,*,#43015,.T.) ;
#60241=ORIENTED_EDGE('',*,*,#43016,.T.) ;
#60242=ORIENTED_EDGE('',*,*,#43017,.T.) ;
#60243=ORIENTED_EDGE('',*,*,#43018,.T.) ;
#60244=ORIENTED_EDGE('',*,*,#43019,.T.) ;
#60245=ORIENTED_EDGE('',*,*,#41584,.F.) ;
#60246=ORIENTED_EDGE('',*,*,#43020,.T.) ;
#60247=ORIENTED_EDGE('',*,*,#41588,.F.) ;
#60248=ORIENTED_EDGE('',*,*,#43021,.T.) ;
#60249=ORIENTED_EDGE('',*,*,#43022,.T.) ;
#60250=ORIENTED_EDGE('',*,*,#43023,.T.) ;
#60251=ORIENTED_EDGE('',*,*,#43024,.T.) ;
#60252=ORIENTED_EDGE('',*,*,#43025,.T.) ;
#60253=ORIENTED_EDGE('',*,*,#43026,.T.) ;
#60254=ORIENTED_EDGE('',*,*,#43027,.T.) ;
#60255=ORIENTED_EDGE('',*,*,#43028,.T.) ;
#60256=ORIENTED_EDGE('',*,*,#43029,.T.) ;
#60257=ORIENTED_EDGE('',*,*,#43030,.T.) ;
#60258=ORIENTED_EDGE('',*,*,#43031,.T.) ;
#60259=ORIENTED_EDGE('',*,*,#43032,.T.) ;
#60260=ORIENTED_EDGE('',*,*,#43033,.T.) ;
#60261=ORIENTED_EDGE('',*,*,#41582,.T.) ;
#60262=ORIENTED_EDGE('',*,*,#43034,.T.) ;
#60263=ORIENTED_EDGE('',*,*,#41586,.F.) ;
#60264=ORIENTED_EDGE('',*,*,#43035,.T.) ;
#60265=ORIENTED_EDGE('',*,*,#43036,.T.) ;
#60266=ORIENTED_EDGE('',*,*,#43037,.T.) ;
#60267=ORIENTED_EDGE('',*,*,#43038,.T.) ;
#60268=ORIENTED_EDGE('',*,*,#43039,.T.) ;
#60269=ORIENTED_EDGE('',*,*,#43040,.T.) ;
#60270=ORIENTED_EDGE('',*,*,#43041,.T.) ;
#60271=ORIENTED_EDGE('',*,*,#43042,.T.) ;
#60272=ORIENTED_EDGE('',*,*,#43043,.T.) ;
#60273=ORIENTED_EDGE('',*,*,#43044,.T.) ;
#60274=ORIENTED_EDGE('',*,*,#43045,.T.) ;
#60275=ORIENTED_EDGE('',*,*,#43046,.T.) ;
#60276=ORIENTED_EDGE('',*,*,#43047,.T.) ;
#60277=ORIENTED_EDGE('',*,*,#43048,.T.) ;
#60278=ORIENTED_EDGE('',*,*,#43049,.T.) ;
#60279=ORIENTED_EDGE('',*,*,#43050,.T.) ;
#60280=ORIENTED_EDGE('',*,*,#43051,.T.) ;
#60281=ORIENTED_EDGE('',*,*,#43052,.T.) ;
#60282=ORIENTED_EDGE('',*,*,#43053,.T.) ;
#60283=ORIENTED_EDGE('',*,*,#43054,.T.) ;
#60284=ORIENTED_EDGE('',*,*,#43055,.T.) ;
#60285=ORIENTED_EDGE('',*,*,#43056,.F.) ;
#60286=ORIENTED_EDGE('',*,*,#43057,.T.) ;
#60287=ORIENTED_EDGE('',*,*,#43058,.T.) ;
#60288=ORIENTED_EDGE('',*,*,#43059,.T.) ;
#60289=ORIENTED_EDGE('',*,*,#42470,.T.) ;
#60290=ORIENTED_EDGE('',*,*,#43060,.T.) ;
#60291=ORIENTED_EDGE('',*,*,#43061,.T.) ;
#60292=ORIENTED_EDGE('',*,*,#43062,.T.) ;
#60293=ORIENTED_EDGE('',*,*,#43063,.T.) ;
#60294=ORIENTED_EDGE('',*,*,#43064,.T.) ;
#60295=ORIENTED_EDGE('',*,*,#39120,.T.) ;
#60296=ORIENTED_EDGE('',*,*,#43065,.T.) ;
#60297=ORIENTED_EDGE('',*,*,#43066,.T.) ;
#60298=ORIENTED_EDGE('',*,*,#43067,.T.) ;
#60299=ORIENTED_EDGE('',*,*,#42467,.T.) ;
#60300=ORIENTED_EDGE('',*,*,#43068,.T.) ;
#60301=ORIENTED_EDGE('',*,*,#43038,.F.) ;
#60302=ORIENTED_EDGE('',*,*,#43069,.T.) ;
#60303=ORIENTED_EDGE('',*,*,#42468,.T.) ;
#60304=ORIENTED_EDGE('',*,*,#43056,.T.) ;
#60305=ORIENTED_EDGE('',*,*,#43070,.T.) ;
#60306=ORIENTED_EDGE('',*,*,#39351,.F.) ;
#60307=ORIENTED_EDGE('',*,*,#43071,.T.) ;
#60308=ORIENTED_EDGE('',*,*,#43072,.T.) ;
#60309=ORIENTED_EDGE('',*,*,#43073,.T.) ;
#60310=ORIENTED_EDGE('',*,*,#43074,.T.) ;
#60311=ORIENTED_EDGE('',*,*,#43075,.T.) ;
#60312=ORIENTED_EDGE('',*,*,#43076,.T.) ;
#60313=ORIENTED_EDGE('',*,*,#43077,.T.) ;
#60314=ORIENTED_EDGE('',*,*,#41592,.F.) ;
#60315=ORIENTED_EDGE('',*,*,#43078,.T.) ;
#60316=ORIENTED_EDGE('',*,*,#41596,.F.) ;
#60317=ORIENTED_EDGE('',*,*,#43079,.T.) ;
#60318=ORIENTED_EDGE('',*,*,#43080,.T.) ;
#60319=ORIENTED_EDGE('',*,*,#43081,.T.) ;
#60320=ORIENTED_EDGE('',*,*,#43082,.T.) ;
#60321=ORIENTED_EDGE('',*,*,#43083,.T.) ;
#60322=ORIENTED_EDGE('',*,*,#43084,.T.) ;
#60323=ORIENTED_EDGE('',*,*,#43085,.T.) ;
#60324=ORIENTED_EDGE('',*,*,#43086,.T.) ;
#60325=ORIENTED_EDGE('',*,*,#43087,.T.) ;
#60326=ORIENTED_EDGE('',*,*,#43088,.T.) ;
#60327=ORIENTED_EDGE('',*,*,#43089,.T.) ;
#60328=ORIENTED_EDGE('',*,*,#43090,.T.) ;
#60329=ORIENTED_EDGE('',*,*,#43091,.T.) ;
#60330=ORIENTED_EDGE('',*,*,#41590,.T.) ;
#60331=ORIENTED_EDGE('',*,*,#43092,.T.) ;
#60332=ORIENTED_EDGE('',*,*,#41594,.F.) ;
#60333=ORIENTED_EDGE('',*,*,#43093,.T.) ;
#60334=ORIENTED_EDGE('',*,*,#43094,.T.) ;
#60335=ORIENTED_EDGE('',*,*,#43095,.T.) ;
#60336=ORIENTED_EDGE('',*,*,#43096,.T.) ;
#60337=ORIENTED_EDGE('',*,*,#43097,.T.) ;
#60338=ORIENTED_EDGE('',*,*,#43098,.T.) ;
#60339=ORIENTED_EDGE('',*,*,#43099,.T.) ;
#60340=ORIENTED_EDGE('',*,*,#43100,.T.) ;
#60341=ORIENTED_EDGE('',*,*,#43101,.T.) ;
#60342=ORIENTED_EDGE('',*,*,#43102,.T.) ;
#60343=ORIENTED_EDGE('',*,*,#43103,.T.) ;
#60344=ORIENTED_EDGE('',*,*,#43104,.T.) ;
#60345=ORIENTED_EDGE('',*,*,#43105,.T.) ;
#60346=ORIENTED_EDGE('',*,*,#43106,.T.) ;
#60347=ORIENTED_EDGE('',*,*,#43107,.T.) ;
#60348=ORIENTED_EDGE('',*,*,#43108,.T.) ;
#60349=ORIENTED_EDGE('',*,*,#43109,.T.) ;
#60350=ORIENTED_EDGE('',*,*,#43110,.T.) ;
#60351=ORIENTED_EDGE('',*,*,#43111,.T.) ;
#60352=ORIENTED_EDGE('',*,*,#43112,.T.) ;
#60353=ORIENTED_EDGE('',*,*,#43113,.T.) ;
#60354=ORIENTED_EDGE('',*,*,#43114,.F.) ;
#60355=ORIENTED_EDGE('',*,*,#43115,.T.) ;
#60356=ORIENTED_EDGE('',*,*,#43116,.T.) ;
#60357=ORIENTED_EDGE('',*,*,#43117,.T.) ;
#60358=ORIENTED_EDGE('',*,*,#42558,.T.) ;
#60359=ORIENTED_EDGE('',*,*,#43118,.T.) ;
#60360=ORIENTED_EDGE('',*,*,#43119,.T.) ;
#60361=ORIENTED_EDGE('',*,*,#43120,.T.) ;
#60362=ORIENTED_EDGE('',*,*,#43121,.T.) ;
#60363=ORIENTED_EDGE('',*,*,#43122,.T.) ;
#60364=ORIENTED_EDGE('',*,*,#39103,.T.) ;
#60365=ORIENTED_EDGE('',*,*,#43123,.T.) ;
#60366=ORIENTED_EDGE('',*,*,#43124,.T.) ;
#60367=ORIENTED_EDGE('',*,*,#43125,.T.) ;
#60368=ORIENTED_EDGE('',*,*,#42555,.T.) ;
#60369=ORIENTED_EDGE('',*,*,#43126,.T.) ;
#60370=ORIENTED_EDGE('',*,*,#43096,.F.) ;
#60371=ORIENTED_EDGE('',*,*,#43127,.T.) ;
#60372=ORIENTED_EDGE('',*,*,#42556,.T.) ;
#60373=ORIENTED_EDGE('',*,*,#43114,.T.) ;
#60374=ORIENTED_EDGE('',*,*,#43128,.T.) ;
#60375=ORIENTED_EDGE('',*,*,#39340,.F.) ;
#60376=ORIENTED_EDGE('',*,*,#43129,.T.) ;
#60377=ORIENTED_EDGE('',*,*,#43130,.T.) ;
#60378=ORIENTED_EDGE('',*,*,#43131,.T.) ;
#60379=ORIENTED_EDGE('',*,*,#43132,.T.) ;
#60380=ORIENTED_EDGE('',*,*,#43133,.T.) ;
#60381=ORIENTED_EDGE('',*,*,#43134,.T.) ;
#60382=ORIENTED_EDGE('',*,*,#43135,.T.) ;
#60383=ORIENTED_EDGE('',*,*,#41600,.F.) ;
#60384=ORIENTED_EDGE('',*,*,#43136,.T.) ;
#60385=ORIENTED_EDGE('',*,*,#41604,.F.) ;
#60386=ORIENTED_EDGE('',*,*,#43137,.T.) ;
#60387=ORIENTED_EDGE('',*,*,#43138,.T.) ;
#60388=ORIENTED_EDGE('',*,*,#43139,.T.) ;
#60389=ORIENTED_EDGE('',*,*,#43140,.T.) ;
#60390=ORIENTED_EDGE('',*,*,#43141,.T.) ;
#60391=ORIENTED_EDGE('',*,*,#43142,.T.) ;
#60392=ORIENTED_EDGE('',*,*,#43143,.T.) ;
#60393=ORIENTED_EDGE('',*,*,#43144,.T.) ;
#60394=ORIENTED_EDGE('',*,*,#43145,.T.) ;
#60395=ORIENTED_EDGE('',*,*,#43146,.T.) ;
#60396=ORIENTED_EDGE('',*,*,#43147,.T.) ;
#60397=ORIENTED_EDGE('',*,*,#43148,.T.) ;
#60398=ORIENTED_EDGE('',*,*,#43149,.T.) ;
#60399=ORIENTED_EDGE('',*,*,#41598,.T.) ;
#60400=ORIENTED_EDGE('',*,*,#43150,.T.) ;
#60401=ORIENTED_EDGE('',*,*,#41602,.F.) ;
#60402=ORIENTED_EDGE('',*,*,#43151,.T.) ;
#60403=ORIENTED_EDGE('',*,*,#43152,.T.) ;
#60404=ORIENTED_EDGE('',*,*,#43153,.T.) ;
#60405=ORIENTED_EDGE('',*,*,#43154,.T.) ;
#60406=ORIENTED_EDGE('',*,*,#43155,.T.) ;
#60407=ORIENTED_EDGE('',*,*,#43156,.T.) ;
#60408=ORIENTED_EDGE('',*,*,#43157,.T.) ;
#60409=ORIENTED_EDGE('',*,*,#43158,.T.) ;
#60410=ORIENTED_EDGE('',*,*,#43159,.T.) ;
#60411=ORIENTED_EDGE('',*,*,#43160,.T.) ;
#60412=ORIENTED_EDGE('',*,*,#43161,.T.) ;
#60413=ORIENTED_EDGE('',*,*,#43162,.T.) ;
#60414=ORIENTED_EDGE('',*,*,#43163,.T.) ;
#60415=ORIENTED_EDGE('',*,*,#43164,.T.) ;
#60416=ORIENTED_EDGE('',*,*,#43165,.T.) ;
#60417=ORIENTED_EDGE('',*,*,#43166,.T.) ;
#60418=ORIENTED_EDGE('',*,*,#43167,.T.) ;
#60419=ORIENTED_EDGE('',*,*,#43168,.T.) ;
#60420=ORIENTED_EDGE('',*,*,#43169,.T.) ;
#60421=ORIENTED_EDGE('',*,*,#43170,.T.) ;
#60422=ORIENTED_EDGE('',*,*,#43171,.T.) ;
#60423=ORIENTED_EDGE('',*,*,#43172,.T.) ;
#60424=ORIENTED_EDGE('',*,*,#43173,.T.) ;
#60425=ORIENTED_EDGE('',*,*,#43174,.T.) ;
#60426=ORIENTED_EDGE('',*,*,#43175,.T.) ;
#60427=ORIENTED_EDGE('',*,*,#43176,.T.) ;
#60428=ORIENTED_EDGE('',*,*,#43177,.T.) ;
#60429=ORIENTED_EDGE('',*,*,#43178,.T.) ;
#60430=ORIENTED_EDGE('',*,*,#43179,.T.) ;
#60431=ORIENTED_EDGE('',*,*,#43180,.T.) ;
#60432=ORIENTED_EDGE('',*,*,#43181,.T.) ;
#60433=ORIENTED_EDGE('',*,*,#43182,.T.) ;
#60434=ORIENTED_EDGE('',*,*,#43183,.T.) ;
#60435=ORIENTED_EDGE('',*,*,#43184,.T.) ;
#60436=ORIENTED_EDGE('',*,*,#43185,.T.) ;
#60437=ORIENTED_EDGE('',*,*,#43186,.T.) ;
#60438=ORIENTED_EDGE('',*,*,#43187,.T.) ;
#60439=ORIENTED_EDGE('',*,*,#43188,.T.) ;
#60440=ORIENTED_EDGE('',*,*,#43189,.T.) ;
#60441=ORIENTED_EDGE('',*,*,#43190,.T.) ;
#60442=ORIENTED_EDGE('',*,*,#43191,.T.) ;
#60443=ORIENTED_EDGE('',*,*,#43192,.T.) ;
#60444=ORIENTED_EDGE('',*,*,#43193,.T.) ;
#60445=ORIENTED_EDGE('',*,*,#43194,.T.) ;
#60446=ORIENTED_EDGE('',*,*,#43195,.T.) ;
#60447=ORIENTED_EDGE('',*,*,#43196,.T.) ;
#60448=ORIENTED_EDGE('',*,*,#43197,.T.) ;
#60449=ORIENTED_EDGE('',*,*,#43198,.T.) ;
#60450=ORIENTED_EDGE('',*,*,#43199,.T.) ;
#60451=ORIENTED_EDGE('',*,*,#43200,.T.) ;
#60452=ORIENTED_EDGE('',*,*,#43201,.T.) ;
#60453=ORIENTED_EDGE('',*,*,#43202,.T.) ;
#60454=ORIENTED_EDGE('',*,*,#43203,.T.) ;
#60455=ORIENTED_EDGE('',*,*,#43204,.T.) ;
#60456=ORIENTED_EDGE('',*,*,#43205,.T.) ;
#60457=ORIENTED_EDGE('',*,*,#43206,.T.) ;
#60458=ORIENTED_EDGE('',*,*,#43207,.T.) ;
#60459=ORIENTED_EDGE('',*,*,#43208,.T.) ;
#60460=ORIENTED_EDGE('',*,*,#43209,.T.) ;
#60461=ORIENTED_EDGE('',*,*,#43210,.T.) ;
#60462=ORIENTED_EDGE('',*,*,#43211,.T.) ;
#60463=ORIENTED_EDGE('',*,*,#43212,.T.) ;
#60464=ORIENTED_EDGE('',*,*,#43213,.T.) ;
#60465=ORIENTED_EDGE('',*,*,#43214,.T.) ;
#60466=ORIENTED_EDGE('',*,*,#43215,.T.) ;
#60467=ORIENTED_EDGE('',*,*,#43216,.T.) ;
#60468=ORIENTED_EDGE('',*,*,#43217,.T.) ;
#60469=ORIENTED_EDGE('',*,*,#43218,.T.) ;
#60470=ORIENTED_EDGE('',*,*,#43219,.T.) ;
#60471=ORIENTED_EDGE('',*,*,#43220,.T.) ;
#60472=ORIENTED_EDGE('',*,*,#43221,.T.) ;
#60473=ORIENTED_EDGE('',*,*,#43222,.T.) ;
#60474=ORIENTED_EDGE('',*,*,#43223,.T.) ;
#60475=ORIENTED_EDGE('',*,*,#43224,.T.) ;
#60476=ORIENTED_EDGE('',*,*,#43225,.T.) ;
#60477=ORIENTED_EDGE('',*,*,#43226,.T.) ;
#60478=ORIENTED_EDGE('',*,*,#43227,.T.) ;
#60479=ORIENTED_EDGE('',*,*,#43228,.T.) ;
#60480=ORIENTED_EDGE('',*,*,#43229,.T.) ;
#60481=ORIENTED_EDGE('',*,*,#43230,.T.) ;
#60482=ORIENTED_EDGE('',*,*,#43231,.T.) ;
#60483=ORIENTED_EDGE('',*,*,#43232,.T.) ;
#60484=ORIENTED_EDGE('',*,*,#43233,.T.) ;
#60485=ORIENTED_EDGE('',*,*,#43234,.T.) ;
#60486=ORIENTED_EDGE('',*,*,#43235,.T.) ;
#60487=ORIENTED_EDGE('',*,*,#43236,.T.) ;
#60488=ORIENTED_EDGE('',*,*,#43237,.T.) ;
#60489=ORIENTED_EDGE('',*,*,#43238,.T.) ;
#60490=ORIENTED_EDGE('',*,*,#43239,.T.) ;
#60491=ORIENTED_EDGE('',*,*,#43240,.T.) ;
#60492=ORIENTED_EDGE('',*,*,#43241,.T.) ;
#60493=ORIENTED_EDGE('',*,*,#43242,.T.) ;
#60494=ORIENTED_EDGE('',*,*,#43243,.T.) ;
#60495=ORIENTED_EDGE('',*,*,#43244,.T.) ;
#60496=ORIENTED_EDGE('',*,*,#43245,.T.) ;
#60497=ORIENTED_EDGE('',*,*,#43246,.T.) ;
#60498=ORIENTED_EDGE('',*,*,#43247,.T.) ;
#60499=ORIENTED_EDGE('',*,*,#43248,.T.) ;
#60500=ORIENTED_EDGE('',*,*,#43249,.T.) ;
#60501=ORIENTED_EDGE('',*,*,#43250,.T.) ;
#60502=ORIENTED_EDGE('',*,*,#43251,.T.) ;
#60503=ORIENTED_EDGE('',*,*,#43252,.T.) ;
#60504=ORIENTED_EDGE('',*,*,#43253,.T.) ;
#60505=ORIENTED_EDGE('',*,*,#43254,.T.) ;
#60506=ORIENTED_EDGE('',*,*,#43255,.T.) ;
#60507=ORIENTED_EDGE('',*,*,#43256,.T.) ;
#60508=ORIENTED_EDGE('',*,*,#43257,.T.) ;
#60509=ORIENTED_EDGE('',*,*,#43258,.T.) ;
#60510=ORIENTED_EDGE('',*,*,#43259,.T.) ;
#60511=ORIENTED_EDGE('',*,*,#43260,.T.) ;
#60512=ORIENTED_EDGE('',*,*,#43261,.T.) ;
#60513=ORIENTED_EDGE('',*,*,#43262,.T.) ;
#60514=ORIENTED_EDGE('',*,*,#43263,.T.) ;
#60515=ORIENTED_EDGE('',*,*,#43264,.T.) ;
#60516=ORIENTED_EDGE('',*,*,#43265,.T.) ;
#60517=ORIENTED_EDGE('',*,*,#43266,.T.) ;
#60518=ORIENTED_EDGE('',*,*,#43267,.T.) ;
#60519=ORIENTED_EDGE('',*,*,#43268,.T.) ;
#60520=ORIENTED_EDGE('',*,*,#43269,.T.) ;
#60521=ORIENTED_EDGE('',*,*,#43270,.T.) ;
#60522=ORIENTED_EDGE('',*,*,#43271,.T.) ;
#60523=ORIENTED_EDGE('',*,*,#43272,.T.) ;
#60524=ORIENTED_EDGE('',*,*,#43273,.T.) ;
#60525=ORIENTED_EDGE('',*,*,#43274,.T.) ;
#60526=ORIENTED_EDGE('',*,*,#43275,.T.) ;
#60527=ORIENTED_EDGE('',*,*,#43276,.T.) ;
#60528=ORIENTED_EDGE('',*,*,#43277,.T.) ;
#60529=ORIENTED_EDGE('',*,*,#43278,.T.) ;
#60530=ORIENTED_EDGE('',*,*,#43279,.T.) ;
#60531=ORIENTED_EDGE('',*,*,#43280,.T.) ;
#60532=ORIENTED_EDGE('',*,*,#43281,.T.) ;
#60533=ORIENTED_EDGE('',*,*,#43282,.T.) ;
#60534=ORIENTED_EDGE('',*,*,#43283,.T.) ;
#60535=ORIENTED_EDGE('',*,*,#43284,.T.) ;
#60536=ORIENTED_EDGE('',*,*,#43285,.T.) ;
#60537=ORIENTED_EDGE('',*,*,#43286,.T.) ;
#60538=ORIENTED_EDGE('',*,*,#43287,.T.) ;
#60539=ORIENTED_EDGE('',*,*,#43288,.T.) ;
#60540=ORIENTED_EDGE('',*,*,#43289,.T.) ;
#60541=ORIENTED_EDGE('',*,*,#43290,.T.) ;
#60542=ORIENTED_EDGE('',*,*,#43291,.T.) ;
#60543=ORIENTED_EDGE('',*,*,#43292,.T.) ;
#60544=ORIENTED_EDGE('',*,*,#43293,.T.) ;
#60545=ORIENTED_EDGE('',*,*,#43294,.T.) ;
#60546=ORIENTED_EDGE('',*,*,#43295,.T.) ;
#60547=ORIENTED_EDGE('',*,*,#43296,.T.) ;
#60548=ORIENTED_EDGE('',*,*,#43297,.T.) ;
#60549=ORIENTED_EDGE('',*,*,#43220,.F.) ;
#60550=ORIENTED_EDGE('',*,*,#43298,.T.) ;
#60551=ORIENTED_EDGE('',*,*,#42647,.F.) ;
#60552=ORIENTED_EDGE('',*,*,#43299,.F.) ;
#60553=ORIENTED_EDGE('',*,*,#42644,.F.) ;
#60554=ORIENTED_EDGE('',*,*,#43300,.T.) ;
#60555=ORIENTED_EDGE('',*,*,#42648,.F.) ;
#60556=ORIENTED_EDGE('',*,*,#43301,.T.) ;
#60557=ORIENTED_EDGE('',*,*,#43302,.F.) ;
#60558=ORIENTED_EDGE('',*,*,#43299,.T.) ;
#60559=ORIENTED_EDGE('',*,*,#43303,.F.) ;
#60560=ORIENTED_EDGE('',*,*,#42645,.F.) ;
#60561=ORIENTED_EDGE('',*,*,#43304,.T.) ;
#60562=ORIENTED_EDGE('',*,*,#43222,.F.) ;
#60563=ORIENTED_EDGE('',*,*,#43305,.F.) ;
#60564=ORIENTED_EDGE('',*,*,#43303,.T.) ;
#60565=ORIENTED_EDGE('',*,*,#42646,.F.) ;
#60566=ORIENTED_EDGE('',*,*,#43306,.F.) ;
#60567=ORIENTED_EDGE('',*,*,#42640,.F.) ;
#60568=ORIENTED_EDGE('',*,*,#43302,.T.) ;
#60569=ORIENTED_EDGE('',*,*,#42643,.F.) ;
#60570=ORIENTED_EDGE('',*,*,#43307,.F.) ;
#60571=ORIENTED_EDGE('',*,*,#43221,.F.) ;
#60572=ORIENTED_EDGE('',*,*,#43306,.T.) ;
#60573=ORIENTED_EDGE('',*,*,#43305,.T.) ;
#60574=ORIENTED_EDGE('',*,*,#43308,.F.) ;
#60575=ORIENTED_EDGE('',*,*,#43309,.F.) ;
#60576=ORIENTED_EDGE('',*,*,#43307,.T.) ;
#60577=ORIENTED_EDGE('',*,*,#43310,.F.) ;
#60578=ORIENTED_EDGE('',*,*,#43308,.T.) ;
#60579=ORIENTED_EDGE('',*,*,#43225,.F.) ;
#60580=ORIENTED_EDGE('',*,*,#43311,.F.) ;
#60581=ORIENTED_EDGE('',*,*,#42641,.F.) ;
#60582=ORIENTED_EDGE('',*,*,#43310,.T.) ;
#60583=ORIENTED_EDGE('',*,*,#42642,.F.) ;
#60584=ORIENTED_EDGE('',*,*,#43312,.F.) ;
#60585=ORIENTED_EDGE('',*,*,#42636,.F.) ;
#60586=ORIENTED_EDGE('',*,*,#42639,.F.) ;
#60587=ORIENTED_EDGE('',*,*,#43313,.T.) ;
#60588=ORIENTED_EDGE('',*,*,#43218,.F.) ;
#60589=ORIENTED_EDGE('',*,*,#43309,.T.) ;
#60590=ORIENTED_EDGE('',*,*,#43312,.T.) ;
#60591=ORIENTED_EDGE('',*,*,#43311,.T.) ;
#60592=ORIENTED_EDGE('',*,*,#43314,.F.) ;
#60593=ORIENTED_EDGE('',*,*,#42634,.F.) ;
#60594=ORIENTED_EDGE('',*,*,#43315,.T.) ;
#60595=ORIENTED_EDGE('',*,*,#42638,.F.) ;
#60596=ORIENTED_EDGE('',*,*,#43316,.T.) ;
#60597=ORIENTED_EDGE('',*,*,#43224,.F.) ;
#60598=ORIENTED_EDGE('',*,*,#43317,.T.) ;
#60599=ORIENTED_EDGE('',*,*,#42637,.F.) ;
#60600=ORIENTED_EDGE('',*,*,#43314,.T.) ;
#60601=ORIENTED_EDGE('',*,*,#43292,.F.) ;
#60602=ORIENTED_EDGE('',*,*,#43318,.T.) ;
#60603=ORIENTED_EDGE('',*,*,#42669,.F.) ;
#60604=ORIENTED_EDGE('',*,*,#43319,.F.) ;
#60605=ORIENTED_EDGE('',*,*,#42666,.F.) ;
#60606=ORIENTED_EDGE('',*,*,#43320,.T.) ;
#60607=ORIENTED_EDGE('',*,*,#42670,.F.) ;
#60608=ORIENTED_EDGE('',*,*,#43321,.T.) ;
#60609=ORIENTED_EDGE('',*,*,#43322,.F.) ;
#60610=ORIENTED_EDGE('',*,*,#43319,.T.) ;
#60611=ORIENTED_EDGE('',*,*,#43323,.F.) ;
#60612=ORIENTED_EDGE('',*,*,#42667,.F.) ;
#60613=ORIENTED_EDGE('',*,*,#43324,.T.) ;
#60614=ORIENTED_EDGE('',*,*,#43294,.F.) ;
#60615=ORIENTED_EDGE('',*,*,#43325,.F.) ;
#60616=ORIENTED_EDGE('',*,*,#43323,.T.) ;
#60617=ORIENTED_EDGE('',*,*,#42668,.F.) ;
#60618=ORIENTED_EDGE('',*,*,#43326,.F.) ;
#60619=ORIENTED_EDGE('',*,*,#42682,.F.) ;
#60620=ORIENTED_EDGE('',*,*,#43322,.T.) ;
#60621=ORIENTED_EDGE('',*,*,#42681,.F.) ;
#60622=ORIENTED_EDGE('',*,*,#43327,.F.) ;
#60623=ORIENTED_EDGE('',*,*,#43293,.F.) ;
#60624=ORIENTED_EDGE('',*,*,#43326,.T.) ;
#60625=ORIENTED_EDGE('',*,*,#43325,.T.) ;
#60626=ORIENTED_EDGE('',*,*,#43328,.F.) ;
#60627=ORIENTED_EDGE('',*,*,#43329,.F.) ;
#60628=ORIENTED_EDGE('',*,*,#43327,.T.) ;
#60629=ORIENTED_EDGE('',*,*,#43330,.F.) ;
#60630=ORIENTED_EDGE('',*,*,#43328,.T.) ;
#60631=ORIENTED_EDGE('',*,*,#43297,.F.) ;
#60632=ORIENTED_EDGE('',*,*,#43331,.F.) ;
#60633=ORIENTED_EDGE('',*,*,#42683,.F.) ;
#60634=ORIENTED_EDGE('',*,*,#43330,.T.) ;
#60635=ORIENTED_EDGE('',*,*,#42680,.F.) ;
#60636=ORIENTED_EDGE('',*,*,#43332,.F.) ;
#60637=ORIENTED_EDGE('',*,*,#42676,.F.) ;
#60638=ORIENTED_EDGE('',*,*,#42679,.F.) ;
#60639=ORIENTED_EDGE('',*,*,#43333,.T.) ;
#60640=ORIENTED_EDGE('',*,*,#43290,.F.) ;
#60641=ORIENTED_EDGE('',*,*,#43329,.T.) ;
#60642=ORIENTED_EDGE('',*,*,#43332,.T.) ;
#60643=ORIENTED_EDGE('',*,*,#43331,.T.) ;
#60644=ORIENTED_EDGE('',*,*,#43334,.F.) ;
#60645=ORIENTED_EDGE('',*,*,#42674,.F.) ;
#60646=ORIENTED_EDGE('',*,*,#43335,.T.) ;
#60647=ORIENTED_EDGE('',*,*,#42678,.F.) ;
#60648=ORIENTED_EDGE('',*,*,#43336,.T.) ;
#60649=ORIENTED_EDGE('',*,*,#43296,.F.) ;
#60650=ORIENTED_EDGE('',*,*,#43337,.T.) ;
#60651=ORIENTED_EDGE('',*,*,#42677,.F.) ;
#60652=ORIENTED_EDGE('',*,*,#43334,.T.) ;
#60653=ORIENTED_EDGE('',*,*,#43212,.F.) ;
#60654=ORIENTED_EDGE('',*,*,#43338,.T.) ;
#60655=ORIENTED_EDGE('',*,*,#42705,.F.) ;
#60656=ORIENTED_EDGE('',*,*,#43339,.F.) ;
#60657=ORIENTED_EDGE('',*,*,#42702,.F.) ;
#60658=ORIENTED_EDGE('',*,*,#43340,.T.) ;
#60659=ORIENTED_EDGE('',*,*,#42706,.F.) ;
#60660=ORIENTED_EDGE('',*,*,#43341,.T.) ;
#60661=ORIENTED_EDGE('',*,*,#43342,.F.) ;
#60662=ORIENTED_EDGE('',*,*,#43339,.T.) ;
#60663=ORIENTED_EDGE('',*,*,#43343,.F.) ;
#60664=ORIENTED_EDGE('',*,*,#42703,.F.) ;
#60665=ORIENTED_EDGE('',*,*,#43344,.T.) ;
#60666=ORIENTED_EDGE('',*,*,#43214,.F.) ;
#60667=ORIENTED_EDGE('',*,*,#43345,.F.) ;
#60668=ORIENTED_EDGE('',*,*,#43343,.T.) ;
#60669=ORIENTED_EDGE('',*,*,#42704,.F.) ;
#60670=ORIENTED_EDGE('',*,*,#43346,.F.) ;
#60671=ORIENTED_EDGE('',*,*,#42698,.F.) ;
#60672=ORIENTED_EDGE('',*,*,#43342,.T.) ;
#60673=ORIENTED_EDGE('',*,*,#42701,.F.) ;
#60674=ORIENTED_EDGE('',*,*,#43347,.F.) ;
#60675=ORIENTED_EDGE('',*,*,#43213,.F.) ;
#60676=ORIENTED_EDGE('',*,*,#43346,.T.) ;
#60677=ORIENTED_EDGE('',*,*,#43345,.T.) ;
#60678=ORIENTED_EDGE('',*,*,#43348,.F.) ;
#60679=ORIENTED_EDGE('',*,*,#43349,.F.) ;
#60680=ORIENTED_EDGE('',*,*,#43347,.T.) ;
#60681=ORIENTED_EDGE('',*,*,#43350,.F.) ;
#60682=ORIENTED_EDGE('',*,*,#43348,.T.) ;
#60683=ORIENTED_EDGE('',*,*,#43217,.F.) ;
#60684=ORIENTED_EDGE('',*,*,#43351,.F.) ;
#60685=ORIENTED_EDGE('',*,*,#42699,.F.) ;
#60686=ORIENTED_EDGE('',*,*,#43350,.T.) ;
#60687=ORIENTED_EDGE('',*,*,#42700,.F.) ;
#60688=ORIENTED_EDGE('',*,*,#43352,.F.) ;
#60689=ORIENTED_EDGE('',*,*,#42694,.F.) ;
#60690=ORIENTED_EDGE('',*,*,#42697,.F.) ;
#60691=ORIENTED_EDGE('',*,*,#43353,.T.) ;
#60692=ORIENTED_EDGE('',*,*,#43210,.F.) ;
#60693=ORIENTED_EDGE('',*,*,#43349,.T.) ;
#60694=ORIENTED_EDGE('',*,*,#43352,.T.) ;
#60695=ORIENTED_EDGE('',*,*,#43351,.T.) ;
#60696=ORIENTED_EDGE('',*,*,#43354,.F.) ;
#60697=ORIENTED_EDGE('',*,*,#42692,.F.) ;
#60698=ORIENTED_EDGE('',*,*,#43355,.T.) ;
#60699=ORIENTED_EDGE('',*,*,#42696,.F.) ;
#60700=ORIENTED_EDGE('',*,*,#43356,.T.) ;
#60701=ORIENTED_EDGE('',*,*,#43216,.F.) ;
#60702=ORIENTED_EDGE('',*,*,#43357,.T.) ;
#60703=ORIENTED_EDGE('',*,*,#42695,.F.) ;
#60704=ORIENTED_EDGE('',*,*,#43354,.T.) ;
#60705=ORIENTED_EDGE('',*,*,#43284,.F.) ;
#60706=ORIENTED_EDGE('',*,*,#43358,.T.) ;
#60707=ORIENTED_EDGE('',*,*,#42727,.F.) ;
#60708=ORIENTED_EDGE('',*,*,#43359,.F.) ;
#60709=ORIENTED_EDGE('',*,*,#42724,.F.) ;
#60710=ORIENTED_EDGE('',*,*,#43360,.T.) ;
#60711=ORIENTED_EDGE('',*,*,#42728,.F.) ;
#60712=ORIENTED_EDGE('',*,*,#43361,.T.) ;
#60713=ORIENTED_EDGE('',*,*,#43362,.F.) ;
#60714=ORIENTED_EDGE('',*,*,#43359,.T.) ;
#60715=ORIENTED_EDGE('',*,*,#43363,.F.) ;
#60716=ORIENTED_EDGE('',*,*,#42725,.F.) ;
#60717=ORIENTED_EDGE('',*,*,#43364,.T.) ;
#60718=ORIENTED_EDGE('',*,*,#43286,.F.) ;
#60719=ORIENTED_EDGE('',*,*,#43365,.F.) ;
#60720=ORIENTED_EDGE('',*,*,#43363,.T.) ;
#60721=ORIENTED_EDGE('',*,*,#42726,.F.) ;
#60722=ORIENTED_EDGE('',*,*,#43366,.F.) ;
#60723=ORIENTED_EDGE('',*,*,#42740,.F.) ;
#60724=ORIENTED_EDGE('',*,*,#43362,.T.) ;
#60725=ORIENTED_EDGE('',*,*,#42739,.F.) ;
#60726=ORIENTED_EDGE('',*,*,#43367,.F.) ;
#60727=ORIENTED_EDGE('',*,*,#43285,.F.) ;
#60728=ORIENTED_EDGE('',*,*,#43366,.T.) ;
#60729=ORIENTED_EDGE('',*,*,#43365,.T.) ;
#60730=ORIENTED_EDGE('',*,*,#43368,.F.) ;
#60731=ORIENTED_EDGE('',*,*,#43369,.F.) ;
#60732=ORIENTED_EDGE('',*,*,#43367,.T.) ;
#60733=ORIENTED_EDGE('',*,*,#43370,.F.) ;
#60734=ORIENTED_EDGE('',*,*,#43368,.T.) ;
#60735=ORIENTED_EDGE('',*,*,#43289,.F.) ;
#60736=ORIENTED_EDGE('',*,*,#43371,.F.) ;
#60737=ORIENTED_EDGE('',*,*,#42741,.F.) ;
#60738=ORIENTED_EDGE('',*,*,#43370,.T.) ;
#60739=ORIENTED_EDGE('',*,*,#42738,.F.) ;
#60740=ORIENTED_EDGE('',*,*,#43372,.F.) ;
#60741=ORIENTED_EDGE('',*,*,#42734,.F.) ;
#60742=ORIENTED_EDGE('',*,*,#42737,.F.) ;
#60743=ORIENTED_EDGE('',*,*,#43373,.T.) ;
#60744=ORIENTED_EDGE('',*,*,#43282,.F.) ;
#60745=ORIENTED_EDGE('',*,*,#43369,.T.) ;
#60746=ORIENTED_EDGE('',*,*,#43372,.T.) ;
#60747=ORIENTED_EDGE('',*,*,#43371,.T.) ;
#60748=ORIENTED_EDGE('',*,*,#43374,.F.) ;
#60749=ORIENTED_EDGE('',*,*,#42732,.F.) ;
#60750=ORIENTED_EDGE('',*,*,#43375,.T.) ;
#60751=ORIENTED_EDGE('',*,*,#42736,.F.) ;
#60752=ORIENTED_EDGE('',*,*,#43376,.T.) ;
#60753=ORIENTED_EDGE('',*,*,#43288,.F.) ;
#60754=ORIENTED_EDGE('',*,*,#43377,.T.) ;
#60755=ORIENTED_EDGE('',*,*,#42735,.F.) ;
#60756=ORIENTED_EDGE('',*,*,#43374,.T.) ;
#60757=ORIENTED_EDGE('',*,*,#43204,.F.) ;
#60758=ORIENTED_EDGE('',*,*,#43378,.T.) ;
#60759=ORIENTED_EDGE('',*,*,#42763,.F.) ;
#60760=ORIENTED_EDGE('',*,*,#43379,.F.) ;
#60761=ORIENTED_EDGE('',*,*,#42760,.F.) ;
#60762=ORIENTED_EDGE('',*,*,#43380,.T.) ;
#60763=ORIENTED_EDGE('',*,*,#42764,.F.) ;
#60764=ORIENTED_EDGE('',*,*,#43381,.T.) ;
#60765=ORIENTED_EDGE('',*,*,#43382,.F.) ;
#60766=ORIENTED_EDGE('',*,*,#43379,.T.) ;
#60767=ORIENTED_EDGE('',*,*,#43383,.F.) ;
#60768=ORIENTED_EDGE('',*,*,#42761,.F.) ;
#60769=ORIENTED_EDGE('',*,*,#43384,.T.) ;
#60770=ORIENTED_EDGE('',*,*,#43206,.F.) ;
#60771=ORIENTED_EDGE('',*,*,#43385,.F.) ;
#60772=ORIENTED_EDGE('',*,*,#43383,.T.) ;
#60773=ORIENTED_EDGE('',*,*,#42762,.F.) ;
#60774=ORIENTED_EDGE('',*,*,#43386,.F.) ;
#60775=ORIENTED_EDGE('',*,*,#42756,.F.) ;
#60776=ORIENTED_EDGE('',*,*,#43382,.T.) ;
#60777=ORIENTED_EDGE('',*,*,#42759,.F.) ;
#60778=ORIENTED_EDGE('',*,*,#43387,.F.) ;
#60779=ORIENTED_EDGE('',*,*,#43205,.F.) ;
#60780=ORIENTED_EDGE('',*,*,#43386,.T.) ;
#60781=ORIENTED_EDGE('',*,*,#43385,.T.) ;
#60782=ORIENTED_EDGE('',*,*,#43388,.F.) ;
#60783=ORIENTED_EDGE('',*,*,#43389,.F.) ;
#60784=ORIENTED_EDGE('',*,*,#43387,.T.) ;
#60785=ORIENTED_EDGE('',*,*,#43390,.F.) ;
#60786=ORIENTED_EDGE('',*,*,#43388,.T.) ;
#60787=ORIENTED_EDGE('',*,*,#43209,.F.) ;
#60788=ORIENTED_EDGE('',*,*,#43391,.F.) ;
#60789=ORIENTED_EDGE('',*,*,#42757,.F.) ;
#60790=ORIENTED_EDGE('',*,*,#43390,.T.) ;
#60791=ORIENTED_EDGE('',*,*,#42758,.F.) ;
#60792=ORIENTED_EDGE('',*,*,#43392,.F.) ;
#60793=ORIENTED_EDGE('',*,*,#42752,.F.) ;
#60794=ORIENTED_EDGE('',*,*,#42755,.F.) ;
#60795=ORIENTED_EDGE('',*,*,#43393,.T.) ;
#60796=ORIENTED_EDGE('',*,*,#43202,.F.) ;
#60797=ORIENTED_EDGE('',*,*,#43389,.T.) ;
#60798=ORIENTED_EDGE('',*,*,#43392,.T.) ;
#60799=ORIENTED_EDGE('',*,*,#43391,.T.) ;
#60800=ORIENTED_EDGE('',*,*,#43394,.F.) ;
#60801=ORIENTED_EDGE('',*,*,#42750,.F.) ;
#60802=ORIENTED_EDGE('',*,*,#43395,.T.) ;
#60803=ORIENTED_EDGE('',*,*,#42754,.F.) ;
#60804=ORIENTED_EDGE('',*,*,#43396,.T.) ;
#60805=ORIENTED_EDGE('',*,*,#43208,.F.) ;
#60806=ORIENTED_EDGE('',*,*,#43397,.T.) ;
#60807=ORIENTED_EDGE('',*,*,#42753,.F.) ;
#60808=ORIENTED_EDGE('',*,*,#43394,.T.) ;
#60809=ORIENTED_EDGE('',*,*,#43276,.F.) ;
#60810=ORIENTED_EDGE('',*,*,#43398,.T.) ;
#60811=ORIENTED_EDGE('',*,*,#42785,.F.) ;
#60812=ORIENTED_EDGE('',*,*,#43399,.F.) ;
#60813=ORIENTED_EDGE('',*,*,#42782,.F.) ;
#60814=ORIENTED_EDGE('',*,*,#43400,.T.) ;
#60815=ORIENTED_EDGE('',*,*,#42786,.F.) ;
#60816=ORIENTED_EDGE('',*,*,#43401,.T.) ;
#60817=ORIENTED_EDGE('',*,*,#43402,.F.) ;
#60818=ORIENTED_EDGE('',*,*,#43399,.T.) ;
#60819=ORIENTED_EDGE('',*,*,#43403,.F.) ;
#60820=ORIENTED_EDGE('',*,*,#42783,.F.) ;
#60821=ORIENTED_EDGE('',*,*,#43404,.T.) ;
#60822=ORIENTED_EDGE('',*,*,#43278,.F.) ;
#60823=ORIENTED_EDGE('',*,*,#43405,.F.) ;
#60824=ORIENTED_EDGE('',*,*,#43403,.T.) ;
#60825=ORIENTED_EDGE('',*,*,#42784,.F.) ;
#60826=ORIENTED_EDGE('',*,*,#43406,.F.) ;
#60827=ORIENTED_EDGE('',*,*,#42798,.F.) ;
#60828=ORIENTED_EDGE('',*,*,#43402,.T.) ;
#60829=ORIENTED_EDGE('',*,*,#42797,.F.) ;
#60830=ORIENTED_EDGE('',*,*,#43407,.F.) ;
#60831=ORIENTED_EDGE('',*,*,#43277,.F.) ;
#60832=ORIENTED_EDGE('',*,*,#43406,.T.) ;
#60833=ORIENTED_EDGE('',*,*,#43405,.T.) ;
#60834=ORIENTED_EDGE('',*,*,#43408,.F.) ;
#60835=ORIENTED_EDGE('',*,*,#43409,.F.) ;
#60836=ORIENTED_EDGE('',*,*,#43407,.T.) ;
#60837=ORIENTED_EDGE('',*,*,#43410,.F.) ;
#60838=ORIENTED_EDGE('',*,*,#43408,.T.) ;
#60839=ORIENTED_EDGE('',*,*,#43281,.F.) ;
#60840=ORIENTED_EDGE('',*,*,#43411,.F.) ;
#60841=ORIENTED_EDGE('',*,*,#42799,.F.) ;
#60842=ORIENTED_EDGE('',*,*,#43410,.T.) ;
#60843=ORIENTED_EDGE('',*,*,#42796,.F.) ;
#60844=ORIENTED_EDGE('',*,*,#43412,.F.) ;
#60845=ORIENTED_EDGE('',*,*,#42792,.F.) ;
#60846=ORIENTED_EDGE('',*,*,#42795,.F.) ;
#60847=ORIENTED_EDGE('',*,*,#43413,.T.) ;
#60848=ORIENTED_EDGE('',*,*,#43274,.F.) ;
#60849=ORIENTED_EDGE('',*,*,#43409,.T.) ;
#60850=ORIENTED_EDGE('',*,*,#43412,.T.) ;
#60851=ORIENTED_EDGE('',*,*,#43411,.T.) ;
#60852=ORIENTED_EDGE('',*,*,#43414,.F.) ;
#60853=ORIENTED_EDGE('',*,*,#42790,.F.) ;
#60854=ORIENTED_EDGE('',*,*,#43415,.T.) ;
#60855=ORIENTED_EDGE('',*,*,#42794,.F.) ;
#60856=ORIENTED_EDGE('',*,*,#43416,.T.) ;
#60857=ORIENTED_EDGE('',*,*,#43280,.F.) ;
#60858=ORIENTED_EDGE('',*,*,#43417,.T.) ;
#60859=ORIENTED_EDGE('',*,*,#42793,.F.) ;
#60860=ORIENTED_EDGE('',*,*,#43414,.T.) ;
#60861=ORIENTED_EDGE('',*,*,#43196,.F.) ;
#60862=ORIENTED_EDGE('',*,*,#43418,.T.) ;
#60863=ORIENTED_EDGE('',*,*,#42821,.F.) ;
#60864=ORIENTED_EDGE('',*,*,#43419,.F.) ;
#60865=ORIENTED_EDGE('',*,*,#42818,.F.) ;
#60866=ORIENTED_EDGE('',*,*,#43420,.T.) ;
#60867=ORIENTED_EDGE('',*,*,#42822,.F.) ;
#60868=ORIENTED_EDGE('',*,*,#43421,.T.) ;
#60869=ORIENTED_EDGE('',*,*,#43422,.F.) ;
#60870=ORIENTED_EDGE('',*,*,#43419,.T.) ;
#60871=ORIENTED_EDGE('',*,*,#43423,.F.) ;
#60872=ORIENTED_EDGE('',*,*,#42819,.F.) ;
#60873=ORIENTED_EDGE('',*,*,#43424,.T.) ;
#60874=ORIENTED_EDGE('',*,*,#43198,.F.) ;
#60875=ORIENTED_EDGE('',*,*,#43425,.F.) ;
#60876=ORIENTED_EDGE('',*,*,#43423,.T.) ;
#60877=ORIENTED_EDGE('',*,*,#42820,.F.) ;
#60878=ORIENTED_EDGE('',*,*,#43426,.F.) ;
#60879=ORIENTED_EDGE('',*,*,#42814,.F.) ;
#60880=ORIENTED_EDGE('',*,*,#43422,.T.) ;
#60881=ORIENTED_EDGE('',*,*,#42817,.F.) ;
#60882=ORIENTED_EDGE('',*,*,#43427,.F.) ;
#60883=ORIENTED_EDGE('',*,*,#43197,.F.) ;
#60884=ORIENTED_EDGE('',*,*,#43426,.T.) ;
#60885=ORIENTED_EDGE('',*,*,#43425,.T.) ;
#60886=ORIENTED_EDGE('',*,*,#43428,.F.) ;
#60887=ORIENTED_EDGE('',*,*,#43429,.F.) ;
#60888=ORIENTED_EDGE('',*,*,#43427,.T.) ;
#60889=ORIENTED_EDGE('',*,*,#43430,.F.) ;
#60890=ORIENTED_EDGE('',*,*,#43428,.T.) ;
#60891=ORIENTED_EDGE('',*,*,#43201,.F.) ;
#60892=ORIENTED_EDGE('',*,*,#43431,.F.) ;
#60893=ORIENTED_EDGE('',*,*,#42815,.F.) ;
#60894=ORIENTED_EDGE('',*,*,#43430,.T.) ;
#60895=ORIENTED_EDGE('',*,*,#42816,.F.) ;
#60896=ORIENTED_EDGE('',*,*,#43432,.F.) ;
#60897=ORIENTED_EDGE('',*,*,#42810,.F.) ;
#60898=ORIENTED_EDGE('',*,*,#42813,.F.) ;
#60899=ORIENTED_EDGE('',*,*,#43433,.T.) ;
#60900=ORIENTED_EDGE('',*,*,#43194,.F.) ;
#60901=ORIENTED_EDGE('',*,*,#43429,.T.) ;
#60902=ORIENTED_EDGE('',*,*,#43432,.T.) ;
#60903=ORIENTED_EDGE('',*,*,#43431,.T.) ;
#60904=ORIENTED_EDGE('',*,*,#43434,.F.) ;
#60905=ORIENTED_EDGE('',*,*,#42808,.F.) ;
#60906=ORIENTED_EDGE('',*,*,#43435,.T.) ;
#60907=ORIENTED_EDGE('',*,*,#42812,.F.) ;
#60908=ORIENTED_EDGE('',*,*,#43436,.T.) ;
#60909=ORIENTED_EDGE('',*,*,#43200,.F.) ;
#60910=ORIENTED_EDGE('',*,*,#43437,.T.) ;
#60911=ORIENTED_EDGE('',*,*,#42811,.F.) ;
#60912=ORIENTED_EDGE('',*,*,#43434,.T.) ;
#60913=ORIENTED_EDGE('',*,*,#43268,.F.) ;
#60914=ORIENTED_EDGE('',*,*,#43438,.T.) ;
#60915=ORIENTED_EDGE('',*,*,#42843,.F.) ;
#60916=ORIENTED_EDGE('',*,*,#43439,.F.) ;
#60917=ORIENTED_EDGE('',*,*,#42840,.F.) ;
#60918=ORIENTED_EDGE('',*,*,#43440,.T.) ;
#60919=ORIENTED_EDGE('',*,*,#42844,.F.) ;
#60920=ORIENTED_EDGE('',*,*,#43441,.T.) ;
#60921=ORIENTED_EDGE('',*,*,#43442,.F.) ;
#60922=ORIENTED_EDGE('',*,*,#43439,.T.) ;
#60923=ORIENTED_EDGE('',*,*,#43443,.F.) ;
#60924=ORIENTED_EDGE('',*,*,#42841,.F.) ;
#60925=ORIENTED_EDGE('',*,*,#43444,.T.) ;
#60926=ORIENTED_EDGE('',*,*,#43270,.F.) ;
#60927=ORIENTED_EDGE('',*,*,#43445,.F.) ;
#60928=ORIENTED_EDGE('',*,*,#43443,.T.) ;
#60929=ORIENTED_EDGE('',*,*,#42842,.F.) ;
#60930=ORIENTED_EDGE('',*,*,#43446,.F.) ;
#60931=ORIENTED_EDGE('',*,*,#42856,.F.) ;
#60932=ORIENTED_EDGE('',*,*,#43442,.T.) ;
#60933=ORIENTED_EDGE('',*,*,#42855,.F.) ;
#60934=ORIENTED_EDGE('',*,*,#43447,.F.) ;
#60935=ORIENTED_EDGE('',*,*,#43269,.F.) ;
#60936=ORIENTED_EDGE('',*,*,#43446,.T.) ;
#60937=ORIENTED_EDGE('',*,*,#43445,.T.) ;
#60938=ORIENTED_EDGE('',*,*,#43448,.F.) ;
#60939=ORIENTED_EDGE('',*,*,#43449,.F.) ;
#60940=ORIENTED_EDGE('',*,*,#43447,.T.) ;
#60941=ORIENTED_EDGE('',*,*,#43450,.F.) ;
#60942=ORIENTED_EDGE('',*,*,#43448,.T.) ;
#60943=ORIENTED_EDGE('',*,*,#43273,.F.) ;
#60944=ORIENTED_EDGE('',*,*,#43451,.F.) ;
#60945=ORIENTED_EDGE('',*,*,#42857,.F.) ;
#60946=ORIENTED_EDGE('',*,*,#43450,.T.) ;
#60947=ORIENTED_EDGE('',*,*,#42854,.F.) ;
#60948=ORIENTED_EDGE('',*,*,#43452,.F.) ;
#60949=ORIENTED_EDGE('',*,*,#42850,.F.) ;
#60950=ORIENTED_EDGE('',*,*,#42853,.F.) ;
#60951=ORIENTED_EDGE('',*,*,#43453,.T.) ;
#60952=ORIENTED_EDGE('',*,*,#43266,.F.) ;
#60953=ORIENTED_EDGE('',*,*,#43449,.T.) ;
#60954=ORIENTED_EDGE('',*,*,#43452,.T.) ;
#60955=ORIENTED_EDGE('',*,*,#43451,.T.) ;
#60956=ORIENTED_EDGE('',*,*,#43454,.F.) ;
#60957=ORIENTED_EDGE('',*,*,#42848,.F.) ;
#60958=ORIENTED_EDGE('',*,*,#43455,.T.) ;
#60959=ORIENTED_EDGE('',*,*,#42852,.F.) ;
#60960=ORIENTED_EDGE('',*,*,#43456,.T.) ;
#60961=ORIENTED_EDGE('',*,*,#43272,.F.) ;
#60962=ORIENTED_EDGE('',*,*,#43457,.T.) ;
#60963=ORIENTED_EDGE('',*,*,#42851,.F.) ;
#60964=ORIENTED_EDGE('',*,*,#43454,.T.) ;
#60965=ORIENTED_EDGE('',*,*,#43188,.F.) ;
#60966=ORIENTED_EDGE('',*,*,#43458,.T.) ;
#60967=ORIENTED_EDGE('',*,*,#42879,.F.) ;
#60968=ORIENTED_EDGE('',*,*,#43459,.F.) ;
#60969=ORIENTED_EDGE('',*,*,#42876,.F.) ;
#60970=ORIENTED_EDGE('',*,*,#43460,.T.) ;
#60971=ORIENTED_EDGE('',*,*,#42880,.F.) ;
#60972=ORIENTED_EDGE('',*,*,#43461,.T.) ;
#60973=ORIENTED_EDGE('',*,*,#43462,.F.) ;
#60974=ORIENTED_EDGE('',*,*,#43459,.T.) ;
#60975=ORIENTED_EDGE('',*,*,#43463,.F.) ;
#60976=ORIENTED_EDGE('',*,*,#42877,.F.) ;
#60977=ORIENTED_EDGE('',*,*,#43464,.T.) ;
#60978=ORIENTED_EDGE('',*,*,#43190,.F.) ;
#60979=ORIENTED_EDGE('',*,*,#43465,.F.) ;
#60980=ORIENTED_EDGE('',*,*,#43463,.T.) ;
#60981=ORIENTED_EDGE('',*,*,#42878,.F.) ;
#60982=ORIENTED_EDGE('',*,*,#43466,.F.) ;
#60983=ORIENTED_EDGE('',*,*,#42872,.F.) ;
#60984=ORIENTED_EDGE('',*,*,#43462,.T.) ;
#60985=ORIENTED_EDGE('',*,*,#42875,.F.) ;
#60986=ORIENTED_EDGE('',*,*,#43467,.F.) ;
#60987=ORIENTED_EDGE('',*,*,#43189,.F.) ;
#60988=ORIENTED_EDGE('',*,*,#43466,.T.) ;
#60989=ORIENTED_EDGE('',*,*,#43465,.T.) ;
#60990=ORIENTED_EDGE('',*,*,#43468,.F.) ;
#60991=ORIENTED_EDGE('',*,*,#43469,.F.) ;
#60992=ORIENTED_EDGE('',*,*,#43467,.T.) ;
#60993=ORIENTED_EDGE('',*,*,#43470,.F.) ;
#60994=ORIENTED_EDGE('',*,*,#43468,.T.) ;
#60995=ORIENTED_EDGE('',*,*,#43193,.F.) ;
#60996=ORIENTED_EDGE('',*,*,#43471,.F.) ;
#60997=ORIENTED_EDGE('',*,*,#42873,.F.) ;
#60998=ORIENTED_EDGE('',*,*,#43470,.T.) ;
#60999=ORIENTED_EDGE('',*,*,#42874,.F.) ;
#61000=ORIENTED_EDGE('',*,*,#43472,.F.) ;
#61001=ORIENTED_EDGE('',*,*,#42868,.F.) ;
#61002=ORIENTED_EDGE('',*,*,#42871,.F.) ;
#61003=ORIENTED_EDGE('',*,*,#43473,.T.) ;
#61004=ORIENTED_EDGE('',*,*,#43186,.F.) ;
#61005=ORIENTED_EDGE('',*,*,#43469,.T.) ;
#61006=ORIENTED_EDGE('',*,*,#43472,.T.) ;
#61007=ORIENTED_EDGE('',*,*,#43471,.T.) ;
#61008=ORIENTED_EDGE('',*,*,#43474,.F.) ;
#61009=ORIENTED_EDGE('',*,*,#42866,.F.) ;
#61010=ORIENTED_EDGE('',*,*,#43475,.T.) ;
#61011=ORIENTED_EDGE('',*,*,#42870,.F.) ;
#61012=ORIENTED_EDGE('',*,*,#43476,.T.) ;
#61013=ORIENTED_EDGE('',*,*,#43192,.F.) ;
#61014=ORIENTED_EDGE('',*,*,#43477,.T.) ;
#61015=ORIENTED_EDGE('',*,*,#42869,.F.) ;
#61016=ORIENTED_EDGE('',*,*,#43474,.T.) ;
#61017=ORIENTED_EDGE('',*,*,#43260,.F.) ;
#61018=ORIENTED_EDGE('',*,*,#43478,.T.) ;
#61019=ORIENTED_EDGE('',*,*,#42901,.F.) ;
#61020=ORIENTED_EDGE('',*,*,#43479,.F.) ;
#61021=ORIENTED_EDGE('',*,*,#42898,.F.) ;
#61022=ORIENTED_EDGE('',*,*,#43480,.T.) ;
#61023=ORIENTED_EDGE('',*,*,#42902,.F.) ;
#61024=ORIENTED_EDGE('',*,*,#43481,.T.) ;
#61025=ORIENTED_EDGE('',*,*,#43482,.F.) ;
#61026=ORIENTED_EDGE('',*,*,#43479,.T.) ;
#61027=ORIENTED_EDGE('',*,*,#43483,.F.) ;
#61028=ORIENTED_EDGE('',*,*,#42899,.F.) ;
#61029=ORIENTED_EDGE('',*,*,#43484,.T.) ;
#61030=ORIENTED_EDGE('',*,*,#43262,.F.) ;
#61031=ORIENTED_EDGE('',*,*,#43485,.F.) ;
#61032=ORIENTED_EDGE('',*,*,#43483,.T.) ;
#61033=ORIENTED_EDGE('',*,*,#42900,.F.) ;
#61034=ORIENTED_EDGE('',*,*,#43486,.F.) ;
#61035=ORIENTED_EDGE('',*,*,#42914,.F.) ;
#61036=ORIENTED_EDGE('',*,*,#43482,.T.) ;
#61037=ORIENTED_EDGE('',*,*,#42913,.F.) ;
#61038=ORIENTED_EDGE('',*,*,#43487,.F.) ;
#61039=ORIENTED_EDGE('',*,*,#43261,.F.) ;
#61040=ORIENTED_EDGE('',*,*,#43486,.T.) ;
#61041=ORIENTED_EDGE('',*,*,#43485,.T.) ;
#61042=ORIENTED_EDGE('',*,*,#43488,.F.) ;
#61043=ORIENTED_EDGE('',*,*,#43489,.F.) ;
#61044=ORIENTED_EDGE('',*,*,#43487,.T.) ;
#61045=ORIENTED_EDGE('',*,*,#43490,.F.) ;
#61046=ORIENTED_EDGE('',*,*,#43488,.T.) ;
#61047=ORIENTED_EDGE('',*,*,#43265,.F.) ;
#61048=ORIENTED_EDGE('',*,*,#43491,.F.) ;
#61049=ORIENTED_EDGE('',*,*,#42915,.F.) ;
#61050=ORIENTED_EDGE('',*,*,#43490,.T.) ;
#61051=ORIENTED_EDGE('',*,*,#42912,.F.) ;
#61052=ORIENTED_EDGE('',*,*,#43492,.F.) ;
#61053=ORIENTED_EDGE('',*,*,#42908,.F.) ;
#61054=ORIENTED_EDGE('',*,*,#42911,.F.) ;
#61055=ORIENTED_EDGE('',*,*,#43493,.T.) ;
#61056=ORIENTED_EDGE('',*,*,#43258,.F.) ;
#61057=ORIENTED_EDGE('',*,*,#43489,.T.) ;
#61058=ORIENTED_EDGE('',*,*,#43492,.T.) ;
#61059=ORIENTED_EDGE('',*,*,#43491,.T.) ;
#61060=ORIENTED_EDGE('',*,*,#43494,.F.) ;
#61061=ORIENTED_EDGE('',*,*,#42906,.F.) ;
#61062=ORIENTED_EDGE('',*,*,#43495,.T.) ;
#61063=ORIENTED_EDGE('',*,*,#42910,.F.) ;
#61064=ORIENTED_EDGE('',*,*,#43496,.T.) ;
#61065=ORIENTED_EDGE('',*,*,#43264,.F.) ;
#61066=ORIENTED_EDGE('',*,*,#43497,.T.) ;
#61067=ORIENTED_EDGE('',*,*,#42909,.F.) ;
#61068=ORIENTED_EDGE('',*,*,#43494,.T.) ;
#61069=ORIENTED_EDGE('',*,*,#43180,.F.) ;
#61070=ORIENTED_EDGE('',*,*,#43498,.T.) ;
#61071=ORIENTED_EDGE('',*,*,#42937,.F.) ;
#61072=ORIENTED_EDGE('',*,*,#43499,.F.) ;
#61073=ORIENTED_EDGE('',*,*,#42934,.F.) ;
#61074=ORIENTED_EDGE('',*,*,#43500,.T.) ;
#61075=ORIENTED_EDGE('',*,*,#42938,.F.) ;
#61076=ORIENTED_EDGE('',*,*,#43501,.T.) ;
#61077=ORIENTED_EDGE('',*,*,#43502,.F.) ;
#61078=ORIENTED_EDGE('',*,*,#43499,.T.) ;
#61079=ORIENTED_EDGE('',*,*,#43503,.F.) ;
#61080=ORIENTED_EDGE('',*,*,#42935,.F.) ;
#61081=ORIENTED_EDGE('',*,*,#43504,.T.) ;
#61082=ORIENTED_EDGE('',*,*,#43182,.F.) ;
#61083=ORIENTED_EDGE('',*,*,#43505,.F.) ;
#61084=ORIENTED_EDGE('',*,*,#43503,.T.) ;
#61085=ORIENTED_EDGE('',*,*,#42936,.F.) ;
#61086=ORIENTED_EDGE('',*,*,#43506,.F.) ;
#61087=ORIENTED_EDGE('',*,*,#42930,.F.) ;
#61088=ORIENTED_EDGE('',*,*,#43502,.T.) ;
#61089=ORIENTED_EDGE('',*,*,#42933,.F.) ;
#61090=ORIENTED_EDGE('',*,*,#43507,.F.) ;
#61091=ORIENTED_EDGE('',*,*,#43181,.F.) ;
#61092=ORIENTED_EDGE('',*,*,#43506,.T.) ;
#61093=ORIENTED_EDGE('',*,*,#43505,.T.) ;
#61094=ORIENTED_EDGE('',*,*,#43508,.F.) ;
#61095=ORIENTED_EDGE('',*,*,#43509,.F.) ;
#61096=ORIENTED_EDGE('',*,*,#43507,.T.) ;
#61097=ORIENTED_EDGE('',*,*,#43510,.F.) ;
#61098=ORIENTED_EDGE('',*,*,#43508,.T.) ;
#61099=ORIENTED_EDGE('',*,*,#43185,.F.) ;
#61100=ORIENTED_EDGE('',*,*,#43511,.F.) ;
#61101=ORIENTED_EDGE('',*,*,#42931,.F.) ;
#61102=ORIENTED_EDGE('',*,*,#43510,.T.) ;
#61103=ORIENTED_EDGE('',*,*,#42932,.F.) ;
#61104=ORIENTED_EDGE('',*,*,#43512,.F.) ;
#61105=ORIENTED_EDGE('',*,*,#42926,.F.) ;
#61106=ORIENTED_EDGE('',*,*,#42929,.F.) ;
#61107=ORIENTED_EDGE('',*,*,#43513,.T.) ;
#61108=ORIENTED_EDGE('',*,*,#43178,.F.) ;
#61109=ORIENTED_EDGE('',*,*,#43509,.T.) ;
#61110=ORIENTED_EDGE('',*,*,#43512,.T.) ;
#61111=ORIENTED_EDGE('',*,*,#43511,.T.) ;
#61112=ORIENTED_EDGE('',*,*,#43514,.F.) ;
#61113=ORIENTED_EDGE('',*,*,#42924,.F.) ;
#61114=ORIENTED_EDGE('',*,*,#43515,.T.) ;
#61115=ORIENTED_EDGE('',*,*,#42928,.F.) ;
#61116=ORIENTED_EDGE('',*,*,#43516,.T.) ;
#61117=ORIENTED_EDGE('',*,*,#43184,.F.) ;
#61118=ORIENTED_EDGE('',*,*,#43517,.T.) ;
#61119=ORIENTED_EDGE('',*,*,#42927,.F.) ;
#61120=ORIENTED_EDGE('',*,*,#43514,.T.) ;
#61121=ORIENTED_EDGE('',*,*,#43252,.F.) ;
#61122=ORIENTED_EDGE('',*,*,#43518,.T.) ;
#61123=ORIENTED_EDGE('',*,*,#42959,.F.) ;
#61124=ORIENTED_EDGE('',*,*,#43519,.F.) ;
#61125=ORIENTED_EDGE('',*,*,#42956,.F.) ;
#61126=ORIENTED_EDGE('',*,*,#43520,.T.) ;
#61127=ORIENTED_EDGE('',*,*,#42960,.F.) ;
#61128=ORIENTED_EDGE('',*,*,#43521,.T.) ;
#61129=ORIENTED_EDGE('',*,*,#43522,.F.) ;
#61130=ORIENTED_EDGE('',*,*,#43519,.T.) ;
#61131=ORIENTED_EDGE('',*,*,#43523,.F.) ;
#61132=ORIENTED_EDGE('',*,*,#42957,.F.) ;
#61133=ORIENTED_EDGE('',*,*,#43524,.T.) ;
#61134=ORIENTED_EDGE('',*,*,#43254,.F.) ;
#61135=ORIENTED_EDGE('',*,*,#43525,.F.) ;
#61136=ORIENTED_EDGE('',*,*,#43523,.T.) ;
#61137=ORIENTED_EDGE('',*,*,#42958,.F.) ;
#61138=ORIENTED_EDGE('',*,*,#43526,.F.) ;
#61139=ORIENTED_EDGE('',*,*,#42972,.F.) ;
#61140=ORIENTED_EDGE('',*,*,#43522,.T.) ;
#61141=ORIENTED_EDGE('',*,*,#42971,.F.) ;
#61142=ORIENTED_EDGE('',*,*,#43527,.F.) ;
#61143=ORIENTED_EDGE('',*,*,#43253,.F.) ;
#61144=ORIENTED_EDGE('',*,*,#43526,.T.) ;
#61145=ORIENTED_EDGE('',*,*,#43525,.T.) ;
#61146=ORIENTED_EDGE('',*,*,#43528,.F.) ;
#61147=ORIENTED_EDGE('',*,*,#43529,.F.) ;
#61148=ORIENTED_EDGE('',*,*,#43527,.T.) ;
#61149=ORIENTED_EDGE('',*,*,#43530,.F.) ;
#61150=ORIENTED_EDGE('',*,*,#43528,.T.) ;
#61151=ORIENTED_EDGE('',*,*,#43257,.F.) ;
#61152=ORIENTED_EDGE('',*,*,#43531,.F.) ;
#61153=ORIENTED_EDGE('',*,*,#42973,.F.) ;
#61154=ORIENTED_EDGE('',*,*,#43530,.T.) ;
#61155=ORIENTED_EDGE('',*,*,#42970,.F.) ;
#61156=ORIENTED_EDGE('',*,*,#43532,.F.) ;
#61157=ORIENTED_EDGE('',*,*,#42966,.F.) ;
#61158=ORIENTED_EDGE('',*,*,#42969,.F.) ;
#61159=ORIENTED_EDGE('',*,*,#43533,.T.) ;
#61160=ORIENTED_EDGE('',*,*,#43250,.F.) ;
#61161=ORIENTED_EDGE('',*,*,#43529,.T.) ;
#61162=ORIENTED_EDGE('',*,*,#43532,.T.) ;
#61163=ORIENTED_EDGE('',*,*,#43531,.T.) ;
#61164=ORIENTED_EDGE('',*,*,#43534,.F.) ;
#61165=ORIENTED_EDGE('',*,*,#42964,.F.) ;
#61166=ORIENTED_EDGE('',*,*,#43535,.T.) ;
#61167=ORIENTED_EDGE('',*,*,#42968,.F.) ;
#61168=ORIENTED_EDGE('',*,*,#43536,.T.) ;
#61169=ORIENTED_EDGE('',*,*,#43256,.F.) ;
#61170=ORIENTED_EDGE('',*,*,#43537,.T.) ;
#61171=ORIENTED_EDGE('',*,*,#42967,.F.) ;
#61172=ORIENTED_EDGE('',*,*,#43534,.T.) ;
#61173=ORIENTED_EDGE('',*,*,#43172,.F.) ;
#61174=ORIENTED_EDGE('',*,*,#43538,.T.) ;
#61175=ORIENTED_EDGE('',*,*,#42995,.F.) ;
#61176=ORIENTED_EDGE('',*,*,#43539,.F.) ;
#61177=ORIENTED_EDGE('',*,*,#42992,.F.) ;
#61178=ORIENTED_EDGE('',*,*,#43540,.T.) ;
#61179=ORIENTED_EDGE('',*,*,#42996,.F.) ;
#61180=ORIENTED_EDGE('',*,*,#43541,.T.) ;
#61181=ORIENTED_EDGE('',*,*,#43542,.F.) ;
#61182=ORIENTED_EDGE('',*,*,#43539,.T.) ;
#61183=ORIENTED_EDGE('',*,*,#43543,.F.) ;
#61184=ORIENTED_EDGE('',*,*,#42993,.F.) ;
#61185=ORIENTED_EDGE('',*,*,#43544,.T.) ;
#61186=ORIENTED_EDGE('',*,*,#43174,.F.) ;
#61187=ORIENTED_EDGE('',*,*,#43545,.F.) ;
#61188=ORIENTED_EDGE('',*,*,#43543,.T.) ;
#61189=ORIENTED_EDGE('',*,*,#42994,.F.) ;
#61190=ORIENTED_EDGE('',*,*,#43546,.F.) ;
#61191=ORIENTED_EDGE('',*,*,#42988,.F.) ;
#61192=ORIENTED_EDGE('',*,*,#43542,.T.) ;
#61193=ORIENTED_EDGE('',*,*,#42991,.F.) ;
#61194=ORIENTED_EDGE('',*,*,#43547,.F.) ;
#61195=ORIENTED_EDGE('',*,*,#43173,.F.) ;
#61196=ORIENTED_EDGE('',*,*,#43546,.T.) ;
#61197=ORIENTED_EDGE('',*,*,#43545,.T.) ;
#61198=ORIENTED_EDGE('',*,*,#43548,.F.) ;
#61199=ORIENTED_EDGE('',*,*,#43549,.F.) ;
#61200=ORIENTED_EDGE('',*,*,#43547,.T.) ;
#61201=ORIENTED_EDGE('',*,*,#43550,.F.) ;
#61202=ORIENTED_EDGE('',*,*,#43548,.T.) ;
#61203=ORIENTED_EDGE('',*,*,#43177,.F.) ;
#61204=ORIENTED_EDGE('',*,*,#43551,.F.) ;
#61205=ORIENTED_EDGE('',*,*,#42989,.F.) ;
#61206=ORIENTED_EDGE('',*,*,#43550,.T.) ;
#61207=ORIENTED_EDGE('',*,*,#42990,.F.) ;
#61208=ORIENTED_EDGE('',*,*,#43552,.F.) ;
#61209=ORIENTED_EDGE('',*,*,#42984,.F.) ;
#61210=ORIENTED_EDGE('',*,*,#42987,.F.) ;
#61211=ORIENTED_EDGE('',*,*,#43553,.T.) ;
#61212=ORIENTED_EDGE('',*,*,#43170,.F.) ;
#61213=ORIENTED_EDGE('',*,*,#43549,.T.) ;
#61214=ORIENTED_EDGE('',*,*,#43552,.T.) ;
#61215=ORIENTED_EDGE('',*,*,#43551,.T.) ;
#61216=ORIENTED_EDGE('',*,*,#43554,.F.) ;
#61217=ORIENTED_EDGE('',*,*,#42982,.F.) ;
#61218=ORIENTED_EDGE('',*,*,#43555,.T.) ;
#61219=ORIENTED_EDGE('',*,*,#42986,.F.) ;
#61220=ORIENTED_EDGE('',*,*,#43556,.T.) ;
#61221=ORIENTED_EDGE('',*,*,#43176,.F.) ;
#61222=ORIENTED_EDGE('',*,*,#43557,.T.) ;
#61223=ORIENTED_EDGE('',*,*,#42985,.F.) ;
#61224=ORIENTED_EDGE('',*,*,#43554,.T.) ;
#61225=ORIENTED_EDGE('',*,*,#43244,.F.) ;
#61226=ORIENTED_EDGE('',*,*,#43558,.T.) ;
#61227=ORIENTED_EDGE('',*,*,#43017,.F.) ;
#61228=ORIENTED_EDGE('',*,*,#43559,.F.) ;
#61229=ORIENTED_EDGE('',*,*,#43014,.F.) ;
#61230=ORIENTED_EDGE('',*,*,#43560,.T.) ;
#61231=ORIENTED_EDGE('',*,*,#43018,.F.) ;
#61232=ORIENTED_EDGE('',*,*,#43561,.T.) ;
#61233=ORIENTED_EDGE('',*,*,#43562,.F.) ;
#61234=ORIENTED_EDGE('',*,*,#43559,.T.) ;
#61235=ORIENTED_EDGE('',*,*,#43563,.F.) ;
#61236=ORIENTED_EDGE('',*,*,#43015,.F.) ;
#61237=ORIENTED_EDGE('',*,*,#43564,.T.) ;
#61238=ORIENTED_EDGE('',*,*,#43246,.F.) ;
#61239=ORIENTED_EDGE('',*,*,#43565,.F.) ;
#61240=ORIENTED_EDGE('',*,*,#43563,.T.) ;
#61241=ORIENTED_EDGE('',*,*,#43016,.F.) ;
#61242=ORIENTED_EDGE('',*,*,#43566,.F.) ;
#61243=ORIENTED_EDGE('',*,*,#43030,.F.) ;
#61244=ORIENTED_EDGE('',*,*,#43562,.T.) ;
#61245=ORIENTED_EDGE('',*,*,#43029,.F.) ;
#61246=ORIENTED_EDGE('',*,*,#43567,.F.) ;
#61247=ORIENTED_EDGE('',*,*,#43245,.F.) ;
#61248=ORIENTED_EDGE('',*,*,#43566,.T.) ;
#61249=ORIENTED_EDGE('',*,*,#43565,.T.) ;
#61250=ORIENTED_EDGE('',*,*,#43568,.F.) ;
#61251=ORIENTED_EDGE('',*,*,#43569,.F.) ;
#61252=ORIENTED_EDGE('',*,*,#43567,.T.) ;
#61253=ORIENTED_EDGE('',*,*,#43570,.F.) ;
#61254=ORIENTED_EDGE('',*,*,#43568,.T.) ;
#61255=ORIENTED_EDGE('',*,*,#43249,.F.) ;
#61256=ORIENTED_EDGE('',*,*,#43571,.F.) ;
#61257=ORIENTED_EDGE('',*,*,#43031,.F.) ;
#61258=ORIENTED_EDGE('',*,*,#43570,.T.) ;
#61259=ORIENTED_EDGE('',*,*,#43028,.F.) ;
#61260=ORIENTED_EDGE('',*,*,#43572,.F.) ;
#61261=ORIENTED_EDGE('',*,*,#43024,.F.) ;
#61262=ORIENTED_EDGE('',*,*,#43027,.F.) ;
#61263=ORIENTED_EDGE('',*,*,#43573,.T.) ;
#61264=ORIENTED_EDGE('',*,*,#43242,.F.) ;
#61265=ORIENTED_EDGE('',*,*,#43569,.T.) ;
#61266=ORIENTED_EDGE('',*,*,#43572,.T.) ;
#61267=ORIENTED_EDGE('',*,*,#43571,.T.) ;
#61268=ORIENTED_EDGE('',*,*,#43574,.F.) ;
#61269=ORIENTED_EDGE('',*,*,#43022,.F.) ;
#61270=ORIENTED_EDGE('',*,*,#43575,.T.) ;
#61271=ORIENTED_EDGE('',*,*,#43026,.F.) ;
#61272=ORIENTED_EDGE('',*,*,#43576,.T.) ;
#61273=ORIENTED_EDGE('',*,*,#43248,.F.) ;
#61274=ORIENTED_EDGE('',*,*,#43577,.T.) ;
#61275=ORIENTED_EDGE('',*,*,#43025,.F.) ;
#61276=ORIENTED_EDGE('',*,*,#43574,.T.) ;
#61277=ORIENTED_EDGE('',*,*,#43164,.F.) ;
#61278=ORIENTED_EDGE('',*,*,#43578,.T.) ;
#61279=ORIENTED_EDGE('',*,*,#43053,.F.) ;
#61280=ORIENTED_EDGE('',*,*,#43579,.F.) ;
#61281=ORIENTED_EDGE('',*,*,#43050,.F.) ;
#61282=ORIENTED_EDGE('',*,*,#43580,.T.) ;
#61283=ORIENTED_EDGE('',*,*,#43054,.F.) ;
#61284=ORIENTED_EDGE('',*,*,#43581,.T.) ;
#61285=ORIENTED_EDGE('',*,*,#43582,.F.) ;
#61286=ORIENTED_EDGE('',*,*,#43579,.T.) ;
#61287=ORIENTED_EDGE('',*,*,#43583,.F.) ;
#61288=ORIENTED_EDGE('',*,*,#43051,.F.) ;
#61289=ORIENTED_EDGE('',*,*,#43584,.T.) ;
#61290=ORIENTED_EDGE('',*,*,#43166,.F.) ;
#61291=ORIENTED_EDGE('',*,*,#43585,.F.) ;
#61292=ORIENTED_EDGE('',*,*,#43583,.T.) ;
#61293=ORIENTED_EDGE('',*,*,#43052,.F.) ;
#61294=ORIENTED_EDGE('',*,*,#43586,.F.) ;
#61295=ORIENTED_EDGE('',*,*,#43046,.F.) ;
#61296=ORIENTED_EDGE('',*,*,#43582,.T.) ;
#61297=ORIENTED_EDGE('',*,*,#43049,.F.) ;
#61298=ORIENTED_EDGE('',*,*,#43587,.F.) ;
#61299=ORIENTED_EDGE('',*,*,#43165,.F.) ;
#61300=ORIENTED_EDGE('',*,*,#43586,.T.) ;
#61301=ORIENTED_EDGE('',*,*,#43585,.T.) ;
#61302=ORIENTED_EDGE('',*,*,#43588,.F.) ;
#61303=ORIENTED_EDGE('',*,*,#43589,.F.) ;
#61304=ORIENTED_EDGE('',*,*,#43587,.T.) ;
#61305=ORIENTED_EDGE('',*,*,#43590,.F.) ;
#61306=ORIENTED_EDGE('',*,*,#43588,.T.) ;
#61307=ORIENTED_EDGE('',*,*,#43169,.F.) ;
#61308=ORIENTED_EDGE('',*,*,#43591,.F.) ;
#61309=ORIENTED_EDGE('',*,*,#43047,.F.) ;
#61310=ORIENTED_EDGE('',*,*,#43590,.T.) ;
#61311=ORIENTED_EDGE('',*,*,#43048,.F.) ;
#61312=ORIENTED_EDGE('',*,*,#43592,.F.) ;
#61313=ORIENTED_EDGE('',*,*,#43042,.F.) ;
#61314=ORIENTED_EDGE('',*,*,#43045,.F.) ;
#61315=ORIENTED_EDGE('',*,*,#43593,.T.) ;
#61316=ORIENTED_EDGE('',*,*,#43162,.F.) ;
#61317=ORIENTED_EDGE('',*,*,#43589,.T.) ;
#61318=ORIENTED_EDGE('',*,*,#43592,.T.) ;
#61319=ORIENTED_EDGE('',*,*,#43591,.T.) ;
#61320=ORIENTED_EDGE('',*,*,#43594,.F.) ;
#61321=ORIENTED_EDGE('',*,*,#43040,.F.) ;
#61322=ORIENTED_EDGE('',*,*,#43595,.T.) ;
#61323=ORIENTED_EDGE('',*,*,#43044,.F.) ;
#61324=ORIENTED_EDGE('',*,*,#43596,.T.) ;
#61325=ORIENTED_EDGE('',*,*,#43168,.F.) ;
#61326=ORIENTED_EDGE('',*,*,#43597,.T.) ;
#61327=ORIENTED_EDGE('',*,*,#43043,.F.) ;
#61328=ORIENTED_EDGE('',*,*,#43594,.T.) ;
#61329=ORIENTED_EDGE('',*,*,#43236,.F.) ;
#61330=ORIENTED_EDGE('',*,*,#43598,.T.) ;
#61331=ORIENTED_EDGE('',*,*,#43075,.F.) ;
#61332=ORIENTED_EDGE('',*,*,#43599,.F.) ;
#61333=ORIENTED_EDGE('',*,*,#43072,.F.) ;
#61334=ORIENTED_EDGE('',*,*,#43600,.T.) ;
#61335=ORIENTED_EDGE('',*,*,#43076,.F.) ;
#61336=ORIENTED_EDGE('',*,*,#43601,.T.) ;
#61337=ORIENTED_EDGE('',*,*,#43602,.F.) ;
#61338=ORIENTED_EDGE('',*,*,#43599,.T.) ;
#61339=ORIENTED_EDGE('',*,*,#43603,.F.) ;
#61340=ORIENTED_EDGE('',*,*,#43073,.F.) ;
#61341=ORIENTED_EDGE('',*,*,#43604,.T.) ;
#61342=ORIENTED_EDGE('',*,*,#43238,.F.) ;
#61343=ORIENTED_EDGE('',*,*,#43605,.F.) ;
#61344=ORIENTED_EDGE('',*,*,#43603,.T.) ;
#61345=ORIENTED_EDGE('',*,*,#43074,.F.) ;
#61346=ORIENTED_EDGE('',*,*,#43606,.F.) ;
#61347=ORIENTED_EDGE('',*,*,#43088,.F.) ;
#61348=ORIENTED_EDGE('',*,*,#43602,.T.) ;
#61349=ORIENTED_EDGE('',*,*,#43087,.F.) ;
#61350=ORIENTED_EDGE('',*,*,#43607,.F.) ;
#61351=ORIENTED_EDGE('',*,*,#43237,.F.) ;
#61352=ORIENTED_EDGE('',*,*,#43606,.T.) ;
#61353=ORIENTED_EDGE('',*,*,#43605,.T.) ;
#61354=ORIENTED_EDGE('',*,*,#43608,.F.) ;
#61355=ORIENTED_EDGE('',*,*,#43609,.F.) ;
#61356=ORIENTED_EDGE('',*,*,#43607,.T.) ;
#61357=ORIENTED_EDGE('',*,*,#43610,.F.) ;
#61358=ORIENTED_EDGE('',*,*,#43608,.T.) ;
#61359=ORIENTED_EDGE('',*,*,#43241,.F.) ;
#61360=ORIENTED_EDGE('',*,*,#43611,.F.) ;
#61361=ORIENTED_EDGE('',*,*,#43089,.F.) ;
#61362=ORIENTED_EDGE('',*,*,#43610,.T.) ;
#61363=ORIENTED_EDGE('',*,*,#43086,.F.) ;
#61364=ORIENTED_EDGE('',*,*,#43612,.F.) ;
#61365=ORIENTED_EDGE('',*,*,#43082,.F.) ;
#61366=ORIENTED_EDGE('',*,*,#43085,.F.) ;
#61367=ORIENTED_EDGE('',*,*,#43613,.T.) ;
#61368=ORIENTED_EDGE('',*,*,#43234,.F.) ;
#61369=ORIENTED_EDGE('',*,*,#43609,.T.) ;
#61370=ORIENTED_EDGE('',*,*,#43612,.T.) ;
#61371=ORIENTED_EDGE('',*,*,#43611,.T.) ;
#61372=ORIENTED_EDGE('',*,*,#43614,.F.) ;
#61373=ORIENTED_EDGE('',*,*,#43080,.F.) ;
#61374=ORIENTED_EDGE('',*,*,#43615,.T.) ;
#61375=ORIENTED_EDGE('',*,*,#43084,.F.) ;
#61376=ORIENTED_EDGE('',*,*,#43616,.T.) ;
#61377=ORIENTED_EDGE('',*,*,#43240,.F.) ;
#61378=ORIENTED_EDGE('',*,*,#43617,.T.) ;
#61379=ORIENTED_EDGE('',*,*,#43083,.F.) ;
#61380=ORIENTED_EDGE('',*,*,#43614,.T.) ;
#61381=ORIENTED_EDGE('',*,*,#43156,.F.) ;
#61382=ORIENTED_EDGE('',*,*,#43618,.T.) ;
#61383=ORIENTED_EDGE('',*,*,#43111,.F.) ;
#61384=ORIENTED_EDGE('',*,*,#43619,.F.) ;
#61385=ORIENTED_EDGE('',*,*,#43108,.F.) ;
#61386=ORIENTED_EDGE('',*,*,#43620,.T.) ;
#61387=ORIENTED_EDGE('',*,*,#43112,.F.) ;
#61388=ORIENTED_EDGE('',*,*,#43621,.T.) ;
#61389=ORIENTED_EDGE('',*,*,#43622,.F.) ;
#61390=ORIENTED_EDGE('',*,*,#43619,.T.) ;
#61391=ORIENTED_EDGE('',*,*,#43623,.F.) ;
#61392=ORIENTED_EDGE('',*,*,#43109,.F.) ;
#61393=ORIENTED_EDGE('',*,*,#43624,.T.) ;
#61394=ORIENTED_EDGE('',*,*,#43158,.F.) ;
#61395=ORIENTED_EDGE('',*,*,#43625,.F.) ;
#61396=ORIENTED_EDGE('',*,*,#43623,.T.) ;
#61397=ORIENTED_EDGE('',*,*,#43110,.F.) ;
#61398=ORIENTED_EDGE('',*,*,#43626,.F.) ;
#61399=ORIENTED_EDGE('',*,*,#43104,.F.) ;
#61400=ORIENTED_EDGE('',*,*,#43622,.T.) ;
#61401=ORIENTED_EDGE('',*,*,#43107,.F.) ;
#61402=ORIENTED_EDGE('',*,*,#43627,.F.) ;
#61403=ORIENTED_EDGE('',*,*,#43157,.F.) ;
#61404=ORIENTED_EDGE('',*,*,#43626,.T.) ;
#61405=ORIENTED_EDGE('',*,*,#43625,.T.) ;
#61406=ORIENTED_EDGE('',*,*,#43628,.F.) ;
#61407=ORIENTED_EDGE('',*,*,#43629,.F.) ;
#61408=ORIENTED_EDGE('',*,*,#43627,.T.) ;
#61409=ORIENTED_EDGE('',*,*,#43630,.F.) ;
#61410=ORIENTED_EDGE('',*,*,#43628,.T.) ;
#61411=ORIENTED_EDGE('',*,*,#43161,.F.) ;
#61412=ORIENTED_EDGE('',*,*,#43631,.F.) ;
#61413=ORIENTED_EDGE('',*,*,#43105,.F.) ;
#61414=ORIENTED_EDGE('',*,*,#43630,.T.) ;
#61415=ORIENTED_EDGE('',*,*,#43106,.F.) ;
#61416=ORIENTED_EDGE('',*,*,#43632,.F.) ;
#61417=ORIENTED_EDGE('',*,*,#43100,.F.) ;
#61418=ORIENTED_EDGE('',*,*,#43103,.F.) ;
#61419=ORIENTED_EDGE('',*,*,#43633,.T.) ;
#61420=ORIENTED_EDGE('',*,*,#43154,.F.) ;
#61421=ORIENTED_EDGE('',*,*,#43629,.T.) ;
#61422=ORIENTED_EDGE('',*,*,#43632,.T.) ;
#61423=ORIENTED_EDGE('',*,*,#43631,.T.) ;
#61424=ORIENTED_EDGE('',*,*,#43634,.F.) ;
#61425=ORIENTED_EDGE('',*,*,#43098,.F.) ;
#61426=ORIENTED_EDGE('',*,*,#43635,.T.) ;
#61427=ORIENTED_EDGE('',*,*,#43102,.F.) ;
#61428=ORIENTED_EDGE('',*,*,#43636,.T.) ;
#61429=ORIENTED_EDGE('',*,*,#43160,.F.) ;
#61430=ORIENTED_EDGE('',*,*,#43637,.T.) ;
#61431=ORIENTED_EDGE('',*,*,#43101,.F.) ;
#61432=ORIENTED_EDGE('',*,*,#43634,.T.) ;
#61433=ORIENTED_EDGE('',*,*,#43228,.F.) ;
#61434=ORIENTED_EDGE('',*,*,#43638,.T.) ;
#61435=ORIENTED_EDGE('',*,*,#43133,.F.) ;
#61436=ORIENTED_EDGE('',*,*,#43639,.F.) ;
#61437=ORIENTED_EDGE('',*,*,#43130,.F.) ;
#61438=ORIENTED_EDGE('',*,*,#43640,.T.) ;
#61439=ORIENTED_EDGE('',*,*,#43134,.F.) ;
#61440=ORIENTED_EDGE('',*,*,#43641,.T.) ;
#61441=ORIENTED_EDGE('',*,*,#43642,.F.) ;
#61442=ORIENTED_EDGE('',*,*,#43639,.T.) ;
#61443=ORIENTED_EDGE('',*,*,#43643,.F.) ;
#61444=ORIENTED_EDGE('',*,*,#43131,.F.) ;
#61445=ORIENTED_EDGE('',*,*,#43644,.T.) ;
#61446=ORIENTED_EDGE('',*,*,#43230,.F.) ;
#61447=ORIENTED_EDGE('',*,*,#43645,.F.) ;
#61448=ORIENTED_EDGE('',*,*,#43643,.T.) ;
#61449=ORIENTED_EDGE('',*,*,#43132,.F.) ;
#61450=ORIENTED_EDGE('',*,*,#43646,.F.) ;
#61451=ORIENTED_EDGE('',*,*,#43146,.F.) ;
#61452=ORIENTED_EDGE('',*,*,#43642,.T.) ;
#61453=ORIENTED_EDGE('',*,*,#43145,.F.) ;
#61454=ORIENTED_EDGE('',*,*,#43647,.F.) ;
#61455=ORIENTED_EDGE('',*,*,#43229,.F.) ;
#61456=ORIENTED_EDGE('',*,*,#43646,.T.) ;
#61457=ORIENTED_EDGE('',*,*,#43645,.T.) ;
#61458=ORIENTED_EDGE('',*,*,#43648,.F.) ;
#61459=ORIENTED_EDGE('',*,*,#43649,.F.) ;
#61460=ORIENTED_EDGE('',*,*,#43647,.T.) ;
#61461=ORIENTED_EDGE('',*,*,#43650,.F.) ;
#61462=ORIENTED_EDGE('',*,*,#43648,.T.) ;
#61463=ORIENTED_EDGE('',*,*,#43233,.F.) ;
#61464=ORIENTED_EDGE('',*,*,#43651,.F.) ;
#61465=ORIENTED_EDGE('',*,*,#43147,.F.) ;
#61466=ORIENTED_EDGE('',*,*,#43650,.T.) ;
#61467=ORIENTED_EDGE('',*,*,#43144,.F.) ;
#61468=ORIENTED_EDGE('',*,*,#43652,.F.) ;
#61469=ORIENTED_EDGE('',*,*,#43140,.F.) ;
#61470=ORIENTED_EDGE('',*,*,#43143,.F.) ;
#61471=ORIENTED_EDGE('',*,*,#43653,.T.) ;
#61472=ORIENTED_EDGE('',*,*,#43226,.F.) ;
#61473=ORIENTED_EDGE('',*,*,#43649,.T.) ;
#61474=ORIENTED_EDGE('',*,*,#43652,.T.) ;
#61475=ORIENTED_EDGE('',*,*,#43651,.T.) ;
#61476=ORIENTED_EDGE('',*,*,#43654,.F.) ;
#61477=ORIENTED_EDGE('',*,*,#43138,.F.) ;
#61478=ORIENTED_EDGE('',*,*,#43655,.T.) ;
#61479=ORIENTED_EDGE('',*,*,#43142,.F.) ;
#61480=ORIENTED_EDGE('',*,*,#43656,.T.) ;
#61481=ORIENTED_EDGE('',*,*,#43232,.F.) ;
#61482=ORIENTED_EDGE('',*,*,#43657,.T.) ;
#61483=ORIENTED_EDGE('',*,*,#43141,.F.) ;
#61484=ORIENTED_EDGE('',*,*,#43654,.T.) ;
#61485=ORIENTED_EDGE('',*,*,#39429,.F.) ;
#61486=ORIENTED_EDGE('',*,*,#42664,.F.) ;
#61487=ORIENTED_EDGE('',*,*,#43658,.F.) ;
#61488=ORIENTED_EDGE('',*,*,#42659,.F.) ;
#61489=ORIENTED_EDGE('',*,*,#43658,.T.) ;
#61490=ORIENTED_EDGE('',*,*,#42649,.F.) ;
#61491=ORIENTED_EDGE('',*,*,#43659,.F.) ;
#61492=ORIENTED_EDGE('',*,*,#42660,.F.) ;
#61493=ORIENTED_EDGE('',*,*,#43659,.T.) ;
#61494=ORIENTED_EDGE('',*,*,#43300,.F.) ;
#61495=ORIENTED_EDGE('',*,*,#43298,.F.) ;
#61496=ORIENTED_EDGE('',*,*,#43660,.F.) ;
#61497=ORIENTED_EDGE('',*,*,#43660,.T.) ;
#61498=ORIENTED_EDGE('',*,*,#43219,.F.) ;
#61499=ORIENTED_EDGE('',*,*,#43661,.F.) ;
#61500=ORIENTED_EDGE('',*,*,#42661,.F.) ;
#61501=ORIENTED_EDGE('',*,*,#43661,.T.) ;
#61502=ORIENTED_EDGE('',*,*,#43313,.F.) ;
#61503=ORIENTED_EDGE('',*,*,#43315,.F.) ;
#61504=ORIENTED_EDGE('',*,*,#43662,.F.) ;
#61505=ORIENTED_EDGE('',*,*,#43662,.T.) ;
#61506=ORIENTED_EDGE('',*,*,#42633,.F.) ;
#61507=ORIENTED_EDGE('',*,*,#43663,.F.) ;
#61508=ORIENTED_EDGE('',*,*,#42657,.F.) ;
#61509=ORIENTED_EDGE('',*,*,#39276,.F.) ;
#61510=ORIENTED_EDGE('',*,*,#42658,.F.) ;
#61511=ORIENTED_EDGE('',*,*,#43663,.T.) ;
#61512=ORIENTED_EDGE('',*,*,#42662,.F.) ;
#61513=ORIENTED_EDGE('',*,*,#41616,.F.) ;
#61514=ORIENTED_EDGE('',*,*,#41619,.F.) ;
#61515=ORIENTED_EDGE('',*,*,#42663,.F.) ;
#61516=ORIENTED_EDGE('',*,*,#43664,.F.) ;
#61517=ORIENTED_EDGE('',*,*,#42654,.F.) ;
#61518=ORIENTED_EDGE('',*,*,#43664,.T.) ;
#61519=ORIENTED_EDGE('',*,*,#42635,.F.) ;
#61520=ORIENTED_EDGE('',*,*,#43665,.F.) ;
#61521=ORIENTED_EDGE('',*,*,#42655,.F.) ;
#61522=ORIENTED_EDGE('',*,*,#43665,.T.) ;
#61523=ORIENTED_EDGE('',*,*,#43316,.F.) ;
#61524=ORIENTED_EDGE('',*,*,#43317,.F.) ;
#61525=ORIENTED_EDGE('',*,*,#43666,.F.) ;
#61526=ORIENTED_EDGE('',*,*,#43666,.T.) ;
#61527=ORIENTED_EDGE('',*,*,#43223,.F.) ;
#61528=ORIENTED_EDGE('',*,*,#43667,.F.) ;
#61529=ORIENTED_EDGE('',*,*,#42656,.F.) ;
#61530=ORIENTED_EDGE('',*,*,#43667,.T.) ;
#61531=ORIENTED_EDGE('',*,*,#43304,.F.) ;
#61532=ORIENTED_EDGE('',*,*,#43301,.F.) ;
#61533=ORIENTED_EDGE('',*,*,#43668,.F.) ;
#61534=ORIENTED_EDGE('',*,*,#43668,.T.) ;
#61535=ORIENTED_EDGE('',*,*,#42651,.F.) ;
#61536=ORIENTED_EDGE('',*,*,#43669,.F.) ;
#61537=ORIENTED_EDGE('',*,*,#42652,.F.) ;
#61538=ORIENTED_EDGE('',*,*,#43669,.T.) ;
#61539=ORIENTED_EDGE('',*,*,#42665,.F.) ;
#61540=ORIENTED_EDGE('',*,*,#39427,.F.) ;
#61541=ORIENTED_EDGE('',*,*,#42653,.F.) ;
#61542=ORIENTED_EDGE('',*,*,#41537,.F.) ;
#61543=ORIENTED_EDGE('',*,*,#42671,.F.) ;
#61544=ORIENTED_EDGE('',*,*,#43670,.F.) ;
#61545=ORIENTED_EDGE('',*,*,#42687,.F.) ;
#61546=ORIENTED_EDGE('',*,*,#43670,.T.) ;
#61547=ORIENTED_EDGE('',*,*,#43320,.F.) ;
#61548=ORIENTED_EDGE('',*,*,#43318,.F.) ;
#61549=ORIENTED_EDGE('',*,*,#43671,.F.) ;
#61550=ORIENTED_EDGE('',*,*,#43671,.T.) ;
#61551=ORIENTED_EDGE('',*,*,#43291,.F.) ;
#61552=ORIENTED_EDGE('',*,*,#43672,.F.) ;
#61553=ORIENTED_EDGE('',*,*,#42688,.F.) ;
#61554=ORIENTED_EDGE('',*,*,#43672,.T.) ;
#61555=ORIENTED_EDGE('',*,*,#43333,.F.) ;
#61556=ORIENTED_EDGE('',*,*,#43335,.F.) ;
#61557=ORIENTED_EDGE('',*,*,#43673,.F.) ;
#61558=ORIENTED_EDGE('',*,*,#41539,.F.) ;
#61559=ORIENTED_EDGE('',*,*,#42689,.F.) ;
#61560=ORIENTED_EDGE('',*,*,#43673,.T.) ;
#61561=ORIENTED_EDGE('',*,*,#42673,.F.) ;
#61562=ORIENTED_EDGE('',*,*,#43674,.F.) ;
#61563=ORIENTED_EDGE('',*,*,#42672,.F.) ;
#61564=ORIENTED_EDGE('',*,*,#41535,.F.) ;
#61565=ORIENTED_EDGE('',*,*,#42685,.F.) ;
#61566=ORIENTED_EDGE('',*,*,#43321,.F.) ;
#61567=ORIENTED_EDGE('',*,*,#43674,.T.) ;
#61568=ORIENTED_EDGE('',*,*,#43675,.F.) ;
#61569=ORIENTED_EDGE('',*,*,#43324,.F.) ;
#61570=ORIENTED_EDGE('',*,*,#43675,.T.) ;
#61571=ORIENTED_EDGE('',*,*,#42684,.F.) ;
#61572=ORIENTED_EDGE('',*,*,#43676,.F.) ;
#61573=ORIENTED_EDGE('',*,*,#43295,.F.) ;
#61574=ORIENTED_EDGE('',*,*,#41541,.F.) ;
#61575=ORIENTED_EDGE('',*,*,#42675,.F.) ;
#61576=ORIENTED_EDGE('',*,*,#43677,.F.) ;
#61577=ORIENTED_EDGE('',*,*,#42686,.F.) ;
#61578=ORIENTED_EDGE('',*,*,#43337,.F.) ;
#61579=ORIENTED_EDGE('',*,*,#43676,.T.) ;
#61580=ORIENTED_EDGE('',*,*,#43677,.T.) ;
#61581=ORIENTED_EDGE('',*,*,#43336,.F.) ;
#61582=ORIENTED_EDGE('',*,*,#39418,.F.) ;
#61583=ORIENTED_EDGE('',*,*,#42722,.F.) ;
#61584=ORIENTED_EDGE('',*,*,#43678,.F.) ;
#61585=ORIENTED_EDGE('',*,*,#42717,.F.) ;
#61586=ORIENTED_EDGE('',*,*,#43678,.T.) ;
#61587=ORIENTED_EDGE('',*,*,#42707,.F.) ;
#61588=ORIENTED_EDGE('',*,*,#43679,.F.) ;
#61589=ORIENTED_EDGE('',*,*,#42718,.F.) ;
#61590=ORIENTED_EDGE('',*,*,#43679,.T.) ;
#61591=ORIENTED_EDGE('',*,*,#43340,.F.) ;
#61592=ORIENTED_EDGE('',*,*,#43338,.F.) ;
#61593=ORIENTED_EDGE('',*,*,#43680,.F.) ;
#61594=ORIENTED_EDGE('',*,*,#43680,.T.) ;
#61595=ORIENTED_EDGE('',*,*,#43211,.F.) ;
#61596=ORIENTED_EDGE('',*,*,#43681,.F.) ;
#61597=ORIENTED_EDGE('',*,*,#42719,.F.) ;
#61598=ORIENTED_EDGE('',*,*,#43681,.T.) ;
#61599=ORIENTED_EDGE('',*,*,#43353,.F.) ;
#61600=ORIENTED_EDGE('',*,*,#43355,.F.) ;
#61601=ORIENTED_EDGE('',*,*,#43682,.F.) ;
#61602=ORIENTED_EDGE('',*,*,#43682,.T.) ;
#61603=ORIENTED_EDGE('',*,*,#42691,.F.) ;
#61604=ORIENTED_EDGE('',*,*,#43683,.F.) ;
#61605=ORIENTED_EDGE('',*,*,#42715,.F.) ;
#61606=ORIENTED_EDGE('',*,*,#39223,.F.) ;
#61607=ORIENTED_EDGE('',*,*,#42716,.F.) ;
#61608=ORIENTED_EDGE('',*,*,#43683,.T.) ;
#61609=ORIENTED_EDGE('',*,*,#42720,.F.) ;
#61610=ORIENTED_EDGE('',*,*,#41938,.F.) ;
#61611=ORIENTED_EDGE('',*,*,#41941,.F.) ;
#61612=ORIENTED_EDGE('',*,*,#42721,.F.) ;
#61613=ORIENTED_EDGE('',*,*,#43684,.F.) ;
#61614=ORIENTED_EDGE('',*,*,#42712,.F.) ;
#61615=ORIENTED_EDGE('',*,*,#43684,.T.) ;
#61616=ORIENTED_EDGE('',*,*,#42693,.F.) ;
#61617=ORIENTED_EDGE('',*,*,#43685,.F.) ;
#61618=ORIENTED_EDGE('',*,*,#42713,.F.) ;
#61619=ORIENTED_EDGE('',*,*,#43685,.T.) ;
#61620=ORIENTED_EDGE('',*,*,#43356,.F.) ;
#61621=ORIENTED_EDGE('',*,*,#43357,.F.) ;
#61622=ORIENTED_EDGE('',*,*,#43686,.F.) ;
#61623=ORIENTED_EDGE('',*,*,#43686,.T.) ;
#61624=ORIENTED_EDGE('',*,*,#43215,.F.) ;
#61625=ORIENTED_EDGE('',*,*,#43687,.F.) ;
#61626=ORIENTED_EDGE('',*,*,#42714,.F.) ;
#61627=ORIENTED_EDGE('',*,*,#43687,.T.) ;
#61628=ORIENTED_EDGE('',*,*,#43344,.F.) ;
#61629=ORIENTED_EDGE('',*,*,#43341,.F.) ;
#61630=ORIENTED_EDGE('',*,*,#43688,.F.) ;
#61631=ORIENTED_EDGE('',*,*,#43688,.T.) ;
#61632=ORIENTED_EDGE('',*,*,#42709,.F.) ;
#61633=ORIENTED_EDGE('',*,*,#43689,.F.) ;
#61634=ORIENTED_EDGE('',*,*,#42710,.F.) ;
#61635=ORIENTED_EDGE('',*,*,#43689,.T.) ;
#61636=ORIENTED_EDGE('',*,*,#42723,.F.) ;
#61637=ORIENTED_EDGE('',*,*,#39416,.F.) ;
#61638=ORIENTED_EDGE('',*,*,#42711,.F.) ;
#61639=ORIENTED_EDGE('',*,*,#41545,.F.) ;
#61640=ORIENTED_EDGE('',*,*,#42729,.F.) ;
#61641=ORIENTED_EDGE('',*,*,#43690,.F.) ;
#61642=ORIENTED_EDGE('',*,*,#42745,.F.) ;
#61643=ORIENTED_EDGE('',*,*,#43690,.T.) ;
#61644=ORIENTED_EDGE('',*,*,#43360,.F.) ;
#61645=ORIENTED_EDGE('',*,*,#43358,.F.) ;
#61646=ORIENTED_EDGE('',*,*,#43691,.F.) ;
#61647=ORIENTED_EDGE('',*,*,#43691,.T.) ;
#61648=ORIENTED_EDGE('',*,*,#43283,.F.) ;
#61649=ORIENTED_EDGE('',*,*,#43692,.F.) ;
#61650=ORIENTED_EDGE('',*,*,#42746,.F.) ;
#61651=ORIENTED_EDGE('',*,*,#43692,.T.) ;
#61652=ORIENTED_EDGE('',*,*,#43373,.F.) ;
#61653=ORIENTED_EDGE('',*,*,#43375,.F.) ;
#61654=ORIENTED_EDGE('',*,*,#43693,.F.) ;
#61655=ORIENTED_EDGE('',*,*,#41547,.F.) ;
#61656=ORIENTED_EDGE('',*,*,#42747,.F.) ;
#61657=ORIENTED_EDGE('',*,*,#43693,.T.) ;
#61658=ORIENTED_EDGE('',*,*,#42731,.F.) ;
#61659=ORIENTED_EDGE('',*,*,#43694,.F.) ;
#61660=ORIENTED_EDGE('',*,*,#42730,.F.) ;
#61661=ORIENTED_EDGE('',*,*,#41543,.F.) ;
#61662=ORIENTED_EDGE('',*,*,#42743,.F.) ;
#61663=ORIENTED_EDGE('',*,*,#43361,.F.) ;
#61664=ORIENTED_EDGE('',*,*,#43694,.T.) ;
#61665=ORIENTED_EDGE('',*,*,#43695,.F.) ;
#61666=ORIENTED_EDGE('',*,*,#43364,.F.) ;
#61667=ORIENTED_EDGE('',*,*,#43695,.T.) ;
#61668=ORIENTED_EDGE('',*,*,#42742,.F.) ;
#61669=ORIENTED_EDGE('',*,*,#43696,.F.) ;
#61670=ORIENTED_EDGE('',*,*,#43287,.F.) ;
#61671=ORIENTED_EDGE('',*,*,#41549,.F.) ;
#61672=ORIENTED_EDGE('',*,*,#42733,.F.) ;
#61673=ORIENTED_EDGE('',*,*,#43697,.F.) ;
#61674=ORIENTED_EDGE('',*,*,#42744,.F.) ;
#61675=ORIENTED_EDGE('',*,*,#43377,.F.) ;
#61676=ORIENTED_EDGE('',*,*,#43696,.T.) ;
#61677=ORIENTED_EDGE('',*,*,#43697,.T.) ;
#61678=ORIENTED_EDGE('',*,*,#43376,.F.) ;
#61679=ORIENTED_EDGE('',*,*,#39407,.F.) ;
#61680=ORIENTED_EDGE('',*,*,#42780,.F.) ;
#61681=ORIENTED_EDGE('',*,*,#43698,.F.) ;
#61682=ORIENTED_EDGE('',*,*,#42775,.F.) ;
#61683=ORIENTED_EDGE('',*,*,#43698,.T.) ;
#61684=ORIENTED_EDGE('',*,*,#42765,.F.) ;
#61685=ORIENTED_EDGE('',*,*,#43699,.F.) ;
#61686=ORIENTED_EDGE('',*,*,#42776,.F.) ;
#61687=ORIENTED_EDGE('',*,*,#43699,.T.) ;
#61688=ORIENTED_EDGE('',*,*,#43380,.F.) ;
#61689=ORIENTED_EDGE('',*,*,#43378,.F.) ;
#61690=ORIENTED_EDGE('',*,*,#43700,.F.) ;
#61691=ORIENTED_EDGE('',*,*,#43700,.T.) ;
#61692=ORIENTED_EDGE('',*,*,#43203,.F.) ;
#61693=ORIENTED_EDGE('',*,*,#43701,.F.) ;
#61694=ORIENTED_EDGE('',*,*,#42777,.F.) ;
#61695=ORIENTED_EDGE('',*,*,#43701,.T.) ;
#61696=ORIENTED_EDGE('',*,*,#43393,.F.) ;
#61697=ORIENTED_EDGE('',*,*,#43395,.F.) ;
#61698=ORIENTED_EDGE('',*,*,#43702,.F.) ;
#61699=ORIENTED_EDGE('',*,*,#43702,.T.) ;
#61700=ORIENTED_EDGE('',*,*,#42749,.F.) ;
#61701=ORIENTED_EDGE('',*,*,#43703,.F.) ;
#61702=ORIENTED_EDGE('',*,*,#42773,.F.) ;
#61703=ORIENTED_EDGE('',*,*,#39206,.F.) ;
#61704=ORIENTED_EDGE('',*,*,#42774,.F.) ;
#61705=ORIENTED_EDGE('',*,*,#43703,.T.) ;
#61706=ORIENTED_EDGE('',*,*,#42778,.F.) ;
#61707=ORIENTED_EDGE('',*,*,#42026,.F.) ;
#61708=ORIENTED_EDGE('',*,*,#42029,.F.) ;
#61709=ORIENTED_EDGE('',*,*,#42779,.F.) ;
#61710=ORIENTED_EDGE('',*,*,#43704,.F.) ;
#61711=ORIENTED_EDGE('',*,*,#42770,.F.) ;
#61712=ORIENTED_EDGE('',*,*,#43704,.T.) ;
#61713=ORIENTED_EDGE('',*,*,#42751,.F.) ;
#61714=ORIENTED_EDGE('',*,*,#43705,.F.) ;
#61715=ORIENTED_EDGE('',*,*,#42771,.F.) ;
#61716=ORIENTED_EDGE('',*,*,#43705,.T.) ;
#61717=ORIENTED_EDGE('',*,*,#43396,.F.) ;
#61718=ORIENTED_EDGE('',*,*,#43397,.F.) ;
#61719=ORIENTED_EDGE('',*,*,#43706,.F.) ;
#61720=ORIENTED_EDGE('',*,*,#43706,.T.) ;
#61721=ORIENTED_EDGE('',*,*,#43207,.F.) ;
#61722=ORIENTED_EDGE('',*,*,#43707,.F.) ;
#61723=ORIENTED_EDGE('',*,*,#42772,.F.) ;
#61724=ORIENTED_EDGE('',*,*,#43707,.T.) ;
#61725=ORIENTED_EDGE('',*,*,#43384,.F.) ;
#61726=ORIENTED_EDGE('',*,*,#43381,.F.) ;
#61727=ORIENTED_EDGE('',*,*,#43708,.F.) ;
#61728=ORIENTED_EDGE('',*,*,#43708,.T.) ;
#61729=ORIENTED_EDGE('',*,*,#42767,.F.) ;
#61730=ORIENTED_EDGE('',*,*,#43709,.F.) ;
#61731=ORIENTED_EDGE('',*,*,#42768,.F.) ;
#61732=ORIENTED_EDGE('',*,*,#43709,.T.) ;
#61733=ORIENTED_EDGE('',*,*,#42781,.F.) ;
#61734=ORIENTED_EDGE('',*,*,#39405,.F.) ;
#61735=ORIENTED_EDGE('',*,*,#42769,.F.) ;
#61736=ORIENTED_EDGE('',*,*,#41553,.F.) ;
#61737=ORIENTED_EDGE('',*,*,#42787,.F.) ;
#61738=ORIENTED_EDGE('',*,*,#43710,.F.) ;
#61739=ORIENTED_EDGE('',*,*,#42803,.F.) ;
#61740=ORIENTED_EDGE('',*,*,#43710,.T.) ;
#61741=ORIENTED_EDGE('',*,*,#43400,.F.) ;
#61742=ORIENTED_EDGE('',*,*,#43398,.F.) ;
#61743=ORIENTED_EDGE('',*,*,#43711,.F.) ;
#61744=ORIENTED_EDGE('',*,*,#43711,.T.) ;
#61745=ORIENTED_EDGE('',*,*,#43275,.F.) ;
#61746=ORIENTED_EDGE('',*,*,#43712,.F.) ;
#61747=ORIENTED_EDGE('',*,*,#42804,.F.) ;
#61748=ORIENTED_EDGE('',*,*,#43712,.T.) ;
#61749=ORIENTED_EDGE('',*,*,#43413,.F.) ;
#61750=ORIENTED_EDGE('',*,*,#43415,.F.) ;
#61751=ORIENTED_EDGE('',*,*,#43713,.F.) ;
#61752=ORIENTED_EDGE('',*,*,#41555,.F.) ;
#61753=ORIENTED_EDGE('',*,*,#42805,.F.) ;
#61754=ORIENTED_EDGE('',*,*,#43713,.T.) ;
#61755=ORIENTED_EDGE('',*,*,#42789,.F.) ;
#61756=ORIENTED_EDGE('',*,*,#43714,.F.) ;
#61757=ORIENTED_EDGE('',*,*,#42788,.F.) ;
#61758=ORIENTED_EDGE('',*,*,#41551,.F.) ;
#61759=ORIENTED_EDGE('',*,*,#42801,.F.) ;
#61760=ORIENTED_EDGE('',*,*,#43401,.F.) ;
#61761=ORIENTED_EDGE('',*,*,#43714,.T.) ;
#61762=ORIENTED_EDGE('',*,*,#43715,.F.) ;
#61763=ORIENTED_EDGE('',*,*,#43404,.F.) ;
#61764=ORIENTED_EDGE('',*,*,#43715,.T.) ;
#61765=ORIENTED_EDGE('',*,*,#42800,.F.) ;
#61766=ORIENTED_EDGE('',*,*,#43716,.F.) ;
#61767=ORIENTED_EDGE('',*,*,#43279,.F.) ;
#61768=ORIENTED_EDGE('',*,*,#41557,.F.) ;
#61769=ORIENTED_EDGE('',*,*,#42791,.F.) ;
#61770=ORIENTED_EDGE('',*,*,#43717,.F.) ;
#61771=ORIENTED_EDGE('',*,*,#42802,.F.) ;
#61772=ORIENTED_EDGE('',*,*,#43417,.F.) ;
#61773=ORIENTED_EDGE('',*,*,#43716,.T.) ;
#61774=ORIENTED_EDGE('',*,*,#43717,.T.) ;
#61775=ORIENTED_EDGE('',*,*,#43416,.F.) ;
#61776=ORIENTED_EDGE('',*,*,#39396,.F.) ;
#61777=ORIENTED_EDGE('',*,*,#42838,.F.) ;
#61778=ORIENTED_EDGE('',*,*,#43718,.F.) ;
#61779=ORIENTED_EDGE('',*,*,#42833,.F.) ;
#61780=ORIENTED_EDGE('',*,*,#43718,.T.) ;
#61781=ORIENTED_EDGE('',*,*,#42823,.F.) ;
#61782=ORIENTED_EDGE('',*,*,#43719,.F.) ;
#61783=ORIENTED_EDGE('',*,*,#42834,.F.) ;
#61784=ORIENTED_EDGE('',*,*,#43719,.T.) ;
#61785=ORIENTED_EDGE('',*,*,#43420,.F.) ;
#61786=ORIENTED_EDGE('',*,*,#43418,.F.) ;
#61787=ORIENTED_EDGE('',*,*,#43720,.F.) ;
#61788=ORIENTED_EDGE('',*,*,#43720,.T.) ;
#61789=ORIENTED_EDGE('',*,*,#43195,.F.) ;
#61790=ORIENTED_EDGE('',*,*,#43721,.F.) ;
#61791=ORIENTED_EDGE('',*,*,#42835,.F.) ;
#61792=ORIENTED_EDGE('',*,*,#43721,.T.) ;
#61793=ORIENTED_EDGE('',*,*,#43433,.F.) ;
#61794=ORIENTED_EDGE('',*,*,#43435,.F.) ;
#61795=ORIENTED_EDGE('',*,*,#43722,.F.) ;
#61796=ORIENTED_EDGE('',*,*,#43722,.T.) ;
#61797=ORIENTED_EDGE('',*,*,#42807,.F.) ;
#61798=ORIENTED_EDGE('',*,*,#43723,.F.) ;
#61799=ORIENTED_EDGE('',*,*,#42831,.F.) ;
#61800=ORIENTED_EDGE('',*,*,#39189,.F.) ;
#61801=ORIENTED_EDGE('',*,*,#42832,.F.) ;
#61802=ORIENTED_EDGE('',*,*,#43723,.T.) ;
#61803=ORIENTED_EDGE('',*,*,#42836,.F.) ;
#61804=ORIENTED_EDGE('',*,*,#42114,.F.) ;
#61805=ORIENTED_EDGE('',*,*,#42117,.F.) ;
#61806=ORIENTED_EDGE('',*,*,#42837,.F.) ;
#61807=ORIENTED_EDGE('',*,*,#43724,.F.) ;
#61808=ORIENTED_EDGE('',*,*,#42828,.F.) ;
#61809=ORIENTED_EDGE('',*,*,#43724,.T.) ;
#61810=ORIENTED_EDGE('',*,*,#42809,.F.) ;
#61811=ORIENTED_EDGE('',*,*,#43725,.F.) ;
#61812=ORIENTED_EDGE('',*,*,#42829,.F.) ;
#61813=ORIENTED_EDGE('',*,*,#43725,.T.) ;
#61814=ORIENTED_EDGE('',*,*,#43436,.F.) ;
#61815=ORIENTED_EDGE('',*,*,#43437,.F.) ;
#61816=ORIENTED_EDGE('',*,*,#43726,.F.) ;
#61817=ORIENTED_EDGE('',*,*,#43726,.T.) ;
#61818=ORIENTED_EDGE('',*,*,#43199,.F.) ;
#61819=ORIENTED_EDGE('',*,*,#43727,.F.) ;
#61820=ORIENTED_EDGE('',*,*,#42830,.F.) ;
#61821=ORIENTED_EDGE('',*,*,#43727,.T.) ;
#61822=ORIENTED_EDGE('',*,*,#43424,.F.) ;
#61823=ORIENTED_EDGE('',*,*,#43421,.F.) ;
#61824=ORIENTED_EDGE('',*,*,#43728,.F.) ;
#61825=ORIENTED_EDGE('',*,*,#43728,.T.) ;
#61826=ORIENTED_EDGE('',*,*,#42825,.F.) ;
#61827=ORIENTED_EDGE('',*,*,#43729,.F.) ;
#61828=ORIENTED_EDGE('',*,*,#42826,.F.) ;
#61829=ORIENTED_EDGE('',*,*,#43729,.T.) ;
#61830=ORIENTED_EDGE('',*,*,#42839,.F.) ;
#61831=ORIENTED_EDGE('',*,*,#39394,.F.) ;
#61832=ORIENTED_EDGE('',*,*,#42827,.F.) ;
#61833=ORIENTED_EDGE('',*,*,#41561,.F.) ;
#61834=ORIENTED_EDGE('',*,*,#42845,.F.) ;
#61835=ORIENTED_EDGE('',*,*,#43730,.F.) ;
#61836=ORIENTED_EDGE('',*,*,#42861,.F.) ;
#61837=ORIENTED_EDGE('',*,*,#43730,.T.) ;
#61838=ORIENTED_EDGE('',*,*,#43440,.F.) ;
#61839=ORIENTED_EDGE('',*,*,#43438,.F.) ;
#61840=ORIENTED_EDGE('',*,*,#43731,.F.) ;
#61841=ORIENTED_EDGE('',*,*,#43731,.T.) ;
#61842=ORIENTED_EDGE('',*,*,#43267,.F.) ;
#61843=ORIENTED_EDGE('',*,*,#43732,.F.) ;
#61844=ORIENTED_EDGE('',*,*,#42862,.F.) ;
#61845=ORIENTED_EDGE('',*,*,#43732,.T.) ;
#61846=ORIENTED_EDGE('',*,*,#43453,.F.) ;
#61847=ORIENTED_EDGE('',*,*,#43455,.F.) ;
#61848=ORIENTED_EDGE('',*,*,#43733,.F.) ;
#61849=ORIENTED_EDGE('',*,*,#41563,.F.) ;
#61850=ORIENTED_EDGE('',*,*,#42863,.F.) ;
#61851=ORIENTED_EDGE('',*,*,#43733,.T.) ;
#61852=ORIENTED_EDGE('',*,*,#42847,.F.) ;
#61853=ORIENTED_EDGE('',*,*,#43734,.F.) ;
#61854=ORIENTED_EDGE('',*,*,#42846,.F.) ;
#61855=ORIENTED_EDGE('',*,*,#41559,.F.) ;
#61856=ORIENTED_EDGE('',*,*,#42859,.F.) ;
#61857=ORIENTED_EDGE('',*,*,#43441,.F.) ;
#61858=ORIENTED_EDGE('',*,*,#43734,.T.) ;
#61859=ORIENTED_EDGE('',*,*,#43735,.F.) ;
#61860=ORIENTED_EDGE('',*,*,#43444,.F.) ;
#61861=ORIENTED_EDGE('',*,*,#43735,.T.) ;
#61862=ORIENTED_EDGE('',*,*,#42858,.F.) ;
#61863=ORIENTED_EDGE('',*,*,#43736,.F.) ;
#61864=ORIENTED_EDGE('',*,*,#43271,.F.) ;
#61865=ORIENTED_EDGE('',*,*,#41565,.F.) ;
#61866=ORIENTED_EDGE('',*,*,#42849,.F.) ;
#61867=ORIENTED_EDGE('',*,*,#43737,.F.) ;
#61868=ORIENTED_EDGE('',*,*,#42860,.F.) ;
#61869=ORIENTED_EDGE('',*,*,#43457,.F.) ;
#61870=ORIENTED_EDGE('',*,*,#43736,.T.) ;
#61871=ORIENTED_EDGE('',*,*,#43737,.T.) ;
#61872=ORIENTED_EDGE('',*,*,#43456,.F.) ;
#61873=ORIENTED_EDGE('',*,*,#39385,.F.) ;
#61874=ORIENTED_EDGE('',*,*,#42896,.F.) ;
#61875=ORIENTED_EDGE('',*,*,#43738,.F.) ;
#61876=ORIENTED_EDGE('',*,*,#42891,.F.) ;
#61877=ORIENTED_EDGE('',*,*,#43738,.T.) ;
#61878=ORIENTED_EDGE('',*,*,#42881,.F.) ;
#61879=ORIENTED_EDGE('',*,*,#43739,.F.) ;
#61880=ORIENTED_EDGE('',*,*,#42892,.F.) ;
#61881=ORIENTED_EDGE('',*,*,#43739,.T.) ;
#61882=ORIENTED_EDGE('',*,*,#43460,.F.) ;
#61883=ORIENTED_EDGE('',*,*,#43458,.F.) ;
#61884=ORIENTED_EDGE('',*,*,#43740,.F.) ;
#61885=ORIENTED_EDGE('',*,*,#43740,.T.) ;
#61886=ORIENTED_EDGE('',*,*,#43187,.F.) ;
#61887=ORIENTED_EDGE('',*,*,#43741,.F.) ;
#61888=ORIENTED_EDGE('',*,*,#42893,.F.) ;
#61889=ORIENTED_EDGE('',*,*,#43741,.T.) ;
#61890=ORIENTED_EDGE('',*,*,#43473,.F.) ;
#61891=ORIENTED_EDGE('',*,*,#43475,.F.) ;
#61892=ORIENTED_EDGE('',*,*,#43742,.F.) ;
#61893=ORIENTED_EDGE('',*,*,#43742,.T.) ;
#61894=ORIENTED_EDGE('',*,*,#42865,.F.) ;
#61895=ORIENTED_EDGE('',*,*,#43743,.F.) ;
#61896=ORIENTED_EDGE('',*,*,#42889,.F.) ;
#61897=ORIENTED_EDGE('',*,*,#39172,.F.) ;
#61898=ORIENTED_EDGE('',*,*,#42890,.F.) ;
#61899=ORIENTED_EDGE('',*,*,#43743,.T.) ;
#61900=ORIENTED_EDGE('',*,*,#42894,.F.) ;
#61901=ORIENTED_EDGE('',*,*,#42202,.F.) ;
#61902=ORIENTED_EDGE('',*,*,#42205,.F.) ;
#61903=ORIENTED_EDGE('',*,*,#42895,.F.) ;
#61904=ORIENTED_EDGE('',*,*,#43744,.F.) ;
#61905=ORIENTED_EDGE('',*,*,#42886,.F.) ;
#61906=ORIENTED_EDGE('',*,*,#43744,.T.) ;
#61907=ORIENTED_EDGE('',*,*,#42867,.F.) ;
#61908=ORIENTED_EDGE('',*,*,#43745,.F.) ;
#61909=ORIENTED_EDGE('',*,*,#42887,.F.) ;
#61910=ORIENTED_EDGE('',*,*,#43745,.T.) ;
#61911=ORIENTED_EDGE('',*,*,#43476,.F.) ;
#61912=ORIENTED_EDGE('',*,*,#43477,.F.) ;
#61913=ORIENTED_EDGE('',*,*,#43746,.F.) ;
#61914=ORIENTED_EDGE('',*,*,#43746,.T.) ;
#61915=ORIENTED_EDGE('',*,*,#43191,.F.) ;
#61916=ORIENTED_EDGE('',*,*,#43747,.F.) ;
#61917=ORIENTED_EDGE('',*,*,#42888,.F.) ;
#61918=ORIENTED_EDGE('',*,*,#43747,.T.) ;
#61919=ORIENTED_EDGE('',*,*,#43464,.F.) ;
#61920=ORIENTED_EDGE('',*,*,#43461,.F.) ;
#61921=ORIENTED_EDGE('',*,*,#43748,.F.) ;
#61922=ORIENTED_EDGE('',*,*,#43748,.T.) ;
#61923=ORIENTED_EDGE('',*,*,#42883,.F.) ;
#61924=ORIENTED_EDGE('',*,*,#43749,.F.) ;
#61925=ORIENTED_EDGE('',*,*,#42884,.F.) ;
#61926=ORIENTED_EDGE('',*,*,#43749,.T.) ;
#61927=ORIENTED_EDGE('',*,*,#42897,.F.) ;
#61928=ORIENTED_EDGE('',*,*,#39383,.F.) ;
#61929=ORIENTED_EDGE('',*,*,#42885,.F.) ;
#61930=ORIENTED_EDGE('',*,*,#41569,.F.) ;
#61931=ORIENTED_EDGE('',*,*,#42903,.F.) ;
#61932=ORIENTED_EDGE('',*,*,#43750,.F.) ;
#61933=ORIENTED_EDGE('',*,*,#42919,.F.) ;
#61934=ORIENTED_EDGE('',*,*,#43750,.T.) ;
#61935=ORIENTED_EDGE('',*,*,#43480,.F.) ;
#61936=ORIENTED_EDGE('',*,*,#43478,.F.) ;
#61937=ORIENTED_EDGE('',*,*,#43751,.F.) ;
#61938=ORIENTED_EDGE('',*,*,#43751,.T.) ;
#61939=ORIENTED_EDGE('',*,*,#43259,.F.) ;
#61940=ORIENTED_EDGE('',*,*,#43752,.F.) ;
#61941=ORIENTED_EDGE('',*,*,#42920,.F.) ;
#61942=ORIENTED_EDGE('',*,*,#43752,.T.) ;
#61943=ORIENTED_EDGE('',*,*,#43493,.F.) ;
#61944=ORIENTED_EDGE('',*,*,#43495,.F.) ;
#61945=ORIENTED_EDGE('',*,*,#43753,.F.) ;
#61946=ORIENTED_EDGE('',*,*,#41571,.F.) ;
#61947=ORIENTED_EDGE('',*,*,#42921,.F.) ;
#61948=ORIENTED_EDGE('',*,*,#43753,.T.) ;
#61949=ORIENTED_EDGE('',*,*,#42905,.F.) ;
#61950=ORIENTED_EDGE('',*,*,#43754,.F.) ;
#61951=ORIENTED_EDGE('',*,*,#42904,.F.) ;
#61952=ORIENTED_EDGE('',*,*,#41567,.F.) ;
#61953=ORIENTED_EDGE('',*,*,#42917,.F.) ;
#61954=ORIENTED_EDGE('',*,*,#43481,.F.) ;
#61955=ORIENTED_EDGE('',*,*,#43754,.T.) ;
#61956=ORIENTED_EDGE('',*,*,#43755,.F.) ;
#61957=ORIENTED_EDGE('',*,*,#43484,.F.) ;
#61958=ORIENTED_EDGE('',*,*,#43755,.T.) ;
#61959=ORIENTED_EDGE('',*,*,#42916,.F.) ;
#61960=ORIENTED_EDGE('',*,*,#43756,.F.) ;
#61961=ORIENTED_EDGE('',*,*,#43263,.F.) ;
#61962=ORIENTED_EDGE('',*,*,#41573,.F.) ;
#61963=ORIENTED_EDGE('',*,*,#42907,.F.) ;
#61964=ORIENTED_EDGE('',*,*,#43757,.F.) ;
#61965=ORIENTED_EDGE('',*,*,#42918,.F.) ;
#61966=ORIENTED_EDGE('',*,*,#43497,.F.) ;
#61967=ORIENTED_EDGE('',*,*,#43756,.T.) ;
#61968=ORIENTED_EDGE('',*,*,#43757,.T.) ;
#61969=ORIENTED_EDGE('',*,*,#43496,.F.) ;
#61970=ORIENTED_EDGE('',*,*,#39374,.F.) ;
#61971=ORIENTED_EDGE('',*,*,#42954,.F.) ;
#61972=ORIENTED_EDGE('',*,*,#43758,.F.) ;
#61973=ORIENTED_EDGE('',*,*,#42949,.F.) ;
#61974=ORIENTED_EDGE('',*,*,#43758,.T.) ;
#61975=ORIENTED_EDGE('',*,*,#42939,.F.) ;
#61976=ORIENTED_EDGE('',*,*,#43759,.F.) ;
#61977=ORIENTED_EDGE('',*,*,#42950,.F.) ;
#61978=ORIENTED_EDGE('',*,*,#43759,.T.) ;
#61979=ORIENTED_EDGE('',*,*,#43500,.F.) ;
#61980=ORIENTED_EDGE('',*,*,#43498,.F.) ;
#61981=ORIENTED_EDGE('',*,*,#43760,.F.) ;
#61982=ORIENTED_EDGE('',*,*,#43760,.T.) ;
#61983=ORIENTED_EDGE('',*,*,#43179,.F.) ;
#61984=ORIENTED_EDGE('',*,*,#43761,.F.) ;
#61985=ORIENTED_EDGE('',*,*,#42951,.F.) ;
#61986=ORIENTED_EDGE('',*,*,#43761,.T.) ;
#61987=ORIENTED_EDGE('',*,*,#43513,.F.) ;
#61988=ORIENTED_EDGE('',*,*,#43515,.F.) ;
#61989=ORIENTED_EDGE('',*,*,#43762,.F.) ;
#61990=ORIENTED_EDGE('',*,*,#43762,.T.) ;
#61991=ORIENTED_EDGE('',*,*,#42923,.F.) ;
#61992=ORIENTED_EDGE('',*,*,#43763,.F.) ;
#61993=ORIENTED_EDGE('',*,*,#42947,.F.) ;
#61994=ORIENTED_EDGE('',*,*,#39155,.F.) ;
#61995=ORIENTED_EDGE('',*,*,#42948,.F.) ;
#61996=ORIENTED_EDGE('',*,*,#43763,.T.) ;
#61997=ORIENTED_EDGE('',*,*,#42952,.F.) ;
#61998=ORIENTED_EDGE('',*,*,#42290,.F.) ;
#61999=ORIENTED_EDGE('',*,*,#42293,.F.) ;
#62000=ORIENTED_EDGE('',*,*,#42953,.F.) ;
#62001=ORIENTED_EDGE('',*,*,#43764,.F.) ;
#62002=ORIENTED_EDGE('',*,*,#42944,.F.) ;
#62003=ORIENTED_EDGE('',*,*,#43764,.T.) ;
#62004=ORIENTED_EDGE('',*,*,#42925,.F.) ;
#62005=ORIENTED_EDGE('',*,*,#43765,.F.) ;
#62006=ORIENTED_EDGE('',*,*,#42945,.F.) ;
#62007=ORIENTED_EDGE('',*,*,#43765,.T.) ;
#62008=ORIENTED_EDGE('',*,*,#43516,.F.) ;
#62009=ORIENTED_EDGE('',*,*,#43517,.F.) ;
#62010=ORIENTED_EDGE('',*,*,#43766,.F.) ;
#62011=ORIENTED_EDGE('',*,*,#43766,.T.) ;
#62012=ORIENTED_EDGE('',*,*,#43183,.F.) ;
#62013=ORIENTED_EDGE('',*,*,#43767,.F.) ;
#62014=ORIENTED_EDGE('',*,*,#42946,.F.) ;
#62015=ORIENTED_EDGE('',*,*,#43767,.T.) ;
#62016=ORIENTED_EDGE('',*,*,#43504,.F.) ;
#62017=ORIENTED_EDGE('',*,*,#43501,.F.) ;
#62018=ORIENTED_EDGE('',*,*,#43768,.F.) ;
#62019=ORIENTED_EDGE('',*,*,#43768,.T.) ;
#62020=ORIENTED_EDGE('',*,*,#42941,.F.) ;
#62021=ORIENTED_EDGE('',*,*,#43769,.F.) ;
#62022=ORIENTED_EDGE('',*,*,#42942,.F.) ;
#62023=ORIENTED_EDGE('',*,*,#43769,.T.) ;
#62024=ORIENTED_EDGE('',*,*,#42955,.F.) ;
#62025=ORIENTED_EDGE('',*,*,#39372,.F.) ;
#62026=ORIENTED_EDGE('',*,*,#42943,.F.) ;
#62027=ORIENTED_EDGE('',*,*,#41577,.F.) ;
#62028=ORIENTED_EDGE('',*,*,#42961,.F.) ;
#62029=ORIENTED_EDGE('',*,*,#43770,.F.) ;
#62030=ORIENTED_EDGE('',*,*,#42977,.F.) ;
#62031=ORIENTED_EDGE('',*,*,#43770,.T.) ;
#62032=ORIENTED_EDGE('',*,*,#43520,.F.) ;
#62033=ORIENTED_EDGE('',*,*,#43518,.F.) ;
#62034=ORIENTED_EDGE('',*,*,#43771,.F.) ;
#62035=ORIENTED_EDGE('',*,*,#43771,.T.) ;
#62036=ORIENTED_EDGE('',*,*,#43251,.F.) ;
#62037=ORIENTED_EDGE('',*,*,#43772,.F.) ;
#62038=ORIENTED_EDGE('',*,*,#42978,.F.) ;
#62039=ORIENTED_EDGE('',*,*,#43772,.T.) ;
#62040=ORIENTED_EDGE('',*,*,#43533,.F.) ;
#62041=ORIENTED_EDGE('',*,*,#43535,.F.) ;
#62042=ORIENTED_EDGE('',*,*,#43773,.F.) ;
#62043=ORIENTED_EDGE('',*,*,#41579,.F.) ;
#62044=ORIENTED_EDGE('',*,*,#42979,.F.) ;
#62045=ORIENTED_EDGE('',*,*,#43773,.T.) ;
#62046=ORIENTED_EDGE('',*,*,#42963,.F.) ;
#62047=ORIENTED_EDGE('',*,*,#43774,.F.) ;
#62048=ORIENTED_EDGE('',*,*,#42962,.F.) ;
#62049=ORIENTED_EDGE('',*,*,#41575,.F.) ;
#62050=ORIENTED_EDGE('',*,*,#42975,.F.) ;
#62051=ORIENTED_EDGE('',*,*,#43521,.F.) ;
#62052=ORIENTED_EDGE('',*,*,#43774,.T.) ;
#62053=ORIENTED_EDGE('',*,*,#43775,.F.) ;
#62054=ORIENTED_EDGE('',*,*,#43524,.F.) ;
#62055=ORIENTED_EDGE('',*,*,#43775,.T.) ;
#62056=ORIENTED_EDGE('',*,*,#42974,.F.) ;
#62057=ORIENTED_EDGE('',*,*,#43776,.F.) ;
#62058=ORIENTED_EDGE('',*,*,#43255,.F.) ;
#62059=ORIENTED_EDGE('',*,*,#41581,.F.) ;
#62060=ORIENTED_EDGE('',*,*,#42965,.F.) ;
#62061=ORIENTED_EDGE('',*,*,#43777,.F.) ;
#62062=ORIENTED_EDGE('',*,*,#42976,.F.) ;
#62063=ORIENTED_EDGE('',*,*,#43537,.F.) ;
#62064=ORIENTED_EDGE('',*,*,#43776,.T.) ;
#62065=ORIENTED_EDGE('',*,*,#43777,.T.) ;
#62066=ORIENTED_EDGE('',*,*,#43536,.F.) ;
#62067=ORIENTED_EDGE('',*,*,#39363,.F.) ;
#62068=ORIENTED_EDGE('',*,*,#43012,.F.) ;
#62069=ORIENTED_EDGE('',*,*,#43778,.F.) ;
#62070=ORIENTED_EDGE('',*,*,#43007,.F.) ;
#62071=ORIENTED_EDGE('',*,*,#43778,.T.) ;
#62072=ORIENTED_EDGE('',*,*,#42997,.F.) ;
#62073=ORIENTED_EDGE('',*,*,#43779,.F.) ;
#62074=ORIENTED_EDGE('',*,*,#43008,.F.) ;
#62075=ORIENTED_EDGE('',*,*,#43779,.T.) ;
#62076=ORIENTED_EDGE('',*,*,#43540,.F.) ;
#62077=ORIENTED_EDGE('',*,*,#43538,.F.) ;
#62078=ORIENTED_EDGE('',*,*,#43780,.F.) ;
#62079=ORIENTED_EDGE('',*,*,#43780,.T.) ;
#62080=ORIENTED_EDGE('',*,*,#43171,.F.) ;
#62081=ORIENTED_EDGE('',*,*,#43781,.F.) ;
#62082=ORIENTED_EDGE('',*,*,#43009,.F.) ;
#62083=ORIENTED_EDGE('',*,*,#43781,.T.) ;
#62084=ORIENTED_EDGE('',*,*,#43553,.F.) ;
#62085=ORIENTED_EDGE('',*,*,#43555,.F.) ;
#62086=ORIENTED_EDGE('',*,*,#43782,.F.) ;
#62087=ORIENTED_EDGE('',*,*,#43782,.T.) ;
#62088=ORIENTED_EDGE('',*,*,#42981,.F.) ;
#62089=ORIENTED_EDGE('',*,*,#43783,.F.) ;
#62090=ORIENTED_EDGE('',*,*,#43005,.F.) ;
#62091=ORIENTED_EDGE('',*,*,#39138,.F.) ;
#62092=ORIENTED_EDGE('',*,*,#43006,.F.) ;
#62093=ORIENTED_EDGE('',*,*,#43783,.T.) ;
#62094=ORIENTED_EDGE('',*,*,#43010,.F.) ;
#62095=ORIENTED_EDGE('',*,*,#42378,.F.) ;
#62096=ORIENTED_EDGE('',*,*,#42381,.F.) ;
#62097=ORIENTED_EDGE('',*,*,#43011,.F.) ;
#62098=ORIENTED_EDGE('',*,*,#43784,.F.) ;
#62099=ORIENTED_EDGE('',*,*,#43002,.F.) ;
#62100=ORIENTED_EDGE('',*,*,#43784,.T.) ;
#62101=ORIENTED_EDGE('',*,*,#42983,.F.) ;
#62102=ORIENTED_EDGE('',*,*,#43785,.F.) ;
#62103=ORIENTED_EDGE('',*,*,#43003,.F.) ;
#62104=ORIENTED_EDGE('',*,*,#43785,.T.) ;
#62105=ORIENTED_EDGE('',*,*,#43556,.F.) ;
#62106=ORIENTED_EDGE('',*,*,#43557,.F.) ;
#62107=ORIENTED_EDGE('',*,*,#43786,.F.) ;
#62108=ORIENTED_EDGE('',*,*,#43786,.T.) ;
#62109=ORIENTED_EDGE('',*,*,#43175,.F.) ;
#62110=ORIENTED_EDGE('',*,*,#43787,.F.) ;
#62111=ORIENTED_EDGE('',*,*,#43004,.F.) ;
#62112=ORIENTED_EDGE('',*,*,#43787,.T.) ;
#62113=ORIENTED_EDGE('',*,*,#43544,.F.) ;
#62114=ORIENTED_EDGE('',*,*,#43541,.F.) ;
#62115=ORIENTED_EDGE('',*,*,#43788,.F.) ;
#62116=ORIENTED_EDGE('',*,*,#43788,.T.) ;
#62117=ORIENTED_EDGE('',*,*,#42999,.F.) ;
#62118=ORIENTED_EDGE('',*,*,#43789,.F.) ;
#62119=ORIENTED_EDGE('',*,*,#43000,.F.) ;
#62120=ORIENTED_EDGE('',*,*,#43789,.T.) ;
#62121=ORIENTED_EDGE('',*,*,#43013,.F.) ;
#62122=ORIENTED_EDGE('',*,*,#39361,.F.) ;
#62123=ORIENTED_EDGE('',*,*,#43001,.F.) ;
#62124=ORIENTED_EDGE('',*,*,#41585,.F.) ;
#62125=ORIENTED_EDGE('',*,*,#43019,.F.) ;
#62126=ORIENTED_EDGE('',*,*,#43790,.F.) ;
#62127=ORIENTED_EDGE('',*,*,#43035,.F.) ;
#62128=ORIENTED_EDGE('',*,*,#43790,.T.) ;
#62129=ORIENTED_EDGE('',*,*,#43560,.F.) ;
#62130=ORIENTED_EDGE('',*,*,#43558,.F.) ;
#62131=ORIENTED_EDGE('',*,*,#43791,.F.) ;
#62132=ORIENTED_EDGE('',*,*,#43791,.T.) ;
#62133=ORIENTED_EDGE('',*,*,#43243,.F.) ;
#62134=ORIENTED_EDGE('',*,*,#43792,.F.) ;
#62135=ORIENTED_EDGE('',*,*,#43036,.F.) ;
#62136=ORIENTED_EDGE('',*,*,#43792,.T.) ;
#62137=ORIENTED_EDGE('',*,*,#43573,.F.) ;
#62138=ORIENTED_EDGE('',*,*,#43575,.F.) ;
#62139=ORIENTED_EDGE('',*,*,#43793,.F.) ;
#62140=ORIENTED_EDGE('',*,*,#41587,.F.) ;
#62141=ORIENTED_EDGE('',*,*,#43037,.F.) ;
#62142=ORIENTED_EDGE('',*,*,#43793,.T.) ;
#62143=ORIENTED_EDGE('',*,*,#43021,.F.) ;
#62144=ORIENTED_EDGE('',*,*,#43794,.F.) ;
#62145=ORIENTED_EDGE('',*,*,#43020,.F.) ;
#62146=ORIENTED_EDGE('',*,*,#41583,.F.) ;
#62147=ORIENTED_EDGE('',*,*,#43033,.F.) ;
#62148=ORIENTED_EDGE('',*,*,#43561,.F.) ;
#62149=ORIENTED_EDGE('',*,*,#43794,.T.) ;
#62150=ORIENTED_EDGE('',*,*,#43795,.F.) ;
#62151=ORIENTED_EDGE('',*,*,#43564,.F.) ;
#62152=ORIENTED_EDGE('',*,*,#43795,.T.) ;
#62153=ORIENTED_EDGE('',*,*,#43032,.F.) ;
#62154=ORIENTED_EDGE('',*,*,#43796,.F.) ;
#62155=ORIENTED_EDGE('',*,*,#43247,.F.) ;
#62156=ORIENTED_EDGE('',*,*,#41589,.F.) ;
#62157=ORIENTED_EDGE('',*,*,#43023,.F.) ;
#62158=ORIENTED_EDGE('',*,*,#43797,.F.) ;
#62159=ORIENTED_EDGE('',*,*,#43034,.F.) ;
#62160=ORIENTED_EDGE('',*,*,#43577,.F.) ;
#62161=ORIENTED_EDGE('',*,*,#43796,.T.) ;
#62162=ORIENTED_EDGE('',*,*,#43797,.T.) ;
#62163=ORIENTED_EDGE('',*,*,#43576,.F.) ;
#62164=ORIENTED_EDGE('',*,*,#39352,.F.) ;
#62165=ORIENTED_EDGE('',*,*,#43070,.F.) ;
#62166=ORIENTED_EDGE('',*,*,#43798,.F.) ;
#62167=ORIENTED_EDGE('',*,*,#43065,.F.) ;
#62168=ORIENTED_EDGE('',*,*,#43798,.T.) ;
#62169=ORIENTED_EDGE('',*,*,#43055,.F.) ;
#62170=ORIENTED_EDGE('',*,*,#43799,.F.) ;
#62171=ORIENTED_EDGE('',*,*,#43066,.F.) ;
#62172=ORIENTED_EDGE('',*,*,#43799,.T.) ;
#62173=ORIENTED_EDGE('',*,*,#43580,.F.) ;
#62174=ORIENTED_EDGE('',*,*,#43578,.F.) ;
#62175=ORIENTED_EDGE('',*,*,#43800,.F.) ;
#62176=ORIENTED_EDGE('',*,*,#43800,.T.) ;
#62177=ORIENTED_EDGE('',*,*,#43163,.F.) ;
#62178=ORIENTED_EDGE('',*,*,#43801,.F.) ;
#62179=ORIENTED_EDGE('',*,*,#43067,.F.) ;
#62180=ORIENTED_EDGE('',*,*,#43801,.T.) ;
#62181=ORIENTED_EDGE('',*,*,#43593,.F.) ;
#62182=ORIENTED_EDGE('',*,*,#43595,.F.) ;
#62183=ORIENTED_EDGE('',*,*,#43802,.F.) ;
#62184=ORIENTED_EDGE('',*,*,#43802,.T.) ;
#62185=ORIENTED_EDGE('',*,*,#43039,.F.) ;
#62186=ORIENTED_EDGE('',*,*,#43803,.F.) ;
#62187=ORIENTED_EDGE('',*,*,#43063,.F.) ;
#62188=ORIENTED_EDGE('',*,*,#39121,.F.) ;
#62189=ORIENTED_EDGE('',*,*,#43064,.F.) ;
#62190=ORIENTED_EDGE('',*,*,#43803,.T.) ;
#62191=ORIENTED_EDGE('',*,*,#43068,.F.) ;
#62192=ORIENTED_EDGE('',*,*,#42466,.F.) ;
#62193=ORIENTED_EDGE('',*,*,#42469,.F.) ;
#62194=ORIENTED_EDGE('',*,*,#43069,.F.) ;
#62195=ORIENTED_EDGE('',*,*,#43804,.F.) ;
#62196=ORIENTED_EDGE('',*,*,#43060,.F.) ;
#62197=ORIENTED_EDGE('',*,*,#43804,.T.) ;
#62198=ORIENTED_EDGE('',*,*,#43041,.F.) ;
#62199=ORIENTED_EDGE('',*,*,#43805,.F.) ;
#62200=ORIENTED_EDGE('',*,*,#43061,.F.) ;
#62201=ORIENTED_EDGE('',*,*,#43805,.T.) ;
#62202=ORIENTED_EDGE('',*,*,#43596,.F.) ;
#62203=ORIENTED_EDGE('',*,*,#43597,.F.) ;
#62204=ORIENTED_EDGE('',*,*,#43806,.F.) ;
#62205=ORIENTED_EDGE('',*,*,#43806,.T.) ;
#62206=ORIENTED_EDGE('',*,*,#43167,.F.) ;
#62207=ORIENTED_EDGE('',*,*,#43807,.F.) ;
#62208=ORIENTED_EDGE('',*,*,#43062,.F.) ;
#62209=ORIENTED_EDGE('',*,*,#43807,.T.) ;
#62210=ORIENTED_EDGE('',*,*,#43584,.F.) ;
#62211=ORIENTED_EDGE('',*,*,#43581,.F.) ;
#62212=ORIENTED_EDGE('',*,*,#43808,.F.) ;
#62213=ORIENTED_EDGE('',*,*,#43808,.T.) ;
#62214=ORIENTED_EDGE('',*,*,#43057,.F.) ;
#62215=ORIENTED_EDGE('',*,*,#43809,.F.) ;
#62216=ORIENTED_EDGE('',*,*,#43058,.F.) ;
#62217=ORIENTED_EDGE('',*,*,#43809,.T.) ;
#62218=ORIENTED_EDGE('',*,*,#43071,.F.) ;
#62219=ORIENTED_EDGE('',*,*,#39350,.F.) ;
#62220=ORIENTED_EDGE('',*,*,#43059,.F.) ;
#62221=ORIENTED_EDGE('',*,*,#41593,.F.) ;
#62222=ORIENTED_EDGE('',*,*,#43077,.F.) ;
#62223=ORIENTED_EDGE('',*,*,#43810,.F.) ;
#62224=ORIENTED_EDGE('',*,*,#43093,.F.) ;
#62225=ORIENTED_EDGE('',*,*,#43810,.T.) ;
#62226=ORIENTED_EDGE('',*,*,#43600,.F.) ;
#62227=ORIENTED_EDGE('',*,*,#43598,.F.) ;
#62228=ORIENTED_EDGE('',*,*,#43811,.F.) ;
#62229=ORIENTED_EDGE('',*,*,#43811,.T.) ;
#62230=ORIENTED_EDGE('',*,*,#43235,.F.) ;
#62231=ORIENTED_EDGE('',*,*,#43812,.F.) ;
#62232=ORIENTED_EDGE('',*,*,#43094,.F.) ;
#62233=ORIENTED_EDGE('',*,*,#43812,.T.) ;
#62234=ORIENTED_EDGE('',*,*,#43613,.F.) ;
#62235=ORIENTED_EDGE('',*,*,#43615,.F.) ;
#62236=ORIENTED_EDGE('',*,*,#43813,.F.) ;
#62237=ORIENTED_EDGE('',*,*,#41595,.F.) ;
#62238=ORIENTED_EDGE('',*,*,#43095,.F.) ;
#62239=ORIENTED_EDGE('',*,*,#43813,.T.) ;
#62240=ORIENTED_EDGE('',*,*,#43079,.F.) ;
#62241=ORIENTED_EDGE('',*,*,#43814,.F.) ;
#62242=ORIENTED_EDGE('',*,*,#43078,.F.) ;
#62243=ORIENTED_EDGE('',*,*,#41591,.F.) ;
#62244=ORIENTED_EDGE('',*,*,#43091,.F.) ;
#62245=ORIENTED_EDGE('',*,*,#43601,.F.) ;
#62246=ORIENTED_EDGE('',*,*,#43814,.T.) ;
#62247=ORIENTED_EDGE('',*,*,#43815,.F.) ;
#62248=ORIENTED_EDGE('',*,*,#43604,.F.) ;
#62249=ORIENTED_EDGE('',*,*,#43815,.T.) ;
#62250=ORIENTED_EDGE('',*,*,#43090,.F.) ;
#62251=ORIENTED_EDGE('',*,*,#43816,.F.) ;
#62252=ORIENTED_EDGE('',*,*,#43239,.F.) ;
#62253=ORIENTED_EDGE('',*,*,#41597,.F.) ;
#62254=ORIENTED_EDGE('',*,*,#43081,.F.) ;
#62255=ORIENTED_EDGE('',*,*,#43817,.F.) ;
#62256=ORIENTED_EDGE('',*,*,#43092,.F.) ;
#62257=ORIENTED_EDGE('',*,*,#43617,.F.) ;
#62258=ORIENTED_EDGE('',*,*,#43816,.T.) ;
#62259=ORIENTED_EDGE('',*,*,#43817,.T.) ;
#62260=ORIENTED_EDGE('',*,*,#43616,.F.) ;
#62261=ORIENTED_EDGE('',*,*,#39341,.F.) ;
#62262=ORIENTED_EDGE('',*,*,#43128,.F.) ;
#62263=ORIENTED_EDGE('',*,*,#43818,.F.) ;
#62264=ORIENTED_EDGE('',*,*,#43123,.F.) ;
#62265=ORIENTED_EDGE('',*,*,#43818,.T.) ;
#62266=ORIENTED_EDGE('',*,*,#43113,.F.) ;
#62267=ORIENTED_EDGE('',*,*,#43819,.F.) ;
#62268=ORIENTED_EDGE('',*,*,#43124,.F.) ;
#62269=ORIENTED_EDGE('',*,*,#43819,.T.) ;
#62270=ORIENTED_EDGE('',*,*,#43620,.F.) ;
#62271=ORIENTED_EDGE('',*,*,#43618,.F.) ;
#62272=ORIENTED_EDGE('',*,*,#43820,.F.) ;
#62273=ORIENTED_EDGE('',*,*,#43820,.T.) ;
#62274=ORIENTED_EDGE('',*,*,#43155,.F.) ;
#62275=ORIENTED_EDGE('',*,*,#43821,.F.) ;
#62276=ORIENTED_EDGE('',*,*,#43125,.F.) ;
#62277=ORIENTED_EDGE('',*,*,#43821,.T.) ;
#62278=ORIENTED_EDGE('',*,*,#43633,.F.) ;
#62279=ORIENTED_EDGE('',*,*,#43635,.F.) ;
#62280=ORIENTED_EDGE('',*,*,#43822,.F.) ;
#62281=ORIENTED_EDGE('',*,*,#43822,.T.) ;
#62282=ORIENTED_EDGE('',*,*,#43097,.F.) ;
#62283=ORIENTED_EDGE('',*,*,#43823,.F.) ;
#62284=ORIENTED_EDGE('',*,*,#43121,.F.) ;
#62285=ORIENTED_EDGE('',*,*,#39104,.F.) ;
#62286=ORIENTED_EDGE('',*,*,#43122,.F.) ;
#62287=ORIENTED_EDGE('',*,*,#43823,.T.) ;
#62288=ORIENTED_EDGE('',*,*,#43126,.F.) ;
#62289=ORIENTED_EDGE('',*,*,#42554,.F.) ;
#62290=ORIENTED_EDGE('',*,*,#42557,.F.) ;
#62291=ORIENTED_EDGE('',*,*,#43127,.F.) ;
#62292=ORIENTED_EDGE('',*,*,#43824,.F.) ;
#62293=ORIENTED_EDGE('',*,*,#43118,.F.) ;
#62294=ORIENTED_EDGE('',*,*,#43824,.T.) ;
#62295=ORIENTED_EDGE('',*,*,#43099,.F.) ;
#62296=ORIENTED_EDGE('',*,*,#43825,.F.) ;
#62297=ORIENTED_EDGE('',*,*,#43119,.F.) ;
#62298=ORIENTED_EDGE('',*,*,#43825,.T.) ;
#62299=ORIENTED_EDGE('',*,*,#43636,.F.) ;
#62300=ORIENTED_EDGE('',*,*,#43637,.F.) ;
#62301=ORIENTED_EDGE('',*,*,#43826,.F.) ;
#62302=ORIENTED_EDGE('',*,*,#43826,.T.) ;
#62303=ORIENTED_EDGE('',*,*,#43159,.F.) ;
#62304=ORIENTED_EDGE('',*,*,#43827,.F.) ;
#62305=ORIENTED_EDGE('',*,*,#43120,.F.) ;
#62306=ORIENTED_EDGE('',*,*,#43827,.T.) ;
#62307=ORIENTED_EDGE('',*,*,#43624,.F.) ;
#62308=ORIENTED_EDGE('',*,*,#43621,.F.) ;
#62309=ORIENTED_EDGE('',*,*,#43828,.F.) ;
#62310=ORIENTED_EDGE('',*,*,#43828,.T.) ;
#62311=ORIENTED_EDGE('',*,*,#43115,.F.) ;
#62312=ORIENTED_EDGE('',*,*,#43829,.F.) ;
#62313=ORIENTED_EDGE('',*,*,#43116,.F.) ;
#62314=ORIENTED_EDGE('',*,*,#43829,.T.) ;
#62315=ORIENTED_EDGE('',*,*,#43129,.F.) ;
#62316=ORIENTED_EDGE('',*,*,#39339,.F.) ;
#62317=ORIENTED_EDGE('',*,*,#43117,.F.) ;
#62318=ORIENTED_EDGE('',*,*,#41601,.F.) ;
#62319=ORIENTED_EDGE('',*,*,#43135,.F.) ;
#62320=ORIENTED_EDGE('',*,*,#43830,.F.) ;
#62321=ORIENTED_EDGE('',*,*,#43151,.F.) ;
#62322=ORIENTED_EDGE('',*,*,#43830,.T.) ;
#62323=ORIENTED_EDGE('',*,*,#43640,.F.) ;
#62324=ORIENTED_EDGE('',*,*,#43638,.F.) ;
#62325=ORIENTED_EDGE('',*,*,#43831,.F.) ;
#62326=ORIENTED_EDGE('',*,*,#43831,.T.) ;
#62327=ORIENTED_EDGE('',*,*,#43227,.F.) ;
#62328=ORIENTED_EDGE('',*,*,#43832,.F.) ;
#62329=ORIENTED_EDGE('',*,*,#43152,.F.) ;
#62330=ORIENTED_EDGE('',*,*,#43832,.T.) ;
#62331=ORIENTED_EDGE('',*,*,#43653,.F.) ;
#62332=ORIENTED_EDGE('',*,*,#43655,.F.) ;
#62333=ORIENTED_EDGE('',*,*,#43833,.F.) ;
#62334=ORIENTED_EDGE('',*,*,#41603,.F.) ;
#62335=ORIENTED_EDGE('',*,*,#43153,.F.) ;
#62336=ORIENTED_EDGE('',*,*,#43833,.T.) ;
#62337=ORIENTED_EDGE('',*,*,#43137,.F.) ;
#62338=ORIENTED_EDGE('',*,*,#43834,.F.) ;
#62339=ORIENTED_EDGE('',*,*,#43136,.F.) ;
#62340=ORIENTED_EDGE('',*,*,#41599,.F.) ;
#62341=ORIENTED_EDGE('',*,*,#43149,.F.) ;
#62342=ORIENTED_EDGE('',*,*,#43641,.F.) ;
#62343=ORIENTED_EDGE('',*,*,#43834,.T.) ;
#62344=ORIENTED_EDGE('',*,*,#43835,.F.) ;
#62345=ORIENTED_EDGE('',*,*,#43644,.F.) ;
#62346=ORIENTED_EDGE('',*,*,#43835,.T.) ;
#62347=ORIENTED_EDGE('',*,*,#43148,.F.) ;
#62348=ORIENTED_EDGE('',*,*,#43836,.F.) ;
#62349=ORIENTED_EDGE('',*,*,#43231,.F.) ;
#62350=ORIENTED_EDGE('',*,*,#41605,.F.) ;
#62351=ORIENTED_EDGE('',*,*,#43139,.F.) ;
#62352=ORIENTED_EDGE('',*,*,#43837,.F.) ;
#62353=ORIENTED_EDGE('',*,*,#43150,.F.) ;
#62354=ORIENTED_EDGE('',*,*,#43657,.F.) ;
#62355=ORIENTED_EDGE('',*,*,#43836,.T.) ;
#62356=ORIENTED_EDGE('',*,*,#43837,.T.) ;
#62357=ORIENTED_EDGE('',*,*,#43656,.F.) ;
#63117=TOROIDAL_SURFACE('',#71867,0.9,0.1) ;
#63118=TOROIDAL_SURFACE('',#71872,1.1,0.1) ;
#63119=TOROIDAL_SURFACE('',#71884,0.9,0.1) ;
#63120=TOROIDAL_SURFACE('',#71889,1.1,0.1) ;
#63121=TOROIDAL_SURFACE('',#71901,0.9,0.1) ;
#63122=TOROIDAL_SURFACE('',#71906,1.1,0.1) ;
#63123=TOROIDAL_SURFACE('',#71918,0.9,0.1) ;
#63124=TOROIDAL_SURFACE('',#71923,1.1,0.1) ;
#63125=TOROIDAL_SURFACE('',#71935,0.9,0.1) ;
#63126=TOROIDAL_SURFACE('',#71940,1.1,0.1) ;
#63127=TOROIDAL_SURFACE('',#71952,0.9,0.1) ;
#63128=TOROIDAL_SURFACE('',#71957,1.1,0.1) ;
#63129=TOROIDAL_SURFACE('',#71969,0.9,0.1) ;
#63130=TOROIDAL_SURFACE('',#71974,1.1,0.1) ;
#63131=TOROIDAL_SURFACE('',#71986,0.9,0.1) ;
#63132=TOROIDAL_SURFACE('',#71991,1.1,0.1) ;
#63133=TOROIDAL_SURFACE('',#72003,0.9,0.1) ;
#63134=TOROIDAL_SURFACE('',#72008,0.2,0.1) ;
#63135=TOROIDAL_SURFACE('',#72013,0.2,0.1) ;
#63136=TOROIDAL_SURFACE('',#72018,0.2,0.1) ;
#63137=TOROIDAL_SURFACE('',#72023,0.2,0.1) ;
#63138=TOROIDAL_SURFACE('',#72028,0.2,0.1) ;
#63139=TOROIDAL_SURFACE('',#72033,0.2,0.1) ;
#63140=TOROIDAL_SURFACE('',#72038,0.2,0.1) ;
#63141=TOROIDAL_SURFACE('',#72043,0.2,0.1) ;
#63142=TOROIDAL_SURFACE('',#72048,0.2,0.1) ;
#63143=TOROIDAL_SURFACE('',#72053,1.1,0.1) ;
#63144=TOROIDAL_SURFACE('',#72092,0.9,0.1) ;
#63145=TOROIDAL_SURFACE('',#72097,0.2,0.1) ;
#63146=TOROIDAL_SURFACE('',#72102,1.1,0.1) ;
#63147=TOROIDAL_SURFACE('',#72500,0.2,0.1) ;
#63148=TOROIDAL_SURFACE('',#72516,0.2,0.1) ;
#63149=TOROIDAL_SURFACE('',#72518,0.2,0.1) ;
#63150=TOROIDAL_SURFACE('',#72521,0.2,0.1) ;
#63151=TOROIDAL_SURFACE('',#72534,0.2,0.1) ;
#63152=TOROIDAL_SURFACE('',#72554,0.2,0.1) ;
#63153=TOROIDAL_SURFACE('',#72565,0.2,0.1) ;
#63154=TOROIDAL_SURFACE('',#72572,0.2,0.1) ;
#63155=TOROIDAL_SURFACE('',#72578,0.2,0.1) ;
#63156=TOROIDAL_SURFACE('',#72581,0.2,0.1) ;
#63157=TOROIDAL_SURFACE('',#72595,0.2,0.1) ;
#63158=TOROIDAL_SURFACE('',#72605,0.2,0.1) ;
#63159=TOROIDAL_SURFACE('',#72627,0.2,0.1) ;
#63160=TOROIDAL_SURFACE('',#72637,0.2,0.1) ;
#63161=TOROIDAL_SURFACE('',#72655,0.2,0.1) ;
#63162=TOROIDAL_SURFACE('',#72663,0.2,0.1) ;
#63163=TOROIDAL_SURFACE('',#72677,1.75625,0.1) ;
#63164=TOROIDAL_SURFACE('',#72700,0.2,0.1) ;
#63165=TOROIDAL_SURFACE('',#72702,0.2,0.1) ;
#63166=TOROIDAL_SURFACE('',#72716,0.2,0.1) ;
#63167=TOROIDAL_SURFACE('',#72718,0.2,0.1) ;
#63168=TOROIDAL_SURFACE('',#72723,0.2,0.1) ;
#63169=TOROIDAL_SURFACE('',#72729,0.2,0.1) ;
#63170=TOROIDAL_SURFACE('',#72731,0.2,0.1) ;
#63171=TOROIDAL_SURFACE('',#72735,1.55625,0.1) ;
#63172=TOROIDAL_SURFACE('',#72737,0.199999999999999,0.1) ;
#63173=TOROIDAL_SURFACE('',#72739,0.2,0.1) ;
#63174=TOROIDAL_SURFACE('',#72747,0.2,0.1) ;
#63175=TOROIDAL_SURFACE('',#72755,0.2,0.1) ;
#63176=TOROIDAL_SURFACE('',#72854,0.3,0.1) ;
#63177=TOROIDAL_SURFACE('',#72866,0.9,0.1) ;
#63178=TOROIDAL_SURFACE('',#72867,0.9,0.1) ;
#63179=TOROIDAL_SURFACE('',#72879,0.3,0.1) ;
#63180=TOROIDAL_SURFACE('',#73567,0.2,0.1) ;
#63181=TOROIDAL_SURFACE('',#73583,0.2,0.1) ;
#63182=TOROIDAL_SURFACE('',#73585,0.2,0.1) ;
#63183=TOROIDAL_SURFACE('',#73588,0.2,0.1) ;
#63184=TOROIDAL_SURFACE('',#73601,0.2,0.1) ;
#63185=TOROIDAL_SURFACE('',#73621,0.2,0.1) ;
#63186=TOROIDAL_SURFACE('',#73632,0.2,0.1) ;
#63187=TOROIDAL_SURFACE('',#73639,0.2,0.1) ;
#63188=TOROIDAL_SURFACE('',#73645,0.2,0.1) ;
#63189=TOROIDAL_SURFACE('',#73648,0.2,0.1) ;
#63190=TOROIDAL_SURFACE('',#73658,0.2,0.1) ;
#63191=TOROIDAL_SURFACE('',#73666,0.2,0.1) ;
#63192=TOROIDAL_SURFACE('',#73680,1.75625,0.1) ;
#63193=TOROIDAL_SURFACE('',#73703,0.2,0.1) ;
#63194=TOROIDAL_SURFACE('',#73705,0.2,0.1) ;
#63195=TOROIDAL_SURFACE('',#73719,0.2,0.1) ;
#63196=TOROIDAL_SURFACE('',#73721,0.2,0.1) ;
#63197=TOROIDAL_SURFACE('',#73726,0.2,0.1) ;
#63198=TOROIDAL_SURFACE('',#73732,0.2,0.1) ;
#63199=TOROIDAL_SURFACE('',#73734,0.2,0.1) ;
#63200=TOROIDAL_SURFACE('',#73738,1.55625,0.1) ;
#63201=TOROIDAL_SURFACE('',#73740,0.199999999999999,0.1) ;
#63202=TOROIDAL_SURFACE('',#73742,0.2,0.1) ;
#63203=TOROIDAL_SURFACE('',#73750,0.2,0.1) ;
#63204=TOROIDAL_SURFACE('',#73758,0.2,0.1) ;
#63205=TOROIDAL_SURFACE('',#73772,0.2,0.1) ;
#63206=TOROIDAL_SURFACE('',#73774,0.2,0.1) ;
#63207=TOROIDAL_SURFACE('',#73779,0.2,0.1) ;
#63208=TOROIDAL_SURFACE('',#73785,0.2,0.1) ;
#63209=TOROIDAL_SURFACE('',#73787,0.2,0.1) ;
#63210=TOROIDAL_SURFACE('',#73791,1.55625,0.1) ;
#63211=TOROIDAL_SURFACE('',#73793,0.199999999999999,0.1) ;
#63212=TOROIDAL_SURFACE('',#73795,0.2,0.1) ;
#63213=TOROIDAL_SURFACE('',#73803,0.2,0.1) ;
#63214=TOROIDAL_SURFACE('',#73811,0.2,0.1) ;
#63215=TOROIDAL_SURFACE('',#73825,0.2,0.1) ;
#63216=TOROIDAL_SURFACE('',#73827,0.2,0.1) ;
#63217=TOROIDAL_SURFACE('',#73832,0.2,0.1) ;
#63218=TOROIDAL_SURFACE('',#73838,0.2,0.1) ;
#63219=TOROIDAL_SURFACE('',#73840,0.2,0.1) ;
#63220=TOROIDAL_SURFACE('',#73844,1.55625,0.1) ;
#63221=TOROIDAL_SURFACE('',#73846,0.199999999999999,0.1) ;
#63222=TOROIDAL_SURFACE('',#73848,0.2,0.1) ;
#63223=TOROIDAL_SURFACE('',#73856,0.2,0.1) ;
#63224=TOROIDAL_SURFACE('',#73864,0.2,0.1) ;
#63225=TOROIDAL_SURFACE('',#73878,0.2,0.1) ;
#63226=TOROIDAL_SURFACE('',#73880,0.2,0.1) ;
#63227=TOROIDAL_SURFACE('',#73885,0.2,0.1) ;
#63228=TOROIDAL_SURFACE('',#73891,0.2,0.1) ;
#63229=TOROIDAL_SURFACE('',#73893,0.2,0.1) ;
#63230=TOROIDAL_SURFACE('',#73897,1.55625,0.1) ;
#63231=TOROIDAL_SURFACE('',#73899,0.199999999999999,0.1) ;
#63232=TOROIDAL_SURFACE('',#73901,0.2,0.1) ;
#63233=TOROIDAL_SURFACE('',#73909,0.2,0.1) ;
#63234=TOROIDAL_SURFACE('',#73917,0.2,0.1) ;
#63235=TOROIDAL_SURFACE('',#73931,0.2,0.1) ;
#63236=TOROIDAL_SURFACE('',#73933,0.2,0.1) ;
#63237=TOROIDAL_SURFACE('',#73938,0.2,0.1) ;
#63238=TOROIDAL_SURFACE('',#73944,0.2,0.1) ;
#63239=TOROIDAL_SURFACE('',#73946,0.2,0.1) ;
#63240=TOROIDAL_SURFACE('',#73950,1.55625,0.1) ;
#63241=TOROIDAL_SURFACE('',#73952,0.199999999999999,0.1) ;
#63242=TOROIDAL_SURFACE('',#73954,0.2,0.1) ;
#63243=TOROIDAL_SURFACE('',#73962,0.2,0.1) ;
#63244=TOROIDAL_SURFACE('',#73970,0.2,0.1) ;
#63245=TOROIDAL_SURFACE('',#73984,0.2,0.1) ;
#63246=TOROIDAL_SURFACE('',#73986,0.2,0.1) ;
#63247=TOROIDAL_SURFACE('',#73991,0.2,0.1) ;
#63248=TOROIDAL_SURFACE('',#73997,0.2,0.1) ;
#63249=TOROIDAL_SURFACE('',#73999,0.2,0.1) ;
#63250=TOROIDAL_SURFACE('',#74003,1.55625,0.1) ;
#63251=TOROIDAL_SURFACE('',#74005,0.199999999999999,0.1) ;
#63252=TOROIDAL_SURFACE('',#74007,0.2,0.1) ;
#63253=TOROIDAL_SURFACE('',#74015,0.2,0.1) ;
#63254=TOROIDAL_SURFACE('',#74023,0.2,0.1) ;
#63255=TOROIDAL_SURFACE('',#74037,0.2,0.1) ;
#63256=TOROIDAL_SURFACE('',#74039,0.2,0.1) ;
#63257=TOROIDAL_SURFACE('',#74044,0.2,0.1) ;
#63258=TOROIDAL_SURFACE('',#74050,0.2,0.1) ;
#63259=TOROIDAL_SURFACE('',#74052,0.2,0.1) ;
#63260=TOROIDAL_SURFACE('',#74056,1.55625,0.1) ;
#63261=TOROIDAL_SURFACE('',#74058,0.199999999999999,0.1) ;
#63262=TOROIDAL_SURFACE('',#74060,0.2,0.1) ;
#63263=TOROIDAL_SURFACE('',#74068,0.2,0.1) ;
#63264=TOROIDAL_SURFACE('',#74076,0.2,0.1) ;
#63265=TOROIDAL_SURFACE('',#74090,0.2,0.1) ;
#63266=TOROIDAL_SURFACE('',#74092,0.2,0.1) ;
#63267=TOROIDAL_SURFACE('',#74097,0.2,0.1) ;
#63268=TOROIDAL_SURFACE('',#74103,0.2,0.1) ;
#63269=TOROIDAL_SURFACE('',#74105,0.2,0.1) ;
#63270=TOROIDAL_SURFACE('',#74109,1.55625,0.1) ;
#63271=TOROIDAL_SURFACE('',#74111,0.199999999999999,0.1) ;
#63272=TOROIDAL_SURFACE('',#74113,0.2,0.1) ;
#63273=TOROIDAL_SURFACE('',#74121,0.2,0.1) ;
#63274=TOROIDAL_SURFACE('',#74129,0.2,0.1) ;
#63275=TOROIDAL_SURFACE('',#74143,0.2,0.1) ;
#63276=TOROIDAL_SURFACE('',#74145,0.2,0.1) ;
#63277=TOROIDAL_SURFACE('',#74150,0.2,0.1) ;
#63278=TOROIDAL_SURFACE('',#74156,0.2,0.1) ;
#63279=TOROIDAL_SURFACE('',#74158,0.2,0.1) ;
#63280=TOROIDAL_SURFACE('',#74162,1.55625,0.1) ;
#63281=TOROIDAL_SURFACE('',#74164,0.199999999999999,0.1) ;
#63282=TOROIDAL_SURFACE('',#74166,0.2,0.1) ;
#63283=TOROIDAL_SURFACE('',#74174,0.2,0.1) ;
#63284=TOROIDAL_SURFACE('',#74182,0.2,0.1) ;
#63285=TOROIDAL_SURFACE('',#74197,0.2,0.1) ;
#63286=TOROIDAL_SURFACE('',#74213,0.2,0.1) ;
#63287=TOROIDAL_SURFACE('',#74215,0.2,0.1) ;
#63288=TOROIDAL_SURFACE('',#74218,0.2,0.1) ;
#63289=TOROIDAL_SURFACE('',#74231,0.2,0.1) ;
#63290=TOROIDAL_SURFACE('',#74251,0.2,0.1) ;
#63291=TOROIDAL_SURFACE('',#74262,0.2,0.1) ;
#63292=TOROIDAL_SURFACE('',#74269,0.2,0.1) ;
#63293=TOROIDAL_SURFACE('',#74275,0.2,0.1) ;
#63294=TOROIDAL_SURFACE('',#74278,0.2,0.1) ;
#63295=TOROIDAL_SURFACE('',#74288,0.2,0.1) ;
#63296=TOROIDAL_SURFACE('',#74296,0.2,0.1) ;
#63297=TOROIDAL_SURFACE('',#74310,1.75625,0.1) ;
#63298=TOROIDAL_SURFACE('',#74333,0.2,0.1) ;
#63299=TOROIDAL_SURFACE('',#74335,0.2,0.1) ;
#63300=TOROIDAL_SURFACE('',#74350,0.2,0.1) ;
#63301=TOROIDAL_SURFACE('',#74366,0.2,0.1) ;
#63302=TOROIDAL_SURFACE('',#74368,0.2,0.1) ;
#63303=TOROIDAL_SURFACE('',#74371,0.2,0.1) ;
#63304=TOROIDAL_SURFACE('',#74384,0.2,0.1) ;
#63305=TOROIDAL_SURFACE('',#74404,0.2,0.1) ;
#63306=TOROIDAL_SURFACE('',#74415,0.2,0.1) ;
#63307=TOROIDAL_SURFACE('',#74422,0.2,0.1) ;
#63308=TOROIDAL_SURFACE('',#74428,0.2,0.1) ;
#63309=TOROIDAL_SURFACE('',#74431,0.2,0.1) ;
#63310=TOROIDAL_SURFACE('',#74441,0.2,0.1) ;
#63311=TOROIDAL_SURFACE('',#74449,0.2,0.1) ;
#63312=TOROIDAL_SURFACE('',#74463,1.75625,0.1) ;
#63313=TOROIDAL_SURFACE('',#74486,0.2,0.1) ;
#63314=TOROIDAL_SURFACE('',#74488,0.2,0.1) ;
#63315=TOROIDAL_SURFACE('',#74503,0.2,0.1) ;
#63316=TOROIDAL_SURFACE('',#74519,0.2,0.1) ;
#63317=TOROIDAL_SURFACE('',#74521,0.2,0.1) ;
#63318=TOROIDAL_SURFACE('',#74524,0.2,0.1) ;
#63319=TOROIDAL_SURFACE('',#74537,0.2,0.1) ;
#63320=TOROIDAL_SURFACE('',#74557,0.2,0.1) ;
#63321=TOROIDAL_SURFACE('',#74568,0.2,0.1) ;
#63322=TOROIDAL_SURFACE('',#74575,0.2,0.1) ;
#63323=TOROIDAL_SURFACE('',#74581,0.2,0.1) ;
#63324=TOROIDAL_SURFACE('',#74584,0.2,0.1) ;
#63325=TOROIDAL_SURFACE('',#74594,0.2,0.1) ;
#63326=TOROIDAL_SURFACE('',#74602,0.2,0.1) ;
#63327=TOROIDAL_SURFACE('',#74616,1.75625,0.1) ;
#63328=TOROIDAL_SURFACE('',#74639,0.2,0.1) ;
#63329=TOROIDAL_SURFACE('',#74641,0.2,0.1) ;
#63330=TOROIDAL_SURFACE('',#74656,0.2,0.1) ;
#63331=TOROIDAL_SURFACE('',#74672,0.2,0.1) ;
#63332=TOROIDAL_SURFACE('',#74674,0.2,0.1) ;
#63333=TOROIDAL_SURFACE('',#74677,0.2,0.1) ;
#63334=TOROIDAL_SURFACE('',#74690,0.2,0.1) ;
#63335=TOROIDAL_SURFACE('',#74710,0.2,0.1) ;
#63336=TOROIDAL_SURFACE('',#74721,0.2,0.1) ;
#63337=TOROIDAL_SURFACE('',#74728,0.2,0.1) ;
#63338=TOROIDAL_SURFACE('',#74734,0.2,0.1) ;
#63339=TOROIDAL_SURFACE('',#74737,0.2,0.1) ;
#63340=TOROIDAL_SURFACE('',#74747,0.2,0.1) ;
#63341=TOROIDAL_SURFACE('',#74755,0.2,0.1) ;
#63342=TOROIDAL_SURFACE('',#74769,1.75625,0.1) ;
#63343=TOROIDAL_SURFACE('',#74792,0.2,0.1) ;
#63344=TOROIDAL_SURFACE('',#74794,0.2,0.1) ;
#63345=TOROIDAL_SURFACE('',#74809,0.2,0.1) ;
#63346=TOROIDAL_SURFACE('',#74825,0.2,0.1) ;
#63347=TOROIDAL_SURFACE('',#74827,0.2,0.1) ;
#63348=TOROIDAL_SURFACE('',#74830,0.2,0.1) ;
#63349=TOROIDAL_SURFACE('',#74843,0.2,0.1) ;
#63350=TOROIDAL_SURFACE('',#74863,0.2,0.1) ;
#63351=TOROIDAL_SURFACE('',#74874,0.2,0.1) ;
#63352=TOROIDAL_SURFACE('',#74881,0.2,0.1) ;
#63353=TOROIDAL_SURFACE('',#74887,0.2,0.1) ;
#63354=TOROIDAL_SURFACE('',#74890,0.2,0.1) ;
#63355=TOROIDAL_SURFACE('',#74900,0.2,0.1) ;
#63356=TOROIDAL_SURFACE('',#74908,0.2,0.1) ;
#63357=TOROIDAL_SURFACE('',#74922,1.75625,0.1) ;
#63358=TOROIDAL_SURFACE('',#74945,0.2,0.1) ;
#63359=TOROIDAL_SURFACE('',#74947,0.2,0.1) ;
#63360=TOROIDAL_SURFACE('',#74962,0.2,0.1) ;
#63361=TOROIDAL_SURFACE('',#74978,0.2,0.1) ;
#63362=TOROIDAL_SURFACE('',#74980,0.2,0.1) ;
#63363=TOROIDAL_SURFACE('',#74983,0.2,0.1) ;
#63364=TOROIDAL_SURFACE('',#74996,0.2,0.1) ;
#63365=TOROIDAL_SURFACE('',#75016,0.2,0.1) ;
#63366=TOROIDAL_SURFACE('',#75027,0.2,0.1) ;
#63367=TOROIDAL_SURFACE('',#75034,0.2,0.1) ;
#63368=TOROIDAL_SURFACE('',#75040,0.2,0.1) ;
#63369=TOROIDAL_SURFACE('',#75043,0.2,0.1) ;
#63370=TOROIDAL_SURFACE('',#75053,0.2,0.1) ;
#63371=TOROIDAL_SURFACE('',#75061,0.2,0.1) ;
#63372=TOROIDAL_SURFACE('',#75075,1.75625,0.1) ;
#63373=TOROIDAL_SURFACE('',#75098,0.2,0.1) ;
#63374=TOROIDAL_SURFACE('',#75100,0.2,0.1) ;
#63375=TOROIDAL_SURFACE('',#75115,0.2,0.1) ;
#63376=TOROIDAL_SURFACE('',#75131,0.2,0.1) ;
#63377=TOROIDAL_SURFACE('',#75133,0.2,0.1) ;
#63378=TOROIDAL_SURFACE('',#75136,0.2,0.1) ;
#63379=TOROIDAL_SURFACE('',#75149,0.2,0.1) ;
#63380=TOROIDAL_SURFACE('',#75169,0.2,0.1) ;
#63381=TOROIDAL_SURFACE('',#75180,0.2,0.1) ;
#63382=TOROIDAL_SURFACE('',#75187,0.2,0.1) ;
#63383=TOROIDAL_SURFACE('',#75193,0.2,0.1) ;
#63384=TOROIDAL_SURFACE('',#75196,0.2,0.1) ;
#63385=TOROIDAL_SURFACE('',#75206,0.2,0.1) ;
#63386=TOROIDAL_SURFACE('',#75214,0.2,0.1) ;
#63387=TOROIDAL_SURFACE('',#75228,1.75625,0.1) ;
#63388=TOROIDAL_SURFACE('',#75251,0.2,0.1) ;
#63389=TOROIDAL_SURFACE('',#75253,0.2,0.1) ;
#63390=TOROIDAL_SURFACE('',#75268,0.2,0.1) ;
#63391=TOROIDAL_SURFACE('',#75284,0.2,0.1) ;
#63392=TOROIDAL_SURFACE('',#75286,0.2,0.1) ;
#63393=TOROIDAL_SURFACE('',#75289,0.2,0.1) ;
#63394=TOROIDAL_SURFACE('',#75302,0.2,0.1) ;
#63395=TOROIDAL_SURFACE('',#75322,0.2,0.1) ;
#63396=TOROIDAL_SURFACE('',#75333,0.2,0.1) ;
#63397=TOROIDAL_SURFACE('',#75340,0.2,0.1) ;
#63398=TOROIDAL_SURFACE('',#75346,0.2,0.1) ;
#63399=TOROIDAL_SURFACE('',#75349,0.2,0.1) ;
#63400=TOROIDAL_SURFACE('',#75359,0.2,0.1) ;
#63401=TOROIDAL_SURFACE('',#75367,0.2,0.1) ;
#63402=TOROIDAL_SURFACE('',#75381,1.75625,0.1) ;
#63403=TOROIDAL_SURFACE('',#75404,0.2,0.1) ;
#63404=TOROIDAL_SURFACE('',#75406,0.2,0.1) ;
#63405=TOROIDAL_SURFACE('',#76273,0.3,0.1) ;
#63406=TOROIDAL_SURFACE('',#76285,0.9,0.1) ;
#63407=TOROIDAL_SURFACE('',#76286,0.9,0.1) ;
#63408=TOROIDAL_SURFACE('',#76298,0.3,0.1) ;
#63409=TOROIDAL_SURFACE('',#76317,0.3,0.1) ;
#63410=TOROIDAL_SURFACE('',#76329,0.9,0.1) ;
#63411=TOROIDAL_SURFACE('',#76330,0.9,0.1) ;
#63412=TOROIDAL_SURFACE('',#76342,0.3,0.1) ;
#63413=TOROIDAL_SURFACE('',#76361,0.3,0.1) ;
#63414=TOROIDAL_SURFACE('',#76373,0.9,0.1) ;
#63415=TOROIDAL_SURFACE('',#76374,0.9,0.1) ;
#63416=TOROIDAL_SURFACE('',#76386,0.3,0.1) ;
#63417=TOROIDAL_SURFACE('',#76405,0.3,0.1) ;
#63418=TOROIDAL_SURFACE('',#76417,0.9,0.1) ;
#63419=TOROIDAL_SURFACE('',#76418,0.9,0.1) ;
#63420=TOROIDAL_SURFACE('',#76430,0.3,0.1) ;
#63421=TOROIDAL_SURFACE('',#76449,0.3,0.1) ;
#63422=TOROIDAL_SURFACE('',#76461,0.9,0.1) ;
#63423=TOROIDAL_SURFACE('',#76462,0.9,0.1) ;
#63424=TOROIDAL_SURFACE('',#76474,0.3,0.1) ;
#63425=TOROIDAL_SURFACE('',#76493,0.3,0.1) ;
#63426=TOROIDAL_SURFACE('',#76505,0.9,0.1) ;
#63427=TOROIDAL_SURFACE('',#76506,0.9,0.1) ;
#63428=TOROIDAL_SURFACE('',#76518,0.3,0.1) ;
#63429=TOROIDAL_SURFACE('',#76537,0.3,0.1) ;
#63430=TOROIDAL_SURFACE('',#76549,0.9,0.1) ;
#63431=TOROIDAL_SURFACE('',#76550,0.9,0.1) ;
#63432=TOROIDAL_SURFACE('',#76562,0.3,0.1) ;
#63433=TOROIDAL_SURFACE('',#76581,0.3,0.1) ;
#63434=TOROIDAL_SURFACE('',#76593,0.9,0.1) ;
#63435=TOROIDAL_SURFACE('',#76594,0.9,0.1) ;
#63436=TOROIDAL_SURFACE('',#76606,0.3,0.1) ;
#63437=TOROIDAL_SURFACE('',#76625,0.3,0.1) ;
#63438=TOROIDAL_SURFACE('',#76637,0.9,0.1) ;
#63439=TOROIDAL_SURFACE('',#76638,0.9,0.1) ;
#63440=TOROIDAL_SURFACE('',#76650,0.3,0.1) ;
#65362=ADVANCED_FACE('',(#18077),#63117,.T.) ;
#65363=ADVANCED_FACE('',(#18078),#63118,.F.) ;
#65364=ADVANCED_FACE('',(#18079),#4427,.F.) ;
#65365=ADVANCED_FACE('',(#18080),#6802,.F.) ;
#65366=ADVANCED_FACE('',(#18081),#63119,.T.) ;
#65367=ADVANCED_FACE('',(#18082),#63120,.F.) ;
#65368=ADVANCED_FACE('',(#18083),#4428,.F.) ;
#65369=ADVANCED_FACE('',(#18084),#6803,.F.) ;
#65370=ADVANCED_FACE('',(#18085),#63121,.T.) ;
#65371=ADVANCED_FACE('',(#18086),#63122,.F.) ;
#65372=ADVANCED_FACE('',(#18087),#4429,.F.) ;
#65373=ADVANCED_FACE('',(#18088),#6804,.F.) ;
#65374=ADVANCED_FACE('',(#18089),#63123,.T.) ;
#65375=ADVANCED_FACE('',(#18090),#63124,.F.) ;
#65376=ADVANCED_FACE('',(#18091),#4430,.F.) ;
#65377=ADVANCED_FACE('',(#18092),#6805,.F.) ;
#65378=ADVANCED_FACE('',(#18093),#63125,.T.) ;
#65379=ADVANCED_FACE('',(#18094),#63126,.F.) ;
#65380=ADVANCED_FACE('',(#18095),#4431,.F.) ;
#65381=ADVANCED_FACE('',(#18096),#6806,.F.) ;
#65382=ADVANCED_FACE('',(#18097),#63127,.T.) ;
#65383=ADVANCED_FACE('',(#18098),#63128,.F.) ;
#65384=ADVANCED_FACE('',(#18099),#4432,.F.) ;
#65385=ADVANCED_FACE('',(#18100),#6807,.F.) ;
#65386=ADVANCED_FACE('',(#18101),#63129,.T.) ;
#65387=ADVANCED_FACE('',(#18102),#63130,.F.) ;
#65388=ADVANCED_FACE('',(#18103),#4433,.F.) ;
#65389=ADVANCED_FACE('',(#18104),#6808,.F.) ;
#65390=ADVANCED_FACE('',(#18105),#63131,.T.) ;
#65391=ADVANCED_FACE('',(#18106),#63132,.F.) ;
#65392=ADVANCED_FACE('',(#18107),#4434,.F.) ;
#65393=ADVANCED_FACE('',(#18108),#6809,.F.) ;
#65394=ADVANCED_FACE('',(#18109),#63133,.T.) ;
#65395=ADVANCED_FACE('',(#18110),#63134,.T.) ;
#65396=ADVANCED_FACE('',(#18111),#63135,.T.) ;
#65397=ADVANCED_FACE('',(#18112),#63136,.T.) ;
#65398=ADVANCED_FACE('',(#18113),#63137,.T.) ;
#65399=ADVANCED_FACE('',(#18114),#63138,.T.) ;
#65400=ADVANCED_FACE('',(#18115),#63139,.T.) ;
#65401=ADVANCED_FACE('',(#18116),#63140,.T.) ;
#65402=ADVANCED_FACE('',(#18117),#63141,.T.) ;
#65403=ADVANCED_FACE('',(#18118),#63142,.T.) ;
#65404=ADVANCED_FACE('',(#18119),#63143,.F.) ;
#65405=ADVANCED_FACE('',(#18120),#4435,.F.) ;
#65406=ADVANCED_FACE('',(#18121),#6810,.F.) ;
#65407=ADVANCED_FACE('',(#18122),#6811,.T.) ;
#65408=ADVANCED_FACE('',(#18123),#6812,.T.) ;
#65409=ADVANCED_FACE('',(#18124),#6813,.T.) ;
#65410=ADVANCED_FACE('',(#18125),#6814,.T.) ;
#65411=ADVANCED_FACE('',(#18126),#6815,.T.) ;
#65412=ADVANCED_FACE('',(#18127),#6816,.T.) ;
#65413=ADVANCED_FACE('',(#18128),#6817,.T.) ;
#65414=ADVANCED_FACE('',(#18129),#6818,.T.) ;
#65415=ADVANCED_FACE('',(#18130),#6819,.T.) ;
#65416=ADVANCED_FACE('',(#18131),#6820,.F.) ;
#65417=ADVANCED_FACE('',(#18132),#6821,.F.) ;
#65418=ADVANCED_FACE('',(#18133),#6822,.F.) ;
#65419=ADVANCED_FACE('',(#18134),#6823,.F.) ;
#65420=ADVANCED_FACE('',(#18135),#6824,.F.) ;
#65421=ADVANCED_FACE('',(#18136),#6825,.F.) ;
#65422=ADVANCED_FACE('',(#18137),#6826,.F.) ;
#65423=ADVANCED_FACE('',(#18138),#6827,.F.) ;
#65424=ADVANCED_FACE('',(#18139),#6828,.F.) ;
#65425=ADVANCED_FACE('',(#18140),#63144,.T.) ;
#65426=ADVANCED_FACE('',(#18141),#63145,.T.) ;
#65427=ADVANCED_FACE('',(#18142),#63146,.F.) ;
#65428=ADVANCED_FACE('',(#18143),#4436,.F.) ;
#65429=ADVANCED_FACE('',(#18144),#6829,.F.) ;
#65430=ADVANCED_FACE('',(#18145),#6830,.T.) ;
#65431=ADVANCED_FACE('',(#18146),#6831,.F.) ;
#65432=ADVANCED_FACE('',(#18147),#5483,.T.) ;
#65433=ADVANCED_FACE('',(#18148),#5484,.T.) ;
#65434=ADVANCED_FACE('',(#18149),#5485,.T.) ;
#65435=ADVANCED_FACE('',(#18150),#5486,.T.) ;
#65436=ADVANCED_FACE('',(#18151),#5487,.T.) ;
#65437=ADVANCED_FACE('',(#18152),#5488,.T.) ;
#65438=ADVANCED_FACE('',(#18153),#5489,.T.) ;
#65439=ADVANCED_FACE('',(#18154),#5490,.T.) ;
#65440=ADVANCED_FACE('',(#18155),#5491,.T.) ;
#65441=ADVANCED_FACE('',(#18156),#5492,.F.) ;
#65442=ADVANCED_FACE('',(#18157),#5493,.F.) ;
#65443=ADVANCED_FACE('',(#18158),#5494,.F.) ;
#65444=ADVANCED_FACE('',(#18159),#5495,.F.) ;
#65445=ADVANCED_FACE('',(#18160),#5496,.F.) ;
#65446=ADVANCED_FACE('',(#18161),#5497,.F.) ;
#65447=ADVANCED_FACE('',(#18162),#5498,.F.) ;
#65448=ADVANCED_FACE('',(#18163),#5499,.F.) ;
#65449=ADVANCED_FACE('',(#18164),#5500,.F.) ;
#65450=ADVANCED_FACE('',(#18165),#5501,.F.) ;
#65451=ADVANCED_FACE('',(#18166),#5502,.F.) ;
#65452=ADVANCED_FACE('',(#18167),#5503,.F.) ;
#65453=ADVANCED_FACE('',(#18168),#5504,.F.) ;
#65454=ADVANCED_FACE('',(#18169),#5505,.F.) ;
#65455=ADVANCED_FACE('',(#18170),#5506,.F.) ;
#65456=ADVANCED_FACE('',(#18171),#5507,.F.) ;
#65457=ADVANCED_FACE('',(#18172),#5508,.F.) ;
#65458=ADVANCED_FACE('',(#18173),#5509,.F.) ;
#65459=ADVANCED_FACE('',(#18174),#6832,.T.) ;
#65460=ADVANCED_FACE('',(#18175),#6833,.T.) ;
#65461=ADVANCED_FACE('',(#18176),#6834,.T.) ;
#65462=ADVANCED_FACE('',(#18177),#6835,.T.) ;
#65463=ADVANCED_FACE('',(#18178),#6836,.T.) ;
#65464=ADVANCED_FACE('',(#18179),#6837,.T.) ;
#65465=ADVANCED_FACE('',(#18180),#6838,.T.) ;
#65466=ADVANCED_FACE('',(#18181),#6839,.T.) ;
#65467=ADVANCED_FACE('',(#18182),#6840,.T.) ;
#65468=ADVANCED_FACE('',(#18183),#5510,.T.) ;
#65469=ADVANCED_FACE('',(#18184),#5511,.F.) ;
#65470=ADVANCED_FACE('',(#18185),#5512,.F.) ;
#65471=ADVANCED_FACE('',(#18186),#6841,.T.) ;
#65472=ADVANCED_FACE('',(#18187),#6842,.T.) ;
#65473=ADVANCED_FACE('',(#18188),#5513,.T.) ;
#65474=ADVANCED_FACE('',(#18189),#6843,.T.) ;
#65475=ADVANCED_FACE('',(#18190),#5514,.T.) ;
#65476=ADVANCED_FACE('',(#18191),#6844,.T.) ;
#65477=ADVANCED_FACE('',(#18192),#5515,.T.) ;
#65478=ADVANCED_FACE('',(#18193),#6845,.F.) ;
#65479=ADVANCED_FACE('',(#18194),#5516,.T.) ;
#65480=ADVANCED_FACE('',(#18195),#6846,.T.) ;
#65481=ADVANCED_FACE('',(#18196),#5517,.T.) ;
#65482=ADVANCED_FACE('',(#18197),#6847,.T.) ;
#65483=ADVANCED_FACE('',(#18198),#5518,.T.) ;
#65484=ADVANCED_FACE('',(#18199),#6848,.F.) ;
#65485=ADVANCED_FACE('',(#18200),#5519,.T.) ;
#65486=ADVANCED_FACE('',(#18201),#6849,.T.) ;
#65487=ADVANCED_FACE('',(#18202,#5031,#5032,#5033,#5034,#5035,#5036,#5037,
#5038,#5039,#5040),#5520,.T.) ;
#65488=ADVANCED_FACE('',(#18203),#5521,.F.) ;
#65489=ADVANCED_FACE('',(#18204),#5522,.T.) ;
#65490=ADVANCED_FACE('',(#18205),#5523,.T.) ;
#65491=ADVANCED_FACE('',(#18206),#5524,.F.) ;
#65492=ADVANCED_FACE('',(#18207),#5525,.F.) ;
#65493=ADVANCED_FACE('',(#18208),#5526,.F.) ;
#65494=ADVANCED_FACE('',(#18209),#5527,.F.) ;
#65495=ADVANCED_FACE('',(#18210),#5528,.F.) ;
#65496=ADVANCED_FACE('',(#18211),#6850,.T.) ;
#65497=ADVANCED_FACE('',(#18212),#5529,.F.) ;
#65498=ADVANCED_FACE('',(#18213),#6851,.T.) ;
#65499=ADVANCED_FACE('',(#18214),#5530,.F.) ;
#65500=ADVANCED_FACE('',(#18215),#6852,.F.) ;
#65501=ADVANCED_FACE('',(#18216),#5531,.F.) ;
#65502=ADVANCED_FACE('',(#18217),#6853,.F.) ;
#65503=ADVANCED_FACE('',(#18218),#5532,.F.) ;
#65504=ADVANCED_FACE('',(#18219),#5533,.F.) ;
#65505=ADVANCED_FACE('',(#18220),#6854,.F.) ;
#65506=ADVANCED_FACE('',(#18221),#5534,.F.) ;
#65507=ADVANCED_FACE('',(#18222),#6855,.T.) ;
#65508=ADVANCED_FACE('',(#18223),#5535,.F.) ;
#65509=ADVANCED_FACE('',(#18224),#6856,.T.) ;
#65510=ADVANCED_FACE('',(#18225),#5536,.F.) ;
#65511=ADVANCED_FACE('',(#18226),#6857,.F.) ;
#65512=ADVANCED_FACE('',(#18227),#5537,.F.) ;
#65513=ADVANCED_FACE('',(#18228),#6858,.F.) ;
#65514=ADVANCED_FACE('',(#18229),#5538,.F.) ;
#65515=ADVANCED_FACE('',(#18230),#6859,.F.) ;
#65516=ADVANCED_FACE('',(#18231),#6860,.T.) ;
#65517=ADVANCED_FACE('',(#18232),#6861,.F.) ;
#65518=ADVANCED_FACE('',(#18233),#5539,.F.) ;
#65519=ADVANCED_FACE('',(#18234),#6862,.F.) ;
#65520=ADVANCED_FACE('',(#18235),#5540,.F.) ;
#65521=ADVANCED_FACE('',(#18236),#6863,.F.) ;
#65522=ADVANCED_FACE('',(#18237),#5541,.F.) ;
#65523=ADVANCED_FACE('',(#18238,#5041),#5542,.F.) ;
#65524=ADVANCED_FACE('',(#18239,#5042),#5543,.T.) ;
#65525=ADVANCED_FACE('',(#18240),#6864,.T.) ;
#65526=ADVANCED_FACE('',(#18241),#6865,.F.) ;
#65527=ADVANCED_FACE('',(#18242),#4437,.F.) ;
#65528=ADVANCED_FACE('',(#18243),#4438,.T.) ;
#65529=ADVANCED_FACE('',(#18244),#63147,.T.) ;
#65530=ADVANCED_FACE('',(#18245),#6866,.F.) ;
#65531=ADVANCED_FACE('',(#18246),#6867,.F.) ;
#65532=ADVANCED_FACE('',(#18247),#6868,.T.) ;
#65533=ADVANCED_FACE('',(#18248),#6869,.T.) ;
#65534=ADVANCED_FACE('',(#18249),#6870,.T.) ;
#65535=ADVANCED_FACE('',(#18250),#6871,.F.) ;
#65536=ADVANCED_FACE('',(#18251),#4439,.F.) ;
#65537=ADVANCED_FACE('',(#18252),#63148,.F.) ;
#65538=ADVANCED_FACE('',(#18253),#63149,.F.) ;
#65539=ADVANCED_FACE('',(#18254),#63150,.T.) ;
#65540=ADVANCED_FACE('',(#18255),#6872,.F.) ;
#65541=ADVANCED_FACE('',(#18256),#6873,.F.) ;
#65542=ADVANCED_FACE('',(#18257),#6874,.F.) ;
#65543=ADVANCED_FACE('',(#18258),#6875,.T.) ;
#65544=ADVANCED_FACE('',(#18259),#6876,.T.) ;
#65545=ADVANCED_FACE('',(#18260),#63151,.F.) ;
#65546=ADVANCED_FACE('',(#18261),#4440,.F.) ;
#65547=ADVANCED_FACE('',(#18262),#4441,.T.) ;
#65548=ADVANCED_FACE('',(#18263),#6877,.T.) ;
#65549=ADVANCED_FACE('',(#18264),#4442,.F.) ;
#65550=ADVANCED_FACE('',(#18265),#4443,.T.) ;
#65551=ADVANCED_FACE('',(#18266),#6878,.F.) ;
#65552=ADVANCED_FACE('',(#18267),#6879,.F.) ;
#65553=ADVANCED_FACE('',(#18268),#6880,.T.) ;
#65554=ADVANCED_FACE('',(#18269),#63152,.T.) ;
#65555=ADVANCED_FACE('',(#18270),#6881,.F.) ;
#65556=ADVANCED_FACE('',(#18271),#6882,.T.) ;
#65557=ADVANCED_FACE('',(#18272),#6883,.F.) ;
#65558=ADVANCED_FACE('',(#18273),#4444,.F.) ;
#65559=ADVANCED_FACE('',(#18274),#63153,.T.) ;
#65560=ADVANCED_FACE('',(#18275),#6884,.T.) ;
#65561=ADVANCED_FACE('',(#18276),#4445,.F.) ;
#65562=ADVANCED_FACE('',(#18277),#63154,.F.) ;
#65563=ADVANCED_FACE('',(#18278),#6885,.F.) ;
#65564=ADVANCED_FACE('',(#18279),#6886,.T.) ;
#65565=ADVANCED_FACE('',(#18280),#63155,.T.) ;
#65566=ADVANCED_FACE('',(#18281),#6887,.F.) ;
#65567=ADVANCED_FACE('',(#18282),#63156,.T.) ;
#65568=ADVANCED_FACE('',(#18283),#6888,.T.) ;
#65569=ADVANCED_FACE('',(#18284),#6889,.T.) ;
#65570=ADVANCED_FACE('',(#18285),#4446,.T.) ;
#65571=ADVANCED_FACE('',(#18286),#4447,.T.) ;
#65572=ADVANCED_FACE('',(#18287),#6890,.T.) ;
#65573=ADVANCED_FACE('',(#18288),#6891,.T.) ;
#65574=ADVANCED_FACE('',(#18289),#63157,.T.) ;
#65575=ADVANCED_FACE('',(#18290),#4448,.T.) ;
#65576=ADVANCED_FACE('',(#18291),#6892,.T.) ;
#65577=ADVANCED_FACE('',(#18292),#6893,.T.) ;
#65578=ADVANCED_FACE('',(#18293),#4449,.T.) ;
#65579=ADVANCED_FACE('',(#18294),#63158,.T.) ;
#65580=ADVANCED_FACE('',(#18295),#6894,.T.) ;
#65581=ADVANCED_FACE('',(#18296),#6895,.T.) ;
#65582=ADVANCED_FACE('',(#18297),#4450,.T.) ;
#65583=ADVANCED_FACE('',(#18298),#4451,.T.) ;
#65584=ADVANCED_FACE('',(#18299),#6896,.T.) ;
#65585=ADVANCED_FACE('',(#18300),#6897,.T.) ;
#65586=ADVANCED_FACE('',(#18301),#4452,.T.) ;
#65587=ADVANCED_FACE('',(#18302),#4453,.T.) ;
#65588=ADVANCED_FACE('',(#18303),#6898,.T.) ;
#65589=ADVANCED_FACE('',(#18304),#6899,.T.) ;
#65590=ADVANCED_FACE('',(#18305),#63159,.T.) ;
#65591=ADVANCED_FACE('',(#18306),#4454,.T.) ;
#65592=ADVANCED_FACE('',(#18307),#6900,.T.) ;
#65593=ADVANCED_FACE('',(#18308),#6901,.T.) ;
#65594=ADVANCED_FACE('',(#18309),#4455,.T.) ;
#65595=ADVANCED_FACE('',(#18310),#63160,.T.) ;
#65596=ADVANCED_FACE('',(#18311),#6902,.T.) ;
#65597=ADVANCED_FACE('',(#18312),#6903,.T.) ;
#65598=ADVANCED_FACE('',(#18313),#4456,.T.) ;
#65599=ADVANCED_FACE('',(#18314),#4457,.T.) ;
#65600=ADVANCED_FACE('',(#18315),#6904,.T.) ;
#65601=ADVANCED_FACE('',(#18316),#6905,.T.) ;
#65602=ADVANCED_FACE('',(#18317),#4458,.T.) ;
#65603=ADVANCED_FACE('',(#18318),#6906,.F.) ;
#65604=ADVANCED_FACE('',(#18319),#63161,.F.) ;
#65605=ADVANCED_FACE('',(#18320),#4459,.F.) ;
#65606=ADVANCED_FACE('',(#18321),#6907,.F.) ;
#65607=ADVANCED_FACE('',(#18322),#6908,.F.) ;
#65608=ADVANCED_FACE('',(#18323),#63162,.F.) ;
#65609=ADVANCED_FACE('',(#18324),#4460,.F.) ;
#65610=ADVANCED_FACE('',(#18325),#6909,.F.) ;
#65611=ADVANCED_FACE('',(#18326),#6910,.F.) ;
#65612=ADVANCED_FACE('',(#18327),#4461,.F.) ;
#65613=ADVANCED_FACE('',(#18328),#4462,.F.) ;
#65614=ADVANCED_FACE('',(#18329),#6911,.F.) ;
#65615=ADVANCED_FACE('',(#18330),#63163,.F.) ;
#65616=ADVANCED_FACE('',(#18331),#4463,.F.) ;
#65617=ADVANCED_FACE('',(#18332),#4464,.F.) ;
#65618=ADVANCED_FACE('',(#18333),#6912,.F.) ;
#65619=ADVANCED_FACE('',(#18334),#6913,.F.) ;
#65620=ADVANCED_FACE('',(#18335),#4465,.F.) ;
#65621=ADVANCED_FACE('',(#18336),#6914,.F.) ;
#65622=ADVANCED_FACE('',(#18337),#6915,.F.) ;
#65623=ADVANCED_FACE('',(#18338),#4466,.F.) ;
#65624=ADVANCED_FACE('',(#18339),#4467,.F.) ;
#65625=ADVANCED_FACE('',(#18340),#6916,.F.) ;
#65626=ADVANCED_FACE('',(#18341),#6917,.F.) ;
#65627=ADVANCED_FACE('',(#18342),#63164,.F.) ;
#65628=ADVANCED_FACE('',(#18343),#63165,.F.) ;
#65629=ADVANCED_FACE('',(#18344),#6918,.F.) ;
#65630=ADVANCED_FACE('',(#18345),#6919,.T.) ;
#65631=ADVANCED_FACE('',(#18346),#4468,.T.) ;
#65632=ADVANCED_FACE('',(#18347),#4469,.T.) ;
#65633=ADVANCED_FACE('',(#18348),#6920,.T.) ;
#65634=ADVANCED_FACE('',(#18349),#6921,.T.) ;
#65635=ADVANCED_FACE('',(#18350),#63166,.T.) ;
#65636=ADVANCED_FACE('',(#18351),#63167,.T.) ;
#65637=ADVANCED_FACE('',(#18352),#6922,.T.) ;
#65638=ADVANCED_FACE('',(#18353),#6923,.T.) ;
#65639=ADVANCED_FACE('',(#18354),#63168,.T.) ;
#65640=ADVANCED_FACE('',(#18355),#6924,.T.) ;
#65641=ADVANCED_FACE('',(#18356),#6925,.T.) ;
#65642=ADVANCED_FACE('',(#18357),#63169,.T.) ;
#65643=ADVANCED_FACE('',(#18358),#63170,.T.) ;
#65644=ADVANCED_FACE('',(#18359),#6926,.T.) ;
#65645=ADVANCED_FACE('',(#18360),#63171,.T.) ;
#65646=ADVANCED_FACE('',(#18361),#63172,.T.) ;
#65647=ADVANCED_FACE('',(#18362),#63173,.T.) ;
#65648=ADVANCED_FACE('',(#18363),#6927,.T.) ;
#65649=ADVANCED_FACE('',(#18364),#6928,.T.) ;
#65650=ADVANCED_FACE('',(#18365),#4470,.T.) ;
#65651=ADVANCED_FACE('',(#18366),#63174,.T.) ;
#65652=ADVANCED_FACE('',(#18367),#6929,.T.) ;
#65653=ADVANCED_FACE('',(#18368),#6930,.T.) ;
#65654=ADVANCED_FACE('',(#18369),#4471,.T.) ;
#65655=ADVANCED_FACE('',(#18370),#63175,.T.) ;
#65656=ADVANCED_FACE('',(#18371),#6931,.T.) ;
#65657=ADVANCED_FACE('',(#18372),#5544,.F.) ;
#65658=ADVANCED_FACE('',(#18373),#5545,.F.) ;
#65659=ADVANCED_FACE('',(#18374),#5546,.F.) ;
#65660=ADVANCED_FACE('',(#18375),#5547,.F.) ;
#65661=ADVANCED_FACE('',(#18376),#5548,.F.) ;
#65662=ADVANCED_FACE('',(#18377),#5549,.T.) ;
#65663=ADVANCED_FACE('',(#18378),#5550,.F.) ;
#65664=ADVANCED_FACE('',(#18379),#6932,.T.) ;
#65665=ADVANCED_FACE('',(#18380),#6933,.F.) ;
#65666=ADVANCED_FACE('',(#18381),#5551,.F.) ;
#65667=ADVANCED_FACE('',(#18382),#5552,.F.) ;
#65668=ADVANCED_FACE('',(#18383),#5553,.F.) ;
#65669=ADVANCED_FACE('',(#18384),#5554,.F.) ;
#65670=ADVANCED_FACE('',(#18385),#5555,.F.) ;
#65671=ADVANCED_FACE('',(#18386),#5556,.T.) ;
#65672=ADVANCED_FACE('',(#18387),#5557,.F.) ;
#65673=ADVANCED_FACE('',(#18388),#5558,.F.) ;
#65674=ADVANCED_FACE('',(#18389),#5559,.F.) ;
#65675=ADVANCED_FACE('',(#18390),#5560,.F.) ;
#65676=ADVANCED_FACE('',(#18391),#5561,.F.) ;
#65677=ADVANCED_FACE('',(#18392),#6934,.T.) ;
#65678=ADVANCED_FACE('',(#18393),#6935,.T.) ;
#65679=ADVANCED_FACE('',(#18394),#4472,.T.) ;
#65680=ADVANCED_FACE('',(#18395),#6936,.T.) ;
#65681=ADVANCED_FACE('',(#18396),#6937,.T.) ;
#65682=ADVANCED_FACE('',(#18397),#6938,.T.) ;
#65683=ADVANCED_FACE('',(#18398),#4473,.T.) ;
#65684=ADVANCED_FACE('',(#18399),#4474,.T.) ;
#65685=ADVANCED_FACE('',(#18400),#6939,.T.) ;
#65686=ADVANCED_FACE('',(#18401),#6940,.T.) ;
#65687=ADVANCED_FACE('',(#18402),#6941,.T.) ;
#65688=ADVANCED_FACE('',(#18403),#4475,.T.) ;
#65689=ADVANCED_FACE('',(#18404),#6942,.T.) ;
#65690=ADVANCED_FACE('',(#18405),#6943,.T.) ;
#65691=ADVANCED_FACE('',(#18406),#6944,.T.) ;
#65692=ADVANCED_FACE('',(#18407),#6945,.T.) ;
#65693=ADVANCED_FACE('',(#18408),#4476,.T.) ;
#65694=ADVANCED_FACE('',(#18409),#6946,.T.) ;
#65695=ADVANCED_FACE('',(#18410),#6947,.T.) ;
#65696=ADVANCED_FACE('',(#18411),#6948,.T.) ;
#65697=ADVANCED_FACE('',(#18412),#4477,.T.) ;
#65698=ADVANCED_FACE('',(#18413),#4478,.T.) ;
#65699=ADVANCED_FACE('',(#18414),#6949,.T.) ;
#65700=ADVANCED_FACE('',(#18415),#6950,.T.) ;
#65701=ADVANCED_FACE('',(#18416),#6951,.T.) ;
#65702=ADVANCED_FACE('',(#18417),#4479,.T.) ;
#65703=ADVANCED_FACE('',(#18418),#6952,.T.) ;
#65704=ADVANCED_FACE('',(#18419),#6953,.T.) ;
#65705=ADVANCED_FACE('',(#18420),#63176,.T.) ;
#65706=ADVANCED_FACE('',(#18421),#6954,.T.) ;
#65707=ADVANCED_FACE('',(#18422),#4480,.T.) ;
#65708=ADVANCED_FACE('',(#18423),#6955,.T.) ;
#65709=ADVANCED_FACE('',(#18424),#4481,.T.) ;
#65710=ADVANCED_FACE('',(#18425),#6956,.T.) ;
#65711=ADVANCED_FACE('',(#18426),#63177,.T.) ;
#65712=ADVANCED_FACE('',(#18427),#63178,.T.) ;
#65713=ADVANCED_FACE('',(#18428),#6957,.T.) ;
#65714=ADVANCED_FACE('',(#18429),#4482,.T.) ;
#65715=ADVANCED_FACE('',(#18430),#6958,.T.) ;
#65716=ADVANCED_FACE('',(#18431),#4483,.T.) ;
#65717=ADVANCED_FACE('',(#18432),#6959,.T.) ;
#65718=ADVANCED_FACE('',(#18433),#63179,.T.) ;
#65719=ADVANCED_FACE('',(#18434),#6960,.T.) ;
#65720=ADVANCED_FACE('',(#18435),#4484,.T.) ;
#65721=ADVANCED_FACE('',(#18436),#6961,.T.) ;
#65722=ADVANCED_FACE('',(#18437),#4485,.T.) ;
#65723=ADVANCED_FACE('',(#18438),#6962,.T.) ;
#65724=ADVANCED_FACE('',(#18439),#6963,.T.) ;
#65725=ADVANCED_FACE('',(#18440),#4486,.T.) ;
#65726=ADVANCED_FACE('',(#18441),#6964,.T.) ;
#65727=ADVANCED_FACE('',(#18442),#6965,.T.) ;
#65728=ADVANCED_FACE('',(#18443),#4487,.T.) ;
#65729=ADVANCED_FACE('',(#18444),#5562,.T.) ;
#65730=ADVANCED_FACE('',(#18445),#5563,.T.) ;
#65731=ADVANCED_FACE('',(#18446),#5564,.T.) ;
#65732=ADVANCED_FACE('',(#18447),#5565,.T.) ;
#65733=ADVANCED_FACE('',(#18448),#5566,.T.) ;
#65734=ADVANCED_FACE('',(#18449),#5567,.T.) ;
#65735=ADVANCED_FACE('',(#18450),#5568,.T.) ;
#65736=ADVANCED_FACE('',(#18451),#5569,.T.) ;
#65737=ADVANCED_FACE('',(#18452),#5570,.T.) ;
#65738=ADVANCED_FACE('',(#18453),#5571,.F.) ;
#65739=ADVANCED_FACE('',(#18454),#5572,.F.) ;
#65740=ADVANCED_FACE('',(#18455),#5573,.F.) ;
#65741=ADVANCED_FACE('',(#18456),#5574,.F.) ;
#65742=ADVANCED_FACE('',(#18457),#5575,.F.) ;
#65743=ADVANCED_FACE('',(#18458),#5576,.F.) ;
#65744=ADVANCED_FACE('',(#18459),#5577,.F.) ;
#65745=ADVANCED_FACE('',(#18460),#5578,.F.) ;
#65746=ADVANCED_FACE('',(#18461),#5579,.F.) ;
#65747=ADVANCED_FACE('',(#18462),#5580,.F.) ;
#65748=ADVANCED_FACE('',(#18463),#5581,.F.) ;
#65749=ADVANCED_FACE('',(#18464),#5582,.F.) ;
#65750=ADVANCED_FACE('',(#18465),#5583,.F.) ;
#65751=ADVANCED_FACE('',(#18466),#5584,.F.) ;
#65752=ADVANCED_FACE('',(#18467),#5585,.F.) ;
#65753=ADVANCED_FACE('',(#18468),#5586,.F.) ;
#65754=ADVANCED_FACE('',(#18469),#5587,.F.) ;
#65755=ADVANCED_FACE('',(#18470),#5588,.F.) ;
#65756=ADVANCED_FACE('',(#18471),#5589,.F.) ;
#65757=ADVANCED_FACE('',(#18472),#5590,.F.) ;
#65758=ADVANCED_FACE('',(#18473),#5591,.F.) ;
#65759=ADVANCED_FACE('',(#18474),#5592,.F.) ;
#65760=ADVANCED_FACE('',(#18475),#5593,.F.) ;
#65761=ADVANCED_FACE('',(#18476),#5594,.F.) ;
#65762=ADVANCED_FACE('',(#18477),#5595,.F.) ;
#65763=ADVANCED_FACE('',(#18478),#5596,.F.) ;
#65764=ADVANCED_FACE('',(#18479),#5597,.F.) ;
#65765=ADVANCED_FACE('',(#18480),#5598,.F.) ;
#65766=ADVANCED_FACE('',(#18481),#5599,.F.) ;
#65767=ADVANCED_FACE('',(#18482),#5600,.F.) ;
#65768=ADVANCED_FACE('',(#18483),#5601,.F.) ;
#65769=ADVANCED_FACE('',(#18484),#5602,.F.) ;
#65770=ADVANCED_FACE('',(#18485),#5603,.F.) ;
#65771=ADVANCED_FACE('',(#18486),#5604,.F.) ;
#65772=ADVANCED_FACE('',(#18487),#5605,.F.) ;
#65773=ADVANCED_FACE('',(#18488),#5606,.F.) ;
#65774=ADVANCED_FACE('',(#18489),#5607,.F.) ;
#65775=ADVANCED_FACE('',(#18490),#5608,.F.) ;
#65776=ADVANCED_FACE('',(#18491),#5609,.F.) ;
#65777=ADVANCED_FACE('',(#18492),#5610,.F.) ;
#65778=ADVANCED_FACE('',(#18493),#5611,.F.) ;
#65779=ADVANCED_FACE('',(#18494),#5612,.F.) ;
#65780=ADVANCED_FACE('',(#18495),#5613,.F.) ;
#65781=ADVANCED_FACE('',(#18496),#5614,.F.) ;
#65782=ADVANCED_FACE('',(#18497),#5615,.F.) ;
#65783=ADVANCED_FACE('',(#18498),#6966,.T.) ;
#65784=ADVANCED_FACE('',(#18499),#5616,.F.) ;
#65785=ADVANCED_FACE('',(#18500),#6967,.T.) ;
#65786=ADVANCED_FACE('',(#18501),#5617,.F.) ;
#65787=ADVANCED_FACE('',(#18502),#6968,.F.) ;
#65788=ADVANCED_FACE('',(#18503),#5618,.F.) ;
#65789=ADVANCED_FACE('',(#18504),#6969,.F.) ;
#65790=ADVANCED_FACE('',(#18505),#5619,.F.) ;
#65791=ADVANCED_FACE('',(#18506),#5620,.F.) ;
#65792=ADVANCED_FACE('',(#18507),#6970,.F.) ;
#65793=ADVANCED_FACE('',(#18508),#5621,.F.) ;
#65794=ADVANCED_FACE('',(#18509),#6971,.T.) ;
#65795=ADVANCED_FACE('',(#18510),#5622,.F.) ;
#65796=ADVANCED_FACE('',(#18511),#6972,.T.) ;
#65797=ADVANCED_FACE('',(#18512),#5623,.F.) ;
#65798=ADVANCED_FACE('',(#18513),#6973,.F.) ;
#65799=ADVANCED_FACE('',(#18514),#5624,.F.) ;
#65800=ADVANCED_FACE('',(#18515),#6974,.F.) ;
#65801=ADVANCED_FACE('',(#18516),#5625,.F.) ;
#65802=ADVANCED_FACE('',(#18517),#6975,.F.) ;
#65803=ADVANCED_FACE('',(#18518),#6976,.T.) ;
#65804=ADVANCED_FACE('',(#18519),#6977,.F.) ;
#65805=ADVANCED_FACE('',(#18520),#5626,.F.) ;
#65806=ADVANCED_FACE('',(#18521),#6978,.F.) ;
#65807=ADVANCED_FACE('',(#18522),#5627,.F.) ;
#65808=ADVANCED_FACE('',(#18523),#6979,.F.) ;
#65809=ADVANCED_FACE('',(#18524),#5628,.F.) ;
#65810=ADVANCED_FACE('',(#18525,#5043),#5629,.F.) ;
#65811=ADVANCED_FACE('',(#18526),#6980,.T.) ;
#65812=ADVANCED_FACE('',(#18527),#5630,.F.) ;
#65813=ADVANCED_FACE('',(#18528),#6981,.T.) ;
#65814=ADVANCED_FACE('',(#18529),#5631,.F.) ;
#65815=ADVANCED_FACE('',(#18530),#6982,.F.) ;
#65816=ADVANCED_FACE('',(#18531),#5632,.F.) ;
#65817=ADVANCED_FACE('',(#18532),#6983,.F.) ;
#65818=ADVANCED_FACE('',(#18533),#5633,.F.) ;
#65819=ADVANCED_FACE('',(#18534),#5634,.F.) ;
#65820=ADVANCED_FACE('',(#18535),#6984,.F.) ;
#65821=ADVANCED_FACE('',(#18536),#5635,.F.) ;
#65822=ADVANCED_FACE('',(#18537),#6985,.T.) ;
#65823=ADVANCED_FACE('',(#18538),#5636,.F.) ;
#65824=ADVANCED_FACE('',(#18539),#6986,.T.) ;
#65825=ADVANCED_FACE('',(#18540),#5637,.F.) ;
#65826=ADVANCED_FACE('',(#18541),#6987,.F.) ;
#65827=ADVANCED_FACE('',(#18542),#5638,.F.) ;
#65828=ADVANCED_FACE('',(#18543),#6988,.F.) ;
#65829=ADVANCED_FACE('',(#18544),#5639,.F.) ;
#65830=ADVANCED_FACE('',(#18545),#6989,.F.) ;
#65831=ADVANCED_FACE('',(#18546),#6990,.T.) ;
#65832=ADVANCED_FACE('',(#18547),#6991,.F.) ;
#65833=ADVANCED_FACE('',(#18548),#5640,.F.) ;
#65834=ADVANCED_FACE('',(#18549),#6992,.F.) ;
#65835=ADVANCED_FACE('',(#18550),#5641,.F.) ;
#65836=ADVANCED_FACE('',(#18551),#6993,.F.) ;
#65837=ADVANCED_FACE('',(#18552),#5642,.F.) ;
#65838=ADVANCED_FACE('',(#18553,#5044),#5643,.F.) ;
#65839=ADVANCED_FACE('',(#18554),#6994,.T.) ;
#65840=ADVANCED_FACE('',(#18555),#5644,.F.) ;
#65841=ADVANCED_FACE('',(#18556),#6995,.T.) ;
#65842=ADVANCED_FACE('',(#18557),#5645,.F.) ;
#65843=ADVANCED_FACE('',(#18558),#6996,.F.) ;
#65844=ADVANCED_FACE('',(#18559),#5646,.F.) ;
#65845=ADVANCED_FACE('',(#18560),#6997,.F.) ;
#65846=ADVANCED_FACE('',(#18561),#5647,.F.) ;
#65847=ADVANCED_FACE('',(#18562),#5648,.F.) ;
#65848=ADVANCED_FACE('',(#18563),#6998,.F.) ;
#65849=ADVANCED_FACE('',(#18564),#5649,.F.) ;
#65850=ADVANCED_FACE('',(#18565),#6999,.T.) ;
#65851=ADVANCED_FACE('',(#18566),#5650,.F.) ;
#65852=ADVANCED_FACE('',(#18567),#7000,.T.) ;
#65853=ADVANCED_FACE('',(#18568),#5651,.F.) ;
#65854=ADVANCED_FACE('',(#18569),#7001,.F.) ;
#65855=ADVANCED_FACE('',(#18570),#5652,.F.) ;
#65856=ADVANCED_FACE('',(#18571),#7002,.F.) ;
#65857=ADVANCED_FACE('',(#18572),#5653,.F.) ;
#65858=ADVANCED_FACE('',(#18573),#7003,.F.) ;
#65859=ADVANCED_FACE('',(#18574),#7004,.T.) ;
#65860=ADVANCED_FACE('',(#18575),#7005,.F.) ;
#65861=ADVANCED_FACE('',(#18576),#5654,.F.) ;
#65862=ADVANCED_FACE('',(#18577),#7006,.F.) ;
#65863=ADVANCED_FACE('',(#18578),#5655,.F.) ;
#65864=ADVANCED_FACE('',(#18579),#7007,.F.) ;
#65865=ADVANCED_FACE('',(#18580),#5656,.F.) ;
#65866=ADVANCED_FACE('',(#18581,#5045),#5657,.F.) ;
#65867=ADVANCED_FACE('',(#18582),#7008,.T.) ;
#65868=ADVANCED_FACE('',(#18583),#5658,.F.) ;
#65869=ADVANCED_FACE('',(#18584),#7009,.T.) ;
#65870=ADVANCED_FACE('',(#18585),#5659,.F.) ;
#65871=ADVANCED_FACE('',(#18586),#7010,.F.) ;
#65872=ADVANCED_FACE('',(#18587),#5660,.F.) ;
#65873=ADVANCED_FACE('',(#18588),#7011,.F.) ;
#65874=ADVANCED_FACE('',(#18589),#5661,.F.) ;
#65875=ADVANCED_FACE('',(#18590),#5662,.F.) ;
#65876=ADVANCED_FACE('',(#18591),#7012,.F.) ;
#65877=ADVANCED_FACE('',(#18592),#5663,.F.) ;
#65878=ADVANCED_FACE('',(#18593),#7013,.T.) ;
#65879=ADVANCED_FACE('',(#18594),#5664,.F.) ;
#65880=ADVANCED_FACE('',(#18595),#7014,.T.) ;
#65881=ADVANCED_FACE('',(#18596),#5665,.F.) ;
#65882=ADVANCED_FACE('',(#18597),#7015,.F.) ;
#65883=ADVANCED_FACE('',(#18598),#5666,.F.) ;
#65884=ADVANCED_FACE('',(#18599),#7016,.F.) ;
#65885=ADVANCED_FACE('',(#18600),#5667,.F.) ;
#65886=ADVANCED_FACE('',(#18601),#7017,.F.) ;
#65887=ADVANCED_FACE('',(#18602),#7018,.T.) ;
#65888=ADVANCED_FACE('',(#18603),#7019,.F.) ;
#65889=ADVANCED_FACE('',(#18604),#5668,.F.) ;
#65890=ADVANCED_FACE('',(#18605),#7020,.F.) ;
#65891=ADVANCED_FACE('',(#18606),#5669,.F.) ;
#65892=ADVANCED_FACE('',(#18607),#7021,.F.) ;
#65893=ADVANCED_FACE('',(#18608),#5670,.F.) ;
#65894=ADVANCED_FACE('',(#18609,#5046),#5671,.F.) ;
#65895=ADVANCED_FACE('',(#18610),#7022,.T.) ;
#65896=ADVANCED_FACE('',(#18611),#5672,.F.) ;
#65897=ADVANCED_FACE('',(#18612),#7023,.T.) ;
#65898=ADVANCED_FACE('',(#18613),#5673,.F.) ;
#65899=ADVANCED_FACE('',(#18614),#7024,.F.) ;
#65900=ADVANCED_FACE('',(#18615),#5674,.F.) ;
#65901=ADVANCED_FACE('',(#18616),#7025,.F.) ;
#65902=ADVANCED_FACE('',(#18617),#5675,.F.) ;
#65903=ADVANCED_FACE('',(#18618),#5676,.F.) ;
#65904=ADVANCED_FACE('',(#18619),#7026,.F.) ;
#65905=ADVANCED_FACE('',(#18620),#5677,.F.) ;
#65906=ADVANCED_FACE('',(#18621),#7027,.T.) ;
#65907=ADVANCED_FACE('',(#18622),#5678,.F.) ;
#65908=ADVANCED_FACE('',(#18623),#7028,.T.) ;
#65909=ADVANCED_FACE('',(#18624),#5679,.F.) ;
#65910=ADVANCED_FACE('',(#18625),#7029,.F.) ;
#65911=ADVANCED_FACE('',(#18626),#5680,.F.) ;
#65912=ADVANCED_FACE('',(#18627),#7030,.F.) ;
#65913=ADVANCED_FACE('',(#18628),#5681,.F.) ;
#65914=ADVANCED_FACE('',(#18629),#7031,.F.) ;
#65915=ADVANCED_FACE('',(#18630),#7032,.T.) ;
#65916=ADVANCED_FACE('',(#18631),#7033,.F.) ;
#65917=ADVANCED_FACE('',(#18632),#5682,.F.) ;
#65918=ADVANCED_FACE('',(#18633),#7034,.F.) ;
#65919=ADVANCED_FACE('',(#18634),#5683,.F.) ;
#65920=ADVANCED_FACE('',(#18635),#7035,.F.) ;
#65921=ADVANCED_FACE('',(#18636),#5684,.F.) ;
#65922=ADVANCED_FACE('',(#18637,#5047),#5685,.F.) ;
#65923=ADVANCED_FACE('',(#18638),#7036,.T.) ;
#65924=ADVANCED_FACE('',(#18639),#5686,.F.) ;
#65925=ADVANCED_FACE('',(#18640),#7037,.T.) ;
#65926=ADVANCED_FACE('',(#18641),#5687,.F.) ;
#65927=ADVANCED_FACE('',(#18642),#7038,.F.) ;
#65928=ADVANCED_FACE('',(#18643),#5688,.F.) ;
#65929=ADVANCED_FACE('',(#18644),#7039,.F.) ;
#65930=ADVANCED_FACE('',(#18645),#5689,.F.) ;
#65931=ADVANCED_FACE('',(#18646),#5690,.F.) ;
#65932=ADVANCED_FACE('',(#18647),#7040,.F.) ;
#65933=ADVANCED_FACE('',(#18648),#5691,.F.) ;
#65934=ADVANCED_FACE('',(#18649),#7041,.T.) ;
#65935=ADVANCED_FACE('',(#18650),#5692,.F.) ;
#65936=ADVANCED_FACE('',(#18651),#7042,.T.) ;
#65937=ADVANCED_FACE('',(#18652),#5693,.F.) ;
#65938=ADVANCED_FACE('',(#18653),#7043,.F.) ;
#65939=ADVANCED_FACE('',(#18654),#5694,.F.) ;
#65940=ADVANCED_FACE('',(#18655),#7044,.F.) ;
#65941=ADVANCED_FACE('',(#18656),#5695,.F.) ;
#65942=ADVANCED_FACE('',(#18657),#7045,.F.) ;
#65943=ADVANCED_FACE('',(#18658),#7046,.T.) ;
#65944=ADVANCED_FACE('',(#18659),#7047,.F.) ;
#65945=ADVANCED_FACE('',(#18660),#5696,.F.) ;
#65946=ADVANCED_FACE('',(#18661),#7048,.F.) ;
#65947=ADVANCED_FACE('',(#18662),#5697,.F.) ;
#65948=ADVANCED_FACE('',(#18663),#7049,.F.) ;
#65949=ADVANCED_FACE('',(#18664),#5698,.F.) ;
#65950=ADVANCED_FACE('',(#18665,#5048),#5699,.F.) ;
#65951=ADVANCED_FACE('',(#18666),#7050,.T.) ;
#65952=ADVANCED_FACE('',(#18667),#5700,.F.) ;
#65953=ADVANCED_FACE('',(#18668),#7051,.T.) ;
#65954=ADVANCED_FACE('',(#18669),#5701,.F.) ;
#65955=ADVANCED_FACE('',(#18670),#7052,.F.) ;
#65956=ADVANCED_FACE('',(#18671),#5702,.F.) ;
#65957=ADVANCED_FACE('',(#18672),#7053,.F.) ;
#65958=ADVANCED_FACE('',(#18673),#5703,.F.) ;
#65959=ADVANCED_FACE('',(#18674),#5704,.F.) ;
#65960=ADVANCED_FACE('',(#18675),#7054,.F.) ;
#65961=ADVANCED_FACE('',(#18676),#5705,.F.) ;
#65962=ADVANCED_FACE('',(#18677),#7055,.T.) ;
#65963=ADVANCED_FACE('',(#18678),#5706,.F.) ;
#65964=ADVANCED_FACE('',(#18679),#7056,.T.) ;
#65965=ADVANCED_FACE('',(#18680),#5707,.F.) ;
#65966=ADVANCED_FACE('',(#18681),#7057,.F.) ;
#65967=ADVANCED_FACE('',(#18682),#5708,.F.) ;
#65968=ADVANCED_FACE('',(#18683),#7058,.F.) ;
#65969=ADVANCED_FACE('',(#18684),#5709,.F.) ;
#65970=ADVANCED_FACE('',(#18685),#7059,.F.) ;
#65971=ADVANCED_FACE('',(#18686),#7060,.T.) ;
#65972=ADVANCED_FACE('',(#18687),#7061,.F.) ;
#65973=ADVANCED_FACE('',(#18688),#5710,.F.) ;
#65974=ADVANCED_FACE('',(#18689),#7062,.F.) ;
#65975=ADVANCED_FACE('',(#18690),#5711,.F.) ;
#65976=ADVANCED_FACE('',(#18691),#7063,.F.) ;
#65977=ADVANCED_FACE('',(#18692),#5712,.F.) ;
#65978=ADVANCED_FACE('',(#18693,#5049),#5713,.F.) ;
#65979=ADVANCED_FACE('',(#18694),#7064,.T.) ;
#65980=ADVANCED_FACE('',(#18695),#5714,.F.) ;
#65981=ADVANCED_FACE('',(#18696),#7065,.T.) ;
#65982=ADVANCED_FACE('',(#18697),#5715,.F.) ;
#65983=ADVANCED_FACE('',(#18698),#7066,.F.) ;
#65984=ADVANCED_FACE('',(#18699),#5716,.F.) ;
#65985=ADVANCED_FACE('',(#18700),#7067,.F.) ;
#65986=ADVANCED_FACE('',(#18701),#5717,.F.) ;
#65987=ADVANCED_FACE('',(#18702),#5718,.F.) ;
#65988=ADVANCED_FACE('',(#18703),#7068,.F.) ;
#65989=ADVANCED_FACE('',(#18704),#5719,.F.) ;
#65990=ADVANCED_FACE('',(#18705),#7069,.T.) ;
#65991=ADVANCED_FACE('',(#18706),#5720,.F.) ;
#65992=ADVANCED_FACE('',(#18707),#7070,.T.) ;
#65993=ADVANCED_FACE('',(#18708),#5721,.F.) ;
#65994=ADVANCED_FACE('',(#18709),#7071,.F.) ;
#65995=ADVANCED_FACE('',(#18710),#5722,.F.) ;
#65996=ADVANCED_FACE('',(#18711),#7072,.F.) ;
#65997=ADVANCED_FACE('',(#18712),#5723,.F.) ;
#65998=ADVANCED_FACE('',(#18713),#7073,.F.) ;
#65999=ADVANCED_FACE('',(#18714),#7074,.T.) ;
#66000=ADVANCED_FACE('',(#18715),#7075,.F.) ;
#66001=ADVANCED_FACE('',(#18716),#5724,.F.) ;
#66002=ADVANCED_FACE('',(#18717),#7076,.F.) ;
#66003=ADVANCED_FACE('',(#18718),#5725,.F.) ;
#66004=ADVANCED_FACE('',(#18719),#7077,.F.) ;
#66005=ADVANCED_FACE('',(#18720),#5726,.F.) ;
#66006=ADVANCED_FACE('',(#18721,#5050),#5727,.F.) ;
#66007=ADVANCED_FACE('',(#18722),#7078,.T.) ;
#66008=ADVANCED_FACE('',(#18723),#5728,.F.) ;
#66009=ADVANCED_FACE('',(#18724),#7079,.T.) ;
#66010=ADVANCED_FACE('',(#18725),#5729,.F.) ;
#66011=ADVANCED_FACE('',(#18726),#7080,.F.) ;
#66012=ADVANCED_FACE('',(#18727),#5730,.F.) ;
#66013=ADVANCED_FACE('',(#18728),#7081,.F.) ;
#66014=ADVANCED_FACE('',(#18729),#5731,.F.) ;
#66015=ADVANCED_FACE('',(#18730),#5732,.F.) ;
#66016=ADVANCED_FACE('',(#18731),#7082,.F.) ;
#66017=ADVANCED_FACE('',(#18732),#5733,.F.) ;
#66018=ADVANCED_FACE('',(#18733),#7083,.T.) ;
#66019=ADVANCED_FACE('',(#18734),#5734,.F.) ;
#66020=ADVANCED_FACE('',(#18735),#7084,.T.) ;
#66021=ADVANCED_FACE('',(#18736),#5735,.F.) ;
#66022=ADVANCED_FACE('',(#18737),#7085,.F.) ;
#66023=ADVANCED_FACE('',(#18738),#5736,.F.) ;
#66024=ADVANCED_FACE('',(#18739),#7086,.F.) ;
#66025=ADVANCED_FACE('',(#18740),#5737,.F.) ;
#66026=ADVANCED_FACE('',(#18741),#7087,.F.) ;
#66027=ADVANCED_FACE('',(#18742),#7088,.T.) ;
#66028=ADVANCED_FACE('',(#18743),#7089,.F.) ;
#66029=ADVANCED_FACE('',(#18744),#5738,.F.) ;
#66030=ADVANCED_FACE('',(#18745),#7090,.F.) ;
#66031=ADVANCED_FACE('',(#18746),#5739,.F.) ;
#66032=ADVANCED_FACE('',(#18747),#7091,.F.) ;
#66033=ADVANCED_FACE('',(#18748),#5740,.F.) ;
#66034=ADVANCED_FACE('',(#18749,#5051),#5741,.F.) ;
#66035=ADVANCED_FACE('',(#18750,#5052),#5742,.T.) ;
#66036=ADVANCED_FACE('',(#18751,#5053),#5743,.T.) ;
#66037=ADVANCED_FACE('',(#18752,#5054),#5744,.T.) ;
#66038=ADVANCED_FACE('',(#18753,#5055),#5745,.T.) ;
#66039=ADVANCED_FACE('',(#18754,#5056),#5746,.T.) ;
#66040=ADVANCED_FACE('',(#18755,#5057),#5747,.T.) ;
#66041=ADVANCED_FACE('',(#18756,#5058),#5748,.T.) ;
#66042=ADVANCED_FACE('',(#18757,#5059),#5749,.T.) ;
#66043=ADVANCED_FACE('',(#18758,#5060),#5750,.T.) ;
#66044=ADVANCED_FACE('',(#18759),#7092,.T.) ;
#66045=ADVANCED_FACE('',(#18760),#7093,.F.) ;
#66046=ADVANCED_FACE('',(#18761),#4488,.F.) ;
#66047=ADVANCED_FACE('',(#18762),#4489,.T.) ;
#66048=ADVANCED_FACE('',(#18763),#63180,.T.) ;
#66049=ADVANCED_FACE('',(#18764),#7094,.F.) ;
#66050=ADVANCED_FACE('',(#18765),#7095,.F.) ;
#66051=ADVANCED_FACE('',(#18766),#7096,.T.) ;
#66052=ADVANCED_FACE('',(#18767),#7097,.T.) ;
#66053=ADVANCED_FACE('',(#18768),#7098,.T.) ;
#66054=ADVANCED_FACE('',(#18769),#7099,.F.) ;
#66055=ADVANCED_FACE('',(#18770),#4490,.F.) ;
#66056=ADVANCED_FACE('',(#18771),#63181,.F.) ;
#66057=ADVANCED_FACE('',(#18772),#63182,.F.) ;
#66058=ADVANCED_FACE('',(#18773),#63183,.T.) ;
#66059=ADVANCED_FACE('',(#18774),#7100,.F.) ;
#66060=ADVANCED_FACE('',(#18775),#7101,.F.) ;
#66061=ADVANCED_FACE('',(#18776),#7102,.F.) ;
#66062=ADVANCED_FACE('',(#18777),#7103,.T.) ;
#66063=ADVANCED_FACE('',(#18778),#7104,.T.) ;
#66064=ADVANCED_FACE('',(#18779),#63184,.F.) ;
#66065=ADVANCED_FACE('',(#18780),#4491,.F.) ;
#66066=ADVANCED_FACE('',(#18781),#4492,.T.) ;
#66067=ADVANCED_FACE('',(#18782),#7105,.T.) ;
#66068=ADVANCED_FACE('',(#18783),#4493,.F.) ;
#66069=ADVANCED_FACE('',(#18784),#4494,.T.) ;
#66070=ADVANCED_FACE('',(#18785),#7106,.F.) ;
#66071=ADVANCED_FACE('',(#18786),#7107,.F.) ;
#66072=ADVANCED_FACE('',(#18787),#7108,.T.) ;
#66073=ADVANCED_FACE('',(#18788),#63185,.T.) ;
#66074=ADVANCED_FACE('',(#18789),#7109,.F.) ;
#66075=ADVANCED_FACE('',(#18790),#7110,.T.) ;
#66076=ADVANCED_FACE('',(#18791),#7111,.F.) ;
#66077=ADVANCED_FACE('',(#18792),#4495,.F.) ;
#66078=ADVANCED_FACE('',(#18793),#63186,.T.) ;
#66079=ADVANCED_FACE('',(#18794),#7112,.T.) ;
#66080=ADVANCED_FACE('',(#18795),#4496,.F.) ;
#66081=ADVANCED_FACE('',(#18796),#63187,.F.) ;
#66082=ADVANCED_FACE('',(#18797),#7113,.F.) ;
#66083=ADVANCED_FACE('',(#18798),#7114,.T.) ;
#66084=ADVANCED_FACE('',(#18799),#63188,.T.) ;
#66085=ADVANCED_FACE('',(#18800),#7115,.F.) ;
#66086=ADVANCED_FACE('',(#18801),#63189,.T.) ;
#66087=ADVANCED_FACE('',(#18802),#7116,.T.) ;
#66088=ADVANCED_FACE('',(#18803),#7117,.T.) ;
#66089=ADVANCED_FACE('',(#18804),#4497,.T.) ;
#66090=ADVANCED_FACE('',(#18805),#7118,.F.) ;
#66091=ADVANCED_FACE('',(#18806),#63190,.F.) ;
#66092=ADVANCED_FACE('',(#18807),#4498,.F.) ;
#66093=ADVANCED_FACE('',(#18808),#7119,.F.) ;
#66094=ADVANCED_FACE('',(#18809),#7120,.F.) ;
#66095=ADVANCED_FACE('',(#18810),#63191,.F.) ;
#66096=ADVANCED_FACE('',(#18811),#4499,.F.) ;
#66097=ADVANCED_FACE('',(#18812),#7121,.F.) ;
#66098=ADVANCED_FACE('',(#18813),#7122,.F.) ;
#66099=ADVANCED_FACE('',(#18814),#4500,.F.) ;
#66100=ADVANCED_FACE('',(#18815),#4501,.F.) ;
#66101=ADVANCED_FACE('',(#18816),#7123,.F.) ;
#66102=ADVANCED_FACE('',(#18817),#63192,.F.) ;
#66103=ADVANCED_FACE('',(#18818),#4502,.F.) ;
#66104=ADVANCED_FACE('',(#18819),#4503,.F.) ;
#66105=ADVANCED_FACE('',(#18820),#7124,.F.) ;
#66106=ADVANCED_FACE('',(#18821),#7125,.F.) ;
#66107=ADVANCED_FACE('',(#18822),#4504,.F.) ;
#66108=ADVANCED_FACE('',(#18823),#7126,.F.) ;
#66109=ADVANCED_FACE('',(#18824),#7127,.F.) ;
#66110=ADVANCED_FACE('',(#18825),#4505,.F.) ;
#66111=ADVANCED_FACE('',(#18826),#4506,.F.) ;
#66112=ADVANCED_FACE('',(#18827),#7128,.F.) ;
#66113=ADVANCED_FACE('',(#18828),#7129,.F.) ;
#66114=ADVANCED_FACE('',(#18829),#63193,.F.) ;
#66115=ADVANCED_FACE('',(#18830),#63194,.F.) ;
#66116=ADVANCED_FACE('',(#18831),#7130,.F.) ;
#66117=ADVANCED_FACE('',(#18832),#7131,.T.) ;
#66118=ADVANCED_FACE('',(#18833),#4507,.T.) ;
#66119=ADVANCED_FACE('',(#18834),#4508,.T.) ;
#66120=ADVANCED_FACE('',(#18835),#7132,.T.) ;
#66121=ADVANCED_FACE('',(#18836),#7133,.T.) ;
#66122=ADVANCED_FACE('',(#18837),#63195,.T.) ;
#66123=ADVANCED_FACE('',(#18838),#63196,.T.) ;
#66124=ADVANCED_FACE('',(#18839),#7134,.T.) ;
#66125=ADVANCED_FACE('',(#18840),#7135,.T.) ;
#66126=ADVANCED_FACE('',(#18841),#63197,.T.) ;
#66127=ADVANCED_FACE('',(#18842),#7136,.T.) ;
#66128=ADVANCED_FACE('',(#18843),#7137,.T.) ;
#66129=ADVANCED_FACE('',(#18844),#63198,.T.) ;
#66130=ADVANCED_FACE('',(#18845),#63199,.T.) ;
#66131=ADVANCED_FACE('',(#18846),#7138,.T.) ;
#66132=ADVANCED_FACE('',(#18847),#63200,.T.) ;
#66133=ADVANCED_FACE('',(#18848),#63201,.T.) ;
#66134=ADVANCED_FACE('',(#18849),#63202,.T.) ;
#66135=ADVANCED_FACE('',(#18850),#7139,.T.) ;
#66136=ADVANCED_FACE('',(#18851),#7140,.T.) ;
#66137=ADVANCED_FACE('',(#18852),#4509,.T.) ;
#66138=ADVANCED_FACE('',(#18853),#63203,.T.) ;
#66139=ADVANCED_FACE('',(#18854),#7141,.T.) ;
#66140=ADVANCED_FACE('',(#18855),#7142,.T.) ;
#66141=ADVANCED_FACE('',(#18856),#4510,.T.) ;
#66142=ADVANCED_FACE('',(#18857),#63204,.T.) ;
#66143=ADVANCED_FACE('',(#18858),#7143,.T.) ;
#66144=ADVANCED_FACE('',(#18859),#7144,.T.) ;
#66145=ADVANCED_FACE('',(#18860),#4511,.T.) ;
#66146=ADVANCED_FACE('',(#18861),#4512,.T.) ;
#66147=ADVANCED_FACE('',(#18862),#7145,.T.) ;
#66148=ADVANCED_FACE('',(#18863),#7146,.T.) ;
#66149=ADVANCED_FACE('',(#18864),#63205,.T.) ;
#66150=ADVANCED_FACE('',(#18865),#63206,.T.) ;
#66151=ADVANCED_FACE('',(#18866),#7147,.T.) ;
#66152=ADVANCED_FACE('',(#18867),#7148,.T.) ;
#66153=ADVANCED_FACE('',(#18868),#63207,.T.) ;
#66154=ADVANCED_FACE('',(#18869),#7149,.T.) ;
#66155=ADVANCED_FACE('',(#18870),#7150,.T.) ;
#66156=ADVANCED_FACE('',(#18871),#63208,.T.) ;
#66157=ADVANCED_FACE('',(#18872),#63209,.T.) ;
#66158=ADVANCED_FACE('',(#18873),#7151,.T.) ;
#66159=ADVANCED_FACE('',(#18874),#63210,.T.) ;
#66160=ADVANCED_FACE('',(#18875),#63211,.T.) ;
#66161=ADVANCED_FACE('',(#18876),#63212,.T.) ;
#66162=ADVANCED_FACE('',(#18877),#7152,.T.) ;
#66163=ADVANCED_FACE('',(#18878),#7153,.T.) ;
#66164=ADVANCED_FACE('',(#18879),#4513,.T.) ;
#66165=ADVANCED_FACE('',(#18880),#63213,.T.) ;
#66166=ADVANCED_FACE('',(#18881),#7154,.T.) ;
#66167=ADVANCED_FACE('',(#18882),#7155,.T.) ;
#66168=ADVANCED_FACE('',(#18883),#4514,.T.) ;
#66169=ADVANCED_FACE('',(#18884),#63214,.T.) ;
#66170=ADVANCED_FACE('',(#18885),#7156,.T.) ;
#66171=ADVANCED_FACE('',(#18886),#7157,.T.) ;
#66172=ADVANCED_FACE('',(#18887),#4515,.T.) ;
#66173=ADVANCED_FACE('',(#18888),#4516,.T.) ;
#66174=ADVANCED_FACE('',(#18889),#7158,.T.) ;
#66175=ADVANCED_FACE('',(#18890),#7159,.T.) ;
#66176=ADVANCED_FACE('',(#18891),#63215,.T.) ;
#66177=ADVANCED_FACE('',(#18892),#63216,.T.) ;
#66178=ADVANCED_FACE('',(#18893),#7160,.T.) ;
#66179=ADVANCED_FACE('',(#18894),#7161,.T.) ;
#66180=ADVANCED_FACE('',(#18895),#63217,.T.) ;
#66181=ADVANCED_FACE('',(#18896),#7162,.T.) ;
#66182=ADVANCED_FACE('',(#18897),#7163,.T.) ;
#66183=ADVANCED_FACE('',(#18898),#63218,.T.) ;
#66184=ADVANCED_FACE('',(#18899),#63219,.T.) ;
#66185=ADVANCED_FACE('',(#18900),#7164,.T.) ;
#66186=ADVANCED_FACE('',(#18901),#63220,.T.) ;
#66187=ADVANCED_FACE('',(#18902),#63221,.T.) ;
#66188=ADVANCED_FACE('',(#18903),#63222,.T.) ;
#66189=ADVANCED_FACE('',(#18904),#7165,.T.) ;
#66190=ADVANCED_FACE('',(#18905),#7166,.T.) ;
#66191=ADVANCED_FACE('',(#18906),#4517,.T.) ;
#66192=ADVANCED_FACE('',(#18907),#63223,.T.) ;
#66193=ADVANCED_FACE('',(#18908),#7167,.T.) ;
#66194=ADVANCED_FACE('',(#18909),#7168,.T.) ;
#66195=ADVANCED_FACE('',(#18910),#4518,.T.) ;
#66196=ADVANCED_FACE('',(#18911),#63224,.T.) ;
#66197=ADVANCED_FACE('',(#18912),#7169,.T.) ;
#66198=ADVANCED_FACE('',(#18913),#7170,.T.) ;
#66199=ADVANCED_FACE('',(#18914),#4519,.T.) ;
#66200=ADVANCED_FACE('',(#18915),#4520,.T.) ;
#66201=ADVANCED_FACE('',(#18916),#7171,.T.) ;
#66202=ADVANCED_FACE('',(#18917),#7172,.T.) ;
#66203=ADVANCED_FACE('',(#18918),#63225,.T.) ;
#66204=ADVANCED_FACE('',(#18919),#63226,.T.) ;
#66205=ADVANCED_FACE('',(#18920),#7173,.T.) ;
#66206=ADVANCED_FACE('',(#18921),#7174,.T.) ;
#66207=ADVANCED_FACE('',(#18922),#63227,.T.) ;
#66208=ADVANCED_FACE('',(#18923),#7175,.T.) ;
#66209=ADVANCED_FACE('',(#18924),#7176,.T.) ;
#66210=ADVANCED_FACE('',(#18925),#63228,.T.) ;
#66211=ADVANCED_FACE('',(#18926),#63229,.T.) ;
#66212=ADVANCED_FACE('',(#18927),#7177,.T.) ;
#66213=ADVANCED_FACE('',(#18928),#63230,.T.) ;
#66214=ADVANCED_FACE('',(#18929),#63231,.T.) ;
#66215=ADVANCED_FACE('',(#18930),#63232,.T.) ;
#66216=ADVANCED_FACE('',(#18931),#7178,.T.) ;
#66217=ADVANCED_FACE('',(#18932),#7179,.T.) ;
#66218=ADVANCED_FACE('',(#18933),#4521,.T.) ;
#66219=ADVANCED_FACE('',(#18934),#63233,.T.) ;
#66220=ADVANCED_FACE('',(#18935),#7180,.T.) ;
#66221=ADVANCED_FACE('',(#18936),#7181,.T.) ;
#66222=ADVANCED_FACE('',(#18937),#4522,.T.) ;
#66223=ADVANCED_FACE('',(#18938),#63234,.T.) ;
#66224=ADVANCED_FACE('',(#18939),#7182,.T.) ;
#66225=ADVANCED_FACE('',(#18940),#7183,.T.) ;
#66226=ADVANCED_FACE('',(#18941),#4523,.T.) ;
#66227=ADVANCED_FACE('',(#18942),#4524,.T.) ;
#66228=ADVANCED_FACE('',(#18943),#7184,.T.) ;
#66229=ADVANCED_FACE('',(#18944),#7185,.T.) ;
#66230=ADVANCED_FACE('',(#18945),#63235,.T.) ;
#66231=ADVANCED_FACE('',(#18946),#63236,.T.) ;
#66232=ADVANCED_FACE('',(#18947),#7186,.T.) ;
#66233=ADVANCED_FACE('',(#18948),#7187,.T.) ;
#66234=ADVANCED_FACE('',(#18949),#63237,.T.) ;
#66235=ADVANCED_FACE('',(#18950),#7188,.T.) ;
#66236=ADVANCED_FACE('',(#18951),#7189,.T.) ;
#66237=ADVANCED_FACE('',(#18952),#63238,.T.) ;
#66238=ADVANCED_FACE('',(#18953),#63239,.T.) ;
#66239=ADVANCED_FACE('',(#18954),#7190,.T.) ;
#66240=ADVANCED_FACE('',(#18955),#63240,.T.) ;
#66241=ADVANCED_FACE('',(#18956),#63241,.T.) ;
#66242=ADVANCED_FACE('',(#18957),#63242,.T.) ;
#66243=ADVANCED_FACE('',(#18958),#7191,.T.) ;
#66244=ADVANCED_FACE('',(#18959),#7192,.T.) ;
#66245=ADVANCED_FACE('',(#18960),#4525,.T.) ;
#66246=ADVANCED_FACE('',(#18961),#63243,.T.) ;
#66247=ADVANCED_FACE('',(#18962),#7193,.T.) ;
#66248=ADVANCED_FACE('',(#18963),#7194,.T.) ;
#66249=ADVANCED_FACE('',(#18964),#4526,.T.) ;
#66250=ADVANCED_FACE('',(#18965),#63244,.T.) ;
#66251=ADVANCED_FACE('',(#18966),#7195,.T.) ;
#66252=ADVANCED_FACE('',(#18967),#7196,.T.) ;
#66253=ADVANCED_FACE('',(#18968),#4527,.T.) ;
#66254=ADVANCED_FACE('',(#18969),#4528,.T.) ;
#66255=ADVANCED_FACE('',(#18970),#7197,.T.) ;
#66256=ADVANCED_FACE('',(#18971),#7198,.T.) ;
#66257=ADVANCED_FACE('',(#18972),#63245,.T.) ;
#66258=ADVANCED_FACE('',(#18973),#63246,.T.) ;
#66259=ADVANCED_FACE('',(#18974),#7199,.T.) ;
#66260=ADVANCED_FACE('',(#18975),#7200,.T.) ;
#66261=ADVANCED_FACE('',(#18976),#63247,.T.) ;
#66262=ADVANCED_FACE('',(#18977),#7201,.T.) ;
#66263=ADVANCED_FACE('',(#18978),#7202,.T.) ;
#66264=ADVANCED_FACE('',(#18979),#63248,.T.) ;
#66265=ADVANCED_FACE('',(#18980),#63249,.T.) ;
#66266=ADVANCED_FACE('',(#18981),#7203,.T.) ;
#66267=ADVANCED_FACE('',(#18982),#63250,.T.) ;
#66268=ADVANCED_FACE('',(#18983),#63251,.T.) ;
#66269=ADVANCED_FACE('',(#18984),#63252,.T.) ;
#66270=ADVANCED_FACE('',(#18985),#7204,.T.) ;
#66271=ADVANCED_FACE('',(#18986),#7205,.T.) ;
#66272=ADVANCED_FACE('',(#18987),#4529,.T.) ;
#66273=ADVANCED_FACE('',(#18988),#63253,.T.) ;
#66274=ADVANCED_FACE('',(#18989),#7206,.T.) ;
#66275=ADVANCED_FACE('',(#18990),#7207,.T.) ;
#66276=ADVANCED_FACE('',(#18991),#4530,.T.) ;
#66277=ADVANCED_FACE('',(#18992),#63254,.T.) ;
#66278=ADVANCED_FACE('',(#18993),#7208,.T.) ;
#66279=ADVANCED_FACE('',(#18994),#7209,.T.) ;
#66280=ADVANCED_FACE('',(#18995),#4531,.T.) ;
#66281=ADVANCED_FACE('',(#18996),#4532,.T.) ;
#66282=ADVANCED_FACE('',(#18997),#7210,.T.) ;
#66283=ADVANCED_FACE('',(#18998),#7211,.T.) ;
#66284=ADVANCED_FACE('',(#18999),#63255,.T.) ;
#66285=ADVANCED_FACE('',(#19000),#63256,.T.) ;
#66286=ADVANCED_FACE('',(#19001),#7212,.T.) ;
#66287=ADVANCED_FACE('',(#19002),#7213,.T.) ;
#66288=ADVANCED_FACE('',(#19003),#63257,.T.) ;
#66289=ADVANCED_FACE('',(#19004),#7214,.T.) ;
#66290=ADVANCED_FACE('',(#19005),#7215,.T.) ;
#66291=ADVANCED_FACE('',(#19006),#63258,.T.) ;
#66292=ADVANCED_FACE('',(#19007),#63259,.T.) ;
#66293=ADVANCED_FACE('',(#19008),#7216,.T.) ;
#66294=ADVANCED_FACE('',(#19009),#63260,.T.) ;
#66295=ADVANCED_FACE('',(#19010),#63261,.T.) ;
#66296=ADVANCED_FACE('',(#19011),#63262,.T.) ;
#66297=ADVANCED_FACE('',(#19012),#7217,.T.) ;
#66298=ADVANCED_FACE('',(#19013),#7218,.T.) ;
#66299=ADVANCED_FACE('',(#19014),#4533,.T.) ;
#66300=ADVANCED_FACE('',(#19015),#63263,.T.) ;
#66301=ADVANCED_FACE('',(#19016),#7219,.T.) ;
#66302=ADVANCED_FACE('',(#19017),#7220,.T.) ;
#66303=ADVANCED_FACE('',(#19018),#4534,.T.) ;
#66304=ADVANCED_FACE('',(#19019),#63264,.T.) ;
#66305=ADVANCED_FACE('',(#19020),#7221,.T.) ;
#66306=ADVANCED_FACE('',(#19021),#7222,.T.) ;
#66307=ADVANCED_FACE('',(#19022),#4535,.T.) ;
#66308=ADVANCED_FACE('',(#19023),#4536,.T.) ;
#66309=ADVANCED_FACE('',(#19024),#7223,.T.) ;
#66310=ADVANCED_FACE('',(#19025),#7224,.T.) ;
#66311=ADVANCED_FACE('',(#19026),#63265,.T.) ;
#66312=ADVANCED_FACE('',(#19027),#63266,.T.) ;
#66313=ADVANCED_FACE('',(#19028),#7225,.T.) ;
#66314=ADVANCED_FACE('',(#19029),#7226,.T.) ;
#66315=ADVANCED_FACE('',(#19030),#63267,.T.) ;
#66316=ADVANCED_FACE('',(#19031),#7227,.T.) ;
#66317=ADVANCED_FACE('',(#19032),#7228,.T.) ;
#66318=ADVANCED_FACE('',(#19033),#63268,.T.) ;
#66319=ADVANCED_FACE('',(#19034),#63269,.T.) ;
#66320=ADVANCED_FACE('',(#19035),#7229,.T.) ;
#66321=ADVANCED_FACE('',(#19036),#63270,.T.) ;
#66322=ADVANCED_FACE('',(#19037),#63271,.T.) ;
#66323=ADVANCED_FACE('',(#19038),#63272,.T.) ;
#66324=ADVANCED_FACE('',(#19039),#7230,.T.) ;
#66325=ADVANCED_FACE('',(#19040),#7231,.T.) ;
#66326=ADVANCED_FACE('',(#19041),#4537,.T.) ;
#66327=ADVANCED_FACE('',(#19042),#63273,.T.) ;
#66328=ADVANCED_FACE('',(#19043),#7232,.T.) ;
#66329=ADVANCED_FACE('',(#19044),#7233,.T.) ;
#66330=ADVANCED_FACE('',(#19045),#4538,.T.) ;
#66331=ADVANCED_FACE('',(#19046),#63274,.T.) ;
#66332=ADVANCED_FACE('',(#19047),#7234,.T.) ;
#66333=ADVANCED_FACE('',(#19048),#7235,.T.) ;
#66334=ADVANCED_FACE('',(#19049),#4539,.T.) ;
#66335=ADVANCED_FACE('',(#19050),#4540,.T.) ;
#66336=ADVANCED_FACE('',(#19051),#7236,.T.) ;
#66337=ADVANCED_FACE('',(#19052),#7237,.T.) ;
#66338=ADVANCED_FACE('',(#19053),#63275,.T.) ;
#66339=ADVANCED_FACE('',(#19054),#63276,.T.) ;
#66340=ADVANCED_FACE('',(#19055),#7238,.T.) ;
#66341=ADVANCED_FACE('',(#19056),#7239,.T.) ;
#66342=ADVANCED_FACE('',(#19057),#63277,.T.) ;
#66343=ADVANCED_FACE('',(#19058),#7240,.T.) ;
#66344=ADVANCED_FACE('',(#19059),#7241,.T.) ;
#66345=ADVANCED_FACE('',(#19060),#63278,.T.) ;
#66346=ADVANCED_FACE('',(#19061),#63279,.T.) ;
#66347=ADVANCED_FACE('',(#19062),#7242,.T.) ;
#66348=ADVANCED_FACE('',(#19063),#63280,.T.) ;
#66349=ADVANCED_FACE('',(#19064),#63281,.T.) ;
#66350=ADVANCED_FACE('',(#19065),#63282,.T.) ;
#66351=ADVANCED_FACE('',(#19066),#7243,.T.) ;
#66352=ADVANCED_FACE('',(#19067),#7244,.T.) ;
#66353=ADVANCED_FACE('',(#19068),#4541,.T.) ;
#66354=ADVANCED_FACE('',(#19069),#63283,.T.) ;
#66355=ADVANCED_FACE('',(#19070),#7245,.T.) ;
#66356=ADVANCED_FACE('',(#19071),#7246,.T.) ;
#66357=ADVANCED_FACE('',(#19072),#4542,.T.) ;
#66358=ADVANCED_FACE('',(#19073),#63284,.T.) ;
#66359=ADVANCED_FACE('',(#19074),#7247,.T.) ;
#66360=ADVANCED_FACE('',(#19075),#7248,.T.) ;
#66361=ADVANCED_FACE('',(#19076),#7249,.F.) ;
#66362=ADVANCED_FACE('',(#19077),#4543,.F.) ;
#66363=ADVANCED_FACE('',(#19078),#4544,.T.) ;
#66364=ADVANCED_FACE('',(#19079),#63285,.T.) ;
#66365=ADVANCED_FACE('',(#19080),#7250,.F.) ;
#66366=ADVANCED_FACE('',(#19081),#7251,.F.) ;
#66367=ADVANCED_FACE('',(#19082),#7252,.T.) ;
#66368=ADVANCED_FACE('',(#19083),#7253,.T.) ;
#66369=ADVANCED_FACE('',(#19084),#7254,.T.) ;
#66370=ADVANCED_FACE('',(#19085),#7255,.F.) ;
#66371=ADVANCED_FACE('',(#19086),#4545,.F.) ;
#66372=ADVANCED_FACE('',(#19087),#63286,.F.) ;
#66373=ADVANCED_FACE('',(#19088),#63287,.F.) ;
#66374=ADVANCED_FACE('',(#19089),#63288,.T.) ;
#66375=ADVANCED_FACE('',(#19090),#7256,.F.) ;
#66376=ADVANCED_FACE('',(#19091),#7257,.F.) ;
#66377=ADVANCED_FACE('',(#19092),#7258,.F.) ;
#66378=ADVANCED_FACE('',(#19093),#7259,.T.) ;
#66379=ADVANCED_FACE('',(#19094),#7260,.T.) ;
#66380=ADVANCED_FACE('',(#19095),#63289,.F.) ;
#66381=ADVANCED_FACE('',(#19096),#4546,.F.) ;
#66382=ADVANCED_FACE('',(#19097),#4547,.T.) ;
#66383=ADVANCED_FACE('',(#19098),#7261,.T.) ;
#66384=ADVANCED_FACE('',(#19099),#4548,.F.) ;
#66385=ADVANCED_FACE('',(#19100),#4549,.T.) ;
#66386=ADVANCED_FACE('',(#19101),#7262,.F.) ;
#66387=ADVANCED_FACE('',(#19102),#7263,.F.) ;
#66388=ADVANCED_FACE('',(#19103),#7264,.T.) ;
#66389=ADVANCED_FACE('',(#19104),#63290,.T.) ;
#66390=ADVANCED_FACE('',(#19105),#7265,.F.) ;
#66391=ADVANCED_FACE('',(#19106),#7266,.T.) ;
#66392=ADVANCED_FACE('',(#19107),#7267,.F.) ;
#66393=ADVANCED_FACE('',(#19108),#4550,.F.) ;
#66394=ADVANCED_FACE('',(#19109),#63291,.T.) ;
#66395=ADVANCED_FACE('',(#19110),#7268,.T.) ;
#66396=ADVANCED_FACE('',(#19111),#4551,.F.) ;
#66397=ADVANCED_FACE('',(#19112),#63292,.F.) ;
#66398=ADVANCED_FACE('',(#19113),#7269,.F.) ;
#66399=ADVANCED_FACE('',(#19114),#7270,.T.) ;
#66400=ADVANCED_FACE('',(#19115),#63293,.T.) ;
#66401=ADVANCED_FACE('',(#19116),#7271,.F.) ;
#66402=ADVANCED_FACE('',(#19117),#63294,.T.) ;
#66403=ADVANCED_FACE('',(#19118),#7272,.T.) ;
#66404=ADVANCED_FACE('',(#19119),#7273,.T.) ;
#66405=ADVANCED_FACE('',(#19120),#4552,.T.) ;
#66406=ADVANCED_FACE('',(#19121),#7274,.F.) ;
#66407=ADVANCED_FACE('',(#19122),#63295,.F.) ;
#66408=ADVANCED_FACE('',(#19123),#4553,.F.) ;
#66409=ADVANCED_FACE('',(#19124),#7275,.F.) ;
#66410=ADVANCED_FACE('',(#19125),#7276,.F.) ;
#66411=ADVANCED_FACE('',(#19126),#63296,.F.) ;
#66412=ADVANCED_FACE('',(#19127),#4554,.F.) ;
#66413=ADVANCED_FACE('',(#19128),#7277,.F.) ;
#66414=ADVANCED_FACE('',(#19129),#7278,.F.) ;
#66415=ADVANCED_FACE('',(#19130),#4555,.F.) ;
#66416=ADVANCED_FACE('',(#19131),#4556,.F.) ;
#66417=ADVANCED_FACE('',(#19132),#7279,.F.) ;
#66418=ADVANCED_FACE('',(#19133),#63297,.F.) ;
#66419=ADVANCED_FACE('',(#19134),#4557,.F.) ;
#66420=ADVANCED_FACE('',(#19135),#4558,.F.) ;
#66421=ADVANCED_FACE('',(#19136),#7280,.F.) ;
#66422=ADVANCED_FACE('',(#19137),#7281,.F.) ;
#66423=ADVANCED_FACE('',(#19138),#4559,.F.) ;
#66424=ADVANCED_FACE('',(#19139),#7282,.F.) ;
#66425=ADVANCED_FACE('',(#19140),#7283,.F.) ;
#66426=ADVANCED_FACE('',(#19141),#4560,.F.) ;
#66427=ADVANCED_FACE('',(#19142),#4561,.F.) ;
#66428=ADVANCED_FACE('',(#19143),#7284,.F.) ;
#66429=ADVANCED_FACE('',(#19144),#7285,.F.) ;
#66430=ADVANCED_FACE('',(#19145),#63298,.F.) ;
#66431=ADVANCED_FACE('',(#19146),#63299,.F.) ;
#66432=ADVANCED_FACE('',(#19147),#7286,.F.) ;
#66433=ADVANCED_FACE('',(#19148),#7287,.T.) ;
#66434=ADVANCED_FACE('',(#19149),#7288,.F.) ;
#66435=ADVANCED_FACE('',(#19150),#4562,.F.) ;
#66436=ADVANCED_FACE('',(#19151),#4563,.T.) ;
#66437=ADVANCED_FACE('',(#19152),#63300,.T.) ;
#66438=ADVANCED_FACE('',(#19153),#7289,.F.) ;
#66439=ADVANCED_FACE('',(#19154),#7290,.F.) ;
#66440=ADVANCED_FACE('',(#19155),#7291,.T.) ;
#66441=ADVANCED_FACE('',(#19156),#7292,.T.) ;
#66442=ADVANCED_FACE('',(#19157),#7293,.T.) ;
#66443=ADVANCED_FACE('',(#19158),#7294,.F.) ;
#66444=ADVANCED_FACE('',(#19159),#4564,.F.) ;
#66445=ADVANCED_FACE('',(#19160),#63301,.F.) ;
#66446=ADVANCED_FACE('',(#19161),#63302,.F.) ;
#66447=ADVANCED_FACE('',(#19162),#63303,.T.) ;
#66448=ADVANCED_FACE('',(#19163),#7295,.F.) ;
#66449=ADVANCED_FACE('',(#19164),#7296,.F.) ;
#66450=ADVANCED_FACE('',(#19165),#7297,.F.) ;
#66451=ADVANCED_FACE('',(#19166),#7298,.T.) ;
#66452=ADVANCED_FACE('',(#19167),#7299,.T.) ;
#66453=ADVANCED_FACE('',(#19168),#63304,.F.) ;
#66454=ADVANCED_FACE('',(#19169),#4565,.F.) ;
#66455=ADVANCED_FACE('',(#19170),#4566,.T.) ;
#66456=ADVANCED_FACE('',(#19171),#7300,.T.) ;
#66457=ADVANCED_FACE('',(#19172),#4567,.F.) ;
#66458=ADVANCED_FACE('',(#19173),#4568,.T.) ;
#66459=ADVANCED_FACE('',(#19174),#7301,.F.) ;
#66460=ADVANCED_FACE('',(#19175),#7302,.F.) ;
#66461=ADVANCED_FACE('',(#19176),#7303,.T.) ;
#66462=ADVANCED_FACE('',(#19177),#63305,.T.) ;
#66463=ADVANCED_FACE('',(#19178),#7304,.F.) ;
#66464=ADVANCED_FACE('',(#19179),#7305,.T.) ;
#66465=ADVANCED_FACE('',(#19180),#7306,.F.) ;
#66466=ADVANCED_FACE('',(#19181),#4569,.F.) ;
#66467=ADVANCED_FACE('',(#19182),#63306,.T.) ;
#66468=ADVANCED_FACE('',(#19183),#7307,.T.) ;
#66469=ADVANCED_FACE('',(#19184),#4570,.F.) ;
#66470=ADVANCED_FACE('',(#19185),#63307,.F.) ;
#66471=ADVANCED_FACE('',(#19186),#7308,.F.) ;
#66472=ADVANCED_FACE('',(#19187),#7309,.T.) ;
#66473=ADVANCED_FACE('',(#19188),#63308,.T.) ;
#66474=ADVANCED_FACE('',(#19189),#7310,.F.) ;
#66475=ADVANCED_FACE('',(#19190),#63309,.T.) ;
#66476=ADVANCED_FACE('',(#19191),#7311,.T.) ;
#66477=ADVANCED_FACE('',(#19192),#7312,.T.) ;
#66478=ADVANCED_FACE('',(#19193),#4571,.T.) ;
#66479=ADVANCED_FACE('',(#19194),#7313,.F.) ;
#66480=ADVANCED_FACE('',(#19195),#63310,.F.) ;
#66481=ADVANCED_FACE('',(#19196),#4572,.F.) ;
#66482=ADVANCED_FACE('',(#19197),#7314,.F.) ;
#66483=ADVANCED_FACE('',(#19198),#7315,.F.) ;
#66484=ADVANCED_FACE('',(#19199),#63311,.F.) ;
#66485=ADVANCED_FACE('',(#19200),#4573,.F.) ;
#66486=ADVANCED_FACE('',(#19201),#7316,.F.) ;
#66487=ADVANCED_FACE('',(#19202),#7317,.F.) ;
#66488=ADVANCED_FACE('',(#19203),#4574,.F.) ;
#66489=ADVANCED_FACE('',(#19204),#4575,.F.) ;
#66490=ADVANCED_FACE('',(#19205),#7318,.F.) ;
#66491=ADVANCED_FACE('',(#19206),#63312,.F.) ;
#66492=ADVANCED_FACE('',(#19207),#4576,.F.) ;
#66493=ADVANCED_FACE('',(#19208),#4577,.F.) ;
#66494=ADVANCED_FACE('',(#19209),#7319,.F.) ;
#66495=ADVANCED_FACE('',(#19210),#7320,.F.) ;
#66496=ADVANCED_FACE('',(#19211),#4578,.F.) ;
#66497=ADVANCED_FACE('',(#19212),#7321,.F.) ;
#66498=ADVANCED_FACE('',(#19213),#7322,.F.) ;
#66499=ADVANCED_FACE('',(#19214),#4579,.F.) ;
#66500=ADVANCED_FACE('',(#19215),#4580,.F.) ;
#66501=ADVANCED_FACE('',(#19216),#7323,.F.) ;
#66502=ADVANCED_FACE('',(#19217),#7324,.F.) ;
#66503=ADVANCED_FACE('',(#19218),#63313,.F.) ;
#66504=ADVANCED_FACE('',(#19219),#63314,.F.) ;
#66505=ADVANCED_FACE('',(#19220),#7325,.F.) ;
#66506=ADVANCED_FACE('',(#19221),#7326,.T.) ;
#66507=ADVANCED_FACE('',(#19222),#7327,.F.) ;
#66508=ADVANCED_FACE('',(#19223),#4581,.F.) ;
#66509=ADVANCED_FACE('',(#19224),#4582,.T.) ;
#66510=ADVANCED_FACE('',(#19225),#63315,.T.) ;
#66511=ADVANCED_FACE('',(#19226),#7328,.F.) ;
#66512=ADVANCED_FACE('',(#19227),#7329,.F.) ;
#66513=ADVANCED_FACE('',(#19228),#7330,.T.) ;
#66514=ADVANCED_FACE('',(#19229),#7331,.T.) ;
#66515=ADVANCED_FACE('',(#19230),#7332,.T.) ;
#66516=ADVANCED_FACE('',(#19231),#7333,.F.) ;
#66517=ADVANCED_FACE('',(#19232),#4583,.F.) ;
#66518=ADVANCED_FACE('',(#19233),#63316,.F.) ;
#66519=ADVANCED_FACE('',(#19234),#63317,.F.) ;
#66520=ADVANCED_FACE('',(#19235),#63318,.T.) ;
#66521=ADVANCED_FACE('',(#19236),#7334,.F.) ;
#66522=ADVANCED_FACE('',(#19237),#7335,.F.) ;
#66523=ADVANCED_FACE('',(#19238),#7336,.F.) ;
#66524=ADVANCED_FACE('',(#19239),#7337,.T.) ;
#66525=ADVANCED_FACE('',(#19240),#7338,.T.) ;
#66526=ADVANCED_FACE('',(#19241),#63319,.F.) ;
#66527=ADVANCED_FACE('',(#19242),#4584,.F.) ;
#66528=ADVANCED_FACE('',(#19243),#4585,.T.) ;
#66529=ADVANCED_FACE('',(#19244),#7339,.T.) ;
#66530=ADVANCED_FACE('',(#19245),#4586,.F.) ;
#66531=ADVANCED_FACE('',(#19246),#4587,.T.) ;
#66532=ADVANCED_FACE('',(#19247),#7340,.F.) ;
#66533=ADVANCED_FACE('',(#19248),#7341,.F.) ;
#66534=ADVANCED_FACE('',(#19249),#7342,.T.) ;
#66535=ADVANCED_FACE('',(#19250),#63320,.T.) ;
#66536=ADVANCED_FACE('',(#19251),#7343,.F.) ;
#66537=ADVANCED_FACE('',(#19252),#7344,.T.) ;
#66538=ADVANCED_FACE('',(#19253),#7345,.F.) ;
#66539=ADVANCED_FACE('',(#19254),#4588,.F.) ;
#66540=ADVANCED_FACE('',(#19255),#63321,.T.) ;
#66541=ADVANCED_FACE('',(#19256),#7346,.T.) ;
#66542=ADVANCED_FACE('',(#19257),#4589,.F.) ;
#66543=ADVANCED_FACE('',(#19258),#63322,.F.) ;
#66544=ADVANCED_FACE('',(#19259),#7347,.F.) ;
#66545=ADVANCED_FACE('',(#19260),#7348,.T.) ;
#66546=ADVANCED_FACE('',(#19261),#63323,.T.) ;
#66547=ADVANCED_FACE('',(#19262),#7349,.F.) ;
#66548=ADVANCED_FACE('',(#19263),#63324,.T.) ;
#66549=ADVANCED_FACE('',(#19264),#7350,.T.) ;
#66550=ADVANCED_FACE('',(#19265),#7351,.T.) ;
#66551=ADVANCED_FACE('',(#19266),#4590,.T.) ;
#66552=ADVANCED_FACE('',(#19267),#7352,.F.) ;
#66553=ADVANCED_FACE('',(#19268),#63325,.F.) ;
#66554=ADVANCED_FACE('',(#19269),#4591,.F.) ;
#66555=ADVANCED_FACE('',(#19270),#7353,.F.) ;
#66556=ADVANCED_FACE('',(#19271),#7354,.F.) ;
#66557=ADVANCED_FACE('',(#19272),#63326,.F.) ;
#66558=ADVANCED_FACE('',(#19273),#4592,.F.) ;
#66559=ADVANCED_FACE('',(#19274),#7355,.F.) ;
#66560=ADVANCED_FACE('',(#19275),#7356,.F.) ;
#66561=ADVANCED_FACE('',(#19276),#4593,.F.) ;
#66562=ADVANCED_FACE('',(#19277),#4594,.F.) ;
#66563=ADVANCED_FACE('',(#19278),#7357,.F.) ;
#66564=ADVANCED_FACE('',(#19279),#63327,.F.) ;
#66565=ADVANCED_FACE('',(#19280),#4595,.F.) ;
#66566=ADVANCED_FACE('',(#19281),#4596,.F.) ;
#66567=ADVANCED_FACE('',(#19282),#7358,.F.) ;
#66568=ADVANCED_FACE('',(#19283),#7359,.F.) ;
#66569=ADVANCED_FACE('',(#19284),#4597,.F.) ;
#66570=ADVANCED_FACE('',(#19285),#7360,.F.) ;
#66571=ADVANCED_FACE('',(#19286),#7361,.F.) ;
#66572=ADVANCED_FACE('',(#19287),#4598,.F.) ;
#66573=ADVANCED_FACE('',(#19288),#4599,.F.) ;
#66574=ADVANCED_FACE('',(#19289),#7362,.F.) ;
#66575=ADVANCED_FACE('',(#19290),#7363,.F.) ;
#66576=ADVANCED_FACE('',(#19291),#63328,.F.) ;
#66577=ADVANCED_FACE('',(#19292),#63329,.F.) ;
#66578=ADVANCED_FACE('',(#19293),#7364,.F.) ;
#66579=ADVANCED_FACE('',(#19294),#7365,.T.) ;
#66580=ADVANCED_FACE('',(#19295),#7366,.F.) ;
#66581=ADVANCED_FACE('',(#19296),#4600,.F.) ;
#66582=ADVANCED_FACE('',(#19297),#4601,.T.) ;
#66583=ADVANCED_FACE('',(#19298),#63330,.T.) ;
#66584=ADVANCED_FACE('',(#19299),#7367,.F.) ;
#66585=ADVANCED_FACE('',(#19300),#7368,.F.) ;
#66586=ADVANCED_FACE('',(#19301),#7369,.T.) ;
#66587=ADVANCED_FACE('',(#19302),#7370,.T.) ;
#66588=ADVANCED_FACE('',(#19303),#7371,.T.) ;
#66589=ADVANCED_FACE('',(#19304),#7372,.F.) ;
#66590=ADVANCED_FACE('',(#19305),#4602,.F.) ;
#66591=ADVANCED_FACE('',(#19306),#63331,.F.) ;
#66592=ADVANCED_FACE('',(#19307),#63332,.F.) ;
#66593=ADVANCED_FACE('',(#19308),#63333,.T.) ;
#66594=ADVANCED_FACE('',(#19309),#7373,.F.) ;
#66595=ADVANCED_FACE('',(#19310),#7374,.F.) ;
#66596=ADVANCED_FACE('',(#19311),#7375,.F.) ;
#66597=ADVANCED_FACE('',(#19312),#7376,.T.) ;
#66598=ADVANCED_FACE('',(#19313),#7377,.T.) ;
#66599=ADVANCED_FACE('',(#19314),#63334,.F.) ;
#66600=ADVANCED_FACE('',(#19315),#4603,.F.) ;
#66601=ADVANCED_FACE('',(#19316),#4604,.T.) ;
#66602=ADVANCED_FACE('',(#19317),#7378,.T.) ;
#66603=ADVANCED_FACE('',(#19318),#4605,.F.) ;
#66604=ADVANCED_FACE('',(#19319),#4606,.T.) ;
#66605=ADVANCED_FACE('',(#19320),#7379,.F.) ;
#66606=ADVANCED_FACE('',(#19321),#7380,.F.) ;
#66607=ADVANCED_FACE('',(#19322),#7381,.T.) ;
#66608=ADVANCED_FACE('',(#19323),#63335,.T.) ;
#66609=ADVANCED_FACE('',(#19324),#7382,.F.) ;
#66610=ADVANCED_FACE('',(#19325),#7383,.T.) ;
#66611=ADVANCED_FACE('',(#19326),#7384,.F.) ;
#66612=ADVANCED_FACE('',(#19327),#4607,.F.) ;
#66613=ADVANCED_FACE('',(#19328),#63336,.T.) ;
#66614=ADVANCED_FACE('',(#19329),#7385,.T.) ;
#66615=ADVANCED_FACE('',(#19330),#4608,.F.) ;
#66616=ADVANCED_FACE('',(#19331),#63337,.F.) ;
#66617=ADVANCED_FACE('',(#19332),#7386,.F.) ;
#66618=ADVANCED_FACE('',(#19333),#7387,.T.) ;
#66619=ADVANCED_FACE('',(#19334),#63338,.T.) ;
#66620=ADVANCED_FACE('',(#19335),#7388,.F.) ;
#66621=ADVANCED_FACE('',(#19336),#63339,.T.) ;
#66622=ADVANCED_FACE('',(#19337),#7389,.T.) ;
#66623=ADVANCED_FACE('',(#19338),#7390,.T.) ;
#66624=ADVANCED_FACE('',(#19339),#4609,.T.) ;
#66625=ADVANCED_FACE('',(#19340),#7391,.F.) ;
#66626=ADVANCED_FACE('',(#19341),#63340,.F.) ;
#66627=ADVANCED_FACE('',(#19342),#4610,.F.) ;
#66628=ADVANCED_FACE('',(#19343),#7392,.F.) ;
#66629=ADVANCED_FACE('',(#19344),#7393,.F.) ;
#66630=ADVANCED_FACE('',(#19345),#63341,.F.) ;
#66631=ADVANCED_FACE('',(#19346),#4611,.F.) ;
#66632=ADVANCED_FACE('',(#19347),#7394,.F.) ;
#66633=ADVANCED_FACE('',(#19348),#7395,.F.) ;
#66634=ADVANCED_FACE('',(#19349),#4612,.F.) ;
#66635=ADVANCED_FACE('',(#19350),#4613,.F.) ;
#66636=ADVANCED_FACE('',(#19351),#7396,.F.) ;
#66637=ADVANCED_FACE('',(#19352),#63342,.F.) ;
#66638=ADVANCED_FACE('',(#19353),#4614,.F.) ;
#66639=ADVANCED_FACE('',(#19354),#4615,.F.) ;
#66640=ADVANCED_FACE('',(#19355),#7397,.F.) ;
#66641=ADVANCED_FACE('',(#19356),#7398,.F.) ;
#66642=ADVANCED_FACE('',(#19357),#4616,.F.) ;
#66643=ADVANCED_FACE('',(#19358),#7399,.F.) ;
#66644=ADVANCED_FACE('',(#19359),#7400,.F.) ;
#66645=ADVANCED_FACE('',(#19360),#4617,.F.) ;
#66646=ADVANCED_FACE('',(#19361),#4618,.F.) ;
#66647=ADVANCED_FACE('',(#19362),#7401,.F.) ;
#66648=ADVANCED_FACE('',(#19363),#7402,.F.) ;
#66649=ADVANCED_FACE('',(#19364),#63343,.F.) ;
#66650=ADVANCED_FACE('',(#19365),#63344,.F.) ;
#66651=ADVANCED_FACE('',(#19366),#7403,.F.) ;
#66652=ADVANCED_FACE('',(#19367),#7404,.T.) ;
#66653=ADVANCED_FACE('',(#19368),#7405,.F.) ;
#66654=ADVANCED_FACE('',(#19369),#4619,.F.) ;
#66655=ADVANCED_FACE('',(#19370),#4620,.T.) ;
#66656=ADVANCED_FACE('',(#19371),#63345,.T.) ;
#66657=ADVANCED_FACE('',(#19372),#7406,.F.) ;
#66658=ADVANCED_FACE('',(#19373),#7407,.F.) ;
#66659=ADVANCED_FACE('',(#19374),#7408,.T.) ;
#66660=ADVANCED_FACE('',(#19375),#7409,.T.) ;
#66661=ADVANCED_FACE('',(#19376),#7410,.T.) ;
#66662=ADVANCED_FACE('',(#19377),#7411,.F.) ;
#66663=ADVANCED_FACE('',(#19378),#4621,.F.) ;
#66664=ADVANCED_FACE('',(#19379),#63346,.F.) ;
#66665=ADVANCED_FACE('',(#19380),#63347,.F.) ;
#66666=ADVANCED_FACE('',(#19381),#63348,.T.) ;
#66667=ADVANCED_FACE('',(#19382),#7412,.F.) ;
#66668=ADVANCED_FACE('',(#19383),#7413,.F.) ;
#66669=ADVANCED_FACE('',(#19384),#7414,.F.) ;
#66670=ADVANCED_FACE('',(#19385),#7415,.T.) ;
#66671=ADVANCED_FACE('',(#19386),#7416,.T.) ;
#66672=ADVANCED_FACE('',(#19387),#63349,.F.) ;
#66673=ADVANCED_FACE('',(#19388),#4622,.F.) ;
#66674=ADVANCED_FACE('',(#19389),#4623,.T.) ;
#66675=ADVANCED_FACE('',(#19390),#7417,.T.) ;
#66676=ADVANCED_FACE('',(#19391),#4624,.F.) ;
#66677=ADVANCED_FACE('',(#19392),#4625,.T.) ;
#66678=ADVANCED_FACE('',(#19393),#7418,.F.) ;
#66679=ADVANCED_FACE('',(#19394),#7419,.F.) ;
#66680=ADVANCED_FACE('',(#19395),#7420,.T.) ;
#66681=ADVANCED_FACE('',(#19396),#63350,.T.) ;
#66682=ADVANCED_FACE('',(#19397),#7421,.F.) ;
#66683=ADVANCED_FACE('',(#19398),#7422,.T.) ;
#66684=ADVANCED_FACE('',(#19399),#7423,.F.) ;
#66685=ADVANCED_FACE('',(#19400),#4626,.F.) ;
#66686=ADVANCED_FACE('',(#19401),#63351,.T.) ;
#66687=ADVANCED_FACE('',(#19402),#7424,.T.) ;
#66688=ADVANCED_FACE('',(#19403),#4627,.F.) ;
#66689=ADVANCED_FACE('',(#19404),#63352,.F.) ;
#66690=ADVANCED_FACE('',(#19405),#7425,.F.) ;
#66691=ADVANCED_FACE('',(#19406),#7426,.T.) ;
#66692=ADVANCED_FACE('',(#19407),#63353,.T.) ;
#66693=ADVANCED_FACE('',(#19408),#7427,.F.) ;
#66694=ADVANCED_FACE('',(#19409),#63354,.T.) ;
#66695=ADVANCED_FACE('',(#19410),#7428,.T.) ;
#66696=ADVANCED_FACE('',(#19411),#7429,.T.) ;
#66697=ADVANCED_FACE('',(#19412),#4628,.T.) ;
#66698=ADVANCED_FACE('',(#19413),#7430,.F.) ;
#66699=ADVANCED_FACE('',(#19414),#63355,.F.) ;
#66700=ADVANCED_FACE('',(#19415),#4629,.F.) ;
#66701=ADVANCED_FACE('',(#19416),#7431,.F.) ;
#66702=ADVANCED_FACE('',(#19417),#7432,.F.) ;
#66703=ADVANCED_FACE('',(#19418),#63356,.F.) ;
#66704=ADVANCED_FACE('',(#19419),#4630,.F.) ;
#66705=ADVANCED_FACE('',(#19420),#7433,.F.) ;
#66706=ADVANCED_FACE('',(#19421),#7434,.F.) ;
#66707=ADVANCED_FACE('',(#19422),#4631,.F.) ;
#66708=ADVANCED_FACE('',(#19423),#4632,.F.) ;
#66709=ADVANCED_FACE('',(#19424),#7435,.F.) ;
#66710=ADVANCED_FACE('',(#19425),#63357,.F.) ;
#66711=ADVANCED_FACE('',(#19426),#4633,.F.) ;
#66712=ADVANCED_FACE('',(#19427),#4634,.F.) ;
#66713=ADVANCED_FACE('',(#19428),#7436,.F.) ;
#66714=ADVANCED_FACE('',(#19429),#7437,.F.) ;
#66715=ADVANCED_FACE('',(#19430),#4635,.F.) ;
#66716=ADVANCED_FACE('',(#19431),#7438,.F.) ;
#66717=ADVANCED_FACE('',(#19432),#7439,.F.) ;
#66718=ADVANCED_FACE('',(#19433),#4636,.F.) ;
#66719=ADVANCED_FACE('',(#19434),#4637,.F.) ;
#66720=ADVANCED_FACE('',(#19435),#7440,.F.) ;
#66721=ADVANCED_FACE('',(#19436),#7441,.F.) ;
#66722=ADVANCED_FACE('',(#19437),#63358,.F.) ;
#66723=ADVANCED_FACE('',(#19438),#63359,.F.) ;
#66724=ADVANCED_FACE('',(#19439),#7442,.F.) ;
#66725=ADVANCED_FACE('',(#19440),#7443,.T.) ;
#66726=ADVANCED_FACE('',(#19441),#7444,.F.) ;
#66727=ADVANCED_FACE('',(#19442),#4638,.F.) ;
#66728=ADVANCED_FACE('',(#19443),#4639,.T.) ;
#66729=ADVANCED_FACE('',(#19444),#63360,.T.) ;
#66730=ADVANCED_FACE('',(#19445),#7445,.F.) ;
#66731=ADVANCED_FACE('',(#19446),#7446,.F.) ;
#66732=ADVANCED_FACE('',(#19447),#7447,.T.) ;
#66733=ADVANCED_FACE('',(#19448),#7448,.T.) ;
#66734=ADVANCED_FACE('',(#19449),#7449,.T.) ;
#66735=ADVANCED_FACE('',(#19450),#7450,.F.) ;
#66736=ADVANCED_FACE('',(#19451),#4640,.F.) ;
#66737=ADVANCED_FACE('',(#19452),#63361,.F.) ;
#66738=ADVANCED_FACE('',(#19453),#63362,.F.) ;
#66739=ADVANCED_FACE('',(#19454),#63363,.T.) ;
#66740=ADVANCED_FACE('',(#19455),#7451,.F.) ;
#66741=ADVANCED_FACE('',(#19456),#7452,.F.) ;
#66742=ADVANCED_FACE('',(#19457),#7453,.F.) ;
#66743=ADVANCED_FACE('',(#19458),#7454,.T.) ;
#66744=ADVANCED_FACE('',(#19459),#7455,.T.) ;
#66745=ADVANCED_FACE('',(#19460),#63364,.F.) ;
#66746=ADVANCED_FACE('',(#19461),#4641,.F.) ;
#66747=ADVANCED_FACE('',(#19462),#4642,.T.) ;
#66748=ADVANCED_FACE('',(#19463),#7456,.T.) ;
#66749=ADVANCED_FACE('',(#19464),#4643,.F.) ;
#66750=ADVANCED_FACE('',(#19465),#4644,.T.) ;
#66751=ADVANCED_FACE('',(#19466),#7457,.F.) ;
#66752=ADVANCED_FACE('',(#19467),#7458,.F.) ;
#66753=ADVANCED_FACE('',(#19468),#7459,.T.) ;
#66754=ADVANCED_FACE('',(#19469),#63365,.T.) ;
#66755=ADVANCED_FACE('',(#19470),#7460,.F.) ;
#66756=ADVANCED_FACE('',(#19471),#7461,.T.) ;
#66757=ADVANCED_FACE('',(#19472),#7462,.F.) ;
#66758=ADVANCED_FACE('',(#19473),#4645,.F.) ;
#66759=ADVANCED_FACE('',(#19474),#63366,.T.) ;
#66760=ADVANCED_FACE('',(#19475),#7463,.T.) ;
#66761=ADVANCED_FACE('',(#19476),#4646,.F.) ;
#66762=ADVANCED_FACE('',(#19477),#63367,.F.) ;
#66763=ADVANCED_FACE('',(#19478),#7464,.F.) ;
#66764=ADVANCED_FACE('',(#19479),#7465,.T.) ;
#66765=ADVANCED_FACE('',(#19480),#63368,.T.) ;
#66766=ADVANCED_FACE('',(#19481),#7466,.F.) ;
#66767=ADVANCED_FACE('',(#19482),#63369,.T.) ;
#66768=ADVANCED_FACE('',(#19483),#7467,.T.) ;
#66769=ADVANCED_FACE('',(#19484),#7468,.T.) ;
#66770=ADVANCED_FACE('',(#19485),#4647,.T.) ;
#66771=ADVANCED_FACE('',(#19486),#7469,.F.) ;
#66772=ADVANCED_FACE('',(#19487),#63370,.F.) ;
#66773=ADVANCED_FACE('',(#19488),#4648,.F.) ;
#66774=ADVANCED_FACE('',(#19489),#7470,.F.) ;
#66775=ADVANCED_FACE('',(#19490),#7471,.F.) ;
#66776=ADVANCED_FACE('',(#19491),#63371,.F.) ;
#66777=ADVANCED_FACE('',(#19492),#4649,.F.) ;
#66778=ADVANCED_FACE('',(#19493),#7472,.F.) ;
#66779=ADVANCED_FACE('',(#19494),#7473,.F.) ;
#66780=ADVANCED_FACE('',(#19495),#4650,.F.) ;
#66781=ADVANCED_FACE('',(#19496),#4651,.F.) ;
#66782=ADVANCED_FACE('',(#19497),#7474,.F.) ;
#66783=ADVANCED_FACE('',(#19498),#63372,.F.) ;
#66784=ADVANCED_FACE('',(#19499),#4652,.F.) ;
#66785=ADVANCED_FACE('',(#19500),#4653,.F.) ;
#66786=ADVANCED_FACE('',(#19501),#7475,.F.) ;
#66787=ADVANCED_FACE('',(#19502),#7476,.F.) ;
#66788=ADVANCED_FACE('',(#19503),#4654,.F.) ;
#66789=ADVANCED_FACE('',(#19504),#7477,.F.) ;
#66790=ADVANCED_FACE('',(#19505),#7478,.F.) ;
#66791=ADVANCED_FACE('',(#19506),#4655,.F.) ;
#66792=ADVANCED_FACE('',(#19507),#4656,.F.) ;
#66793=ADVANCED_FACE('',(#19508),#7479,.F.) ;
#66794=ADVANCED_FACE('',(#19509),#7480,.F.) ;
#66795=ADVANCED_FACE('',(#19510),#63373,.F.) ;
#66796=ADVANCED_FACE('',(#19511),#63374,.F.) ;
#66797=ADVANCED_FACE('',(#19512),#7481,.F.) ;
#66798=ADVANCED_FACE('',(#19513),#7482,.T.) ;
#66799=ADVANCED_FACE('',(#19514),#7483,.F.) ;
#66800=ADVANCED_FACE('',(#19515),#4657,.F.) ;
#66801=ADVANCED_FACE('',(#19516),#4658,.T.) ;
#66802=ADVANCED_FACE('',(#19517),#63375,.T.) ;
#66803=ADVANCED_FACE('',(#19518),#7484,.F.) ;
#66804=ADVANCED_FACE('',(#19519),#7485,.F.) ;
#66805=ADVANCED_FACE('',(#19520),#7486,.T.) ;
#66806=ADVANCED_FACE('',(#19521),#7487,.T.) ;
#66807=ADVANCED_FACE('',(#19522),#7488,.T.) ;
#66808=ADVANCED_FACE('',(#19523),#7489,.F.) ;
#66809=ADVANCED_FACE('',(#19524),#4659,.F.) ;
#66810=ADVANCED_FACE('',(#19525),#63376,.F.) ;
#66811=ADVANCED_FACE('',(#19526),#63377,.F.) ;
#66812=ADVANCED_FACE('',(#19527),#63378,.T.) ;
#66813=ADVANCED_FACE('',(#19528),#7490,.F.) ;
#66814=ADVANCED_FACE('',(#19529),#7491,.F.) ;
#66815=ADVANCED_FACE('',(#19530),#7492,.F.) ;
#66816=ADVANCED_FACE('',(#19531),#7493,.T.) ;
#66817=ADVANCED_FACE('',(#19532),#7494,.T.) ;
#66818=ADVANCED_FACE('',(#19533),#63379,.F.) ;
#66819=ADVANCED_FACE('',(#19534),#4660,.F.) ;
#66820=ADVANCED_FACE('',(#19535),#4661,.T.) ;
#66821=ADVANCED_FACE('',(#19536),#7495,.T.) ;
#66822=ADVANCED_FACE('',(#19537),#4662,.F.) ;
#66823=ADVANCED_FACE('',(#19538),#4663,.T.) ;
#66824=ADVANCED_FACE('',(#19539),#7496,.F.) ;
#66825=ADVANCED_FACE('',(#19540),#7497,.F.) ;
#66826=ADVANCED_FACE('',(#19541),#7498,.T.) ;
#66827=ADVANCED_FACE('',(#19542),#63380,.T.) ;
#66828=ADVANCED_FACE('',(#19543),#7499,.F.) ;
#66829=ADVANCED_FACE('',(#19544),#7500,.T.) ;
#66830=ADVANCED_FACE('',(#19545),#7501,.F.) ;
#66831=ADVANCED_FACE('',(#19546),#4664,.F.) ;
#66832=ADVANCED_FACE('',(#19547),#63381,.T.) ;
#66833=ADVANCED_FACE('',(#19548),#7502,.T.) ;
#66834=ADVANCED_FACE('',(#19549),#4665,.F.) ;
#66835=ADVANCED_FACE('',(#19550),#63382,.F.) ;
#66836=ADVANCED_FACE('',(#19551),#7503,.F.) ;
#66837=ADVANCED_FACE('',(#19552),#7504,.T.) ;
#66838=ADVANCED_FACE('',(#19553),#63383,.T.) ;
#66839=ADVANCED_FACE('',(#19554),#7505,.F.) ;
#66840=ADVANCED_FACE('',(#19555),#63384,.T.) ;
#66841=ADVANCED_FACE('',(#19556),#7506,.T.) ;
#66842=ADVANCED_FACE('',(#19557),#7507,.T.) ;
#66843=ADVANCED_FACE('',(#19558),#4666,.T.) ;
#66844=ADVANCED_FACE('',(#19559),#7508,.F.) ;
#66845=ADVANCED_FACE('',(#19560),#63385,.F.) ;
#66846=ADVANCED_FACE('',(#19561),#4667,.F.) ;
#66847=ADVANCED_FACE('',(#19562),#7509,.F.) ;
#66848=ADVANCED_FACE('',(#19563),#7510,.F.) ;
#66849=ADVANCED_FACE('',(#19564),#63386,.F.) ;
#66850=ADVANCED_FACE('',(#19565),#4668,.F.) ;
#66851=ADVANCED_FACE('',(#19566),#7511,.F.) ;
#66852=ADVANCED_FACE('',(#19567),#7512,.F.) ;
#66853=ADVANCED_FACE('',(#19568),#4669,.F.) ;
#66854=ADVANCED_FACE('',(#19569),#4670,.F.) ;
#66855=ADVANCED_FACE('',(#19570),#7513,.F.) ;
#66856=ADVANCED_FACE('',(#19571),#63387,.F.) ;
#66857=ADVANCED_FACE('',(#19572),#4671,.F.) ;
#66858=ADVANCED_FACE('',(#19573),#4672,.F.) ;
#66859=ADVANCED_FACE('',(#19574),#7514,.F.) ;
#66860=ADVANCED_FACE('',(#19575),#7515,.F.) ;
#66861=ADVANCED_FACE('',(#19576),#4673,.F.) ;
#66862=ADVANCED_FACE('',(#19577),#7516,.F.) ;
#66863=ADVANCED_FACE('',(#19578),#7517,.F.) ;
#66864=ADVANCED_FACE('',(#19579),#4674,.F.) ;
#66865=ADVANCED_FACE('',(#19580),#4675,.F.) ;
#66866=ADVANCED_FACE('',(#19581),#7518,.F.) ;
#66867=ADVANCED_FACE('',(#19582),#7519,.F.) ;
#66868=ADVANCED_FACE('',(#19583),#63388,.F.) ;
#66869=ADVANCED_FACE('',(#19584),#63389,.F.) ;
#66870=ADVANCED_FACE('',(#19585),#7520,.F.) ;
#66871=ADVANCED_FACE('',(#19586),#7521,.T.) ;
#66872=ADVANCED_FACE('',(#19587),#7522,.F.) ;
#66873=ADVANCED_FACE('',(#19588),#4676,.F.) ;
#66874=ADVANCED_FACE('',(#19589),#4677,.T.) ;
#66875=ADVANCED_FACE('',(#19590),#63390,.T.) ;
#66876=ADVANCED_FACE('',(#19591),#7523,.F.) ;
#66877=ADVANCED_FACE('',(#19592),#7524,.F.) ;
#66878=ADVANCED_FACE('',(#19593),#7525,.T.) ;
#66879=ADVANCED_FACE('',(#19594),#7526,.T.) ;
#66880=ADVANCED_FACE('',(#19595),#7527,.T.) ;
#66881=ADVANCED_FACE('',(#19596),#7528,.F.) ;
#66882=ADVANCED_FACE('',(#19597),#4678,.F.) ;
#66883=ADVANCED_FACE('',(#19598),#63391,.F.) ;
#66884=ADVANCED_FACE('',(#19599),#63392,.F.) ;
#66885=ADVANCED_FACE('',(#19600),#63393,.T.) ;
#66886=ADVANCED_FACE('',(#19601),#7529,.F.) ;
#66887=ADVANCED_FACE('',(#19602),#7530,.F.) ;
#66888=ADVANCED_FACE('',(#19603),#7531,.F.) ;
#66889=ADVANCED_FACE('',(#19604),#7532,.T.) ;
#66890=ADVANCED_FACE('',(#19605),#7533,.T.) ;
#66891=ADVANCED_FACE('',(#19606),#63394,.F.) ;
#66892=ADVANCED_FACE('',(#19607),#4679,.F.) ;
#66893=ADVANCED_FACE('',(#19608),#4680,.T.) ;
#66894=ADVANCED_FACE('',(#19609),#7534,.T.) ;
#66895=ADVANCED_FACE('',(#19610),#4681,.F.) ;
#66896=ADVANCED_FACE('',(#19611),#4682,.T.) ;
#66897=ADVANCED_FACE('',(#19612),#7535,.F.) ;
#66898=ADVANCED_FACE('',(#19613),#7536,.F.) ;
#66899=ADVANCED_FACE('',(#19614),#7537,.T.) ;
#66900=ADVANCED_FACE('',(#19615),#63395,.T.) ;
#66901=ADVANCED_FACE('',(#19616),#7538,.F.) ;
#66902=ADVANCED_FACE('',(#19617),#7539,.T.) ;
#66903=ADVANCED_FACE('',(#19618),#7540,.F.) ;
#66904=ADVANCED_FACE('',(#19619),#4683,.F.) ;
#66905=ADVANCED_FACE('',(#19620),#63396,.T.) ;
#66906=ADVANCED_FACE('',(#19621),#7541,.T.) ;
#66907=ADVANCED_FACE('',(#19622),#4684,.F.) ;
#66908=ADVANCED_FACE('',(#19623),#63397,.F.) ;
#66909=ADVANCED_FACE('',(#19624),#7542,.F.) ;
#66910=ADVANCED_FACE('',(#19625),#7543,.T.) ;
#66911=ADVANCED_FACE('',(#19626),#63398,.T.) ;
#66912=ADVANCED_FACE('',(#19627),#7544,.F.) ;
#66913=ADVANCED_FACE('',(#19628),#63399,.T.) ;
#66914=ADVANCED_FACE('',(#19629),#7545,.T.) ;
#66915=ADVANCED_FACE('',(#19630),#7546,.T.) ;
#66916=ADVANCED_FACE('',(#19631),#4685,.T.) ;
#66917=ADVANCED_FACE('',(#19632),#7547,.F.) ;
#66918=ADVANCED_FACE('',(#19633),#63400,.F.) ;
#66919=ADVANCED_FACE('',(#19634),#4686,.F.) ;
#66920=ADVANCED_FACE('',(#19635),#7548,.F.) ;
#66921=ADVANCED_FACE('',(#19636),#7549,.F.) ;
#66922=ADVANCED_FACE('',(#19637),#63401,.F.) ;
#66923=ADVANCED_FACE('',(#19638),#4687,.F.) ;
#66924=ADVANCED_FACE('',(#19639),#7550,.F.) ;
#66925=ADVANCED_FACE('',(#19640),#7551,.F.) ;
#66926=ADVANCED_FACE('',(#19641),#4688,.F.) ;
#66927=ADVANCED_FACE('',(#19642),#4689,.F.) ;
#66928=ADVANCED_FACE('',(#19643),#7552,.F.) ;
#66929=ADVANCED_FACE('',(#19644),#63402,.F.) ;
#66930=ADVANCED_FACE('',(#19645),#4690,.F.) ;
#66931=ADVANCED_FACE('',(#19646),#4691,.F.) ;
#66932=ADVANCED_FACE('',(#19647),#7553,.F.) ;
#66933=ADVANCED_FACE('',(#19648),#7554,.F.) ;
#66934=ADVANCED_FACE('',(#19649),#4692,.F.) ;
#66935=ADVANCED_FACE('',(#19650),#7555,.F.) ;
#66936=ADVANCED_FACE('',(#19651),#7556,.F.) ;
#66937=ADVANCED_FACE('',(#19652),#4693,.F.) ;
#66938=ADVANCED_FACE('',(#19653),#4694,.F.) ;
#66939=ADVANCED_FACE('',(#19654),#7557,.F.) ;
#66940=ADVANCED_FACE('',(#19655),#7558,.F.) ;
#66941=ADVANCED_FACE('',(#19656),#63403,.F.) ;
#66942=ADVANCED_FACE('',(#19657),#63404,.F.) ;
#66943=ADVANCED_FACE('',(#19658),#7559,.F.) ;
#66944=ADVANCED_FACE('',(#19659),#5751,.F.) ;
#66945=ADVANCED_FACE('',(#19660),#5752,.F.) ;
#66946=ADVANCED_FACE('',(#19661),#5753,.F.) ;
#66947=ADVANCED_FACE('',(#19662),#5754,.F.) ;
#66948=ADVANCED_FACE('',(#19663),#5755,.F.) ;
#66949=ADVANCED_FACE('',(#19664),#5756,.T.) ;
#66950=ADVANCED_FACE('',(#19665),#5757,.F.) ;
#66951=ADVANCED_FACE('',(#19666),#7560,.T.) ;
#66952=ADVANCED_FACE('',(#19667),#7561,.F.) ;
#66953=ADVANCED_FACE('',(#19668),#5758,.F.) ;
#66954=ADVANCED_FACE('',(#19669),#5759,.F.) ;
#66955=ADVANCED_FACE('',(#19670),#5760,.F.) ;
#66956=ADVANCED_FACE('',(#19671),#5761,.F.) ;
#66957=ADVANCED_FACE('',(#19672),#5762,.F.) ;
#66958=ADVANCED_FACE('',(#19673),#5763,.T.) ;
#66959=ADVANCED_FACE('',(#19674),#5764,.F.) ;
#66960=ADVANCED_FACE('',(#19675),#5765,.F.) ;
#66961=ADVANCED_FACE('',(#19676),#5766,.F.) ;
#66962=ADVANCED_FACE('',(#19677),#5767,.F.) ;
#66963=ADVANCED_FACE('',(#19678),#5768,.F.) ;
#66964=ADVANCED_FACE('',(#19679),#5769,.F.) ;
#66965=ADVANCED_FACE('',(#19680),#5770,.T.) ;
#66966=ADVANCED_FACE('',(#19681),#5771,.F.) ;
#66967=ADVANCED_FACE('',(#19682),#7562,.T.) ;
#66968=ADVANCED_FACE('',(#19683),#7563,.F.) ;
#66969=ADVANCED_FACE('',(#19684),#5772,.F.) ;
#66970=ADVANCED_FACE('',(#19685),#5773,.F.) ;
#66971=ADVANCED_FACE('',(#19686),#5774,.F.) ;
#66972=ADVANCED_FACE('',(#19687),#5775,.F.) ;
#66973=ADVANCED_FACE('',(#19688),#5776,.F.) ;
#66974=ADVANCED_FACE('',(#19689),#5777,.T.) ;
#66975=ADVANCED_FACE('',(#19690),#5778,.F.) ;
#66976=ADVANCED_FACE('',(#19691),#5779,.F.) ;
#66977=ADVANCED_FACE('',(#19692),#5780,.F.) ;
#66978=ADVANCED_FACE('',(#19693),#5781,.F.) ;
#66979=ADVANCED_FACE('',(#19694),#5782,.F.) ;
#66980=ADVANCED_FACE('',(#19695),#5783,.F.) ;
#66981=ADVANCED_FACE('',(#19696),#5784,.T.) ;
#66982=ADVANCED_FACE('',(#19697),#5785,.F.) ;
#66983=ADVANCED_FACE('',(#19698),#7564,.T.) ;
#66984=ADVANCED_FACE('',(#19699),#7565,.F.) ;
#66985=ADVANCED_FACE('',(#19700),#5786,.F.) ;
#66986=ADVANCED_FACE('',(#19701),#5787,.F.) ;
#66987=ADVANCED_FACE('',(#19702),#5788,.F.) ;
#66988=ADVANCED_FACE('',(#19703),#5789,.F.) ;
#66989=ADVANCED_FACE('',(#19704),#5790,.F.) ;
#66990=ADVANCED_FACE('',(#19705),#5791,.T.) ;
#66991=ADVANCED_FACE('',(#19706),#5792,.F.) ;
#66992=ADVANCED_FACE('',(#19707),#5793,.F.) ;
#66993=ADVANCED_FACE('',(#19708),#5794,.F.) ;
#66994=ADVANCED_FACE('',(#19709),#5795,.F.) ;
#66995=ADVANCED_FACE('',(#19710),#5796,.F.) ;
#66996=ADVANCED_FACE('',(#19711),#5797,.F.) ;
#66997=ADVANCED_FACE('',(#19712),#5798,.T.) ;
#66998=ADVANCED_FACE('',(#19713),#5799,.F.) ;
#66999=ADVANCED_FACE('',(#19714),#7566,.T.) ;
#67000=ADVANCED_FACE('',(#19715),#7567,.F.) ;
#67001=ADVANCED_FACE('',(#19716),#5800,.F.) ;
#67002=ADVANCED_FACE('',(#19717),#5801,.F.) ;
#67003=ADVANCED_FACE('',(#19718),#5802,.F.) ;
#67004=ADVANCED_FACE('',(#19719),#5803,.F.) ;
#67005=ADVANCED_FACE('',(#19720),#5804,.F.) ;
#67006=ADVANCED_FACE('',(#19721),#5805,.T.) ;
#67007=ADVANCED_FACE('',(#19722),#5806,.F.) ;
#67008=ADVANCED_FACE('',(#19723),#5807,.F.) ;
#67009=ADVANCED_FACE('',(#19724),#5808,.F.) ;
#67010=ADVANCED_FACE('',(#19725),#5809,.F.) ;
#67011=ADVANCED_FACE('',(#19726),#5810,.F.) ;
#67012=ADVANCED_FACE('',(#19727),#5811,.F.) ;
#67013=ADVANCED_FACE('',(#19728),#5812,.T.) ;
#67014=ADVANCED_FACE('',(#19729),#5813,.F.) ;
#67015=ADVANCED_FACE('',(#19730),#7568,.T.) ;
#67016=ADVANCED_FACE('',(#19731),#7569,.F.) ;
#67017=ADVANCED_FACE('',(#19732),#5814,.F.) ;
#67018=ADVANCED_FACE('',(#19733),#5815,.F.) ;
#67019=ADVANCED_FACE('',(#19734),#5816,.F.) ;
#67020=ADVANCED_FACE('',(#19735),#5817,.F.) ;
#67021=ADVANCED_FACE('',(#19736),#5818,.F.) ;
#67022=ADVANCED_FACE('',(#19737),#5819,.T.) ;
#67023=ADVANCED_FACE('',(#19738),#5820,.F.) ;
#67024=ADVANCED_FACE('',(#19739),#5821,.F.) ;
#67025=ADVANCED_FACE('',(#19740),#5822,.F.) ;
#67026=ADVANCED_FACE('',(#19741),#5823,.F.) ;
#67027=ADVANCED_FACE('',(#19742),#5824,.F.) ;
#67028=ADVANCED_FACE('',(#19743),#5825,.F.) ;
#67029=ADVANCED_FACE('',(#19744),#5826,.T.) ;
#67030=ADVANCED_FACE('',(#19745),#5827,.F.) ;
#67031=ADVANCED_FACE('',(#19746),#7570,.T.) ;
#67032=ADVANCED_FACE('',(#19747),#7571,.F.) ;
#67033=ADVANCED_FACE('',(#19748),#5828,.F.) ;
#67034=ADVANCED_FACE('',(#19749),#5829,.F.) ;
#67035=ADVANCED_FACE('',(#19750),#5830,.F.) ;
#67036=ADVANCED_FACE('',(#19751),#5831,.F.) ;
#67037=ADVANCED_FACE('',(#19752),#5832,.F.) ;
#67038=ADVANCED_FACE('',(#19753),#5833,.T.) ;
#67039=ADVANCED_FACE('',(#19754),#5834,.F.) ;
#67040=ADVANCED_FACE('',(#19755),#5835,.F.) ;
#67041=ADVANCED_FACE('',(#19756),#5836,.F.) ;
#67042=ADVANCED_FACE('',(#19757),#5837,.F.) ;
#67043=ADVANCED_FACE('',(#19758),#5838,.F.) ;
#67044=ADVANCED_FACE('',(#19759),#5839,.F.) ;
#67045=ADVANCED_FACE('',(#19760),#5840,.T.) ;
#67046=ADVANCED_FACE('',(#19761),#5841,.F.) ;
#67047=ADVANCED_FACE('',(#19762),#7572,.T.) ;
#67048=ADVANCED_FACE('',(#19763),#7573,.F.) ;
#67049=ADVANCED_FACE('',(#19764),#5842,.F.) ;
#67050=ADVANCED_FACE('',(#19765),#5843,.F.) ;
#67051=ADVANCED_FACE('',(#19766),#5844,.F.) ;
#67052=ADVANCED_FACE('',(#19767),#5845,.F.) ;
#67053=ADVANCED_FACE('',(#19768),#5846,.F.) ;
#67054=ADVANCED_FACE('',(#19769),#5847,.T.) ;
#67055=ADVANCED_FACE('',(#19770),#5848,.F.) ;
#67056=ADVANCED_FACE('',(#19771),#5849,.F.) ;
#67057=ADVANCED_FACE('',(#19772),#5850,.F.) ;
#67058=ADVANCED_FACE('',(#19773),#5851,.F.) ;
#67059=ADVANCED_FACE('',(#19774),#5852,.F.) ;
#67060=ADVANCED_FACE('',(#19775),#5853,.F.) ;
#67061=ADVANCED_FACE('',(#19776),#5854,.T.) ;
#67062=ADVANCED_FACE('',(#19777),#5855,.F.) ;
#67063=ADVANCED_FACE('',(#19778),#7574,.T.) ;
#67064=ADVANCED_FACE('',(#19779),#7575,.F.) ;
#67065=ADVANCED_FACE('',(#19780),#5856,.F.) ;
#67066=ADVANCED_FACE('',(#19781),#5857,.F.) ;
#67067=ADVANCED_FACE('',(#19782),#5858,.F.) ;
#67068=ADVANCED_FACE('',(#19783),#5859,.F.) ;
#67069=ADVANCED_FACE('',(#19784),#5860,.F.) ;
#67070=ADVANCED_FACE('',(#19785),#5861,.T.) ;
#67071=ADVANCED_FACE('',(#19786),#5862,.F.) ;
#67072=ADVANCED_FACE('',(#19787),#5863,.F.) ;
#67073=ADVANCED_FACE('',(#19788),#5864,.F.) ;
#67074=ADVANCED_FACE('',(#19789),#5865,.F.) ;
#67075=ADVANCED_FACE('',(#19790),#5866,.F.) ;
#67076=ADVANCED_FACE('',(#19791),#5867,.F.) ;
#67077=ADVANCED_FACE('',(#19792),#5868,.T.) ;
#67078=ADVANCED_FACE('',(#19793),#5869,.F.) ;
#67079=ADVANCED_FACE('',(#19794),#7576,.T.) ;
#67080=ADVANCED_FACE('',(#19795),#7577,.F.) ;
#67081=ADVANCED_FACE('',(#19796),#5870,.F.) ;
#67082=ADVANCED_FACE('',(#19797),#5871,.F.) ;
#67083=ADVANCED_FACE('',(#19798),#5872,.F.) ;
#67084=ADVANCED_FACE('',(#19799),#5873,.F.) ;
#67085=ADVANCED_FACE('',(#19800),#5874,.F.) ;
#67086=ADVANCED_FACE('',(#19801),#5875,.T.) ;
#67087=ADVANCED_FACE('',(#19802),#5876,.F.) ;
#67088=ADVANCED_FACE('',(#19803),#5877,.F.) ;
#67089=ADVANCED_FACE('',(#19804),#5878,.F.) ;
#67090=ADVANCED_FACE('',(#19805),#5879,.F.) ;
#67091=ADVANCED_FACE('',(#19806),#5880,.F.) ;
#67092=ADVANCED_FACE('',(#19807),#5881,.F.) ;
#67093=ADVANCED_FACE('',(#19808),#5882,.F.) ;
#67094=ADVANCED_FACE('',(#19809),#5883,.F.) ;
#67095=ADVANCED_FACE('',(#19810),#5884,.F.) ;
#67096=ADVANCED_FACE('',(#19811),#5885,.F.) ;
#67097=ADVANCED_FACE('',(#19812),#5886,.F.) ;
#67098=ADVANCED_FACE('',(#19813),#5887,.F.) ;
#67099=ADVANCED_FACE('',(#19814),#5888,.F.) ;
#67100=ADVANCED_FACE('',(#19815),#5889,.F.) ;
#67101=ADVANCED_FACE('',(#19816),#5890,.F.) ;
#67102=ADVANCED_FACE('',(#19817),#5891,.F.) ;
#67103=ADVANCED_FACE('',(#19818),#5892,.F.) ;
#67104=ADVANCED_FACE('',(#19819),#5893,.F.) ;
#67105=ADVANCED_FACE('',(#19820),#5894,.F.) ;
#67106=ADVANCED_FACE('',(#19821),#5895,.F.) ;
#67107=ADVANCED_FACE('',(#19822),#5896,.F.) ;
#67108=ADVANCED_FACE('',(#19823),#5897,.F.) ;
#67109=ADVANCED_FACE('',(#19824),#5898,.F.) ;
#67110=ADVANCED_FACE('',(#19825),#5899,.F.) ;
#67111=ADVANCED_FACE('',(#19826),#5900,.F.) ;
#67112=ADVANCED_FACE('',(#19827),#5901,.F.) ;
#67113=ADVANCED_FACE('',(#19828),#5902,.F.) ;
#67114=ADVANCED_FACE('',(#19829),#5903,.F.) ;
#67115=ADVANCED_FACE('',(#19830),#5904,.F.) ;
#67116=ADVANCED_FACE('',(#19831),#5905,.F.) ;
#67117=ADVANCED_FACE('',(#19832),#5906,.F.) ;
#67118=ADVANCED_FACE('',(#19833),#5907,.F.) ;
#67119=ADVANCED_FACE('',(#19834),#5908,.F.) ;
#67120=ADVANCED_FACE('',(#19835),#5909,.F.) ;
#67121=ADVANCED_FACE('',(#19836),#5910,.F.) ;
#67122=ADVANCED_FACE('',(#19837),#5911,.F.) ;
#67123=ADVANCED_FACE('',(#19838),#5912,.F.) ;
#67124=ADVANCED_FACE('',(#19839),#7578,.T.) ;
#67125=ADVANCED_FACE('',(#19840),#7579,.T.) ;
#67126=ADVANCED_FACE('',(#19841),#4695,.T.) ;
#67127=ADVANCED_FACE('',(#19842),#7580,.T.) ;
#67128=ADVANCED_FACE('',(#19843),#7581,.T.) ;
#67129=ADVANCED_FACE('',(#19844),#7582,.T.) ;
#67130=ADVANCED_FACE('',(#19845),#4696,.T.) ;
#67131=ADVANCED_FACE('',(#19846),#4697,.T.) ;
#67132=ADVANCED_FACE('',(#19847),#7583,.T.) ;
#67133=ADVANCED_FACE('',(#19848),#7584,.T.) ;
#67134=ADVANCED_FACE('',(#19849),#7585,.T.) ;
#67135=ADVANCED_FACE('',(#19850),#4698,.T.) ;
#67136=ADVANCED_FACE('',(#19851),#7586,.T.) ;
#67137=ADVANCED_FACE('',(#19852),#7587,.T.) ;
#67138=ADVANCED_FACE('',(#19853),#7588,.T.) ;
#67139=ADVANCED_FACE('',(#19854),#7589,.T.) ;
#67140=ADVANCED_FACE('',(#19855),#4699,.T.) ;
#67141=ADVANCED_FACE('',(#19856),#7590,.T.) ;
#67142=ADVANCED_FACE('',(#19857),#7591,.T.) ;
#67143=ADVANCED_FACE('',(#19858),#7592,.T.) ;
#67144=ADVANCED_FACE('',(#19859),#4700,.T.) ;
#67145=ADVANCED_FACE('',(#19860),#4701,.T.) ;
#67146=ADVANCED_FACE('',(#19861),#7593,.T.) ;
#67147=ADVANCED_FACE('',(#19862),#7594,.T.) ;
#67148=ADVANCED_FACE('',(#19863),#7595,.T.) ;
#67149=ADVANCED_FACE('',(#19864),#4702,.T.) ;
#67150=ADVANCED_FACE('',(#19865),#7596,.T.) ;
#67151=ADVANCED_FACE('',(#19866),#7597,.T.) ;
#67152=ADVANCED_FACE('',(#19867),#7598,.T.) ;
#67153=ADVANCED_FACE('',(#19868),#7599,.T.) ;
#67154=ADVANCED_FACE('',(#19869),#4703,.T.) ;
#67155=ADVANCED_FACE('',(#19870),#7600,.T.) ;
#67156=ADVANCED_FACE('',(#19871),#7601,.T.) ;
#67157=ADVANCED_FACE('',(#19872),#7602,.T.) ;
#67158=ADVANCED_FACE('',(#19873),#4704,.T.) ;
#67159=ADVANCED_FACE('',(#19874),#4705,.T.) ;
#67160=ADVANCED_FACE('',(#19875),#7603,.T.) ;
#67161=ADVANCED_FACE('',(#19876),#7604,.T.) ;
#67162=ADVANCED_FACE('',(#19877),#7605,.T.) ;
#67163=ADVANCED_FACE('',(#19878),#4706,.T.) ;
#67164=ADVANCED_FACE('',(#19879),#7606,.T.) ;
#67165=ADVANCED_FACE('',(#19880),#7607,.T.) ;
#67166=ADVANCED_FACE('',(#19881),#7608,.T.) ;
#67167=ADVANCED_FACE('',(#19882),#7609,.T.) ;
#67168=ADVANCED_FACE('',(#19883),#4707,.T.) ;
#67169=ADVANCED_FACE('',(#19884),#7610,.T.) ;
#67170=ADVANCED_FACE('',(#19885),#7611,.T.) ;
#67171=ADVANCED_FACE('',(#19886),#7612,.T.) ;
#67172=ADVANCED_FACE('',(#19887),#4708,.T.) ;
#67173=ADVANCED_FACE('',(#19888),#4709,.T.) ;
#67174=ADVANCED_FACE('',(#19889),#7613,.T.) ;
#67175=ADVANCED_FACE('',(#19890),#7614,.T.) ;
#67176=ADVANCED_FACE('',(#19891),#7615,.T.) ;
#67177=ADVANCED_FACE('',(#19892),#4710,.T.) ;
#67178=ADVANCED_FACE('',(#19893),#7616,.T.) ;
#67179=ADVANCED_FACE('',(#19894),#7617,.T.) ;
#67180=ADVANCED_FACE('',(#19895),#7618,.T.) ;
#67181=ADVANCED_FACE('',(#19896),#7619,.T.) ;
#67182=ADVANCED_FACE('',(#19897),#4711,.T.) ;
#67183=ADVANCED_FACE('',(#19898),#7620,.T.) ;
#67184=ADVANCED_FACE('',(#19899),#7621,.T.) ;
#67185=ADVANCED_FACE('',(#19900),#7622,.T.) ;
#67186=ADVANCED_FACE('',(#19901),#4712,.T.) ;
#67187=ADVANCED_FACE('',(#19902),#4713,.T.) ;
#67188=ADVANCED_FACE('',(#19903),#7623,.T.) ;
#67189=ADVANCED_FACE('',(#19904),#7624,.T.) ;
#67190=ADVANCED_FACE('',(#19905),#7625,.T.) ;
#67191=ADVANCED_FACE('',(#19906),#4714,.T.) ;
#67192=ADVANCED_FACE('',(#19907),#7626,.T.) ;
#67193=ADVANCED_FACE('',(#19908),#7627,.T.) ;
#67194=ADVANCED_FACE('',(#19909),#7628,.T.) ;
#67195=ADVANCED_FACE('',(#19910),#7629,.T.) ;
#67196=ADVANCED_FACE('',(#19911),#4715,.T.) ;
#67197=ADVANCED_FACE('',(#19912),#7630,.T.) ;
#67198=ADVANCED_FACE('',(#19913),#7631,.T.) ;
#67199=ADVANCED_FACE('',(#19914),#7632,.T.) ;
#67200=ADVANCED_FACE('',(#19915),#4716,.T.) ;
#67201=ADVANCED_FACE('',(#19916),#4717,.T.) ;
#67202=ADVANCED_FACE('',(#19917),#7633,.T.) ;
#67203=ADVANCED_FACE('',(#19918),#7634,.T.) ;
#67204=ADVANCED_FACE('',(#19919),#7635,.T.) ;
#67205=ADVANCED_FACE('',(#19920),#4718,.T.) ;
#67206=ADVANCED_FACE('',(#19921),#7636,.T.) ;
#67207=ADVANCED_FACE('',(#19922),#7637,.T.) ;
#67208=ADVANCED_FACE('',(#19923),#7638,.T.) ;
#67209=ADVANCED_FACE('',(#19924),#7639,.T.) ;
#67210=ADVANCED_FACE('',(#19925),#4719,.T.) ;
#67211=ADVANCED_FACE('',(#19926),#7640,.T.) ;
#67212=ADVANCED_FACE('',(#19927),#7641,.T.) ;
#67213=ADVANCED_FACE('',(#19928),#7642,.T.) ;
#67214=ADVANCED_FACE('',(#19929),#4720,.T.) ;
#67215=ADVANCED_FACE('',(#19930),#4721,.T.) ;
#67216=ADVANCED_FACE('',(#19931),#7643,.T.) ;
#67217=ADVANCED_FACE('',(#19932),#7644,.T.) ;
#67218=ADVANCED_FACE('',(#19933),#7645,.T.) ;
#67219=ADVANCED_FACE('',(#19934),#4722,.T.) ;
#67220=ADVANCED_FACE('',(#19935),#7646,.T.) ;
#67221=ADVANCED_FACE('',(#19936),#7647,.T.) ;
#67222=ADVANCED_FACE('',(#19937),#7648,.T.) ;
#67223=ADVANCED_FACE('',(#19938),#7649,.T.) ;
#67224=ADVANCED_FACE('',(#19939),#4723,.T.) ;
#67225=ADVANCED_FACE('',(#19940),#7650,.T.) ;
#67226=ADVANCED_FACE('',(#19941),#7651,.T.) ;
#67227=ADVANCED_FACE('',(#19942),#7652,.T.) ;
#67228=ADVANCED_FACE('',(#19943),#4724,.T.) ;
#67229=ADVANCED_FACE('',(#19944),#4725,.T.) ;
#67230=ADVANCED_FACE('',(#19945),#7653,.T.) ;
#67231=ADVANCED_FACE('',(#19946),#7654,.T.) ;
#67232=ADVANCED_FACE('',(#19947),#7655,.T.) ;
#67233=ADVANCED_FACE('',(#19948),#4726,.T.) ;
#67234=ADVANCED_FACE('',(#19949),#7656,.T.) ;
#67235=ADVANCED_FACE('',(#19950),#7657,.T.) ;
#67236=ADVANCED_FACE('',(#19951),#7658,.T.) ;
#67237=ADVANCED_FACE('',(#19952),#7659,.T.) ;
#67238=ADVANCED_FACE('',(#19953),#4727,.T.) ;
#67239=ADVANCED_FACE('',(#19954),#7660,.T.) ;
#67240=ADVANCED_FACE('',(#19955),#7661,.T.) ;
#67241=ADVANCED_FACE('',(#19956),#7662,.T.) ;
#67242=ADVANCED_FACE('',(#19957),#4728,.T.) ;
#67243=ADVANCED_FACE('',(#19958),#4729,.T.) ;
#67244=ADVANCED_FACE('',(#19959),#7663,.T.) ;
#67245=ADVANCED_FACE('',(#19960),#7664,.T.) ;
#67246=ADVANCED_FACE('',(#19961),#7665,.T.) ;
#67247=ADVANCED_FACE('',(#19962),#4730,.T.) ;
#67248=ADVANCED_FACE('',(#19963),#7666,.T.) ;
#67249=ADVANCED_FACE('',(#19964),#7667,.T.) ;
#67250=ADVANCED_FACE('',(#19965),#7668,.T.) ;
#67251=ADVANCED_FACE('',(#19966),#7669,.T.) ;
#67252=ADVANCED_FACE('',(#19967),#4731,.T.) ;
#67253=ADVANCED_FACE('',(#19968),#7670,.T.) ;
#67254=ADVANCED_FACE('',(#19969),#7671,.T.) ;
#67255=ADVANCED_FACE('',(#19970),#7672,.T.) ;
#67256=ADVANCED_FACE('',(#19971),#4732,.T.) ;
#67257=ADVANCED_FACE('',(#19972),#4733,.T.) ;
#67258=ADVANCED_FACE('',(#19973),#7673,.T.) ;
#67259=ADVANCED_FACE('',(#19974),#7674,.T.) ;
#67260=ADVANCED_FACE('',(#19975),#7675,.T.) ;
#67261=ADVANCED_FACE('',(#19976),#4734,.T.) ;
#67262=ADVANCED_FACE('',(#19977),#7676,.T.) ;
#67263=ADVANCED_FACE('',(#19978),#7677,.T.) ;
#67264=ADVANCED_FACE('',(#19979),#7678,.T.) ;
#67265=ADVANCED_FACE('',(#19980),#7679,.T.) ;
#67266=ADVANCED_FACE('',(#19981),#4735,.T.) ;
#67267=ADVANCED_FACE('',(#19982),#7680,.T.) ;
#67268=ADVANCED_FACE('',(#19983),#7681,.T.) ;
#67269=ADVANCED_FACE('',(#19984),#7682,.T.) ;
#67270=ADVANCED_FACE('',(#19985),#4736,.T.) ;
#67271=ADVANCED_FACE('',(#19986),#4737,.T.) ;
#67272=ADVANCED_FACE('',(#19987),#7683,.T.) ;
#67273=ADVANCED_FACE('',(#19988),#7684,.T.) ;
#67274=ADVANCED_FACE('',(#19989),#7685,.T.) ;
#67275=ADVANCED_FACE('',(#19990),#4738,.T.) ;
#67276=ADVANCED_FACE('',(#19991),#7686,.T.) ;
#67277=ADVANCED_FACE('',(#19992),#7687,.T.) ;
#67278=ADVANCED_FACE('',(#19993),#7688,.T.) ;
#67279=ADVANCED_FACE('',(#19994),#7689,.T.) ;
#67280=ADVANCED_FACE('',(#19995),#4739,.T.) ;
#67281=ADVANCED_FACE('',(#19996),#7690,.T.) ;
#67282=ADVANCED_FACE('',(#19997),#7691,.T.) ;
#67283=ADVANCED_FACE('',(#19998),#7692,.T.) ;
#67284=ADVANCED_FACE('',(#19999),#4740,.T.) ;
#67285=ADVANCED_FACE('',(#20000),#4741,.T.) ;
#67286=ADVANCED_FACE('',(#20001),#7693,.T.) ;
#67287=ADVANCED_FACE('',(#20002),#7694,.T.) ;
#67288=ADVANCED_FACE('',(#20003),#7695,.T.) ;
#67289=ADVANCED_FACE('',(#20004),#4742,.T.) ;
#67290=ADVANCED_FACE('',(#20005),#7696,.T.) ;
#67291=ADVANCED_FACE('',(#20006),#7697,.T.) ;
#67292=ADVANCED_FACE('',(#20007),#7698,.T.) ;
#67293=ADVANCED_FACE('',(#20008),#7699,.T.) ;
#67294=ADVANCED_FACE('',(#20009),#4743,.T.) ;
#67295=ADVANCED_FACE('',(#20010),#7700,.T.) ;
#67296=ADVANCED_FACE('',(#20011),#7701,.T.) ;
#67297=ADVANCED_FACE('',(#20012),#7702,.T.) ;
#67298=ADVANCED_FACE('',(#20013),#4744,.T.) ;
#67299=ADVANCED_FACE('',(#20014),#4745,.T.) ;
#67300=ADVANCED_FACE('',(#20015),#7703,.T.) ;
#67301=ADVANCED_FACE('',(#20016),#7704,.T.) ;
#67302=ADVANCED_FACE('',(#20017),#7705,.T.) ;
#67303=ADVANCED_FACE('',(#20018),#4746,.T.) ;
#67304=ADVANCED_FACE('',(#20019),#7706,.T.) ;
#67305=ADVANCED_FACE('',(#20020),#7707,.T.) ;
#67306=ADVANCED_FACE('',(#20021),#7708,.T.) ;
#67307=ADVANCED_FACE('',(#20022),#7709,.T.) ;
#67308=ADVANCED_FACE('',(#20023),#4747,.T.) ;
#67309=ADVANCED_FACE('',(#20024),#7710,.T.) ;
#67310=ADVANCED_FACE('',(#20025),#7711,.T.) ;
#67311=ADVANCED_FACE('',(#20026),#7712,.T.) ;
#67312=ADVANCED_FACE('',(#20027),#4748,.T.) ;
#67313=ADVANCED_FACE('',(#20028),#4749,.T.) ;
#67314=ADVANCED_FACE('',(#20029),#7713,.T.) ;
#67315=ADVANCED_FACE('',(#20030),#7714,.T.) ;
#67316=ADVANCED_FACE('',(#20031),#7715,.T.) ;
#67317=ADVANCED_FACE('',(#20032),#4750,.T.) ;
#67318=ADVANCED_FACE('',(#20033),#7716,.T.) ;
#67319=ADVANCED_FACE('',(#20034),#7717,.T.) ;
#67320=ADVANCED_FACE('',(#20035),#7718,.T.) ;
#67321=ADVANCED_FACE('',(#20036),#7719,.T.) ;
#67322=ADVANCED_FACE('',(#20037),#4751,.T.) ;
#67323=ADVANCED_FACE('',(#20038),#7720,.T.) ;
#67324=ADVANCED_FACE('',(#20039),#7721,.T.) ;
#67325=ADVANCED_FACE('',(#20040),#7722,.T.) ;
#67326=ADVANCED_FACE('',(#20041),#4752,.T.) ;
#67327=ADVANCED_FACE('',(#20042),#4753,.T.) ;
#67328=ADVANCED_FACE('',(#20043),#7723,.T.) ;
#67329=ADVANCED_FACE('',(#20044),#7724,.T.) ;
#67330=ADVANCED_FACE('',(#20045),#7725,.T.) ;
#67331=ADVANCED_FACE('',(#20046),#4754,.T.) ;
#67332=ADVANCED_FACE('',(#20047),#7726,.T.) ;
#67333=ADVANCED_FACE('',(#20048),#7727,.T.) ;
#67334=ADVANCED_FACE('',(#20049),#7728,.T.) ;
#67335=ADVANCED_FACE('',(#20050),#7729,.T.) ;
#67336=ADVANCED_FACE('',(#20051),#4755,.T.) ;
#67337=ADVANCED_FACE('',(#20052),#7730,.T.) ;
#67338=ADVANCED_FACE('',(#20053),#7731,.T.) ;
#67339=ADVANCED_FACE('',(#20054),#7732,.T.) ;
#67340=ADVANCED_FACE('',(#20055),#4756,.T.) ;
#67341=ADVANCED_FACE('',(#20056),#4757,.T.) ;
#67342=ADVANCED_FACE('',(#20057),#7733,.T.) ;
#67343=ADVANCED_FACE('',(#20058),#7734,.T.) ;
#67344=ADVANCED_FACE('',(#20059),#7735,.T.) ;
#67345=ADVANCED_FACE('',(#20060),#4758,.T.) ;
#67346=ADVANCED_FACE('',(#20061),#7736,.T.) ;
#67347=ADVANCED_FACE('',(#20062),#7737,.T.) ;
#67348=ADVANCED_FACE('',(#20063),#7738,.T.) ;
#67349=ADVANCED_FACE('',(#20064),#7739,.T.) ;
#67350=ADVANCED_FACE('',(#20065),#4759,.T.) ;
#67351=ADVANCED_FACE('',(#20066),#7740,.T.) ;
#67352=ADVANCED_FACE('',(#20067),#7741,.T.) ;
#67353=ADVANCED_FACE('',(#20068),#7742,.T.) ;
#67354=ADVANCED_FACE('',(#20069),#4760,.T.) ;
#67355=ADVANCED_FACE('',(#20070),#4761,.T.) ;
#67356=ADVANCED_FACE('',(#20071),#7743,.T.) ;
#67357=ADVANCED_FACE('',(#20072),#7744,.T.) ;
#67358=ADVANCED_FACE('',(#20073),#7745,.T.) ;
#67359=ADVANCED_FACE('',(#20074),#4762,.T.) ;
#67360=ADVANCED_FACE('',(#20075),#7746,.T.) ;
#67361=ADVANCED_FACE('',(#20076),#7747,.T.) ;
#67362=ADVANCED_FACE('',(#20077),#7748,.T.) ;
#67363=ADVANCED_FACE('',(#20078),#7749,.T.) ;
#67364=ADVANCED_FACE('',(#20079),#4763,.T.) ;
#67365=ADVANCED_FACE('',(#20080),#7750,.T.) ;
#67366=ADVANCED_FACE('',(#20081),#7751,.T.) ;
#67367=ADVANCED_FACE('',(#20082),#7752,.T.) ;
#67368=ADVANCED_FACE('',(#20083),#4764,.T.) ;
#67369=ADVANCED_FACE('',(#20084),#4765,.T.) ;
#67370=ADVANCED_FACE('',(#20085),#7753,.T.) ;
#67371=ADVANCED_FACE('',(#20086),#7754,.T.) ;
#67372=ADVANCED_FACE('',(#20087),#7755,.T.) ;
#67373=ADVANCED_FACE('',(#20088),#4766,.T.) ;
#67374=ADVANCED_FACE('',(#20089),#7756,.T.) ;
#67375=ADVANCED_FACE('',(#20090),#7757,.T.) ;
#67376=ADVANCED_FACE('',(#20091),#63405,.T.) ;
#67377=ADVANCED_FACE('',(#20092),#7758,.T.) ;
#67378=ADVANCED_FACE('',(#20093),#4767,.T.) ;
#67379=ADVANCED_FACE('',(#20094),#7759,.T.) ;
#67380=ADVANCED_FACE('',(#20095),#4768,.T.) ;
#67381=ADVANCED_FACE('',(#20096),#7760,.T.) ;
#67382=ADVANCED_FACE('',(#20097),#63406,.T.) ;
#67383=ADVANCED_FACE('',(#20098),#63407,.T.) ;
#67384=ADVANCED_FACE('',(#20099),#7761,.T.) ;
#67385=ADVANCED_FACE('',(#20100),#4769,.T.) ;
#67386=ADVANCED_FACE('',(#20101),#7762,.T.) ;
#67387=ADVANCED_FACE('',(#20102),#4770,.T.) ;
#67388=ADVANCED_FACE('',(#20103),#7763,.T.) ;
#67389=ADVANCED_FACE('',(#20104),#63408,.T.) ;
#67390=ADVANCED_FACE('',(#20105),#7764,.T.) ;
#67391=ADVANCED_FACE('',(#20106),#4771,.T.) ;
#67392=ADVANCED_FACE('',(#20107),#7765,.T.) ;
#67393=ADVANCED_FACE('',(#20108),#4772,.T.) ;
#67394=ADVANCED_FACE('',(#20109),#7766,.T.) ;
#67395=ADVANCED_FACE('',(#20110),#7767,.T.) ;
#67396=ADVANCED_FACE('',(#20111),#4773,.T.) ;
#67397=ADVANCED_FACE('',(#20112),#7768,.T.) ;
#67398=ADVANCED_FACE('',(#20113),#7769,.T.) ;
#67399=ADVANCED_FACE('',(#20114),#4774,.T.) ;
#67400=ADVANCED_FACE('',(#20115),#63409,.T.) ;
#67401=ADVANCED_FACE('',(#20116),#7770,.T.) ;
#67402=ADVANCED_FACE('',(#20117),#4775,.T.) ;
#67403=ADVANCED_FACE('',(#20118),#7771,.T.) ;
#67404=ADVANCED_FACE('',(#20119),#4776,.T.) ;
#67405=ADVANCED_FACE('',(#20120),#7772,.T.) ;
#67406=ADVANCED_FACE('',(#20121),#63410,.T.) ;
#67407=ADVANCED_FACE('',(#20122),#63411,.T.) ;
#67408=ADVANCED_FACE('',(#20123),#7773,.T.) ;
#67409=ADVANCED_FACE('',(#20124),#4777,.T.) ;
#67410=ADVANCED_FACE('',(#20125),#7774,.T.) ;
#67411=ADVANCED_FACE('',(#20126),#4778,.T.) ;
#67412=ADVANCED_FACE('',(#20127),#7775,.T.) ;
#67413=ADVANCED_FACE('',(#20128),#63412,.T.) ;
#67414=ADVANCED_FACE('',(#20129),#7776,.T.) ;
#67415=ADVANCED_FACE('',(#20130),#4779,.T.) ;
#67416=ADVANCED_FACE('',(#20131),#7777,.T.) ;
#67417=ADVANCED_FACE('',(#20132),#4780,.T.) ;
#67418=ADVANCED_FACE('',(#20133),#7778,.T.) ;
#67419=ADVANCED_FACE('',(#20134),#7779,.T.) ;
#67420=ADVANCED_FACE('',(#20135),#4781,.T.) ;
#67421=ADVANCED_FACE('',(#20136),#7780,.T.) ;
#67422=ADVANCED_FACE('',(#20137),#7781,.T.) ;
#67423=ADVANCED_FACE('',(#20138),#4782,.T.) ;
#67424=ADVANCED_FACE('',(#20139),#63413,.T.) ;
#67425=ADVANCED_FACE('',(#20140),#7782,.T.) ;
#67426=ADVANCED_FACE('',(#20141),#4783,.T.) ;
#67427=ADVANCED_FACE('',(#20142),#7783,.T.) ;
#67428=ADVANCED_FACE('',(#20143),#4784,.T.) ;
#67429=ADVANCED_FACE('',(#20144),#7784,.T.) ;
#67430=ADVANCED_FACE('',(#20145),#63414,.T.) ;
#67431=ADVANCED_FACE('',(#20146),#63415,.T.) ;
#67432=ADVANCED_FACE('',(#20147),#7785,.T.) ;
#67433=ADVANCED_FACE('',(#20148),#4785,.T.) ;
#67434=ADVANCED_FACE('',(#20149),#7786,.T.) ;
#67435=ADVANCED_FACE('',(#20150),#4786,.T.) ;
#67436=ADVANCED_FACE('',(#20151),#7787,.T.) ;
#67437=ADVANCED_FACE('',(#20152),#63416,.T.) ;
#67438=ADVANCED_FACE('',(#20153),#7788,.T.) ;
#67439=ADVANCED_FACE('',(#20154),#4787,.T.) ;
#67440=ADVANCED_FACE('',(#20155),#7789,.T.) ;
#67441=ADVANCED_FACE('',(#20156),#4788,.T.) ;
#67442=ADVANCED_FACE('',(#20157),#7790,.T.) ;
#67443=ADVANCED_FACE('',(#20158),#7791,.T.) ;
#67444=ADVANCED_FACE('',(#20159),#4789,.T.) ;
#67445=ADVANCED_FACE('',(#20160),#7792,.T.) ;
#67446=ADVANCED_FACE('',(#20161),#7793,.T.) ;
#67447=ADVANCED_FACE('',(#20162),#4790,.T.) ;
#67448=ADVANCED_FACE('',(#20163),#63417,.T.) ;
#67449=ADVANCED_FACE('',(#20164),#7794,.T.) ;
#67450=ADVANCED_FACE('',(#20165),#4791,.T.) ;
#67451=ADVANCED_FACE('',(#20166),#7795,.T.) ;
#67452=ADVANCED_FACE('',(#20167),#4792,.T.) ;
#67453=ADVANCED_FACE('',(#20168),#7796,.T.) ;
#67454=ADVANCED_FACE('',(#20169),#63418,.T.) ;
#67455=ADVANCED_FACE('',(#20170),#63419,.T.) ;
#67456=ADVANCED_FACE('',(#20171),#7797,.T.) ;
#67457=ADVANCED_FACE('',(#20172),#4793,.T.) ;
#67458=ADVANCED_FACE('',(#20173),#7798,.T.) ;
#67459=ADVANCED_FACE('',(#20174),#4794,.T.) ;
#67460=ADVANCED_FACE('',(#20175),#7799,.T.) ;
#67461=ADVANCED_FACE('',(#20176),#63420,.T.) ;
#67462=ADVANCED_FACE('',(#20177),#7800,.T.) ;
#67463=ADVANCED_FACE('',(#20178),#4795,.T.) ;
#67464=ADVANCED_FACE('',(#20179),#7801,.T.) ;
#67465=ADVANCED_FACE('',(#20180),#4796,.T.) ;
#67466=ADVANCED_FACE('',(#20181),#7802,.T.) ;
#67467=ADVANCED_FACE('',(#20182),#7803,.T.) ;
#67468=ADVANCED_FACE('',(#20183),#4797,.T.) ;
#67469=ADVANCED_FACE('',(#20184),#7804,.T.) ;
#67470=ADVANCED_FACE('',(#20185),#7805,.T.) ;
#67471=ADVANCED_FACE('',(#20186),#4798,.T.) ;
#67472=ADVANCED_FACE('',(#20187),#63421,.T.) ;
#67473=ADVANCED_FACE('',(#20188),#7806,.T.) ;
#67474=ADVANCED_FACE('',(#20189),#4799,.T.) ;
#67475=ADVANCED_FACE('',(#20190),#7807,.T.) ;
#67476=ADVANCED_FACE('',(#20191),#4800,.T.) ;
#67477=ADVANCED_FACE('',(#20192),#7808,.T.) ;
#67478=ADVANCED_FACE('',(#20193),#63422,.T.) ;
#67479=ADVANCED_FACE('',(#20194),#63423,.T.) ;
#67480=ADVANCED_FACE('',(#20195),#7809,.T.) ;
#67481=ADVANCED_FACE('',(#20196),#4801,.T.) ;
#67482=ADVANCED_FACE('',(#20197),#7810,.T.) ;
#67483=ADVANCED_FACE('',(#20198),#4802,.T.) ;
#67484=ADVANCED_FACE('',(#20199),#7811,.T.) ;
#67485=ADVANCED_FACE('',(#20200),#63424,.T.) ;
#67486=ADVANCED_FACE('',(#20201),#7812,.T.) ;
#67487=ADVANCED_FACE('',(#20202),#4803,.T.) ;
#67488=ADVANCED_FACE('',(#20203),#7813,.T.) ;
#67489=ADVANCED_FACE('',(#20204),#4804,.T.) ;
#67490=ADVANCED_FACE('',(#20205),#7814,.T.) ;
#67491=ADVANCED_FACE('',(#20206),#7815,.T.) ;
#67492=ADVANCED_FACE('',(#20207),#4805,.T.) ;
#67493=ADVANCED_FACE('',(#20208),#7816,.T.) ;
#67494=ADVANCED_FACE('',(#20209),#7817,.T.) ;
#67495=ADVANCED_FACE('',(#20210),#4806,.T.) ;
#67496=ADVANCED_FACE('',(#20211),#63425,.T.) ;
#67497=ADVANCED_FACE('',(#20212),#7818,.T.) ;
#67498=ADVANCED_FACE('',(#20213),#4807,.T.) ;
#67499=ADVANCED_FACE('',(#20214),#7819,.T.) ;
#67500=ADVANCED_FACE('',(#20215),#4808,.T.) ;
#67501=ADVANCED_FACE('',(#20216),#7820,.T.) ;
#67502=ADVANCED_FACE('',(#20217),#63426,.T.) ;
#67503=ADVANCED_FACE('',(#20218),#63427,.T.) ;
#67504=ADVANCED_FACE('',(#20219),#7821,.T.) ;
#67505=ADVANCED_FACE('',(#20220),#4809,.T.) ;
#67506=ADVANCED_FACE('',(#20221),#7822,.T.) ;
#67507=ADVANCED_FACE('',(#20222),#4810,.T.) ;
#67508=ADVANCED_FACE('',(#20223),#7823,.T.) ;
#67509=ADVANCED_FACE('',(#20224),#63428,.T.) ;
#67510=ADVANCED_FACE('',(#20225),#7824,.T.) ;
#67511=ADVANCED_FACE('',(#20226),#4811,.T.) ;
#67512=ADVANCED_FACE('',(#20227),#7825,.T.) ;
#67513=ADVANCED_FACE('',(#20228),#4812,.T.) ;
#67514=ADVANCED_FACE('',(#20229),#7826,.T.) ;
#67515=ADVANCED_FACE('',(#20230),#7827,.T.) ;
#67516=ADVANCED_FACE('',(#20231),#4813,.T.) ;
#67517=ADVANCED_FACE('',(#20232),#7828,.T.) ;
#67518=ADVANCED_FACE('',(#20233),#7829,.T.) ;
#67519=ADVANCED_FACE('',(#20234),#4814,.T.) ;
#67520=ADVANCED_FACE('',(#20235),#63429,.T.) ;
#67521=ADVANCED_FACE('',(#20236),#7830,.T.) ;
#67522=ADVANCED_FACE('',(#20237),#4815,.T.) ;
#67523=ADVANCED_FACE('',(#20238),#7831,.T.) ;
#67524=ADVANCED_FACE('',(#20239),#4816,.T.) ;
#67525=ADVANCED_FACE('',(#20240),#7832,.T.) ;
#67526=ADVANCED_FACE('',(#20241),#63430,.T.) ;
#67527=ADVANCED_FACE('',(#20242),#63431,.T.) ;
#67528=ADVANCED_FACE('',(#20243),#7833,.T.) ;
#67529=ADVANCED_FACE('',(#20244),#4817,.T.) ;
#67530=ADVANCED_FACE('',(#20245),#7834,.T.) ;
#67531=ADVANCED_FACE('',(#20246),#4818,.T.) ;
#67532=ADVANCED_FACE('',(#20247),#7835,.T.) ;
#67533=ADVANCED_FACE('',(#20248),#63432,.T.) ;
#67534=ADVANCED_FACE('',(#20249),#7836,.T.) ;
#67535=ADVANCED_FACE('',(#20250),#4819,.T.) ;
#67536=ADVANCED_FACE('',(#20251),#7837,.T.) ;
#67537=ADVANCED_FACE('',(#20252),#4820,.T.) ;
#67538=ADVANCED_FACE('',(#20253),#7838,.T.) ;
#67539=ADVANCED_FACE('',(#20254),#7839,.T.) ;
#67540=ADVANCED_FACE('',(#20255),#4821,.T.) ;
#67541=ADVANCED_FACE('',(#20256),#7840,.T.) ;
#67542=ADVANCED_FACE('',(#20257),#7841,.T.) ;
#67543=ADVANCED_FACE('',(#20258),#4822,.T.) ;
#67544=ADVANCED_FACE('',(#20259),#63433,.T.) ;
#67545=ADVANCED_FACE('',(#20260),#7842,.T.) ;
#67546=ADVANCED_FACE('',(#20261),#4823,.T.) ;
#67547=ADVANCED_FACE('',(#20262),#7843,.T.) ;
#67548=ADVANCED_FACE('',(#20263),#4824,.T.) ;
#67549=ADVANCED_FACE('',(#20264),#7844,.T.) ;
#67550=ADVANCED_FACE('',(#20265),#63434,.T.) ;
#67551=ADVANCED_FACE('',(#20266),#63435,.T.) ;
#67552=ADVANCED_FACE('',(#20267),#7845,.T.) ;
#67553=ADVANCED_FACE('',(#20268),#4825,.T.) ;
#67554=ADVANCED_FACE('',(#20269),#7846,.T.) ;
#67555=ADVANCED_FACE('',(#20270),#4826,.T.) ;
#67556=ADVANCED_FACE('',(#20271),#7847,.T.) ;
#67557=ADVANCED_FACE('',(#20272),#63436,.T.) ;
#67558=ADVANCED_FACE('',(#20273),#7848,.T.) ;
#67559=ADVANCED_FACE('',(#20274),#4827,.T.) ;
#67560=ADVANCED_FACE('',(#20275),#7849,.T.) ;
#67561=ADVANCED_FACE('',(#20276),#4828,.T.) ;
#67562=ADVANCED_FACE('',(#20277),#7850,.T.) ;
#67563=ADVANCED_FACE('',(#20278),#7851,.T.) ;
#67564=ADVANCED_FACE('',(#20279),#4829,.T.) ;
#67565=ADVANCED_FACE('',(#20280),#7852,.T.) ;
#67566=ADVANCED_FACE('',(#20281),#7853,.T.) ;
#67567=ADVANCED_FACE('',(#20282),#4830,.T.) ;
#67568=ADVANCED_FACE('',(#20283),#63437,.T.) ;
#67569=ADVANCED_FACE('',(#20284),#7854,.T.) ;
#67570=ADVANCED_FACE('',(#20285),#4831,.T.) ;
#67571=ADVANCED_FACE('',(#20286),#7855,.T.) ;
#67572=ADVANCED_FACE('',(#20287),#4832,.T.) ;
#67573=ADVANCED_FACE('',(#20288),#7856,.T.) ;
#67574=ADVANCED_FACE('',(#20289),#63438,.T.) ;
#67575=ADVANCED_FACE('',(#20290),#63439,.T.) ;
#67576=ADVANCED_FACE('',(#20291),#7857,.T.) ;
#67577=ADVANCED_FACE('',(#20292),#4833,.T.) ;
#67578=ADVANCED_FACE('',(#20293),#7858,.T.) ;
#67579=ADVANCED_FACE('',(#20294),#4834,.T.) ;
#67580=ADVANCED_FACE('',(#20295),#7859,.T.) ;
#67581=ADVANCED_FACE('',(#20296),#63440,.T.) ;
#67582=ADVANCED_FACE('',(#20297),#7860,.T.) ;
#67583=ADVANCED_FACE('',(#20298),#4835,.T.) ;
#67584=ADVANCED_FACE('',(#20299),#7861,.T.) ;
#67585=ADVANCED_FACE('',(#20300),#4836,.T.) ;
#67586=ADVANCED_FACE('',(#20301),#7862,.T.) ;
#67587=ADVANCED_FACE('',(#20302),#7863,.T.) ;
#67588=ADVANCED_FACE('',(#20303),#4837,.T.) ;
#67589=ADVANCED_FACE('',(#20304),#7864,.T.) ;
#67590=ADVANCED_FACE('',(#20305),#7865,.T.) ;
#67591=ADVANCED_FACE('',(#20306),#4838,.T.) ;
#67693=CLOSED_SHELL('',(#65362,#65363,#65364,#65365,#65366,#65367,#65368,
#65369,#65370,#65371,#65372,#65373,#65374,#65375,#65376,#65377,#65378,#65379,
#65380,#65381,#65382,#65383,#65384,#65385,#65386,#65387,#65388,#65389,#65390,
#65391,#65392,#65393,#65394,#65395,#65396,#65397,#65398,#65399,#65400,#65401,
#65402,#65403,#65404,#65405,#65406,#65407,#65408,#65409,#65410,#65411,#65412,
#65413,#65414,#65415,#65416,#65417,#65418,#65419,#65420,#65421,#65422,#65423,
#65424,#65425,#65426,#65427,#65428,#65429,#65430,#65431,#65432,#65433,#65434,
#65435,#65436,#65437,#65438,#65439,#65440,#65441,#65442,#65443,#65444,#65445,
#65446,#65447,#65448,#65449,#65450,#65451,#65452,#65453,#65454,#65455,#65456,
#65457,#65458,#65459,#65460,#65461,#65462,#65463,#65464,#65465,#65466,#65467,
#65468,#65469,#65470,#65471,#65472,#65473,#65474,#65475,#65476,#65477,#65478,
#65479,#65480,#65481,#65482,#65483,#65484,#65485,#65486,#65487,#65488,#65489,
#65490,#65491,#65492,#65493,#65494,#65495,#65496,#65497,#65498,#65499,#65500,
#65501,#65502,#65503,#65504,#65505,#65506,#65507,#65508,#65509,#65510,#65511,
#65512,#65513,#65514,#65515,#65516,#65517,#65518,#65519,#65520,#65521,#65522,
#65523,#65524,#65525,#65526,#65527,#65528,#65529,#65530,#65531,#65532,#65533,
#65534,#65535,#65536,#65537,#65538,#65539,#65540,#65541,#65542,#65543,#65544,
#65545,#65546,#65547,#65548,#65549,#65550,#65551,#65552,#65553,#65554,#65555,
#65556,#65557,#65558,#65559,#65560,#65561,#65562,#65563,#65564,#65565,#65566,
#65567,#65568,#65569,#65570,#65571,#65572,#65573,#65574,#65575,#65576,#65577,
#65578,#65579,#65580,#65581,#65582,#65583,#65584,#65585,#65586,#65587,#65588,
#65589,#65590,#65591,#65592,#65593,#65594,#65595,#65596,#65597,#65598,#65599,
#65600,#65601,#65602,#65603,#65604,#65605,#65606,#65607,#65608,#65609,#65610,
#65611,#65612,#65613,#65614,#65615,#65616,#65617,#65618,#65619,#65620,#65621,
#65622,#65623,#65624,#65625,#65626,#65627,#65628,#65629,#65630,#65631,#65632,
#65633,#65634,#65635,#65636,#65637,#65638,#65639,#65640,#65641,#65642,#65643,
#65644,#65645,#65646,#65647,#65648,#65649,#65650,#65651,#65652,#65653,#65654,
#65655,#65656,#65657,#65658,#65659,#65660,#65661,#65662,#65663,#65664,#65665,
#65666,#65667,#65668,#65669,#65670,#65671,#65672,#65673,#65674,#65675,#65676,
#65677,#65678,#65679,#65680,#65681,#65682,#65683,#65684,#65685,#65686,#65687,
#65688,#65689,#65690,#65691,#65692,#65693,#65694,#65695,#65696,#65697,#65698,
#65699,#65700,#65701,#65702,#65703,#65704,#65705,#65706,#65707,#65708,#65709,
#65710,#65711,#65712,#65713,#65714,#65715,#65716,#65717,#65718,#65719,#65720,
#65721,#65722,#65723,#65724,#65725,#65726,#65727,#65728,#65729,#65730,#65731,
#65732,#65733,#65734,#65735,#65736,#65737,#65738,#65739,#65740,#65741,#65742,
#65743,#65744,#65745,#65746,#65747,#65748,#65749,#65750,#65751,#65752,#65753,
#65754,#65755,#65756,#65757,#65758,#65759,#65760,#65761,#65762,#65763,#65764,
#65765,#65766,#65767,#65768,#65769,#65770,#65771,#65772,#65773,#65774,#65775,
#65776,#65777,#65778,#65779,#65780,#65781,#65782,#65783,#65784,#65785,#65786,
#65787,#65788,#65789,#65790,#65791,#65792,#65793,#65794,#65795,#65796,#65797,
#65798,#65799,#65800,#65801,#65802,#65803,#65804,#65805,#65806,#65807,#65808,
#65809,#65810,#65811,#65812,#65813,#65814,#65815,#65816,#65817,#65818,#65819,
#65820,#65821,#65822,#65823,#65824,#65825,#65826,#65827,#65828,#65829,#65830,
#65831,#65832,#65833,#65834,#65835,#65836,#65837,#65838,#65839,#65840,#65841,
#65842,#65843,#65844,#65845,#65846,#65847,#65848,#65849,#65850,#65851,#65852,
#65853,#65854,#65855,#65856,#65857,#65858,#65859,#65860,#65861,#65862,#65863,
#65864,#65865,#65866,#65867,#65868,#65869,#65870,#65871,#65872,#65873,#65874,
#65875,#65876,#65877,#65878,#65879,#65880,#65881,#65882,#65883,#65884,#65885,
#65886,#65887,#65888,#65889,#65890,#65891,#65892,#65893,#65894,#65895,#65896,
#65897,#65898,#65899,#65900,#65901,#65902,#65903,#65904,#65905,#65906,#65907,
#65908,#65909,#65910,#65911,#65912,#65913,#65914,#65915,#65916,#65917,#65918,
#65919,#65920,#65921,#65922,#65923,#65924,#65925,#65926,#65927,#65928,#65929,
#65930,#65931,#65932,#65933,#65934,#65935,#65936,#65937,#65938,#65939,#65940,
#65941,#65942,#65943,#65944,#65945,#65946,#65947,#65948,#65949,#65950,#65951,
#65952,#65953,#65954,#65955,#65956,#65957,#65958,#65959,#65960,#65961,#65962,
#65963,#65964,#65965,#65966,#65967,#65968,#65969,#65970,#65971,#65972,#65973,
#65974,#65975,#65976,#65977,#65978,#65979,#65980,#65981,#65982,#65983,#65984,
#65985,#65986,#65987,#65988,#65989,#65990,#65991,#65992,#65993,#65994,#65995,
#65996,#65997,#65998,#65999,#66000,#66001,#66002,#66003,#66004,#66005,#66006,
#66007,#66008,#66009,#66010,#66011,#66012,#66013,#66014,#66015,#66016,#66017,
#66018,#66019,#66020,#66021,#66022,#66023,#66024,#66025,#66026,#66027,#66028,
#66029,#66030,#66031,#66032,#66033,#66034,#66035,#66036,#66037,#66038,#66039,
#66040,#66041,#66042,#66043,#66044,#66045,#66046,#66047,#66048,#66049,#66050,
#66051,#66052,#66053,#66054,#66055,#66056,#66057,#66058,#66059,#66060,#66061,
#66062,#66063,#66064,#66065,#66066,#66067,#66068,#66069,#66070,#66071,#66072,
#66073,#66074,#66075,#66076,#66077,#66078,#66079,#66080,#66081,#66082,#66083,
#66084,#66085,#66086,#66087,#66088,#66089,#66090,#66091,#66092,#66093,#66094,
#66095,#66096,#66097,#66098,#66099,#66100,#66101,#66102,#66103,#66104,#66105,
#66106,#66107,#66108,#66109,#66110,#66111,#66112,#66113,#66114,#66115,#66116,
#66117,#66118,#66119,#66120,#66121,#66122,#66123,#66124,#66125,#66126,#66127,
#66128,#66129,#66130,#66131,#66132,#66133,#66134,#66135,#66136,#66137,#66138,
#66139,#66140,#66141,#66142,#66143,#66144,#66145,#66146,#66147,#66148,#66149,
#66150,#66151,#66152,#66153,#66154,#66155,#66156,#66157,#66158,#66159,#66160,
#66161,#66162,#66163,#66164,#66165,#66166,#66167,#66168,#66169,#66170,#66171,
#66172,#66173,#66174,#66175,#66176,#66177,#66178,#66179,#66180,#66181,#66182,
#66183,#66184,#66185,#66186,#66187,#66188,#66189,#66190,#66191,#66192,#66193,
#66194,#66195,#66196,#66197,#66198,#66199,#66200,#66201,#66202,#66203,#66204,
#66205,#66206,#66207,#66208,#66209,#66210,#66211,#66212,#66213,#66214,#66215,
#66216,#66217,#66218,#66219,#66220,#66221,#66222,#66223,#66224,#66225,#66226,
#66227,#66228,#66229,#66230,#66231,#66232,#66233,#66234,#66235,#66236,#66237,
#66238,#66239,#66240,#66241,#66242,#66243,#66244,#66245,#66246,#66247,#66248,
#66249,#66250,#66251,#66252,#66253,#66254,#66255,#66256,#66257,#66258,#66259,
#66260,#66261,#66262,#66263,#66264,#66265,#66266,#66267,#66268,#66269,#66270,
#66271,#66272,#66273,#66274,#66275,#66276,#66277,#66278,#66279,#66280,#66281,
#66282,#66283,#66284,#66285,#66286,#66287,#66288,#66289,#66290,#66291,#66292,
#66293,#66294,#66295,#66296,#66297,#66298,#66299,#66300,#66301,#66302,#66303,
#66304,#66305,#66306,#66307,#66308,#66309,#66310,#66311,#66312,#66313,#66314,
#66315,#66316,#66317,#66318,#66319,#66320,#66321,#66322,#66323,#66324,#66325,
#66326,#66327,#66328,#66329,#66330,#66331,#66332,#66333,#66334,#66335,#66336,
#66337,#66338,#66339,#66340,#66341,#66342,#66343,#66344,#66345,#66346,#66347,
#66348,#66349,#66350,#66351,#66352,#66353,#66354,#66355,#66356,#66357,#66358,
#66359,#66360,#66361,#66362,#66363,#66364,#66365,#66366,#66367,#66368,#66369,
#66370,#66371,#66372,#66373,#66374,#66375,#66376,#66377,#66378,#66379,#66380,
#66381,#66382,#66383,#66384,#66385,#66386,#66387,#66388,#66389,#66390,#66391,
#66392,#66393,#66394,#66395,#66396,#66397,#66398,#66399,#66400,#66401,#66402,
#66403,#66404,#66405,#66406,#66407,#66408,#66409,#66410,#66411,#66412,#66413,
#66414,#66415,#66416,#66417,#66418,#66419,#66420,#66421,#66422,#66423,#66424,
#66425,#66426,#66427,#66428,#66429,#66430,#66431,#66432,#66433,#66434,#66435,
#66436,#66437,#66438,#66439,#66440,#66441,#66442,#66443,#66444,#66445,#66446,
#66447,#66448,#66449,#66450,#66451,#66452,#66453,#66454,#66455,#66456,#66457,
#66458,#66459,#66460,#66461,#66462,#66463,#66464,#66465,#66466,#66467,#66468,
#66469,#66470,#66471,#66472,#66473,#66474,#66475,#66476,#66477,#66478,#66479,
#66480,#66481,#66482,#66483,#66484,#66485,#66486,#66487,#66488,#66489,#66490,
#66491,#66492,#66493,#66494,#66495,#66496,#66497,#66498,#66499,#66500,#66501,
#66502,#66503,#66504,#66505,#66506,#66507,#66508,#66509,#66510,#66511,#66512,
#66513,#66514,#66515,#66516,#66517,#66518,#66519,#66520,#66521,#66522,#66523,
#66524,#66525,#66526,#66527,#66528,#66529,#66530,#66531,#66532,#66533,#66534,
#66535,#66536,#66537,#66538,#66539,#66540,#66541,#66542,#66543,#66544,#66545,
#66546,#66547,#66548,#66549,#66550,#66551,#66552,#66553,#66554,#66555,#66556,
#66557,#66558,#66559,#66560,#66561,#66562,#66563,#66564,#66565,#66566,#66567,
#66568,#66569,#66570,#66571,#66572,#66573,#66574,#66575,#66576,#66577,#66578,
#66579,#66580,#66581,#66582,#66583,#66584,#66585,#66586,#66587,#66588,#66589,
#66590,#66591,#66592,#66593,#66594,#66595,#66596,#66597,#66598,#66599,#66600,
#66601,#66602,#66603,#66604,#66605,#66606,#66607,#66608,#66609,#66610,#66611,
#66612,#66613,#66614,#66615,#66616,#66617,#66618,#66619,#66620,#66621,#66622,
#66623,#66624,#66625,#66626,#66627,#66628,#66629,#66630,#66631,#66632,#66633,
#66634,#66635,#66636,#66637,#66638,#66639,#66640,#66641,#66642,#66643,#66644,
#66645,#66646,#66647,#66648,#66649,#66650,#66651,#66652,#66653,#66654,#66655,
#66656,#66657,#66658,#66659,#66660,#66661,#66662,#66663,#66664,#66665,#66666,
#66667,#66668,#66669,#66670,#66671,#66672,#66673,#66674,#66675,#66676,#66677,
#66678,#66679,#66680,#66681,#66682,#66683,#66684,#66685,#66686,#66687,#66688,
#66689,#66690,#66691,#66692,#66693,#66694,#66695,#66696,#66697,#66698,#66699,
#66700,#66701,#66702,#66703,#66704,#66705,#66706,#66707,#66708,#66709,#66710,
#66711,#66712,#66713,#66714,#66715,#66716,#66717,#66718,#66719,#66720,#66721,
#66722,#66723,#66724,#66725,#66726,#66727,#66728,#66729,#66730,#66731,#66732,
#66733,#66734,#66735,#66736,#66737,#66738,#66739,#66740,#66741,#66742,#66743,
#66744,#66745,#66746,#66747,#66748,#66749,#66750,#66751,#66752,#66753,#66754,
#66755,#66756,#66757,#66758,#66759,#66760,#66761,#66762,#66763,#66764,#66765,
#66766,#66767,#66768,#66769,#66770,#66771,#66772,#66773,#66774,#66775,#66776,
#66777,#66778,#66779,#66780,#66781,#66782,#66783,#66784,#66785,#66786,#66787,
#66788,#66789,#66790,#66791,#66792,#66793,#66794,#66795,#66796,#66797,#66798,
#66799,#66800,#66801,#66802,#66803,#66804,#66805,#66806,#66807,#66808,#66809,
#66810,#66811,#66812,#66813,#66814,#66815,#66816,#66817,#66818,#66819,#66820,
#66821,#66822,#66823,#66824,#66825,#66826,#66827,#66828,#66829,#66830,#66831,
#66832,#66833,#66834,#66835,#66836,#66837,#66838,#66839,#66840,#66841,#66842,
#66843,#66844,#66845,#66846,#66847,#66848,#66849,#66850,#66851,#66852,#66853,
#66854,#66855,#66856,#66857,#66858,#66859,#66860,#66861,#66862,#66863,#66864,
#66865,#66866,#66867,#66868,#66869,#66870,#66871,#66872,#66873,#66874,#66875,
#66876,#66877,#66878,#66879,#66880,#66881,#66882,#66883,#66884,#66885,#66886,
#66887,#66888,#66889,#66890,#66891,#66892,#66893,#66894,#66895,#66896,#66897,
#66898,#66899,#66900,#66901,#66902,#66903,#66904,#66905,#66906,#66907,#66908,
#66909,#66910,#66911,#66912,#66913,#66914,#66915,#66916,#66917,#66918,#66919,
#66920,#66921,#66922,#66923,#66924,#66925,#66926,#66927,#66928,#66929,#66930,
#66931,#66932,#66933,#66934,#66935,#66936,#66937,#66938,#66939,#66940,#66941,
#66942,#66943,#66944,#66945,#66946,#66947,#66948,#66949,#66950,#66951,#66952,
#66953,#66954,#66955,#66956,#66957,#66958,#66959,#66960,#66961,#66962,#66963,
#66964,#66965,#66966,#66967,#66968,#66969,#66970,#66971,#66972,#66973,#66974,
#66975,#66976,#66977,#66978,#66979,#66980,#66981,#66982,#66983,#66984,#66985,
#66986,#66987,#66988,#66989,#66990,#66991,#66992,#66993,#66994,#66995,#66996,
#66997,#66998,#66999,#67000,#67001,#67002,#67003,#67004,#67005,#67006,#67007,
#67008,#67009,#67010,#67011,#67012,#67013,#67014,#67015,#67016,#67017,#67018,
#67019,#67020,#67021,#67022,#67023,#67024,#67025,#67026,#67027,#67028,#67029,
#67030,#67031,#67032,#67033,#67034,#67035,#67036,#67037,#67038,#67039,#67040,
#67041,#67042,#67043,#67044,#67045,#67046,#67047,#67048,#67049,#67050,#67051,
#67052,#67053,#67054,#67055,#67056,#67057,#67058,#67059,#67060,#67061,#67062,
#67063,#67064,#67065,#67066,#67067,#67068,#67069,#67070,#67071,#67072,#67073,
#67074,#67075,#67076,#67077,#67078,#67079,#67080,#67081,#67082,#67083,#67084,
#67085,#67086,#67087,#67088,#67089,#67090,#67091,#67092,#67093,#67094,#67095,
#67096,#67097,#67098,#67099,#67100,#67101,#67102,#67103,#67104,#67105,#67106,
#67107,#67108,#67109,#67110,#67111,#67112,#67113,#67114,#67115,#67116,#67117,
#67118,#67119,#67120,#67121,#67122,#67123,#67124,#67125,#67126,#67127,#67128,
#67129,#67130,#67131,#67132,#67133,#67134,#67135,#67136,#67137,#67138,#67139,
#67140,#67141,#67142,#67143,#67144,#67145,#67146,#67147,#67148,#67149,#67150,
#67151,#67152,#67153,#67154,#67155,#67156,#67157,#67158,#67159,#67160,#67161,
#67162,#67163,#67164,#67165,#67166,#67167,#67168,#67169,#67170,#67171,#67172,
#67173,#67174,#67175,#67176,#67177,#67178,#67179,#67180,#67181,#67182,#67183,
#67184,#67185,#67186,#67187,#67188,#67189,#67190,#67191,#67192,#67193,#67194,
#67195,#67196,#67197,#67198,#67199,#67200,#67201,#67202,#67203,#67204,#67205,
#67206,#67207,#67208,#67209,#67210,#67211,#67212,#67213,#67214,#67215,#67216,
#67217,#67218,#67219,#67220,#67221,#67222,#67223,#67224,#67225,#67226,#67227,
#67228,#67229,#67230,#67231,#67232,#67233,#67234,#67235,#67236,#67237,#67238,
#67239,#67240,#67241,#67242,#67243,#67244,#67245,#67246,#67247,#67248,#67249,
#67250,#67251,#67252,#67253,#67254,#67255,#67256,#67257,#67258,#67259,#67260,
#67261,#67262,#67263,#67264,#67265,#67266,#67267,#67268,#67269,#67270,#67271,
#67272,#67273,#67274,#67275,#67276,#67277,#67278,#67279,#67280,#67281,#67282,
#67283,#67284,#67285,#67286,#67287,#67288,#67289,#67290,#67291,#67292,#67293,
#67294,#67295,#67296,#67297,#67298,#67299,#67300,#67301,#67302,#67303,#67304,
#67305,#67306,#67307,#67308,#67309,#67310,#67311,#67312,#67313,#67314,#67315,
#67316,#67317,#67318,#67319,#67320,#67321,#67322,#67323,#67324,#67325,#67326,
#67327,#67328,#67329,#67330,#67331,#67332,#67333,#67334,#67335,#67336,#67337,
#67338,#67339,#67340,#67341,#67342,#67343,#67344,#67345,#67346,#67347,#67348,
#67349,#67350,#67351,#67352,#67353,#67354,#67355,#67356,#67357,#67358,#67359,
#67360,#67361,#67362,#67363,#67364,#67365,#67366,#67367,#67368,#67369,#67370,
#67371,#67372,#67373,#67374,#67375,#67376,#67377,#67378,#67379,#67380,#67381,
#67382,#67383,#67384,#67385,#67386,#67387,#67388,#67389,#67390,#67391,#67392,
#67393,#67394,#67395,#67396,#67397,#67398,#67399,#67400,#67401,#67402,#67403,
#67404,#67405,#67406,#67407,#67408,#67409,#67410,#67411,#67412,#67413,#67414,
#67415,#67416,#67417,#67418,#67419,#67420,#67421,#67422,#67423,#67424,#67425,
#67426,#67427,#67428,#67429,#67430,#67431,#67432,#67433,#67434,#67435,#67436,
#67437,#67438,#67439,#67440,#67441,#67442,#67443,#67444,#67445,#67446,#67447,
#67448,#67449,#67450,#67451,#67452,#67453,#67454,#67455,#67456,#67457,#67458,
#67459,#67460,#67461,#67462,#67463,#67464,#67465,#67466,#67467,#67468,#67469,
#67470,#67471,#67472,#67473,#67474,#67475,#67476,#67477,#67478,#67479,#67480,
#67481,#67482,#67483,#67484,#67485,#67486,#67487,#67488,#67489,#67490,#67491,
#67492,#67493,#67494,#67495,#67496,#67497,#67498,#67499,#67500,#67501,#67502,
#67503,#67504,#67505,#67506,#67507,#67508,#67509,#67510,#67511,#67512,#67513,
#67514,#67515,#67516,#67517,#67518,#67519,#67520,#67521,#67522,#67523,#67524,
#67525,#67526,#67527,#67528,#67529,#67530,#67531,#67532,#67533,#67534,#67535,
#67536,#67537,#67538,#67539,#67540,#67541,#67542,#67543,#67544,#67545,#67546,
#67547,#67548,#67549,#67550,#67551,#67552,#67553,#67554,#67555,#67556,#67557,
#67558,#67559,#67560,#67561,#67562,#67563,#67564,#67565,#67566,#67567,#67568,
#67569,#67570,#67571,#67572,#67573,#67574,#67575,#67576,#67577,#67578,#67579,
#67580,#67581,#67582,#67583,#67584,#67585,#67586,#67587,#67588,#67589,#67590,
#67591)) ;
#71866=AXIS2_PLACEMENT_3D('',#113858,#86968,#86969) ;
#71867=AXIS2_PLACEMENT_3D('',#113859,#86970,#86971) ;
#71868=AXIS2_PLACEMENT_3D('',#113861,#86972,#86973) ;
#71869=AXIS2_PLACEMENT_3D('',#113863,#86974,#86975) ;
#71870=AXIS2_PLACEMENT_3D('',#113865,#86976,#86977) ;
#71871=AXIS2_PLACEMENT_3D('',#113866,#86978,#86979) ;
#71872=AXIS2_PLACEMENT_3D('',#113867,#86980,#86981) ;
#71873=AXIS2_PLACEMENT_3D('',#113869,#86982,#86983) ;
#71874=AXIS2_PLACEMENT_3D('',#113871,#86984,#86985) ;
#71875=AXIS2_PLACEMENT_3D('',#113872,#86986,#86987) ;
#71876=AXIS2_PLACEMENT_3D('',#113873,#86988,#86989) ;
#71877=AXIS2_PLACEMENT_3D('',#113876,#86990,#86991) ;
#71878=AXIS2_PLACEMENT_3D('',#113878,#86992,#86993) ;
#71879=AXIS2_PLACEMENT_3D('',#113879,#86994,#86995) ;
#71880=AXIS2_PLACEMENT_3D('',#113880,#86996,#86997) ;
#71881=AXIS2_PLACEMENT_3D('',#113883,#86998,#86999) ;
#71882=AXIS2_PLACEMENT_3D('',#113885,#87000,#87001) ;
#71883=AXIS2_PLACEMENT_3D('',#113889,#87003,#87004) ;
#71884=AXIS2_PLACEMENT_3D('',#113902,#87007,#87008) ;
#71885=AXIS2_PLACEMENT_3D('',#113904,#87009,#87010) ;
#71886=AXIS2_PLACEMENT_3D('',#113906,#87011,#87012) ;
#71887=AXIS2_PLACEMENT_3D('',#113908,#87013,#87014) ;
#71888=AXIS2_PLACEMENT_3D('',#113909,#87015,#87016) ;
#71889=AXIS2_PLACEMENT_3D('',#113910,#87017,#87018) ;
#71890=AXIS2_PLACEMENT_3D('',#113912,#87019,#87020) ;
#71891=AXIS2_PLACEMENT_3D('',#113914,#87021,#87022) ;
#71892=AXIS2_PLACEMENT_3D('',#113915,#87023,#87024) ;
#71893=AXIS2_PLACEMENT_3D('',#113916,#87025,#87026) ;
#71894=AXIS2_PLACEMENT_3D('',#113919,#87027,#87028) ;
#71895=AXIS2_PLACEMENT_3D('',#113921,#87029,#87030) ;
#71896=AXIS2_PLACEMENT_3D('',#113922,#87031,#87032) ;
#71897=AXIS2_PLACEMENT_3D('',#113923,#87033,#87034) ;
#71898=AXIS2_PLACEMENT_3D('',#113926,#87035,#87036) ;
#71899=AXIS2_PLACEMENT_3D('',#113928,#87037,#87038) ;
#71900=AXIS2_PLACEMENT_3D('',#113932,#87040,#87041) ;
#71901=AXIS2_PLACEMENT_3D('',#113945,#87044,#87045) ;
#71902=AXIS2_PLACEMENT_3D('',#113947,#87046,#87047) ;
#71903=AXIS2_PLACEMENT_3D('',#113949,#87048,#87049) ;
#71904=AXIS2_PLACEMENT_3D('',#113951,#87050,#87051) ;
#71905=AXIS2_PLACEMENT_3D('',#113952,#87052,#87053) ;
#71906=AXIS2_PLACEMENT_3D('',#113953,#87054,#87055) ;
#71907=AXIS2_PLACEMENT_3D('',#113955,#87056,#87057) ;
#71908=AXIS2_PLACEMENT_3D('',#113957,#87058,#87059) ;
#71909=AXIS2_PLACEMENT_3D('',#113958,#87060,#87061) ;
#71910=AXIS2_PLACEMENT_3D('',#113959,#87062,#87063) ;
#71911=AXIS2_PLACEMENT_3D('',#113962,#87064,#87065) ;
#71912=AXIS2_PLACEMENT_3D('',#113964,#87066,#87067) ;
#71913=AXIS2_PLACEMENT_3D('',#113965,#87068,#87069) ;
#71914=AXIS2_PLACEMENT_3D('',#113966,#87070,#87071) ;
#71915=AXIS2_PLACEMENT_3D('',#113969,#87072,#87073) ;
#71916=AXIS2_PLACEMENT_3D('',#113971,#87074,#87075) ;
#71917=AXIS2_PLACEMENT_3D('',#113975,#87077,#87078) ;
#71918=AXIS2_PLACEMENT_3D('',#113988,#87081,#87082) ;
#71919=AXIS2_PLACEMENT_3D('',#113990,#87083,#87084) ;
#71920=AXIS2_PLACEMENT_3D('',#113992,#87085,#87086) ;
#71921=AXIS2_PLACEMENT_3D('',#113994,#87087,#87088) ;
#71922=AXIS2_PLACEMENT_3D('',#113995,#87089,#87090) ;
#71923=AXIS2_PLACEMENT_3D('',#113996,#87091,#87092) ;
#71924=AXIS2_PLACEMENT_3D('',#113998,#87093,#87094) ;
#71925=AXIS2_PLACEMENT_3D('',#114000,#87095,#87096) ;
#71926=AXIS2_PLACEMENT_3D('',#114001,#87097,#87098) ;
#71927=AXIS2_PLACEMENT_3D('',#114002,#87099,#87100) ;
#71928=AXIS2_PLACEMENT_3D('',#114005,#87101,#87102) ;
#71929=AXIS2_PLACEMENT_3D('',#114007,#87103,#87104) ;
#71930=AXIS2_PLACEMENT_3D('',#114008,#87105,#87106) ;
#71931=AXIS2_PLACEMENT_3D('',#114009,#87107,#87108) ;
#71932=AXIS2_PLACEMENT_3D('',#114012,#87109,#87110) ;
#71933=AXIS2_PLACEMENT_3D('',#114014,#87111,#87112) ;
#71934=AXIS2_PLACEMENT_3D('',#114018,#87114,#87115) ;
#71935=AXIS2_PLACEMENT_3D('',#114031,#87118,#87119) ;
#71936=AXIS2_PLACEMENT_3D('',#114033,#87120,#87121) ;
#71937=AXIS2_PLACEMENT_3D('',#114035,#87122,#87123) ;
#71938=AXIS2_PLACEMENT_3D('',#114037,#87124,#87125) ;
#71939=AXIS2_PLACEMENT_3D('',#114038,#87126,#87127) ;
#71940=AXIS2_PLACEMENT_3D('',#114039,#87128,#87129) ;
#71941=AXIS2_PLACEMENT_3D('',#114041,#87130,#87131) ;
#71942=AXIS2_PLACEMENT_3D('',#114043,#87132,#87133) ;
#71943=AXIS2_PLACEMENT_3D('',#114044,#87134,#87135) ;
#71944=AXIS2_PLACEMENT_3D('',#114045,#87136,#87137) ;
#71945=AXIS2_PLACEMENT_3D('',#114048,#87138,#87139) ;
#71946=AXIS2_PLACEMENT_3D('',#114050,#87140,#87141) ;
#71947=AXIS2_PLACEMENT_3D('',#114051,#87142,#87143) ;
#71948=AXIS2_PLACEMENT_3D('',#114052,#87144,#87145) ;
#71949=AXIS2_PLACEMENT_3D('',#114055,#87146,#87147) ;
#71950=AXIS2_PLACEMENT_3D('',#114057,#87148,#87149) ;
#71951=AXIS2_PLACEMENT_3D('',#114061,#87151,#87152) ;
#71952=AXIS2_PLACEMENT_3D('',#114074,#87155,#87156) ;
#71953=AXIS2_PLACEMENT_3D('',#114076,#87157,#87158) ;
#71954=AXIS2_PLACEMENT_3D('',#114078,#87159,#87160) ;
#71955=AXIS2_PLACEMENT_3D('',#114080,#87161,#87162) ;
#71956=AXIS2_PLACEMENT_3D('',#114081,#87163,#87164) ;
#71957=AXIS2_PLACEMENT_3D('',#114082,#87165,#87166) ;
#71958=AXIS2_PLACEMENT_3D('',#114084,#87167,#87168) ;
#71959=AXIS2_PLACEMENT_3D('',#114086,#87169,#87170) ;
#71960=AXIS2_PLACEMENT_3D('',#114087,#87171,#87172) ;
#71961=AXIS2_PLACEMENT_3D('',#114088,#87173,#87174) ;
#71962=AXIS2_PLACEMENT_3D('',#114091,#87175,#87176) ;
#71963=AXIS2_PLACEMENT_3D('',#114093,#87177,#87178) ;
#71964=AXIS2_PLACEMENT_3D('',#114094,#87179,#87180) ;
#71965=AXIS2_PLACEMENT_3D('',#114095,#87181,#87182) ;
#71966=AXIS2_PLACEMENT_3D('',#114098,#87183,#87184) ;
#71967=AXIS2_PLACEMENT_3D('',#114100,#87185,#87186) ;
#71968=AXIS2_PLACEMENT_3D('',#114104,#87188,#87189) ;
#71969=AXIS2_PLACEMENT_3D('',#114117,#87192,#87193) ;
#71970=AXIS2_PLACEMENT_3D('',#114119,#87194,#87195) ;
#71971=AXIS2_PLACEMENT_3D('',#114121,#87196,#87197) ;
#71972=AXIS2_PLACEMENT_3D('',#114123,#87198,#87199) ;
#71973=AXIS2_PLACEMENT_3D('',#114124,#87200,#87201) ;
#71974=AXIS2_PLACEMENT_3D('',#114125,#87202,#87203) ;
#71975=AXIS2_PLACEMENT_3D('',#114127,#87204,#87205) ;
#71976=AXIS2_PLACEMENT_3D('',#114129,#87206,#87207) ;
#71977=AXIS2_PLACEMENT_3D('',#114130,#87208,#87209) ;
#71978=AXIS2_PLACEMENT_3D('',#114131,#87210,#87211) ;
#71979=AXIS2_PLACEMENT_3D('',#114134,#87212,#87213) ;
#71980=AXIS2_PLACEMENT_3D('',#114136,#87214,#87215) ;
#71981=AXIS2_PLACEMENT_3D('',#114137,#87216,#87217) ;
#71982=AXIS2_PLACEMENT_3D('',#114138,#87218,#87219) ;
#71983=AXIS2_PLACEMENT_3D('',#114141,#87220,#87221) ;
#71984=AXIS2_PLACEMENT_3D('',#114143,#87222,#87223) ;
#71985=AXIS2_PLACEMENT_3D('',#114147,#87225,#87226) ;
#71986=AXIS2_PLACEMENT_3D('',#114160,#87229,#87230) ;
#71987=AXIS2_PLACEMENT_3D('',#114162,#87231,#87232) ;
#71988=AXIS2_PLACEMENT_3D('',#114164,#87233,#87234) ;
#71989=AXIS2_PLACEMENT_3D('',#114166,#87235,#87236) ;
#71990=AXIS2_PLACEMENT_3D('',#114167,#87237,#87238) ;
#71991=AXIS2_PLACEMENT_3D('',#114168,#87239,#87240) ;
#71992=AXIS2_PLACEMENT_3D('',#114170,#87241,#87242) ;
#71993=AXIS2_PLACEMENT_3D('',#114172,#87243,#87244) ;
#71994=AXIS2_PLACEMENT_3D('',#114173,#87245,#87246) ;
#71995=AXIS2_PLACEMENT_3D('',#114174,#87247,#87248) ;
#71996=AXIS2_PLACEMENT_3D('',#114177,#87249,#87250) ;
#71997=AXIS2_PLACEMENT_3D('',#114179,#87251,#87252) ;
#71998=AXIS2_PLACEMENT_3D('',#114180,#87253,#87254) ;
#71999=AXIS2_PLACEMENT_3D('',#114181,#87255,#87256) ;
#72000=AXIS2_PLACEMENT_3D('',#114184,#87257,#87258) ;
#72001=AXIS2_PLACEMENT_3D('',#114186,#87259,#87260) ;
#72002=AXIS2_PLACEMENT_3D('',#114190,#87262,#87263) ;
#72003=AXIS2_PLACEMENT_3D('',#114203,#87266,#87267) ;
#72004=AXIS2_PLACEMENT_3D('',#114205,#87268,#87269) ;
#72005=AXIS2_PLACEMENT_3D('',#114207,#87270,#87271) ;
#72006=AXIS2_PLACEMENT_3D('',#114209,#87272,#87273) ;
#72007=AXIS2_PLACEMENT_3D('',#114210,#87274,#87275) ;
#72008=AXIS2_PLACEMENT_3D('',#114211,#87276,#87277) ;
#72009=AXIS2_PLACEMENT_3D('',#114214,#87278,#87279) ;
#72010=AXIS2_PLACEMENT_3D('',#114216,#87280,#87281) ;
#72011=AXIS2_PLACEMENT_3D('',#114218,#87282,#87283) ;
#72012=AXIS2_PLACEMENT_3D('',#114219,#87284,#87285) ;
#72013=AXIS2_PLACEMENT_3D('',#114220,#87286,#87287) ;
#72014=AXIS2_PLACEMENT_3D('',#114223,#87288,#87289) ;
#72015=AXIS2_PLACEMENT_3D('',#114225,#87290,#87291) ;
#72016=AXIS2_PLACEMENT_3D('',#114227,#87292,#87293) ;
#72017=AXIS2_PLACEMENT_3D('',#114228,#87294,#87295) ;
#72018=AXIS2_PLACEMENT_3D('',#114229,#87296,#87297) ;
#72019=AXIS2_PLACEMENT_3D('',#114232,#87298,#87299) ;
#72020=AXIS2_PLACEMENT_3D('',#114234,#87300,#87301) ;
#72021=AXIS2_PLACEMENT_3D('',#114236,#87302,#87303) ;
#72022=AXIS2_PLACEMENT_3D('',#114237,#87304,#87305) ;
#72023=AXIS2_PLACEMENT_3D('',#114238,#87306,#87307) ;
#72024=AXIS2_PLACEMENT_3D('',#114241,#87308,#87309) ;
#72025=AXIS2_PLACEMENT_3D('',#114243,#87310,#87311) ;
#72026=AXIS2_PLACEMENT_3D('',#114245,#87312,#87313) ;
#72027=AXIS2_PLACEMENT_3D('',#114246,#87314,#87315) ;
#72028=AXIS2_PLACEMENT_3D('',#114247,#87316,#87317) ;
#72029=AXIS2_PLACEMENT_3D('',#114250,#87318,#87319) ;
#72030=AXIS2_PLACEMENT_3D('',#114252,#87320,#87321) ;
#72031=AXIS2_PLACEMENT_3D('',#114254,#87322,#87323) ;
#72032=AXIS2_PLACEMENT_3D('',#114255,#87324,#87325) ;
#72033=AXIS2_PLACEMENT_3D('',#114256,#87326,#87327) ;
#72034=AXIS2_PLACEMENT_3D('',#114259,#87328,#87329) ;
#72035=AXIS2_PLACEMENT_3D('',#114261,#87330,#87331) ;
#72036=AXIS2_PLACEMENT_3D('',#114263,#87332,#87333) ;
#72037=AXIS2_PLACEMENT_3D('',#114264,#87334,#87335) ;
#72038=AXIS2_PLACEMENT_3D('',#114265,#87336,#87337) ;
#72039=AXIS2_PLACEMENT_3D('',#114268,#87338,#87339) ;
#72040=AXIS2_PLACEMENT_3D('',#114270,#87340,#87341) ;
#72041=AXIS2_PLACEMENT_3D('',#114272,#87342,#87343) ;
#72042=AXIS2_PLACEMENT_3D('',#114273,#87344,#87345) ;
#72043=AXIS2_PLACEMENT_3D('',#114274,#87346,#87347) ;
#72044=AXIS2_PLACEMENT_3D('',#114277,#87348,#87349) ;
#72045=AXIS2_PLACEMENT_3D('',#114279,#87350,#87351) ;
#72046=AXIS2_PLACEMENT_3D('',#114281,#87352,#87353) ;
#72047=AXIS2_PLACEMENT_3D('',#114282,#87354,#87355) ;
#72048=AXIS2_PLACEMENT_3D('',#114283,#87356,#87357) ;
#72049=AXIS2_PLACEMENT_3D('',#114286,#87358,#87359) ;
#72050=AXIS2_PLACEMENT_3D('',#114288,#87360,#87361) ;
#72051=AXIS2_PLACEMENT_3D('',#114290,#87362,#87363) ;
#72052=AXIS2_PLACEMENT_3D('',#114291,#87364,#87365) ;
#72053=AXIS2_PLACEMENT_3D('',#114292,#87366,#87367) ;
#72054=AXIS2_PLACEMENT_3D('',#114294,#87368,#87369) ;
#72055=AXIS2_PLACEMENT_3D('',#114296,#87370,#87371) ;
#72056=AXIS2_PLACEMENT_3D('',#114297,#87372,#87373) ;
#72057=AXIS2_PLACEMENT_3D('',#114298,#87374,#87375) ;
#72058=AXIS2_PLACEMENT_3D('',#114301,#87376,#87377) ;
#72059=AXIS2_PLACEMENT_3D('',#114303,#87378,#87379) ;
#72060=AXIS2_PLACEMENT_3D('',#114304,#87380,#87381) ;
#72061=AXIS2_PLACEMENT_3D('',#114305,#87382,#87383) ;
#72062=AXIS2_PLACEMENT_3D('',#114308,#87384,#87385) ;
#72063=AXIS2_PLACEMENT_3D('',#114310,#87386,#87387) ;
#72064=AXIS2_PLACEMENT_3D('',#114314,#87389,#87390) ;
#72065=AXIS2_PLACEMENT_3D('',#114327,#87393,#87394) ;
#72066=AXIS2_PLACEMENT_3D('',#114329,#87396,#87397) ;
#72067=AXIS2_PLACEMENT_3D('',#114331,#87399,#87400) ;
#72068=AXIS2_PLACEMENT_3D('',#114333,#87402,#87403) ;
#72069=AXIS2_PLACEMENT_3D('',#114335,#87405,#87406) ;
#72070=AXIS2_PLACEMENT_3D('',#114337,#87408,#87409) ;
#72071=AXIS2_PLACEMENT_3D('',#114339,#87411,#87412) ;
#72072=AXIS2_PLACEMENT_3D('',#114341,#87414,#87415) ;
#72073=AXIS2_PLACEMENT_3D('',#114343,#87417,#87418) ;
#72074=AXIS2_PLACEMENT_3D('',#114345,#87420,#87421) ;
#72075=AXIS2_PLACEMENT_3D('',#114348,#87422,#87423) ;
#72076=AXIS2_PLACEMENT_3D('',#114351,#87426,#87427) ;
#72077=AXIS2_PLACEMENT_3D('',#114354,#87428,#87429) ;
#72078=AXIS2_PLACEMENT_3D('',#114357,#87432,#87433) ;
#72079=AXIS2_PLACEMENT_3D('',#114360,#87434,#87435) ;
#72080=AXIS2_PLACEMENT_3D('',#114363,#87438,#87439) ;
#72081=AXIS2_PLACEMENT_3D('',#114366,#87440,#87441) ;
#72082=AXIS2_PLACEMENT_3D('',#114369,#87444,#87445) ;
#72083=AXIS2_PLACEMENT_3D('',#114372,#87446,#87447) ;
#72084=AXIS2_PLACEMENT_3D('',#114375,#87450,#87451) ;
#72085=AXIS2_PLACEMENT_3D('',#114378,#87452,#87453) ;
#72086=AXIS2_PLACEMENT_3D('',#114381,#87456,#87457) ;
#72087=AXIS2_PLACEMENT_3D('',#114384,#87458,#87459) ;
#72088=AXIS2_PLACEMENT_3D('',#114387,#87462,#87463) ;
#72089=AXIS2_PLACEMENT_3D('',#114390,#87464,#87465) ;
#72090=AXIS2_PLACEMENT_3D('',#114393,#87468,#87469) ;
#72091=AXIS2_PLACEMENT_3D('',#114396,#87470,#87471) ;
#72092=AXIS2_PLACEMENT_3D('',#114399,#87474,#87475) ;
#72093=AXIS2_PLACEMENT_3D('',#114401,#87476,#87477) ;
#72094=AXIS2_PLACEMENT_3D('',#114403,#87478,#87479) ;
#72095=AXIS2_PLACEMENT_3D('',#114405,#87480,#87481) ;
#72096=AXIS2_PLACEMENT_3D('',#114406,#87482,#87483) ;
#72097=AXIS2_PLACEMENT_3D('',#114407,#87484,#87485) ;
#72098=AXIS2_PLACEMENT_3D('',#114410,#87486,#87487) ;
#72099=AXIS2_PLACEMENT_3D('',#114412,#87488,#87489) ;
#72100=AXIS2_PLACEMENT_3D('',#114414,#87490,#87491) ;
#72101=AXIS2_PLACEMENT_3D('',#114415,#87492,#87493) ;
#72102=AXIS2_PLACEMENT_3D('',#114416,#87494,#87495) ;
#72103=AXIS2_PLACEMENT_3D('',#114418,#87496,#87497) ;
#72104=AXIS2_PLACEMENT_3D('',#114420,#87498,#87499) ;
#72105=AXIS2_PLACEMENT_3D('',#114421,#87500,#87501) ;
#72106=AXIS2_PLACEMENT_3D('',#114422,#87502,#87503) ;
#72107=AXIS2_PLACEMENT_3D('',#114425,#87504,#87505) ;
#72108=AXIS2_PLACEMENT_3D('',#114427,#87506,#87507) ;
#72109=AXIS2_PLACEMENT_3D('',#114428,#87508,#87509) ;
#72110=AXIS2_PLACEMENT_3D('',#114429,#87510,#87511) ;
#72111=AXIS2_PLACEMENT_3D('',#114432,#87512,#87513) ;
#72112=AXIS2_PLACEMENT_3D('',#114434,#87514,#87515) ;
#72113=AXIS2_PLACEMENT_3D('',#114438,#87517,#87518) ;
#72114=AXIS2_PLACEMENT_3D('',#114451,#87521,#87522) ;
#72115=AXIS2_PLACEMENT_3D('',#114453,#87524,#87525) ;
#72116=AXIS2_PLACEMENT_3D('',#114456,#87526,#87527) ;
#72117=AXIS2_PLACEMENT_3D('',#114459,#87530,#87531) ;
#72118=AXIS2_PLACEMENT_3D('',#114464,#87533,#87534) ;
#72119=AXIS2_PLACEMENT_3D('',#114467,#87536,#87537) ;
#72120=AXIS2_PLACEMENT_3D('',#114469,#87538,#87539) ;
#72121=AXIS2_PLACEMENT_3D('',#114480,#87545,#87546) ;
#72122=AXIS2_PLACEMENT_3D('',#114481,#87547,#87548) ;
#72123=AXIS2_PLACEMENT_3D('',#114486,#87550,#87551) ;
#72124=AXIS2_PLACEMENT_3D('',#114489,#87553,#87554) ;
#72125=AXIS2_PLACEMENT_3D('',#114491,#87555,#87556) ;
#72126=AXIS2_PLACEMENT_3D('',#114502,#87562,#87563) ;
#72127=AXIS2_PLACEMENT_3D('',#114503,#87564,#87565) ;
#72128=AXIS2_PLACEMENT_3D('',#114508,#87567,#87568) ;
#72129=AXIS2_PLACEMENT_3D('',#114511,#87570,#87571) ;
#72130=AXIS2_PLACEMENT_3D('',#114513,#87572,#87573) ;
#72131=AXIS2_PLACEMENT_3D('',#114524,#87579,#87580) ;
#72132=AXIS2_PLACEMENT_3D('',#114525,#87581,#87582) ;
#72133=AXIS2_PLACEMENT_3D('',#114530,#87584,#87585) ;
#72134=AXIS2_PLACEMENT_3D('',#114533,#87587,#87588) ;
#72135=AXIS2_PLACEMENT_3D('',#114535,#87589,#87590) ;
#72136=AXIS2_PLACEMENT_3D('',#114546,#87596,#87597) ;
#72137=AXIS2_PLACEMENT_3D('',#114547,#87598,#87599) ;
#72138=AXIS2_PLACEMENT_3D('',#114552,#87601,#87602) ;
#72139=AXIS2_PLACEMENT_3D('',#114555,#87604,#87605) ;
#72140=AXIS2_PLACEMENT_3D('',#114557,#87606,#87607) ;
#72141=AXIS2_PLACEMENT_3D('',#114568,#87613,#87614) ;
#72142=AXIS2_PLACEMENT_3D('',#114569,#87615,#87616) ;
#72143=AXIS2_PLACEMENT_3D('',#114574,#87618,#87619) ;
#72144=AXIS2_PLACEMENT_3D('',#114577,#87621,#87622) ;
#72145=AXIS2_PLACEMENT_3D('',#114579,#87623,#87624) ;
#72146=AXIS2_PLACEMENT_3D('',#114590,#87630,#87631) ;
#72147=AXIS2_PLACEMENT_3D('',#114591,#87632,#87633) ;
#72148=AXIS2_PLACEMENT_3D('',#114596,#87635,#87636) ;
#72149=AXIS2_PLACEMENT_3D('',#114599,#87638,#87639) ;
#72150=AXIS2_PLACEMENT_3D('',#114601,#87640,#87641) ;
#72151=AXIS2_PLACEMENT_3D('',#114612,#87647,#87648) ;
#72152=AXIS2_PLACEMENT_3D('',#114613,#87649,#87650) ;
#72153=AXIS2_PLACEMENT_3D('',#114618,#87652,#87653) ;
#72154=AXIS2_PLACEMENT_3D('',#114621,#87655,#87656) ;
#72155=AXIS2_PLACEMENT_3D('',#114623,#87657,#87658) ;
#72156=AXIS2_PLACEMENT_3D('',#114634,#87664,#87665) ;
#72157=AXIS2_PLACEMENT_3D('',#114635,#87666,#87667) ;
#72158=AXIS2_PLACEMENT_3D('',#114640,#87669,#87670) ;
#72159=AXIS2_PLACEMENT_3D('',#114643,#87672,#87673) ;
#72160=AXIS2_PLACEMENT_3D('',#114645,#87674,#87675) ;
#72161=AXIS2_PLACEMENT_3D('',#114656,#87681,#87682) ;
#72162=AXIS2_PLACEMENT_3D('',#114657,#87683,#87684) ;
#72163=AXIS2_PLACEMENT_3D('',#114660,#87685,#87686) ;
#72164=AXIS2_PLACEMENT_3D('',#114668,#87691,#87692) ;
#72165=AXIS2_PLACEMENT_3D('',#114671,#87693,#87694) ;
#72166=AXIS2_PLACEMENT_3D('',#114679,#87699,#87700) ;
#72167=AXIS2_PLACEMENT_3D('',#114682,#87701,#87702) ;
#72168=AXIS2_PLACEMENT_3D('',#114690,#87707,#87708) ;
#72169=AXIS2_PLACEMENT_3D('',#114693,#87709,#87710) ;
#72170=AXIS2_PLACEMENT_3D('',#114701,#87715,#87716) ;
#72171=AXIS2_PLACEMENT_3D('',#114704,#87717,#87718) ;
#72172=AXIS2_PLACEMENT_3D('',#114712,#87723,#87724) ;
#72173=AXIS2_PLACEMENT_3D('',#114715,#87725,#87726) ;
#72174=AXIS2_PLACEMENT_3D('',#114723,#87731,#87732) ;
#72175=AXIS2_PLACEMENT_3D('',#114726,#87733,#87734) ;
#72176=AXIS2_PLACEMENT_3D('',#114734,#87739,#87740) ;
#72177=AXIS2_PLACEMENT_3D('',#114737,#87741,#87742) ;
#72178=AXIS2_PLACEMENT_3D('',#114745,#87747,#87748) ;
#72179=AXIS2_PLACEMENT_3D('',#114748,#87749,#87750) ;
#72180=AXIS2_PLACEMENT_3D('',#114756,#87755,#87756) ;
#72181=AXIS2_PLACEMENT_3D('',#114759,#87757,#87758) ;
#72182=AXIS2_PLACEMENT_3D('',#114767,#87763,#87764) ;
#72183=AXIS2_PLACEMENT_3D('',#114770,#87765,#87766) ;
#72184=AXIS2_PLACEMENT_3D('',#114778,#87771,#87772) ;
#72185=AXIS2_PLACEMENT_3D('',#114781,#87773,#87774) ;
#72186=AXIS2_PLACEMENT_3D('',#114789,#87779,#87780) ;
#72187=AXIS2_PLACEMENT_3D('',#114792,#87781,#87782) ;
#72188=AXIS2_PLACEMENT_3D('',#114800,#87787,#87788) ;
#72189=AXIS2_PLACEMENT_3D('',#114803,#87789,#87790) ;
#72190=AXIS2_PLACEMENT_3D('',#114811,#87795,#87796) ;
#72191=AXIS2_PLACEMENT_3D('',#114814,#87797,#87798) ;
#72192=AXIS2_PLACEMENT_3D('',#114822,#87803,#87804) ;
#72193=AXIS2_PLACEMENT_3D('',#114825,#87805,#87806) ;
#72194=AXIS2_PLACEMENT_3D('',#114833,#87811,#87812) ;
#72195=AXIS2_PLACEMENT_3D('',#114836,#87813,#87814) ;
#72196=AXIS2_PLACEMENT_3D('',#114844,#87819,#87820) ;
#72197=AXIS2_PLACEMENT_3D('',#114847,#87821,#87822) ;
#72198=AXIS2_PLACEMENT_3D('',#114855,#87827,#87828) ;
#72199=AXIS2_PLACEMENT_3D('',#114860,#87830,#87831) ;
#72200=AXIS2_PLACEMENT_3D('',#114863,#87833,#87834) ;
#72201=AXIS2_PLACEMENT_3D('',#114864,#87835,#87836) ;
#72202=AXIS2_PLACEMENT_3D('',#114869,#87838,#87839) ;
#72203=AXIS2_PLACEMENT_3D('',#114872,#87841,#87842) ;
#72204=AXIS2_PLACEMENT_3D('',#114873,#87843,#87844) ;
#72205=AXIS2_PLACEMENT_3D('',#114878,#87846,#87847) ;
#72206=AXIS2_PLACEMENT_3D('',#114881,#87849,#87850) ;
#72207=AXIS2_PLACEMENT_3D('',#114882,#87851,#87852) ;
#72208=AXIS2_PLACEMENT_3D('',#114887,#87854,#87855) ;
#72209=AXIS2_PLACEMENT_3D('',#114890,#87857,#87858) ;
#72210=AXIS2_PLACEMENT_3D('',#114891,#87859,#87860) ;
#72211=AXIS2_PLACEMENT_3D('',#114896,#87862,#87863) ;
#72212=AXIS2_PLACEMENT_3D('',#114899,#87865,#87866) ;
#72213=AXIS2_PLACEMENT_3D('',#114900,#87867,#87868) ;
#72214=AXIS2_PLACEMENT_3D('',#114905,#87870,#87871) ;
#72215=AXIS2_PLACEMENT_3D('',#114908,#87873,#87874) ;
#72216=AXIS2_PLACEMENT_3D('',#114909,#87875,#87876) ;
#72217=AXIS2_PLACEMENT_3D('',#114914,#87878,#87879) ;
#72218=AXIS2_PLACEMENT_3D('',#114917,#87881,#87882) ;
#72219=AXIS2_PLACEMENT_3D('',#114918,#87883,#87884) ;
#72220=AXIS2_PLACEMENT_3D('',#114923,#87886,#87887) ;
#72221=AXIS2_PLACEMENT_3D('',#114926,#87889,#87890) ;
#72222=AXIS2_PLACEMENT_3D('',#114927,#87891,#87892) ;
#72223=AXIS2_PLACEMENT_3D('',#114932,#87894,#87895) ;
#72224=AXIS2_PLACEMENT_3D('',#114935,#87897,#87898) ;
#72225=AXIS2_PLACEMENT_3D('',#114936,#87899,#87900) ;
#72226=AXIS2_PLACEMENT_3D('',#114941,#87902,#87903) ;
#72227=AXIS2_PLACEMENT_3D('',#114944,#87905,#87906) ;
#72228=AXIS2_PLACEMENT_3D('',#114946,#87907,#87908) ;
#72229=AXIS2_PLACEMENT_3D('',#114957,#87914,#87915) ;
#72230=AXIS2_PLACEMENT_3D('',#114958,#87916,#87917) ;
#72231=AXIS2_PLACEMENT_3D('',#114961,#87918,#87919) ;
#72232=AXIS2_PLACEMENT_3D('',#114969,#87924,#87925) ;
#72233=AXIS2_PLACEMENT_3D('',#114972,#87926,#87927) ;
#72234=AXIS2_PLACEMENT_3D('',#114980,#87932,#87933) ;
#72235=AXIS2_PLACEMENT_3D('',#114985,#87935,#87936) ;
#72236=AXIS2_PLACEMENT_3D('',#114988,#87938,#87939) ;
#72237=AXIS2_PLACEMENT_3D('',#114989,#87940,#87941) ;
#72238=AXIS2_PLACEMENT_3D('',#114994,#87943,#87944) ;
#72239=AXIS2_PLACEMENT_3D('',#114997,#87946,#87947) ;
#72240=AXIS2_PLACEMENT_3D('',#114998,#87948,#87949) ;
#72241=AXIS2_PLACEMENT_3D('',#115001,#87950,#87951) ;
#72242=AXIS2_PLACEMENT_3D('',#115011,#87957,#87958) ;
#72243=AXIS2_PLACEMENT_3D('',#115015,#87960,#87961) ;
#72244=AXIS2_PLACEMENT_3D('',#115020,#87964,#87965) ;
#72245=AXIS2_PLACEMENT_3D('',#115024,#87967,#87968) ;
#72246=AXIS2_PLACEMENT_3D('',#115029,#87971,#87972) ;
#72247=AXIS2_PLACEMENT_3D('',#115033,#87974,#87975) ;
#72248=AXIS2_PLACEMENT_3D('',#115038,#87978,#87979) ;
#72249=AXIS2_PLACEMENT_3D('',#115042,#87981,#87982) ;
#72250=AXIS2_PLACEMENT_3D('',#115047,#87985,#87986) ;
#72251=AXIS2_PLACEMENT_3D('',#115051,#87988,#87989) ;
#72252=AXIS2_PLACEMENT_3D('',#115056,#87992,#87993) ;
#72253=AXIS2_PLACEMENT_3D('',#115060,#87995,#87996) ;
#72254=AXIS2_PLACEMENT_3D('',#115065,#87999,#88000) ;
#72255=AXIS2_PLACEMENT_3D('',#115069,#88002,#88003) ;
#72256=AXIS2_PLACEMENT_3D('',#115074,#88006,#88007) ;
#72257=AXIS2_PLACEMENT_3D('',#115078,#88009,#88010) ;
#72258=AXIS2_PLACEMENT_3D('',#115083,#88013,#88014) ;
#72259=AXIS2_PLACEMENT_3D('',#115087,#88016,#88017) ;
#72260=AXIS2_PLACEMENT_3D('',#115092,#88020,#88021) ;
#72261=AXIS2_PLACEMENT_3D('',#115094,#88023,#88024) ;
#72262=AXIS2_PLACEMENT_3D('',#115096,#88025,#88026) ;
#72263=AXIS2_PLACEMENT_3D('',#115099,#88028,#88029) ;
#72264=AXIS2_PLACEMENT_3D('',#115100,#88030,#88031) ;
#72265=AXIS2_PLACEMENT_3D('',#115103,#88032,#88033) ;
#72266=AXIS2_PLACEMENT_3D('',#115108,#88036,#88037) ;
#72267=AXIS2_PLACEMENT_3D('',#115112,#88039,#88040) ;
#72268=AXIS2_PLACEMENT_3D('',#115117,#88043,#88044) ;
#72269=AXIS2_PLACEMENT_3D('',#115121,#88046,#88047) ;
#72270=AXIS2_PLACEMENT_3D('',#115126,#88050,#88051) ;
#72271=AXIS2_PLACEMENT_3D('',#115130,#88053,#88054) ;
#72272=AXIS2_PLACEMENT_3D('',#115135,#88057,#88058) ;
#72273=AXIS2_PLACEMENT_3D('',#115139,#88060,#88061) ;
#72274=AXIS2_PLACEMENT_3D('',#115144,#88064,#88065) ;
#72275=AXIS2_PLACEMENT_3D('',#115148,#88067,#88068) ;
#72276=AXIS2_PLACEMENT_3D('',#115153,#88071,#88072) ;
#72277=AXIS2_PLACEMENT_3D('',#115157,#88074,#88075) ;
#72278=AXIS2_PLACEMENT_3D('',#115162,#88078,#88079) ;
#72279=AXIS2_PLACEMENT_3D('',#115166,#88081,#88082) ;
#72280=AXIS2_PLACEMENT_3D('',#115171,#88085,#88086) ;
#72281=AXIS2_PLACEMENT_3D('',#115175,#88088,#88089) ;
#72282=AXIS2_PLACEMENT_3D('',#115180,#88092,#88093) ;
#72283=AXIS2_PLACEMENT_3D('',#115184,#88095,#88096) ;
#72284=AXIS2_PLACEMENT_3D('',#115194,#88102,#88103) ;
#72285=AXIS2_PLACEMENT_3D('',#115196,#88105,#88106) ;
#72286=AXIS2_PLACEMENT_3D('',#115200,#88108,#88109) ;
#72287=AXIS2_PLACEMENT_3D('',#115201,#88110,#88111) ;
#72288=AXIS2_PLACEMENT_3D('',#115202,#88112,#88113) ;
#72289=AXIS2_PLACEMENT_3D('',#115208,#88117,#88118) ;
#72290=AXIS2_PLACEMENT_3D('',#115212,#88120,#88121) ;
#72291=AXIS2_PLACEMENT_3D('',#115213,#88122,#88123) ;
#72292=AXIS2_PLACEMENT_3D('',#115214,#88124,#88125) ;
#72293=AXIS2_PLACEMENT_3D('',#115220,#88129,#88130) ;
#72294=AXIS2_PLACEMENT_3D('',#115224,#88132,#88133) ;
#72295=AXIS2_PLACEMENT_3D('',#115225,#88134,#88135) ;
#72296=AXIS2_PLACEMENT_3D('',#115226,#88136,#88137) ;
#72297=AXIS2_PLACEMENT_3D('',#115232,#88141,#88142) ;
#72298=AXIS2_PLACEMENT_3D('',#115236,#88144,#88145) ;
#72299=AXIS2_PLACEMENT_3D('',#115237,#88146,#88147) ;
#72300=AXIS2_PLACEMENT_3D('',#115238,#88148,#88149) ;
#72301=AXIS2_PLACEMENT_3D('',#115244,#88153,#88154) ;
#72302=AXIS2_PLACEMENT_3D('',#115248,#88156,#88157) ;
#72303=AXIS2_PLACEMENT_3D('',#115249,#88158,#88159) ;
#72304=AXIS2_PLACEMENT_3D('',#115250,#88160,#88161) ;
#72305=AXIS2_PLACEMENT_3D('',#115256,#88165,#88166) ;
#72306=AXIS2_PLACEMENT_3D('',#115260,#88168,#88169) ;
#72307=AXIS2_PLACEMENT_3D('',#115261,#88170,#88171) ;
#72308=AXIS2_PLACEMENT_3D('',#115262,#88172,#88173) ;
#72309=AXIS2_PLACEMENT_3D('',#115267,#88176,#88177) ;
#72310=AXIS2_PLACEMENT_3D('',#115275,#88181,#88182) ;
#72311=AXIS2_PLACEMENT_3D('',#115279,#88184,#88185) ;
#72312=AXIS2_PLACEMENT_3D('',#115284,#88188,#88189) ;
#72313=AXIS2_PLACEMENT_3D('',#115292,#88193,#88194) ;
#72314=AXIS2_PLACEMENT_3D('',#115296,#88196,#88197) ;
#72315=AXIS2_PLACEMENT_3D('',#115300,#88199,#88200) ;
#72316=AXIS2_PLACEMENT_3D('',#115302,#88201,#88202) ;
#72317=AXIS2_PLACEMENT_3D('',#115304,#88203,#88204) ;
#72318=AXIS2_PLACEMENT_3D('',#115308,#88206,#88207) ;
#72319=AXIS2_PLACEMENT_3D('',#115312,#88209,#88210) ;
#72320=AXIS2_PLACEMENT_3D('',#115320,#88214,#88215) ;
#72321=AXIS2_PLACEMENT_3D('',#115324,#88217,#88218) ;
#72322=AXIS2_PLACEMENT_3D('',#115329,#88221,#88222) ;
#72323=AXIS2_PLACEMENT_3D('',#115337,#88226,#88227) ;
#72324=AXIS2_PLACEMENT_3D('',#115341,#88229,#88230) ;
#72325=AXIS2_PLACEMENT_3D('',#115345,#88232,#88233) ;
#72326=AXIS2_PLACEMENT_3D('',#115347,#88234,#88235) ;
#72327=AXIS2_PLACEMENT_3D('',#115349,#88236,#88237) ;
#72328=AXIS2_PLACEMENT_3D('',#115353,#88239,#88240) ;
#72329=AXIS2_PLACEMENT_3D('',#115357,#88242,#88243) ;
#72330=AXIS2_PLACEMENT_3D('',#115365,#88247,#88248) ;
#72331=AXIS2_PLACEMENT_3D('',#115369,#88250,#88251) ;
#72332=AXIS2_PLACEMENT_3D('',#115374,#88254,#88255) ;
#72333=AXIS2_PLACEMENT_3D('',#115382,#88259,#88260) ;
#72334=AXIS2_PLACEMENT_3D('',#115386,#88262,#88263) ;
#72335=AXIS2_PLACEMENT_3D('',#115390,#88265,#88266) ;
#72336=AXIS2_PLACEMENT_3D('',#115392,#88267,#88268) ;
#72337=AXIS2_PLACEMENT_3D('',#115394,#88269,#88270) ;
#72338=AXIS2_PLACEMENT_3D('',#115398,#88272,#88273) ;
#72339=AXIS2_PLACEMENT_3D('',#115402,#88275,#88276) ;
#72340=AXIS2_PLACEMENT_3D('',#115410,#88280,#88281) ;
#72341=AXIS2_PLACEMENT_3D('',#115414,#88283,#88284) ;
#72342=AXIS2_PLACEMENT_3D('',#115419,#88287,#88288) ;
#72343=AXIS2_PLACEMENT_3D('',#115427,#88292,#88293) ;
#72344=AXIS2_PLACEMENT_3D('',#115431,#88295,#88296) ;
#72345=AXIS2_PLACEMENT_3D('',#115435,#88298,#88299) ;
#72346=AXIS2_PLACEMENT_3D('',#115437,#88300,#88301) ;
#72347=AXIS2_PLACEMENT_3D('',#115439,#88302,#88303) ;
#72348=AXIS2_PLACEMENT_3D('',#115443,#88305,#88306) ;
#72349=AXIS2_PLACEMENT_3D('',#115447,#88308,#88309) ;
#72350=AXIS2_PLACEMENT_3D('',#115455,#88313,#88314) ;
#72351=AXIS2_PLACEMENT_3D('',#115459,#88316,#88317) ;
#72352=AXIS2_PLACEMENT_3D('',#115464,#88320,#88321) ;
#72353=AXIS2_PLACEMENT_3D('',#115472,#88325,#88326) ;
#72354=AXIS2_PLACEMENT_3D('',#115476,#88328,#88329) ;
#72355=AXIS2_PLACEMENT_3D('',#115480,#88331,#88332) ;
#72356=AXIS2_PLACEMENT_3D('',#115482,#88333,#88334) ;
#72357=AXIS2_PLACEMENT_3D('',#115484,#88335,#88336) ;
#72358=AXIS2_PLACEMENT_3D('',#115488,#88338,#88339) ;
#72359=AXIS2_PLACEMENT_3D('',#115492,#88341,#88342) ;
#72360=AXIS2_PLACEMENT_3D('',#115500,#88346,#88347) ;
#72361=AXIS2_PLACEMENT_3D('',#115504,#88349,#88350) ;
#72362=AXIS2_PLACEMENT_3D('',#115509,#88353,#88354) ;
#72363=AXIS2_PLACEMENT_3D('',#115517,#88358,#88359) ;
#72364=AXIS2_PLACEMENT_3D('',#115521,#88361,#88362) ;
#72365=AXIS2_PLACEMENT_3D('',#115525,#88364,#88365) ;
#72366=AXIS2_PLACEMENT_3D('',#115527,#88366,#88367) ;
#72367=AXIS2_PLACEMENT_3D('',#115529,#88368,#88369) ;
#72368=AXIS2_PLACEMENT_3D('',#115533,#88371,#88372) ;
#72369=AXIS2_PLACEMENT_3D('',#115537,#88374,#88375) ;
#72370=AXIS2_PLACEMENT_3D('',#115545,#88379,#88380) ;
#72371=AXIS2_PLACEMENT_3D('',#115549,#88382,#88383) ;
#72372=AXIS2_PLACEMENT_3D('',#115554,#88386,#88387) ;
#72373=AXIS2_PLACEMENT_3D('',#115562,#88391,#88392) ;
#72374=AXIS2_PLACEMENT_3D('',#115566,#88394,#88395) ;
#72375=AXIS2_PLACEMENT_3D('',#115570,#88397,#88398) ;
#72376=AXIS2_PLACEMENT_3D('',#115572,#88399,#88400) ;
#72377=AXIS2_PLACEMENT_3D('',#115574,#88401,#88402) ;
#72378=AXIS2_PLACEMENT_3D('',#115578,#88404,#88405) ;
#72379=AXIS2_PLACEMENT_3D('',#115582,#88407,#88408) ;
#72380=AXIS2_PLACEMENT_3D('',#115590,#88412,#88413) ;
#72381=AXIS2_PLACEMENT_3D('',#115594,#88415,#88416) ;
#72382=AXIS2_PLACEMENT_3D('',#115599,#88419,#88420) ;
#72383=AXIS2_PLACEMENT_3D('',#115607,#88424,#88425) ;
#72384=AXIS2_PLACEMENT_3D('',#115611,#88427,#88428) ;
#72385=AXIS2_PLACEMENT_3D('',#115615,#88430,#88431) ;
#72386=AXIS2_PLACEMENT_3D('',#115617,#88432,#88433) ;
#72387=AXIS2_PLACEMENT_3D('',#115619,#88434,#88435) ;
#72388=AXIS2_PLACEMENT_3D('',#115623,#88437,#88438) ;
#72389=AXIS2_PLACEMENT_3D('',#115627,#88440,#88441) ;
#72390=AXIS2_PLACEMENT_3D('',#115635,#88445,#88446) ;
#72391=AXIS2_PLACEMENT_3D('',#115639,#88448,#88449) ;
#72392=AXIS2_PLACEMENT_3D('',#115644,#88452,#88453) ;
#72393=AXIS2_PLACEMENT_3D('',#115652,#88457,#88458) ;
#72394=AXIS2_PLACEMENT_3D('',#115656,#88460,#88461) ;
#72395=AXIS2_PLACEMENT_3D('',#115660,#88463,#88464) ;
#72396=AXIS2_PLACEMENT_3D('',#115662,#88465,#88466) ;
#72397=AXIS2_PLACEMENT_3D('',#115664,#88467,#88468) ;
#72398=AXIS2_PLACEMENT_3D('',#115668,#88470,#88471) ;
#72399=AXIS2_PLACEMENT_3D('',#115672,#88473,#88474) ;
#72400=AXIS2_PLACEMENT_3D('',#115680,#88478,#88479) ;
#72401=AXIS2_PLACEMENT_3D('',#115684,#88481,#88482) ;
#72402=AXIS2_PLACEMENT_3D('',#115689,#88485,#88486) ;
#72403=AXIS2_PLACEMENT_3D('',#115697,#88490,#88491) ;
#72404=AXIS2_PLACEMENT_3D('',#115701,#88493,#88494) ;
#72405=AXIS2_PLACEMENT_3D('',#115705,#88496,#88497) ;
#72406=AXIS2_PLACEMENT_3D('',#115707,#88498,#88499) ;
#72407=AXIS2_PLACEMENT_3D('',#115709,#88500,#88501) ;
#72408=AXIS2_PLACEMENT_3D('',#115713,#88503,#88504) ;
#72409=AXIS2_PLACEMENT_3D('',#115715,#88506,#88507) ;
#72410=AXIS2_PLACEMENT_3D('',#115726,#88512,#88513) ;
#72411=AXIS2_PLACEMENT_3D('',#115734,#88517,#88518) ;
#72412=AXIS2_PLACEMENT_3D('',#115736,#88520,#88521) ;
#72413=AXIS2_PLACEMENT_3D('',#115747,#88526,#88527) ;
#72414=AXIS2_PLACEMENT_3D('',#115755,#88531,#88532) ;
#72415=AXIS2_PLACEMENT_3D('',#115757,#88534,#88535) ;
#72416=AXIS2_PLACEMENT_3D('',#115772,#88542,#88543) ;
#72417=AXIS2_PLACEMENT_3D('',#115776,#88545,#88546) ;
#72418=AXIS2_PLACEMENT_3D('',#115778,#88548,#88549) ;
#72419=AXIS2_PLACEMENT_3D('',#115787,#88554,#88555) ;
#72420=AXIS2_PLACEMENT_3D('',#115793,#88559,#88560) ;
#72421=AXIS2_PLACEMENT_3D('',#115802,#88565,#88566) ;
#72422=AXIS2_PLACEMENT_3D('',#115811,#88571,#88572) ;
#72423=AXIS2_PLACEMENT_3D('',#115820,#88577,#88578) ;
#72424=AXIS2_PLACEMENT_3D('',#115825,#88580,#88581) ;
#72425=AXIS2_PLACEMENT_3D('',#115828,#88583,#88584) ;
#72426=AXIS2_PLACEMENT_3D('',#115829,#88585,#88586) ;
#72427=AXIS2_PLACEMENT_3D('',#115835,#88590,#88591) ;
#72428=AXIS2_PLACEMENT_3D('',#115837,#88592,#88593) ;
#72429=AXIS2_PLACEMENT_3D('',#115840,#88595,#88596) ;
#72430=AXIS2_PLACEMENT_3D('',#115841,#88597,#88598) ;
#72431=AXIS2_PLACEMENT_3D('',#115847,#88602,#88603) ;
#72432=AXIS2_PLACEMENT_3D('',#115849,#88604,#88605) ;
#72433=AXIS2_PLACEMENT_3D('',#115852,#88607,#88608) ;
#72434=AXIS2_PLACEMENT_3D('',#115853,#88609,#88610) ;
#72435=AXIS2_PLACEMENT_3D('',#115858,#88614,#88615) ;
#72436=AXIS2_PLACEMENT_3D('',#115861,#88617,#88618) ;
#72437=AXIS2_PLACEMENT_3D('',#115862,#88619,#88620) ;
#72438=AXIS2_PLACEMENT_3D('',#115865,#88623,#88624) ;
#72439=AXIS2_PLACEMENT_3D('',#115871,#88628,#88629) ;
#72440=AXIS2_PLACEMENT_3D('',#115873,#88630,#88631) ;
#72441=AXIS2_PLACEMENT_3D('',#115876,#88633,#88634) ;
#72442=AXIS2_PLACEMENT_3D('',#115877,#88635,#88636) ;
#72443=AXIS2_PLACEMENT_3D('',#115883,#88640,#88641) ;
#72444=AXIS2_PLACEMENT_3D('',#115885,#88642,#88643) ;
#72445=AXIS2_PLACEMENT_3D('',#115888,#88645,#88646) ;
#72446=AXIS2_PLACEMENT_3D('',#115889,#88647,#88648) ;
#72447=AXIS2_PLACEMENT_3D('',#115895,#88652,#88653) ;
#72448=AXIS2_PLACEMENT_3D('',#115897,#88654,#88655) ;
#72449=AXIS2_PLACEMENT_3D('',#115900,#88657,#88658) ;
#72450=AXIS2_PLACEMENT_3D('',#115901,#88659,#88660) ;
#72451=AXIS2_PLACEMENT_3D('',#115907,#88664,#88665) ;
#72452=AXIS2_PLACEMENT_3D('',#115909,#88666,#88667) ;
#72453=AXIS2_PLACEMENT_3D('',#115912,#88669,#88670) ;
#72454=AXIS2_PLACEMENT_3D('',#115913,#88671,#88672) ;
#72455=AXIS2_PLACEMENT_3D('',#115919,#88676,#88677) ;
#72456=AXIS2_PLACEMENT_3D('',#115921,#88678,#88679) ;
#72457=AXIS2_PLACEMENT_3D('',#115924,#88681,#88682) ;
#72458=AXIS2_PLACEMENT_3D('',#115925,#88683,#88684) ;
#72459=AXIS2_PLACEMENT_3D('',#115931,#88688,#88689) ;
#72460=AXIS2_PLACEMENT_3D('',#115933,#88690,#88691) ;
#72461=AXIS2_PLACEMENT_3D('',#115936,#88693,#88694) ;
#72462=AXIS2_PLACEMENT_3D('',#115937,#88695,#88696) ;
#72463=AXIS2_PLACEMENT_3D('',#115939,#88697,#88698) ;
#72464=AXIS2_PLACEMENT_3D('',#115942,#88700,#88701) ;
#72465=AXIS2_PLACEMENT_3D('',#115943,#88702,#88703) ;
#72466=AXIS2_PLACEMENT_3D('',#115945,#88704,#88705) ;
#72467=AXIS2_PLACEMENT_3D('',#115948,#88707,#88708) ;
#72468=AXIS2_PLACEMENT_3D('',#115949,#88709,#88710) ;
#72469=AXIS2_PLACEMENT_3D('',#115955,#88714,#88715) ;
#72470=AXIS2_PLACEMENT_3D('',#115957,#88716,#88717) ;
#72471=AXIS2_PLACEMENT_3D('',#115960,#88719,#88720) ;
#72472=AXIS2_PLACEMENT_3D('',#115961,#88721,#88722) ;
#72473=AXIS2_PLACEMENT_3D('',#115967,#88726,#88727) ;
#72474=AXIS2_PLACEMENT_3D('',#115969,#88728,#88729) ;
#72475=AXIS2_PLACEMENT_3D('',#115972,#88731,#88732) ;
#72476=AXIS2_PLACEMENT_3D('',#115973,#88733,#88734) ;
#72477=AXIS2_PLACEMENT_3D('',#115976,#88737,#88738) ;
#72478=AXIS2_PLACEMENT_3D('',#115979,#88739,#88740) ;
#72479=AXIS2_PLACEMENT_3D('',#115983,#88742,#88743) ;
#72480=AXIS2_PLACEMENT_3D('',#115991,#88747,#88748) ;
#72481=AXIS2_PLACEMENT_3D('',#115999,#88752,#88753) ;
#72482=AXIS2_PLACEMENT_3D('',#116003,#88755,#88756) ;
#72483=AXIS2_PLACEMENT_3D('',#116012,#88762,#88763) ;
#72484=AXIS2_PLACEMENT_3D('',#116017,#88765,#88766) ;
#72485=AXIS2_PLACEMENT_3D('',#116021,#88768,#88769) ;
#72486=AXIS2_PLACEMENT_3D('',#116025,#88771,#88772) ;
#72487=AXIS2_PLACEMENT_3D('',#116028,#88774,#88775) ;
#72488=AXIS2_PLACEMENT_3D('',#116029,#88776,#88777) ;
#72489=AXIS2_PLACEMENT_3D('',#116030,#88778,#88779) ;
#72490=AXIS2_PLACEMENT_3D('',#116031,#88780,#88781) ;
#72491=AXIS2_PLACEMENT_3D('',#116032,#88782,#88783) ;
#72492=AXIS2_PLACEMENT_3D('',#116033,#88784,#88785) ;
#72493=AXIS2_PLACEMENT_3D('',#116034,#88786,#88787) ;
#72494=AXIS2_PLACEMENT_3D('',#116035,#88788,#88789) ;
#72495=AXIS2_PLACEMENT_3D('',#116037,#88790,#88791) ;
#72496=AXIS2_PLACEMENT_3D('',#116038,#88792,#88793) ;
#72497=AXIS2_PLACEMENT_3D('',#116039,#88794,#88795) ;
#72498=AXIS2_PLACEMENT_3D('',#116040,#88796,#88797) ;
#72499=AXIS2_PLACEMENT_3D('',#116041,#88798,#88799) ;
#72500=AXIS2_PLACEMENT_3D('',#116042,#88800,#88801) ;
#72501=AXIS2_PLACEMENT_3D('',#116043,#88802,#88803) ;
#72502=AXIS2_PLACEMENT_3D('',#116044,#88804,#88805) ;
#72503=AXIS2_PLACEMENT_3D('',#116045,#88806,#88807) ;
#72504=AXIS2_PLACEMENT_3D('',#116056,#88809,#88810) ;
#72505=AXIS2_PLACEMENT_3D('',#116113,#88812,#88813) ;
#72506=AXIS2_PLACEMENT_3D('',#116114,#88814,#88815) ;
#72507=AXIS2_PLACEMENT_3D('',#116115,#88816,#88817) ;
#72508=AXIS2_PLACEMENT_3D('',#116116,#88818,#88819) ;
#72509=AXIS2_PLACEMENT_3D('',#116117,#88820,#88821) ;
#72510=AXIS2_PLACEMENT_3D('',#116118,#88822,#88823) ;
#72511=AXIS2_PLACEMENT_3D('',#116119,#88824,#88825) ;
#72512=AXIS2_PLACEMENT_3D('',#116120,#88826,#88827) ;
#72513=AXIS2_PLACEMENT_3D('',#116121,#88828,#88829) ;
#72514=AXIS2_PLACEMENT_3D('',#116122,#88830,#88831) ;
#72515=AXIS2_PLACEMENT_3D('',#116123,#88832,#88833) ;
#72516=AXIS2_PLACEMENT_3D('',#116124,#88834,#88835) ;
#72517=AXIS2_PLACEMENT_3D('',#116125,#88836,#88837) ;
#72518=AXIS2_PLACEMENT_3D('',#116126,#88838,#88839) ;
#72519=AXIS2_PLACEMENT_3D('',#116127,#88840,#88841) ;
#72520=AXIS2_PLACEMENT_3D('',#116128,#88842,#88843) ;
#72521=AXIS2_PLACEMENT_3D('',#116129,#88844,#88845) ;
#72522=AXIS2_PLACEMENT_3D('',#116130,#88846,#88847) ;
#72523=AXIS2_PLACEMENT_3D('',#116131,#88848,#88849) ;
#72524=AXIS2_PLACEMENT_3D('',#116132,#88850,#88851) ;
#72525=AXIS2_PLACEMENT_3D('',#116133,#88852,#88853) ;
#72526=AXIS2_PLACEMENT_3D('',#116134,#88854,#88855) ;
#72527=AXIS2_PLACEMENT_3D('',#116135,#88856,#88857) ;
#72528=AXIS2_PLACEMENT_3D('',#116138,#88859,#88860) ;
#72529=AXIS2_PLACEMENT_3D('',#116139,#88861,#88862) ;
#72530=AXIS2_PLACEMENT_3D('',#116140,#88863,#88864) ;
#72531=AXIS2_PLACEMENT_3D('',#116141,#88865,#88866) ;
#72532=AXIS2_PLACEMENT_3D('',#116142,#88867,#88868) ;
#72533=AXIS2_PLACEMENT_3D('',#116143,#88869,#88870) ;
#72534=AXIS2_PLACEMENT_3D('',#116144,#88871,#88872) ;
#72535=AXIS2_PLACEMENT_3D('',#116145,#88873,#88874) ;
#72536=AXIS2_PLACEMENT_3D('',#116146,#88875,#88876) ;
#72537=AXIS2_PLACEMENT_3D('',#116147,#88877,#88878) ;
#72538=AXIS2_PLACEMENT_3D('',#116148,#88879,#88880) ;
#72539=AXIS2_PLACEMENT_3D('',#116149,#88881,#88882) ;
#72540=AXIS2_PLACEMENT_3D('',#116150,#88883,#88884) ;
#72541=AXIS2_PLACEMENT_3D('',#116151,#88885,#88886) ;
#72542=AXIS2_PLACEMENT_3D('',#116152,#88887,#88888) ;
#72543=AXIS2_PLACEMENT_3D('',#116153,#88889,#88890) ;
#72544=AXIS2_PLACEMENT_3D('',#116155,#88891,#88892) ;
#72545=AXIS2_PLACEMENT_3D('',#116156,#88893,#88894) ;
#72546=AXIS2_PLACEMENT_3D('',#116157,#88895,#88896) ;
#72547=AXIS2_PLACEMENT_3D('',#116158,#88897,#88898) ;
#72548=AXIS2_PLACEMENT_3D('',#116159,#88899,#88900) ;
#72549=AXIS2_PLACEMENT_3D('',#116160,#88901,#88902) ;
#72550=AXIS2_PLACEMENT_3D('',#116161,#88903,#88904) ;
#72551=AXIS2_PLACEMENT_3D('',#116162,#88905,#88906) ;
#72552=AXIS2_PLACEMENT_3D('',#116163,#88907,#88908) ;
#72553=AXIS2_PLACEMENT_3D('',#116164,#88909,#88910) ;
#72554=AXIS2_PLACEMENT_3D('',#116165,#88911,#88912) ;
#72555=AXIS2_PLACEMENT_3D('',#116166,#88913,#88914) ;
#72556=AXIS2_PLACEMENT_3D('',#116167,#88915,#88916) ;
#72557=AXIS2_PLACEMENT_3D('',#116170,#88918,#88919) ;
#72558=AXIS2_PLACEMENT_3D('',#116171,#88920,#88921) ;
#72559=AXIS2_PLACEMENT_3D('',#116172,#88922,#88923) ;
#72560=AXIS2_PLACEMENT_3D('',#116173,#88924,#88925) ;
#72561=AXIS2_PLACEMENT_3D('',#116174,#88926,#88927) ;
#72562=AXIS2_PLACEMENT_3D('',#116175,#88928,#88929) ;
#72563=AXIS2_PLACEMENT_3D('',#116176,#88930,#88931) ;
#72564=AXIS2_PLACEMENT_3D('',#116177,#88932,#88933) ;
#72565=AXIS2_PLACEMENT_3D('',#116178,#88934,#88935) ;
#72566=AXIS2_PLACEMENT_3D('',#116179,#88936,#88937) ;
#72567=AXIS2_PLACEMENT_3D('',#116180,#88938,#88939) ;
#72568=AXIS2_PLACEMENT_3D('',#116181,#88940,#88941) ;
#72569=AXIS2_PLACEMENT_3D('',#116182,#88942,#88943) ;
#72570=AXIS2_PLACEMENT_3D('',#116184,#88944,#88945) ;
#72571=AXIS2_PLACEMENT_3D('',#116185,#88946,#88947) ;
#72572=AXIS2_PLACEMENT_3D('',#116186,#88948,#88949) ;
#72573=AXIS2_PLACEMENT_3D('',#116187,#88950,#88951) ;
#72574=AXIS2_PLACEMENT_3D('',#116188,#88952,#88953) ;
#72575=AXIS2_PLACEMENT_3D('',#116189,#88954,#88955) ;
#72576=AXIS2_PLACEMENT_3D('',#116190,#88956,#88957) ;
#72577=AXIS2_PLACEMENT_3D('',#116191,#88958,#88959) ;
#72578=AXIS2_PLACEMENT_3D('',#116192,#88960,#88961) ;
#72579=AXIS2_PLACEMENT_3D('',#116193,#88962,#88963) ;
#72580=AXIS2_PLACEMENT_3D('',#116194,#88964,#88965) ;
#72581=AXIS2_PLACEMENT_3D('',#116196,#88967,#88968) ;
#72582=AXIS2_PLACEMENT_3D('',#116197,#88969,#88970) ;
#72583=AXIS2_PLACEMENT_3D('',#116198,#88971,#88972) ;
#72584=AXIS2_PLACEMENT_3D('',#116199,#88973,#88974) ;
#72585=AXIS2_PLACEMENT_3D('',#116200,#88975,#88976) ;
#72586=AXIS2_PLACEMENT_3D('',#116201,#88977,#88978) ;
#72587=AXIS2_PLACEMENT_3D('',#116202,#88979,#88980) ;
#72588=AXIS2_PLACEMENT_3D('',#116203,#88981,#88982) ;
#72589=AXIS2_PLACEMENT_3D('',#116204,#88983,#88984) ;
#72590=AXIS2_PLACEMENT_3D('',#116205,#88985,#88986) ;
#72591=AXIS2_PLACEMENT_3D('',#116206,#88987,#88988) ;
#72592=AXIS2_PLACEMENT_3D('',#116207,#88989,#88990) ;
#72593=AXIS2_PLACEMENT_3D('',#116208,#88991,#88992) ;
#72594=AXIS2_PLACEMENT_3D('',#116209,#88993,#88994) ;
#72595=AXIS2_PLACEMENT_3D('',#116210,#88995,#88996) ;
#72596=AXIS2_PLACEMENT_3D('',#116211,#88997,#88998) ;
#72597=AXIS2_PLACEMENT_3D('',#116212,#88999,#89000) ;
#72598=AXIS2_PLACEMENT_3D('',#116213,#89001,#89002) ;
#72599=AXIS2_PLACEMENT_3D('',#116214,#89003,#89004) ;
#72600=AXIS2_PLACEMENT_3D('',#116215,#89005,#89006) ;
#72601=AXIS2_PLACEMENT_3D('',#116216,#89007,#89008) ;
#72602=AXIS2_PLACEMENT_3D('',#116217,#89009,#89010) ;
#72603=AXIS2_PLACEMENT_3D('',#116218,#89011,#89012) ;
#72604=AXIS2_PLACEMENT_3D('',#116219,#89013,#89014) ;
#72605=AXIS2_PLACEMENT_3D('',#116220,#89015,#89016) ;
#72606=AXIS2_PLACEMENT_3D('',#116221,#89017,#89018) ;
#72607=AXIS2_PLACEMENT_3D('',#116222,#89019,#89020) ;
#72608=AXIS2_PLACEMENT_3D('',#116223,#89021,#89022) ;
#72609=AXIS2_PLACEMENT_3D('',#116224,#89023,#89024) ;
#72610=AXIS2_PLACEMENT_3D('',#116225,#89025,#89026) ;
#72611=AXIS2_PLACEMENT_3D('',#116226,#89027,#89028) ;
#72612=AXIS2_PLACEMENT_3D('',#116227,#89029,#89030) ;
#72613=AXIS2_PLACEMENT_3D('',#116228,#89031,#89032) ;
#72614=AXIS2_PLACEMENT_3D('',#116229,#89033,#89034) ;
#72615=AXIS2_PLACEMENT_3D('',#116230,#89035,#89036) ;
#72616=AXIS2_PLACEMENT_3D('',#116231,#89037,#89038) ;
#72617=AXIS2_PLACEMENT_3D('',#116232,#89039,#89040) ;
#72618=AXIS2_PLACEMENT_3D('',#116233,#89041,#89042) ;
#72619=AXIS2_PLACEMENT_3D('',#116234,#89043,#89044) ;
#72620=AXIS2_PLACEMENT_3D('',#116235,#89045,#89046) ;
#72621=AXIS2_PLACEMENT_3D('',#116236,#89047,#89048) ;
#72622=AXIS2_PLACEMENT_3D('',#116237,#89049,#89050) ;
#72623=AXIS2_PLACEMENT_3D('',#116238,#89051,#89052) ;
#72624=AXIS2_PLACEMENT_3D('',#116239,#89053,#89054) ;
#72625=AXIS2_PLACEMENT_3D('',#116240,#89055,#89056) ;
#72626=AXIS2_PLACEMENT_3D('',#116241,#89057,#89058) ;
#72627=AXIS2_PLACEMENT_3D('',#116242,#89059,#89060) ;
#72628=AXIS2_PLACEMENT_3D('',#116243,#89061,#89062) ;
#72629=AXIS2_PLACEMENT_3D('',#116244,#89063,#89064) ;
#72630=AXIS2_PLACEMENT_3D('',#116245,#89065,#89066) ;
#72631=AXIS2_PLACEMENT_3D('',#116246,#89067,#89068) ;
#72632=AXIS2_PLACEMENT_3D('',#116247,#89069,#89070) ;
#72633=AXIS2_PLACEMENT_3D('',#116248,#89071,#89072) ;
#72634=AXIS2_PLACEMENT_3D('',#116249,#89073,#89074) ;
#72635=AXIS2_PLACEMENT_3D('',#116250,#89075,#89076) ;
#72636=AXIS2_PLACEMENT_3D('',#116251,#89077,#89078) ;
#72637=AXIS2_PLACEMENT_3D('',#116252,#89079,#89080) ;
#72638=AXIS2_PLACEMENT_3D('',#116253,#89081,#89082) ;
#72639=AXIS2_PLACEMENT_3D('',#116254,#89083,#89084) ;
#72640=AXIS2_PLACEMENT_3D('',#116255,#89085,#89086) ;
#72641=AXIS2_PLACEMENT_3D('',#116256,#89087,#89088) ;
#72642=AXIS2_PLACEMENT_3D('',#116257,#89089,#89090) ;
#72643=AXIS2_PLACEMENT_3D('',#116258,#89091,#89092) ;
#72644=AXIS2_PLACEMENT_3D('',#116259,#89093,#89094) ;
#72645=AXIS2_PLACEMENT_3D('',#116260,#89095,#89096) ;
#72646=AXIS2_PLACEMENT_3D('',#116261,#89097,#89098) ;
#72647=AXIS2_PLACEMENT_3D('',#116262,#89099,#89100) ;
#72648=AXIS2_PLACEMENT_3D('',#116263,#89101,#89102) ;
#72649=AXIS2_PLACEMENT_3D('',#116264,#89103,#89104) ;
#72650=AXIS2_PLACEMENT_3D('',#116265,#89105,#89106) ;
#72651=AXIS2_PLACEMENT_3D('',#116266,#89107,#89108) ;
#72652=AXIS2_PLACEMENT_3D('',#116267,#89109,#89110) ;
#72653=AXIS2_PLACEMENT_3D('',#116268,#89111,#89112) ;
#72654=AXIS2_PLACEMENT_3D('',#116269,#89113,#89114) ;
#72655=AXIS2_PLACEMENT_3D('',#116270,#89115,#89116) ;
#72656=AXIS2_PLACEMENT_3D('',#116271,#89117,#89118) ;
#72657=AXIS2_PLACEMENT_3D('',#116272,#89119,#89120) ;
#72658=AXIS2_PLACEMENT_3D('',#116273,#89121,#89122) ;
#72659=AXIS2_PLACEMENT_3D('',#116274,#89123,#89124) ;
#72660=AXIS2_PLACEMENT_3D('',#116275,#89125,#89126) ;
#72661=AXIS2_PLACEMENT_3D('',#116276,#89127,#89128) ;
#72662=AXIS2_PLACEMENT_3D('',#116277,#89129,#89130) ;
#72663=AXIS2_PLACEMENT_3D('',#116278,#89131,#89132) ;
#72664=AXIS2_PLACEMENT_3D('',#116279,#89133,#89134) ;
#72665=AXIS2_PLACEMENT_3D('',#116280,#89135,#89136) ;
#72666=AXIS2_PLACEMENT_3D('',#116281,#89137,#89138) ;
#72667=AXIS2_PLACEMENT_3D('',#116282,#89139,#89140) ;
#72668=AXIS2_PLACEMENT_3D('',#116283,#89141,#89142) ;
#72669=AXIS2_PLACEMENT_3D('',#116284,#89143,#89144) ;
#72670=AXIS2_PLACEMENT_3D('',#116285,#89145,#89146) ;
#72671=AXIS2_PLACEMENT_3D('',#116286,#89147,#89148) ;
#72672=AXIS2_PLACEMENT_3D('',#116287,#89149,#89150) ;
#72673=AXIS2_PLACEMENT_3D('',#116288,#89151,#89152) ;
#72674=AXIS2_PLACEMENT_3D('',#116289,#89153,#89154) ;
#72675=AXIS2_PLACEMENT_3D('',#116290,#89155,#89156) ;
#72676=AXIS2_PLACEMENT_3D('',#116291,#89157,#89158) ;
#72677=AXIS2_PLACEMENT_3D('',#116292,#89159,#89160) ;
#72678=AXIS2_PLACEMENT_3D('',#116293,#89161,#89162) ;
#72679=AXIS2_PLACEMENT_3D('',#116294,#89163,#89164) ;
#72680=AXIS2_PLACEMENT_3D('',#116295,#89165,#89166) ;
#72681=AXIS2_PLACEMENT_3D('',#116296,#89167,#89168) ;
#72682=AXIS2_PLACEMENT_3D('',#116297,#89169,#89170) ;
#72683=AXIS2_PLACEMENT_3D('',#116298,#89171,#89172) ;
#72684=AXIS2_PLACEMENT_3D('',#116299,#89173,#89174) ;
#72685=AXIS2_PLACEMENT_3D('',#116300,#89175,#89176) ;
#72686=AXIS2_PLACEMENT_3D('',#116301,#89177,#89178) ;
#72687=AXIS2_PLACEMENT_3D('',#116302,#89179,#89180) ;
#72688=AXIS2_PLACEMENT_3D('',#116303,#89181,#89182) ;
#72689=AXIS2_PLACEMENT_3D('',#116304,#89183,#89184) ;
#72690=AXIS2_PLACEMENT_3D('',#116305,#89185,#89186) ;
#72691=AXIS2_PLACEMENT_3D('',#116306,#89187,#89188) ;
#72692=AXIS2_PLACEMENT_3D('',#116307,#89189,#89190) ;
#72693=AXIS2_PLACEMENT_3D('',#116308,#89191,#89192) ;
#72694=AXIS2_PLACEMENT_3D('',#116309,#89193,#89194) ;
#72695=AXIS2_PLACEMENT_3D('',#116310,#89195,#89196) ;
#72696=AXIS2_PLACEMENT_3D('',#116311,#89197,#89198) ;
#72697=AXIS2_PLACEMENT_3D('',#116312,#89199,#89200) ;
#72698=AXIS2_PLACEMENT_3D('',#116313,#89201,#89202) ;
#72699=AXIS2_PLACEMENT_3D('',#116314,#89203,#89204) ;
#72700=AXIS2_PLACEMENT_3D('',#116315,#89205,#89206) ;
#72701=AXIS2_PLACEMENT_3D('',#116316,#89207,#89208) ;
#72702=AXIS2_PLACEMENT_3D('',#116317,#89209,#89210) ;
#72703=AXIS2_PLACEMENT_3D('',#116318,#89211,#89212) ;
#72704=AXIS2_PLACEMENT_3D('',#116319,#89213,#89214) ;
#72705=AXIS2_PLACEMENT_3D('',#116320,#89215,#89216) ;
#72706=AXIS2_PLACEMENT_3D('',#116321,#89217,#89218) ;
#72707=AXIS2_PLACEMENT_3D('',#116322,#89219,#89220) ;
#72708=AXIS2_PLACEMENT_3D('',#116323,#89221,#89222) ;
#72709=AXIS2_PLACEMENT_3D('',#116324,#89223,#89224) ;
#72710=AXIS2_PLACEMENT_3D('',#116325,#89225,#89226) ;
#72711=AXIS2_PLACEMENT_3D('',#116326,#89227,#89228) ;
#72712=AXIS2_PLACEMENT_3D('',#116327,#89229,#89230) ;
#72713=AXIS2_PLACEMENT_3D('',#116328,#89231,#89232) ;
#72714=AXIS2_PLACEMENT_3D('',#116329,#89233,#89234) ;
#72715=AXIS2_PLACEMENT_3D('',#116330,#89235,#89236) ;
#72716=AXIS2_PLACEMENT_3D('',#116331,#89237,#89238) ;
#72717=AXIS2_PLACEMENT_3D('',#116332,#89239,#89240) ;
#72718=AXIS2_PLACEMENT_3D('',#116333,#89241,#89242) ;
#72719=AXIS2_PLACEMENT_3D('',#116334,#89243,#89244) ;
#72720=AXIS2_PLACEMENT_3D('',#116335,#89245,#89246) ;
#72721=AXIS2_PLACEMENT_3D('',#116336,#89247,#89248) ;
#72722=AXIS2_PLACEMENT_3D('',#116337,#89249,#89250) ;
#72723=AXIS2_PLACEMENT_3D('',#116338,#89251,#89252) ;
#72724=AXIS2_PLACEMENT_3D('',#116339,#89253,#89254) ;
#72725=AXIS2_PLACEMENT_3D('',#116340,#89255,#89256) ;
#72726=AXIS2_PLACEMENT_3D('',#116341,#89257,#89258) ;
#72727=AXIS2_PLACEMENT_3D('',#116342,#89259,#89260) ;
#72728=AXIS2_PLACEMENT_3D('',#116343,#89261,#89262) ;
#72729=AXIS2_PLACEMENT_3D('',#116344,#89263,#89264) ;
#72730=AXIS2_PLACEMENT_3D('',#116345,#89265,#89266) ;
#72731=AXIS2_PLACEMENT_3D('',#116346,#89267,#89268) ;
#72732=AXIS2_PLACEMENT_3D('',#116347,#89269,#89270) ;
#72733=AXIS2_PLACEMENT_3D('',#116348,#89271,#89272) ;
#72734=AXIS2_PLACEMENT_3D('',#116349,#89273,#89274) ;
#72735=AXIS2_PLACEMENT_3D('',#116350,#89275,#89276) ;
#72736=AXIS2_PLACEMENT_3D('',#116351,#89277,#89278) ;
#72737=AXIS2_PLACEMENT_3D('',#116352,#89279,#89280) ;
#72738=AXIS2_PLACEMENT_3D('',#116353,#89281,#89282) ;
#72739=AXIS2_PLACEMENT_3D('',#116354,#89283,#89284) ;
#72740=AXIS2_PLACEMENT_3D('',#116355,#89285,#89286) ;
#72741=AXIS2_PLACEMENT_3D('',#116356,#89287,#89288) ;
#72742=AXIS2_PLACEMENT_3D('',#116357,#89289,#89290) ;
#72743=AXIS2_PLACEMENT_3D('',#116358,#89291,#89292) ;
#72744=AXIS2_PLACEMENT_3D('',#116359,#89293,#89294) ;
#72745=AXIS2_PLACEMENT_3D('',#116360,#89295,#89296) ;
#72746=AXIS2_PLACEMENT_3D('',#116361,#89297,#89298) ;
#72747=AXIS2_PLACEMENT_3D('',#116362,#89299,#89300) ;
#72748=AXIS2_PLACEMENT_3D('',#116363,#89301,#89302) ;
#72749=AXIS2_PLACEMENT_3D('',#116364,#89303,#89304) ;
#72750=AXIS2_PLACEMENT_3D('',#116365,#89305,#89306) ;
#72751=AXIS2_PLACEMENT_3D('',#116366,#89307,#89308) ;
#72752=AXIS2_PLACEMENT_3D('',#116367,#89309,#89310) ;
#72753=AXIS2_PLACEMENT_3D('',#116368,#89311,#89312) ;
#72754=AXIS2_PLACEMENT_3D('',#116369,#89313,#89314) ;
#72755=AXIS2_PLACEMENT_3D('',#116370,#89315,#89316) ;
#72756=AXIS2_PLACEMENT_3D('',#116371,#89317,#89318) ;
#72757=AXIS2_PLACEMENT_3D('',#116372,#89319,#89320) ;
#72758=AXIS2_PLACEMENT_3D('',#116373,#89321,#89322) ;
#72759=AXIS2_PLACEMENT_3D('',#116382,#89327,#89328) ;
#72760=AXIS2_PLACEMENT_3D('',#116391,#89333,#89334) ;
#72761=AXIS2_PLACEMENT_3D('',#116400,#89339,#89340) ;
#72762=AXIS2_PLACEMENT_3D('',#116409,#89345,#89346) ;
#72763=AXIS2_PLACEMENT_3D('',#116418,#89351,#89352) ;
#72764=AXIS2_PLACEMENT_3D('',#116422,#89354,#89355) ;
#72765=AXIS2_PLACEMENT_3D('',#116424,#89356,#89357) ;
#72766=AXIS2_PLACEMENT_3D('',#116428,#89360,#89361) ;
#72767=AXIS2_PLACEMENT_3D('',#116432,#89363,#89364) ;
#72768=AXIS2_PLACEMENT_3D('',#116434,#89365,#89366) ;
#72769=AXIS2_PLACEMENT_3D('',#116438,#89369,#89370) ;
#72770=AXIS2_PLACEMENT_3D('',#116439,#89371,#89372) ;
#72771=AXIS2_PLACEMENT_3D('',#116440,#89373,#89374) ;
#72772=AXIS2_PLACEMENT_3D('',#116441,#89375,#89376) ;
#72773=AXIS2_PLACEMENT_3D('',#116442,#89377,#89378) ;
#72774=AXIS2_PLACEMENT_3D('',#116443,#89379,#89380) ;
#72775=AXIS2_PLACEMENT_3D('',#116444,#89381,#89382) ;
#72776=AXIS2_PLACEMENT_3D('',#116453,#89387,#89388) ;
#72777=AXIS2_PLACEMENT_3D('',#116459,#89392,#89393) ;
#72778=AXIS2_PLACEMENT_3D('',#116465,#89397,#89398) ;
#72779=AXIS2_PLACEMENT_3D('',#116474,#89403,#89404) ;
#72780=AXIS2_PLACEMENT_3D('',#116483,#89409,#89410) ;
#72781=AXIS2_PLACEMENT_3D('',#116489,#89414,#89415) ;
#72782=AXIS2_PLACEMENT_3D('',#116495,#89419,#89420) ;
#72783=AXIS2_PLACEMENT_3D('',#116504,#89425,#89426) ;
#72784=AXIS2_PLACEMENT_3D('',#116513,#89431,#89432) ;
#72785=AXIS2_PLACEMENT_3D('',#116522,#89437,#89438) ;
#72786=AXIS2_PLACEMENT_3D('',#116531,#89443,#89444) ;
#72787=AXIS2_PLACEMENT_3D('',#116532,#89445,#89446) ;
#72788=AXIS2_PLACEMENT_3D('',#116533,#89447,#89448) ;
#72789=AXIS2_PLACEMENT_3D('',#116534,#89449,#89450) ;
#72790=AXIS2_PLACEMENT_3D('',#116535,#89451,#89452) ;
#72791=AXIS2_PLACEMENT_3D('',#116536,#89453,#89454) ;
#72792=AXIS2_PLACEMENT_3D('',#116537,#89455,#89456) ;
#72793=AXIS2_PLACEMENT_3D('',#116538,#89457,#89458) ;
#72794=AXIS2_PLACEMENT_3D('',#116539,#89459,#89460) ;
#72795=AXIS2_PLACEMENT_3D('',#116540,#89461,#89462) ;
#72796=AXIS2_PLACEMENT_3D('',#116541,#89463,#89464) ;
#72797=AXIS2_PLACEMENT_3D('',#116542,#89465,#89466) ;
#72798=AXIS2_PLACEMENT_3D('',#116543,#89467,#89468) ;
#72799=AXIS2_PLACEMENT_3D('',#116544,#89469,#89470) ;
#72800=AXIS2_PLACEMENT_3D('',#116545,#89471,#89472) ;
#72801=AXIS2_PLACEMENT_3D('',#116546,#89473,#89474) ;
#72802=AXIS2_PLACEMENT_3D('',#116547,#89475,#89476) ;
#72803=AXIS2_PLACEMENT_3D('',#116548,#89477,#89478) ;
#72804=AXIS2_PLACEMENT_3D('',#116549,#89479,#89480) ;
#72805=AXIS2_PLACEMENT_3D('',#116550,#89481,#89482) ;
#72806=AXIS2_PLACEMENT_3D('',#116551,#89483,#89484) ;
#72807=AXIS2_PLACEMENT_3D('',#116552,#89485,#89486) ;
#72808=AXIS2_PLACEMENT_3D('',#116553,#89487,#89488) ;
#72809=AXIS2_PLACEMENT_3D('',#116554,#89489,#89490) ;
#72810=AXIS2_PLACEMENT_3D('',#116555,#89491,#89492) ;
#72811=AXIS2_PLACEMENT_3D('',#116556,#89493,#89494) ;
#72812=AXIS2_PLACEMENT_3D('',#116557,#89495,#89496) ;
#72813=AXIS2_PLACEMENT_3D('',#116558,#89497,#89498) ;
#72814=AXIS2_PLACEMENT_3D('',#116559,#89499,#89500) ;
#72815=AXIS2_PLACEMENT_3D('',#116560,#89501,#89502) ;
#72816=AXIS2_PLACEMENT_3D('',#116561,#89503,#89504) ;
#72817=AXIS2_PLACEMENT_3D('',#116562,#89505,#89506) ;
#72818=AXIS2_PLACEMENT_3D('',#116563,#89507,#89508) ;
#72819=AXIS2_PLACEMENT_3D('',#116564,#89509,#89510) ;
#72820=AXIS2_PLACEMENT_3D('',#116565,#89511,#89512) ;
#72821=AXIS2_PLACEMENT_3D('',#116566,#89513,#89514) ;
#72822=AXIS2_PLACEMENT_3D('',#116567,#89515,#89516) ;
#72823=AXIS2_PLACEMENT_3D('',#116568,#89517,#89518) ;
#72824=AXIS2_PLACEMENT_3D('',#116569,#89519,#89520) ;
#72825=AXIS2_PLACEMENT_3D('',#116570,#89521,#89522) ;
#72826=AXIS2_PLACEMENT_3D('',#116571,#89523,#89524) ;
#72827=AXIS2_PLACEMENT_3D('',#116572,#89525,#89526) ;
#72828=AXIS2_PLACEMENT_3D('',#116573,#89527,#89528) ;
#72829=AXIS2_PLACEMENT_3D('',#116574,#89529,#89530) ;
#72830=AXIS2_PLACEMENT_3D('',#116575,#89531,#89532) ;
#72831=AXIS2_PLACEMENT_3D('',#116576,#89533,#89534) ;
#72832=AXIS2_PLACEMENT_3D('',#116577,#89535,#89536) ;
#72833=AXIS2_PLACEMENT_3D('',#116578,#89537,#89538) ;
#72834=AXIS2_PLACEMENT_3D('',#116579,#89539,#89540) ;
#72835=AXIS2_PLACEMENT_3D('',#116580,#89541,#89542) ;
#72836=AXIS2_PLACEMENT_3D('',#116581,#89543,#89544) ;
#72837=AXIS2_PLACEMENT_3D('',#116582,#89545,#89546) ;
#72838=AXIS2_PLACEMENT_3D('',#116583,#89547,#89548) ;
#72839=AXIS2_PLACEMENT_3D('',#116584,#89549,#89550) ;
#72840=AXIS2_PLACEMENT_3D('',#116585,#89551,#89552) ;
#72841=AXIS2_PLACEMENT_3D('',#116586,#89553,#89554) ;
#72842=AXIS2_PLACEMENT_3D('',#116587,#89555,#89556) ;
#72843=AXIS2_PLACEMENT_3D('',#116588,#89557,#89558) ;
#72844=AXIS2_PLACEMENT_3D('',#116589,#89559,#89560) ;
#72845=AXIS2_PLACEMENT_3D('',#116590,#89561,#89562) ;
#72846=AXIS2_PLACEMENT_3D('',#116591,#89563,#89564) ;
#72847=AXIS2_PLACEMENT_3D('',#116592,#89565,#89566) ;
#72848=AXIS2_PLACEMENT_3D('',#116593,#89567,#89568) ;
#72849=AXIS2_PLACEMENT_3D('',#116594,#89569,#89570) ;
#72850=AXIS2_PLACEMENT_3D('',#116595,#89571,#89572) ;
#72851=AXIS2_PLACEMENT_3D('',#116596,#89573,#89574) ;
#72852=AXIS2_PLACEMENT_3D('',#116597,#89575,#89576) ;
#72853=AXIS2_PLACEMENT_3D('',#116598,#89577,#89578) ;
#72854=AXIS2_PLACEMENT_3D('',#116599,#89579,#89580) ;
#72855=AXIS2_PLACEMENT_3D('',#116600,#89581,#89582) ;
#72856=AXIS2_PLACEMENT_3D('',#116601,#89583,#89584) ;
#72857=AXIS2_PLACEMENT_3D('',#116602,#89585,#89586) ;
#72858=AXIS2_PLACEMENT_3D('',#116603,#89587,#89588) ;
#72859=AXIS2_PLACEMENT_3D('',#116604,#89589,#89590) ;
#72860=AXIS2_PLACEMENT_3D('',#116605,#89591,#89592) ;
#72861=AXIS2_PLACEMENT_3D('',#116606,#89593,#89594) ;
#72862=AXIS2_PLACEMENT_3D('',#116607,#89595,#89596) ;
#72863=AXIS2_PLACEMENT_3D('',#116608,#89597,#89598) ;
#72864=AXIS2_PLACEMENT_3D('',#116609,#89599,#89600) ;
#72865=AXIS2_PLACEMENT_3D('',#116610,#89601,#89602) ;
#72866=AXIS2_PLACEMENT_3D('',#116611,#89603,#89604) ;
#72867=AXIS2_PLACEMENT_3D('',#116612,#89605,#89606) ;
#72868=AXIS2_PLACEMENT_3D('',#116613,#89607,#89608) ;
#72869=AXIS2_PLACEMENT_3D('',#116614,#89609,#89610) ;
#72870=AXIS2_PLACEMENT_3D('',#116615,#89611,#89612) ;
#72871=AXIS2_PLACEMENT_3D('',#116616,#89613,#89614) ;
#72872=AXIS2_PLACEMENT_3D('',#116617,#89615,#89616) ;
#72873=AXIS2_PLACEMENT_3D('',#116618,#89617,#89618) ;
#72874=AXIS2_PLACEMENT_3D('',#116619,#89619,#89620) ;
#72875=AXIS2_PLACEMENT_3D('',#116620,#89621,#89622) ;
#72876=AXIS2_PLACEMENT_3D('',#116621,#89623,#89624) ;
#72877=AXIS2_PLACEMENT_3D('',#116622,#89625,#89626) ;
#72878=AXIS2_PLACEMENT_3D('',#116623,#89627,#89628) ;
#72879=AXIS2_PLACEMENT_3D('',#116624,#89629,#89630) ;
#72880=AXIS2_PLACEMENT_3D('',#116625,#89631,#89632) ;
#72881=AXIS2_PLACEMENT_3D('',#116626,#89633,#89634) ;
#72882=AXIS2_PLACEMENT_3D('',#116627,#89635,#89636) ;
#72883=AXIS2_PLACEMENT_3D('',#116628,#89637,#89638) ;
#72884=AXIS2_PLACEMENT_3D('',#116629,#89639,#89640) ;
#72885=AXIS2_PLACEMENT_3D('',#116630,#89641,#89642) ;
#72886=AXIS2_PLACEMENT_3D('',#116631,#89643,#89644) ;
#72887=AXIS2_PLACEMENT_3D('',#116632,#89645,#89646) ;
#72888=AXIS2_PLACEMENT_3D('',#116633,#89647,#89648) ;
#72889=AXIS2_PLACEMENT_3D('',#116634,#89649,#89650) ;
#72890=AXIS2_PLACEMENT_3D('',#116635,#89651,#89652) ;
#72891=AXIS2_PLACEMENT_3D('',#116636,#89653,#89654) ;
#72892=AXIS2_PLACEMENT_3D('',#116637,#89655,#89656) ;
#72893=AXIS2_PLACEMENT_3D('',#116638,#89657,#89658) ;
#72894=AXIS2_PLACEMENT_3D('',#116639,#89659,#89660) ;
#72895=AXIS2_PLACEMENT_3D('',#116640,#89661,#89662) ;
#72896=AXIS2_PLACEMENT_3D('',#116641,#89663,#89664) ;
#72897=AXIS2_PLACEMENT_3D('',#116642,#89665,#89666) ;
#72898=AXIS2_PLACEMENT_3D('',#116643,#89667,#89668) ;
#72899=AXIS2_PLACEMENT_3D('',#116658,#89675,#89676) ;
#72900=AXIS2_PLACEMENT_3D('',#116662,#89678,#89679) ;
#72901=AXIS2_PLACEMENT_3D('',#116664,#89681,#89682) ;
#72902=AXIS2_PLACEMENT_3D('',#116679,#89689,#89690) ;
#72903=AXIS2_PLACEMENT_3D('',#116683,#89692,#89693) ;
#72904=AXIS2_PLACEMENT_3D('',#116685,#89695,#89696) ;
#72905=AXIS2_PLACEMENT_3D('',#116700,#89703,#89704) ;
#72906=AXIS2_PLACEMENT_3D('',#116704,#89706,#89707) ;
#72907=AXIS2_PLACEMENT_3D('',#116706,#89709,#89710) ;
#72908=AXIS2_PLACEMENT_3D('',#116721,#89717,#89718) ;
#72909=AXIS2_PLACEMENT_3D('',#116725,#89720,#89721) ;
#72910=AXIS2_PLACEMENT_3D('',#116727,#89723,#89724) ;
#72911=AXIS2_PLACEMENT_3D('',#116742,#89731,#89732) ;
#72912=AXIS2_PLACEMENT_3D('',#116746,#89734,#89735) ;
#72913=AXIS2_PLACEMENT_3D('',#116748,#89737,#89738) ;
#72914=AXIS2_PLACEMENT_3D('',#116763,#89745,#89746) ;
#72915=AXIS2_PLACEMENT_3D('',#116767,#89748,#89749) ;
#72916=AXIS2_PLACEMENT_3D('',#116769,#89751,#89752) ;
#72917=AXIS2_PLACEMENT_3D('',#116784,#89759,#89760) ;
#72918=AXIS2_PLACEMENT_3D('',#116788,#89762,#89763) ;
#72919=AXIS2_PLACEMENT_3D('',#116790,#89765,#89766) ;
#72920=AXIS2_PLACEMENT_3D('',#116805,#89773,#89774) ;
#72921=AXIS2_PLACEMENT_3D('',#116809,#89776,#89777) ;
#72922=AXIS2_PLACEMENT_3D('',#116811,#89779,#89780) ;
#72923=AXIS2_PLACEMENT_3D('',#116826,#89787,#89788) ;
#72924=AXIS2_PLACEMENT_3D('',#116830,#89790,#89791) ;
#72925=AXIS2_PLACEMENT_3D('',#116832,#89793,#89794) ;
#72926=AXIS2_PLACEMENT_3D('',#116841,#89799,#89800) ;
#72927=AXIS2_PLACEMENT_3D('',#116847,#89804,#89805) ;
#72928=AXIS2_PLACEMENT_3D('',#116856,#89810,#89811) ;
#72929=AXIS2_PLACEMENT_3D('',#116865,#89816,#89817) ;
#72930=AXIS2_PLACEMENT_3D('',#116874,#89822,#89823) ;
#72931=AXIS2_PLACEMENT_3D('',#116883,#89828,#89829) ;
#72932=AXIS2_PLACEMENT_3D('',#116889,#89833,#89834) ;
#72933=AXIS2_PLACEMENT_3D('',#116898,#89839,#89840) ;
#72934=AXIS2_PLACEMENT_3D('',#116907,#89845,#89846) ;
#72935=AXIS2_PLACEMENT_3D('',#116916,#89851,#89852) ;
#72936=AXIS2_PLACEMENT_3D('',#116925,#89857,#89858) ;
#72937=AXIS2_PLACEMENT_3D('',#116931,#89862,#89863) ;
#72938=AXIS2_PLACEMENT_3D('',#116940,#89868,#89869) ;
#72939=AXIS2_PLACEMENT_3D('',#116949,#89874,#89875) ;
#72940=AXIS2_PLACEMENT_3D('',#116958,#89880,#89881) ;
#72941=AXIS2_PLACEMENT_3D('',#116967,#89886,#89887) ;
#72942=AXIS2_PLACEMENT_3D('',#116973,#89891,#89892) ;
#72943=AXIS2_PLACEMENT_3D('',#116982,#89897,#89898) ;
#72944=AXIS2_PLACEMENT_3D('',#116991,#89903,#89904) ;
#72945=AXIS2_PLACEMENT_3D('',#117000,#89909,#89910) ;
#72946=AXIS2_PLACEMENT_3D('',#117009,#89915,#89916) ;
#72947=AXIS2_PLACEMENT_3D('',#117015,#89920,#89921) ;
#72948=AXIS2_PLACEMENT_3D('',#117024,#89926,#89927) ;
#72949=AXIS2_PLACEMENT_3D('',#117033,#89932,#89933) ;
#72950=AXIS2_PLACEMENT_3D('',#117042,#89938,#89939) ;
#72951=AXIS2_PLACEMENT_3D('',#117051,#89944,#89945) ;
#72952=AXIS2_PLACEMENT_3D('',#117057,#89949,#89950) ;
#72953=AXIS2_PLACEMENT_3D('',#117066,#89955,#89956) ;
#72954=AXIS2_PLACEMENT_3D('',#117075,#89961,#89962) ;
#72955=AXIS2_PLACEMENT_3D('',#117084,#89967,#89968) ;
#72956=AXIS2_PLACEMENT_3D('',#117093,#89973,#89974) ;
#72957=AXIS2_PLACEMENT_3D('',#117099,#89978,#89979) ;
#72958=AXIS2_PLACEMENT_3D('',#117108,#89984,#89985) ;
#72959=AXIS2_PLACEMENT_3D('',#117117,#89990,#89991) ;
#72960=AXIS2_PLACEMENT_3D('',#117126,#89996,#89997) ;
#72961=AXIS2_PLACEMENT_3D('',#117135,#90002,#90003) ;
#72962=AXIS2_PLACEMENT_3D('',#117141,#90007,#90008) ;
#72963=AXIS2_PLACEMENT_3D('',#117150,#90013,#90014) ;
#72964=AXIS2_PLACEMENT_3D('',#117159,#90019,#90020) ;
#72965=AXIS2_PLACEMENT_3D('',#117168,#90025,#90026) ;
#72966=AXIS2_PLACEMENT_3D('',#117177,#90031,#90032) ;
#72967=AXIS2_PLACEMENT_3D('',#117183,#90036,#90037) ;
#72968=AXIS2_PLACEMENT_3D('',#117192,#90042,#90043) ;
#72969=AXIS2_PLACEMENT_3D('',#117201,#90048,#90049) ;
#72970=AXIS2_PLACEMENT_3D('',#117210,#90054,#90055) ;
#72971=AXIS2_PLACEMENT_3D('',#117215,#90057,#90058) ;
#72972=AXIS2_PLACEMENT_3D('',#117218,#90060,#90061) ;
#72973=AXIS2_PLACEMENT_3D('',#117219,#90062,#90063) ;
#72974=AXIS2_PLACEMENT_3D('',#117225,#90067,#90068) ;
#72975=AXIS2_PLACEMENT_3D('',#117227,#90069,#90070) ;
#72976=AXIS2_PLACEMENT_3D('',#117230,#90072,#90073) ;
#72977=AXIS2_PLACEMENT_3D('',#117231,#90074,#90075) ;
#72978=AXIS2_PLACEMENT_3D('',#117237,#90079,#90080) ;
#72979=AXIS2_PLACEMENT_3D('',#117239,#90081,#90082) ;
#72980=AXIS2_PLACEMENT_3D('',#117242,#90084,#90085) ;
#72981=AXIS2_PLACEMENT_3D('',#117243,#90086,#90087) ;
#72982=AXIS2_PLACEMENT_3D('',#117248,#90091,#90092) ;
#72983=AXIS2_PLACEMENT_3D('',#117251,#90094,#90095) ;
#72984=AXIS2_PLACEMENT_3D('',#117252,#90096,#90097) ;
#72985=AXIS2_PLACEMENT_3D('',#117255,#90100,#90101) ;
#72986=AXIS2_PLACEMENT_3D('',#117261,#90105,#90106) ;
#72987=AXIS2_PLACEMENT_3D('',#117263,#90107,#90108) ;
#72988=AXIS2_PLACEMENT_3D('',#117266,#90110,#90111) ;
#72989=AXIS2_PLACEMENT_3D('',#117267,#90112,#90113) ;
#72990=AXIS2_PLACEMENT_3D('',#117273,#90117,#90118) ;
#72991=AXIS2_PLACEMENT_3D('',#117275,#90119,#90120) ;
#72992=AXIS2_PLACEMENT_3D('',#117278,#90122,#90123) ;
#72993=AXIS2_PLACEMENT_3D('',#117279,#90124,#90125) ;
#72994=AXIS2_PLACEMENT_3D('',#117285,#90129,#90130) ;
#72995=AXIS2_PLACEMENT_3D('',#117287,#90131,#90132) ;
#72996=AXIS2_PLACEMENT_3D('',#117290,#90134,#90135) ;
#72997=AXIS2_PLACEMENT_3D('',#117291,#90136,#90137) ;
#72998=AXIS2_PLACEMENT_3D('',#117297,#90141,#90142) ;
#72999=AXIS2_PLACEMENT_3D('',#117299,#90143,#90144) ;
#73000=AXIS2_PLACEMENT_3D('',#117302,#90146,#90147) ;
#73001=AXIS2_PLACEMENT_3D('',#117303,#90148,#90149) ;
#73002=AXIS2_PLACEMENT_3D('',#117309,#90153,#90154) ;
#73003=AXIS2_PLACEMENT_3D('',#117311,#90155,#90156) ;
#73004=AXIS2_PLACEMENT_3D('',#117314,#90158,#90159) ;
#73005=AXIS2_PLACEMENT_3D('',#117315,#90160,#90161) ;
#73006=AXIS2_PLACEMENT_3D('',#117321,#90165,#90166) ;
#73007=AXIS2_PLACEMENT_3D('',#117323,#90167,#90168) ;
#73008=AXIS2_PLACEMENT_3D('',#117326,#90170,#90171) ;
#73009=AXIS2_PLACEMENT_3D('',#117327,#90172,#90173) ;
#73010=AXIS2_PLACEMENT_3D('',#117329,#90174,#90175) ;
#73011=AXIS2_PLACEMENT_3D('',#117332,#90177,#90178) ;
#73012=AXIS2_PLACEMENT_3D('',#117333,#90179,#90180) ;
#73013=AXIS2_PLACEMENT_3D('',#117335,#90181,#90182) ;
#73014=AXIS2_PLACEMENT_3D('',#117338,#90184,#90185) ;
#73015=AXIS2_PLACEMENT_3D('',#117339,#90186,#90187) ;
#73016=AXIS2_PLACEMENT_3D('',#117345,#90191,#90192) ;
#73017=AXIS2_PLACEMENT_3D('',#117347,#90193,#90194) ;
#73018=AXIS2_PLACEMENT_3D('',#117350,#90196,#90197) ;
#73019=AXIS2_PLACEMENT_3D('',#117351,#90198,#90199) ;
#73020=AXIS2_PLACEMENT_3D('',#117357,#90203,#90204) ;
#73021=AXIS2_PLACEMENT_3D('',#117359,#90205,#90206) ;
#73022=AXIS2_PLACEMENT_3D('',#117362,#90208,#90209) ;
#73023=AXIS2_PLACEMENT_3D('',#117363,#90210,#90211) ;
#73024=AXIS2_PLACEMENT_3D('',#117366,#90214,#90215) ;
#73025=AXIS2_PLACEMENT_3D('',#117369,#90216,#90217) ;
#73026=AXIS2_PLACEMENT_3D('',#117373,#90219,#90220) ;
#73027=AXIS2_PLACEMENT_3D('',#117381,#90224,#90225) ;
#73028=AXIS2_PLACEMENT_3D('',#117389,#90229,#90230) ;
#73029=AXIS2_PLACEMENT_3D('',#117393,#90232,#90233) ;
#73030=AXIS2_PLACEMENT_3D('',#117402,#90239,#90240) ;
#73031=AXIS2_PLACEMENT_3D('',#117407,#90242,#90243) ;
#73032=AXIS2_PLACEMENT_3D('',#117410,#90245,#90246) ;
#73033=AXIS2_PLACEMENT_3D('',#117411,#90247,#90248) ;
#73034=AXIS2_PLACEMENT_3D('',#117417,#90252,#90253) ;
#73035=AXIS2_PLACEMENT_3D('',#117419,#90254,#90255) ;
#73036=AXIS2_PLACEMENT_3D('',#117422,#90257,#90258) ;
#73037=AXIS2_PLACEMENT_3D('',#117423,#90259,#90260) ;
#73038=AXIS2_PLACEMENT_3D('',#117429,#90264,#90265) ;
#73039=AXIS2_PLACEMENT_3D('',#117431,#90266,#90267) ;
#73040=AXIS2_PLACEMENT_3D('',#117434,#90269,#90270) ;
#73041=AXIS2_PLACEMENT_3D('',#117435,#90271,#90272) ;
#73042=AXIS2_PLACEMENT_3D('',#117440,#90276,#90277) ;
#73043=AXIS2_PLACEMENT_3D('',#117443,#90279,#90280) ;
#73044=AXIS2_PLACEMENT_3D('',#117444,#90281,#90282) ;
#73045=AXIS2_PLACEMENT_3D('',#117447,#90285,#90286) ;
#73046=AXIS2_PLACEMENT_3D('',#117453,#90290,#90291) ;
#73047=AXIS2_PLACEMENT_3D('',#117455,#90292,#90293) ;
#73048=AXIS2_PLACEMENT_3D('',#117458,#90295,#90296) ;
#73049=AXIS2_PLACEMENT_3D('',#117459,#90297,#90298) ;
#73050=AXIS2_PLACEMENT_3D('',#117465,#90302,#90303) ;
#73051=AXIS2_PLACEMENT_3D('',#117467,#90304,#90305) ;
#73052=AXIS2_PLACEMENT_3D('',#117470,#90307,#90308) ;
#73053=AXIS2_PLACEMENT_3D('',#117471,#90309,#90310) ;
#73054=AXIS2_PLACEMENT_3D('',#117477,#90314,#90315) ;
#73055=AXIS2_PLACEMENT_3D('',#117479,#90316,#90317) ;
#73056=AXIS2_PLACEMENT_3D('',#117482,#90319,#90320) ;
#73057=AXIS2_PLACEMENT_3D('',#117483,#90321,#90322) ;
#73058=AXIS2_PLACEMENT_3D('',#117489,#90326,#90327) ;
#73059=AXIS2_PLACEMENT_3D('',#117491,#90328,#90329) ;
#73060=AXIS2_PLACEMENT_3D('',#117494,#90331,#90332) ;
#73061=AXIS2_PLACEMENT_3D('',#117495,#90333,#90334) ;
#73062=AXIS2_PLACEMENT_3D('',#117501,#90338,#90339) ;
#73063=AXIS2_PLACEMENT_3D('',#117503,#90340,#90341) ;
#73064=AXIS2_PLACEMENT_3D('',#117506,#90343,#90344) ;
#73065=AXIS2_PLACEMENT_3D('',#117507,#90345,#90346) ;
#73066=AXIS2_PLACEMENT_3D('',#117513,#90350,#90351) ;
#73067=AXIS2_PLACEMENT_3D('',#117515,#90352,#90353) ;
#73068=AXIS2_PLACEMENT_3D('',#117518,#90355,#90356) ;
#73069=AXIS2_PLACEMENT_3D('',#117519,#90357,#90358) ;
#73070=AXIS2_PLACEMENT_3D('',#117521,#90359,#90360) ;
#73071=AXIS2_PLACEMENT_3D('',#117524,#90362,#90363) ;
#73072=AXIS2_PLACEMENT_3D('',#117525,#90364,#90365) ;
#73073=AXIS2_PLACEMENT_3D('',#117527,#90366,#90367) ;
#73074=AXIS2_PLACEMENT_3D('',#117530,#90369,#90370) ;
#73075=AXIS2_PLACEMENT_3D('',#117531,#90371,#90372) ;
#73076=AXIS2_PLACEMENT_3D('',#117537,#90376,#90377) ;
#73077=AXIS2_PLACEMENT_3D('',#117539,#90378,#90379) ;
#73078=AXIS2_PLACEMENT_3D('',#117542,#90381,#90382) ;
#73079=AXIS2_PLACEMENT_3D('',#117543,#90383,#90384) ;
#73080=AXIS2_PLACEMENT_3D('',#117549,#90388,#90389) ;
#73081=AXIS2_PLACEMENT_3D('',#117551,#90390,#90391) ;
#73082=AXIS2_PLACEMENT_3D('',#117554,#90393,#90394) ;
#73083=AXIS2_PLACEMENT_3D('',#117555,#90395,#90396) ;
#73084=AXIS2_PLACEMENT_3D('',#117558,#90399,#90400) ;
#73085=AXIS2_PLACEMENT_3D('',#117561,#90401,#90402) ;
#73086=AXIS2_PLACEMENT_3D('',#117565,#90404,#90405) ;
#73087=AXIS2_PLACEMENT_3D('',#117573,#90409,#90410) ;
#73088=AXIS2_PLACEMENT_3D('',#117581,#90414,#90415) ;
#73089=AXIS2_PLACEMENT_3D('',#117585,#90417,#90418) ;
#73090=AXIS2_PLACEMENT_3D('',#117594,#90424,#90425) ;
#73091=AXIS2_PLACEMENT_3D('',#117599,#90427,#90428) ;
#73092=AXIS2_PLACEMENT_3D('',#117602,#90430,#90431) ;
#73093=AXIS2_PLACEMENT_3D('',#117603,#90432,#90433) ;
#73094=AXIS2_PLACEMENT_3D('',#117609,#90437,#90438) ;
#73095=AXIS2_PLACEMENT_3D('',#117611,#90439,#90440) ;
#73096=AXIS2_PLACEMENT_3D('',#117614,#90442,#90443) ;
#73097=AXIS2_PLACEMENT_3D('',#117615,#90444,#90445) ;
#73098=AXIS2_PLACEMENT_3D('',#117621,#90449,#90450) ;
#73099=AXIS2_PLACEMENT_3D('',#117623,#90451,#90452) ;
#73100=AXIS2_PLACEMENT_3D('',#117626,#90454,#90455) ;
#73101=AXIS2_PLACEMENT_3D('',#117627,#90456,#90457) ;
#73102=AXIS2_PLACEMENT_3D('',#117632,#90461,#90462) ;
#73103=AXIS2_PLACEMENT_3D('',#117635,#90464,#90465) ;
#73104=AXIS2_PLACEMENT_3D('',#117636,#90466,#90467) ;
#73105=AXIS2_PLACEMENT_3D('',#117639,#90470,#90471) ;
#73106=AXIS2_PLACEMENT_3D('',#117645,#90475,#90476) ;
#73107=AXIS2_PLACEMENT_3D('',#117647,#90477,#90478) ;
#73108=AXIS2_PLACEMENT_3D('',#117650,#90480,#90481) ;
#73109=AXIS2_PLACEMENT_3D('',#117651,#90482,#90483) ;
#73110=AXIS2_PLACEMENT_3D('',#117657,#90487,#90488) ;
#73111=AXIS2_PLACEMENT_3D('',#117659,#90489,#90490) ;
#73112=AXIS2_PLACEMENT_3D('',#117662,#90492,#90493) ;
#73113=AXIS2_PLACEMENT_3D('',#117663,#90494,#90495) ;
#73114=AXIS2_PLACEMENT_3D('',#117669,#90499,#90500) ;
#73115=AXIS2_PLACEMENT_3D('',#117671,#90501,#90502) ;
#73116=AXIS2_PLACEMENT_3D('',#117674,#90504,#90505) ;
#73117=AXIS2_PLACEMENT_3D('',#117675,#90506,#90507) ;
#73118=AXIS2_PLACEMENT_3D('',#117681,#90511,#90512) ;
#73119=AXIS2_PLACEMENT_3D('',#117683,#90513,#90514) ;
#73120=AXIS2_PLACEMENT_3D('',#117686,#90516,#90517) ;
#73121=AXIS2_PLACEMENT_3D('',#117687,#90518,#90519) ;
#73122=AXIS2_PLACEMENT_3D('',#117693,#90523,#90524) ;
#73123=AXIS2_PLACEMENT_3D('',#117695,#90525,#90526) ;
#73124=AXIS2_PLACEMENT_3D('',#117698,#90528,#90529) ;
#73125=AXIS2_PLACEMENT_3D('',#117699,#90530,#90531) ;
#73126=AXIS2_PLACEMENT_3D('',#117705,#90535,#90536) ;
#73127=AXIS2_PLACEMENT_3D('',#117707,#90537,#90538) ;
#73128=AXIS2_PLACEMENT_3D('',#117710,#90540,#90541) ;
#73129=AXIS2_PLACEMENT_3D('',#117711,#90542,#90543) ;
#73130=AXIS2_PLACEMENT_3D('',#117713,#90544,#90545) ;
#73131=AXIS2_PLACEMENT_3D('',#117716,#90547,#90548) ;
#73132=AXIS2_PLACEMENT_3D('',#117717,#90549,#90550) ;
#73133=AXIS2_PLACEMENT_3D('',#117719,#90551,#90552) ;
#73134=AXIS2_PLACEMENT_3D('',#117722,#90554,#90555) ;
#73135=AXIS2_PLACEMENT_3D('',#117723,#90556,#90557) ;
#73136=AXIS2_PLACEMENT_3D('',#117729,#90561,#90562) ;
#73137=AXIS2_PLACEMENT_3D('',#117731,#90563,#90564) ;
#73138=AXIS2_PLACEMENT_3D('',#117734,#90566,#90567) ;
#73139=AXIS2_PLACEMENT_3D('',#117735,#90568,#90569) ;
#73140=AXIS2_PLACEMENT_3D('',#117741,#90573,#90574) ;
#73141=AXIS2_PLACEMENT_3D('',#117743,#90575,#90576) ;
#73142=AXIS2_PLACEMENT_3D('',#117746,#90578,#90579) ;
#73143=AXIS2_PLACEMENT_3D('',#117747,#90580,#90581) ;
#73144=AXIS2_PLACEMENT_3D('',#117750,#90584,#90585) ;
#73145=AXIS2_PLACEMENT_3D('',#117753,#90586,#90587) ;
#73146=AXIS2_PLACEMENT_3D('',#117757,#90589,#90590) ;
#73147=AXIS2_PLACEMENT_3D('',#117765,#90594,#90595) ;
#73148=AXIS2_PLACEMENT_3D('',#117773,#90599,#90600) ;
#73149=AXIS2_PLACEMENT_3D('',#117777,#90602,#90603) ;
#73150=AXIS2_PLACEMENT_3D('',#117786,#90609,#90610) ;
#73151=AXIS2_PLACEMENT_3D('',#117791,#90612,#90613) ;
#73152=AXIS2_PLACEMENT_3D('',#117794,#90615,#90616) ;
#73153=AXIS2_PLACEMENT_3D('',#117795,#90617,#90618) ;
#73154=AXIS2_PLACEMENT_3D('',#117801,#90622,#90623) ;
#73155=AXIS2_PLACEMENT_3D('',#117803,#90624,#90625) ;
#73156=AXIS2_PLACEMENT_3D('',#117806,#90627,#90628) ;
#73157=AXIS2_PLACEMENT_3D('',#117807,#90629,#90630) ;
#73158=AXIS2_PLACEMENT_3D('',#117813,#90634,#90635) ;
#73159=AXIS2_PLACEMENT_3D('',#117815,#90636,#90637) ;
#73160=AXIS2_PLACEMENT_3D('',#117818,#90639,#90640) ;
#73161=AXIS2_PLACEMENT_3D('',#117819,#90641,#90642) ;
#73162=AXIS2_PLACEMENT_3D('',#117824,#90646,#90647) ;
#73163=AXIS2_PLACEMENT_3D('',#117827,#90649,#90650) ;
#73164=AXIS2_PLACEMENT_3D('',#117828,#90651,#90652) ;
#73165=AXIS2_PLACEMENT_3D('',#117831,#90655,#90656) ;
#73166=AXIS2_PLACEMENT_3D('',#117837,#90660,#90661) ;
#73167=AXIS2_PLACEMENT_3D('',#117839,#90662,#90663) ;
#73168=AXIS2_PLACEMENT_3D('',#117842,#90665,#90666) ;
#73169=AXIS2_PLACEMENT_3D('',#117843,#90667,#90668) ;
#73170=AXIS2_PLACEMENT_3D('',#117849,#90672,#90673) ;
#73171=AXIS2_PLACEMENT_3D('',#117851,#90674,#90675) ;
#73172=AXIS2_PLACEMENT_3D('',#117854,#90677,#90678) ;
#73173=AXIS2_PLACEMENT_3D('',#117855,#90679,#90680) ;
#73174=AXIS2_PLACEMENT_3D('',#117861,#90684,#90685) ;
#73175=AXIS2_PLACEMENT_3D('',#117863,#90686,#90687) ;
#73176=AXIS2_PLACEMENT_3D('',#117866,#90689,#90690) ;
#73177=AXIS2_PLACEMENT_3D('',#117867,#90691,#90692) ;
#73178=AXIS2_PLACEMENT_3D('',#117873,#90696,#90697) ;
#73179=AXIS2_PLACEMENT_3D('',#117875,#90698,#90699) ;
#73180=AXIS2_PLACEMENT_3D('',#117878,#90701,#90702) ;
#73181=AXIS2_PLACEMENT_3D('',#117879,#90703,#90704) ;
#73182=AXIS2_PLACEMENT_3D('',#117885,#90708,#90709) ;
#73183=AXIS2_PLACEMENT_3D('',#117887,#90710,#90711) ;
#73184=AXIS2_PLACEMENT_3D('',#117890,#90713,#90714) ;
#73185=AXIS2_PLACEMENT_3D('',#117891,#90715,#90716) ;
#73186=AXIS2_PLACEMENT_3D('',#117897,#90720,#90721) ;
#73187=AXIS2_PLACEMENT_3D('',#117899,#90722,#90723) ;
#73188=AXIS2_PLACEMENT_3D('',#117902,#90725,#90726) ;
#73189=AXIS2_PLACEMENT_3D('',#117903,#90727,#90728) ;
#73190=AXIS2_PLACEMENT_3D('',#117905,#90729,#90730) ;
#73191=AXIS2_PLACEMENT_3D('',#117908,#90732,#90733) ;
#73192=AXIS2_PLACEMENT_3D('',#117909,#90734,#90735) ;
#73193=AXIS2_PLACEMENT_3D('',#117911,#90736,#90737) ;
#73194=AXIS2_PLACEMENT_3D('',#117914,#90739,#90740) ;
#73195=AXIS2_PLACEMENT_3D('',#117915,#90741,#90742) ;
#73196=AXIS2_PLACEMENT_3D('',#117921,#90746,#90747) ;
#73197=AXIS2_PLACEMENT_3D('',#117923,#90748,#90749) ;
#73198=AXIS2_PLACEMENT_3D('',#117926,#90751,#90752) ;
#73199=AXIS2_PLACEMENT_3D('',#117927,#90753,#90754) ;
#73200=AXIS2_PLACEMENT_3D('',#117933,#90758,#90759) ;
#73201=AXIS2_PLACEMENT_3D('',#117935,#90760,#90761) ;
#73202=AXIS2_PLACEMENT_3D('',#117938,#90763,#90764) ;
#73203=AXIS2_PLACEMENT_3D('',#117939,#90765,#90766) ;
#73204=AXIS2_PLACEMENT_3D('',#117942,#90769,#90770) ;
#73205=AXIS2_PLACEMENT_3D('',#117945,#90771,#90772) ;
#73206=AXIS2_PLACEMENT_3D('',#117949,#90774,#90775) ;
#73207=AXIS2_PLACEMENT_3D('',#117957,#90779,#90780) ;
#73208=AXIS2_PLACEMENT_3D('',#117965,#90784,#90785) ;
#73209=AXIS2_PLACEMENT_3D('',#117969,#90787,#90788) ;
#73210=AXIS2_PLACEMENT_3D('',#117978,#90794,#90795) ;
#73211=AXIS2_PLACEMENT_3D('',#117983,#90797,#90798) ;
#73212=AXIS2_PLACEMENT_3D('',#117986,#90800,#90801) ;
#73213=AXIS2_PLACEMENT_3D('',#117987,#90802,#90803) ;
#73214=AXIS2_PLACEMENT_3D('',#117993,#90807,#90808) ;
#73215=AXIS2_PLACEMENT_3D('',#117995,#90809,#90810) ;
#73216=AXIS2_PLACEMENT_3D('',#117998,#90812,#90813) ;
#73217=AXIS2_PLACEMENT_3D('',#117999,#90814,#90815) ;
#73218=AXIS2_PLACEMENT_3D('',#118005,#90819,#90820) ;
#73219=AXIS2_PLACEMENT_3D('',#118007,#90821,#90822) ;
#73220=AXIS2_PLACEMENT_3D('',#118010,#90824,#90825) ;
#73221=AXIS2_PLACEMENT_3D('',#118011,#90826,#90827) ;
#73222=AXIS2_PLACEMENT_3D('',#118016,#90831,#90832) ;
#73223=AXIS2_PLACEMENT_3D('',#118019,#90834,#90835) ;
#73224=AXIS2_PLACEMENT_3D('',#118020,#90836,#90837) ;
#73225=AXIS2_PLACEMENT_3D('',#118023,#90840,#90841) ;
#73226=AXIS2_PLACEMENT_3D('',#118029,#90845,#90846) ;
#73227=AXIS2_PLACEMENT_3D('',#118031,#90847,#90848) ;
#73228=AXIS2_PLACEMENT_3D('',#118034,#90850,#90851) ;
#73229=AXIS2_PLACEMENT_3D('',#118035,#90852,#90853) ;
#73230=AXIS2_PLACEMENT_3D('',#118041,#90857,#90858) ;
#73231=AXIS2_PLACEMENT_3D('',#118043,#90859,#90860) ;
#73232=AXIS2_PLACEMENT_3D('',#118046,#90862,#90863) ;
#73233=AXIS2_PLACEMENT_3D('',#118047,#90864,#90865) ;
#73234=AXIS2_PLACEMENT_3D('',#118053,#90869,#90870) ;
#73235=AXIS2_PLACEMENT_3D('',#118055,#90871,#90872) ;
#73236=AXIS2_PLACEMENT_3D('',#118058,#90874,#90875) ;
#73237=AXIS2_PLACEMENT_3D('',#118059,#90876,#90877) ;
#73238=AXIS2_PLACEMENT_3D('',#118065,#90881,#90882) ;
#73239=AXIS2_PLACEMENT_3D('',#118067,#90883,#90884) ;
#73240=AXIS2_PLACEMENT_3D('',#118070,#90886,#90887) ;
#73241=AXIS2_PLACEMENT_3D('',#118071,#90888,#90889) ;
#73242=AXIS2_PLACEMENT_3D('',#118077,#90893,#90894) ;
#73243=AXIS2_PLACEMENT_3D('',#118079,#90895,#90896) ;
#73244=AXIS2_PLACEMENT_3D('',#118082,#90898,#90899) ;
#73245=AXIS2_PLACEMENT_3D('',#118083,#90900,#90901) ;
#73246=AXIS2_PLACEMENT_3D('',#118089,#90905,#90906) ;
#73247=AXIS2_PLACEMENT_3D('',#118091,#90907,#90908) ;
#73248=AXIS2_PLACEMENT_3D('',#118094,#90910,#90911) ;
#73249=AXIS2_PLACEMENT_3D('',#118095,#90912,#90913) ;
#73250=AXIS2_PLACEMENT_3D('',#118097,#90914,#90915) ;
#73251=AXIS2_PLACEMENT_3D('',#118100,#90917,#90918) ;
#73252=AXIS2_PLACEMENT_3D('',#118101,#90919,#90920) ;
#73253=AXIS2_PLACEMENT_3D('',#118103,#90921,#90922) ;
#73254=AXIS2_PLACEMENT_3D('',#118106,#90924,#90925) ;
#73255=AXIS2_PLACEMENT_3D('',#118107,#90926,#90927) ;
#73256=AXIS2_PLACEMENT_3D('',#118113,#90931,#90932) ;
#73257=AXIS2_PLACEMENT_3D('',#118115,#90933,#90934) ;
#73258=AXIS2_PLACEMENT_3D('',#118118,#90936,#90937) ;
#73259=AXIS2_PLACEMENT_3D('',#118119,#90938,#90939) ;
#73260=AXIS2_PLACEMENT_3D('',#118125,#90943,#90944) ;
#73261=AXIS2_PLACEMENT_3D('',#118127,#90945,#90946) ;
#73262=AXIS2_PLACEMENT_3D('',#118130,#90948,#90949) ;
#73263=AXIS2_PLACEMENT_3D('',#118131,#90950,#90951) ;
#73264=AXIS2_PLACEMENT_3D('',#118134,#90954,#90955) ;
#73265=AXIS2_PLACEMENT_3D('',#118137,#90956,#90957) ;
#73266=AXIS2_PLACEMENT_3D('',#118141,#90959,#90960) ;
#73267=AXIS2_PLACEMENT_3D('',#118149,#90964,#90965) ;
#73268=AXIS2_PLACEMENT_3D('',#118157,#90969,#90970) ;
#73269=AXIS2_PLACEMENT_3D('',#118161,#90972,#90973) ;
#73270=AXIS2_PLACEMENT_3D('',#118170,#90979,#90980) ;
#73271=AXIS2_PLACEMENT_3D('',#118175,#90982,#90983) ;
#73272=AXIS2_PLACEMENT_3D('',#118178,#90985,#90986) ;
#73273=AXIS2_PLACEMENT_3D('',#118179,#90987,#90988) ;
#73274=AXIS2_PLACEMENT_3D('',#118185,#90992,#90993) ;
#73275=AXIS2_PLACEMENT_3D('',#118187,#90994,#90995) ;
#73276=AXIS2_PLACEMENT_3D('',#118190,#90997,#90998) ;
#73277=AXIS2_PLACEMENT_3D('',#118191,#90999,#91000) ;
#73278=AXIS2_PLACEMENT_3D('',#118197,#91004,#91005) ;
#73279=AXIS2_PLACEMENT_3D('',#118199,#91006,#91007) ;
#73280=AXIS2_PLACEMENT_3D('',#118202,#91009,#91010) ;
#73281=AXIS2_PLACEMENT_3D('',#118203,#91011,#91012) ;
#73282=AXIS2_PLACEMENT_3D('',#118208,#91016,#91017) ;
#73283=AXIS2_PLACEMENT_3D('',#118211,#91019,#91020) ;
#73284=AXIS2_PLACEMENT_3D('',#118212,#91021,#91022) ;
#73285=AXIS2_PLACEMENT_3D('',#118215,#91025,#91026) ;
#73286=AXIS2_PLACEMENT_3D('',#118221,#91030,#91031) ;
#73287=AXIS2_PLACEMENT_3D('',#118223,#91032,#91033) ;
#73288=AXIS2_PLACEMENT_3D('',#118226,#91035,#91036) ;
#73289=AXIS2_PLACEMENT_3D('',#118227,#91037,#91038) ;
#73290=AXIS2_PLACEMENT_3D('',#118233,#91042,#91043) ;
#73291=AXIS2_PLACEMENT_3D('',#118235,#91044,#91045) ;
#73292=AXIS2_PLACEMENT_3D('',#118238,#91047,#91048) ;
#73293=AXIS2_PLACEMENT_3D('',#118239,#91049,#91050) ;
#73294=AXIS2_PLACEMENT_3D('',#118245,#91054,#91055) ;
#73295=AXIS2_PLACEMENT_3D('',#118247,#91056,#91057) ;
#73296=AXIS2_PLACEMENT_3D('',#118250,#91059,#91060) ;
#73297=AXIS2_PLACEMENT_3D('',#118251,#91061,#91062) ;
#73298=AXIS2_PLACEMENT_3D('',#118257,#91066,#91067) ;
#73299=AXIS2_PLACEMENT_3D('',#118259,#91068,#91069) ;
#73300=AXIS2_PLACEMENT_3D('',#118262,#91071,#91072) ;
#73301=AXIS2_PLACEMENT_3D('',#118263,#91073,#91074) ;
#73302=AXIS2_PLACEMENT_3D('',#118269,#91078,#91079) ;
#73303=AXIS2_PLACEMENT_3D('',#118271,#91080,#91081) ;
#73304=AXIS2_PLACEMENT_3D('',#118274,#91083,#91084) ;
#73305=AXIS2_PLACEMENT_3D('',#118275,#91085,#91086) ;
#73306=AXIS2_PLACEMENT_3D('',#118281,#91090,#91091) ;
#73307=AXIS2_PLACEMENT_3D('',#118283,#91092,#91093) ;
#73308=AXIS2_PLACEMENT_3D('',#118286,#91095,#91096) ;
#73309=AXIS2_PLACEMENT_3D('',#118287,#91097,#91098) ;
#73310=AXIS2_PLACEMENT_3D('',#118289,#91099,#91100) ;
#73311=AXIS2_PLACEMENT_3D('',#118292,#91102,#91103) ;
#73312=AXIS2_PLACEMENT_3D('',#118293,#91104,#91105) ;
#73313=AXIS2_PLACEMENT_3D('',#118295,#91106,#91107) ;
#73314=AXIS2_PLACEMENT_3D('',#118298,#91109,#91110) ;
#73315=AXIS2_PLACEMENT_3D('',#118299,#91111,#91112) ;
#73316=AXIS2_PLACEMENT_3D('',#118305,#91116,#91117) ;
#73317=AXIS2_PLACEMENT_3D('',#118307,#91118,#91119) ;
#73318=AXIS2_PLACEMENT_3D('',#118310,#91121,#91122) ;
#73319=AXIS2_PLACEMENT_3D('',#118311,#91123,#91124) ;
#73320=AXIS2_PLACEMENT_3D('',#118317,#91128,#91129) ;
#73321=AXIS2_PLACEMENT_3D('',#118319,#91130,#91131) ;
#73322=AXIS2_PLACEMENT_3D('',#118322,#91133,#91134) ;
#73323=AXIS2_PLACEMENT_3D('',#118323,#91135,#91136) ;
#73324=AXIS2_PLACEMENT_3D('',#118326,#91139,#91140) ;
#73325=AXIS2_PLACEMENT_3D('',#118329,#91141,#91142) ;
#73326=AXIS2_PLACEMENT_3D('',#118333,#91144,#91145) ;
#73327=AXIS2_PLACEMENT_3D('',#118341,#91149,#91150) ;
#73328=AXIS2_PLACEMENT_3D('',#118349,#91154,#91155) ;
#73329=AXIS2_PLACEMENT_3D('',#118353,#91157,#91158) ;
#73330=AXIS2_PLACEMENT_3D('',#118362,#91164,#91165) ;
#73331=AXIS2_PLACEMENT_3D('',#118367,#91167,#91168) ;
#73332=AXIS2_PLACEMENT_3D('',#118370,#91170,#91171) ;
#73333=AXIS2_PLACEMENT_3D('',#118371,#91172,#91173) ;
#73334=AXIS2_PLACEMENT_3D('',#118377,#91177,#91178) ;
#73335=AXIS2_PLACEMENT_3D('',#118379,#91179,#91180) ;
#73336=AXIS2_PLACEMENT_3D('',#118382,#91182,#91183) ;
#73337=AXIS2_PLACEMENT_3D('',#118383,#91184,#91185) ;
#73338=AXIS2_PLACEMENT_3D('',#118389,#91189,#91190) ;
#73339=AXIS2_PLACEMENT_3D('',#118391,#91191,#91192) ;
#73340=AXIS2_PLACEMENT_3D('',#118394,#91194,#91195) ;
#73341=AXIS2_PLACEMENT_3D('',#118395,#91196,#91197) ;
#73342=AXIS2_PLACEMENT_3D('',#118400,#91201,#91202) ;
#73343=AXIS2_PLACEMENT_3D('',#118403,#91204,#91205) ;
#73344=AXIS2_PLACEMENT_3D('',#118404,#91206,#91207) ;
#73345=AXIS2_PLACEMENT_3D('',#118407,#91210,#91211) ;
#73346=AXIS2_PLACEMENT_3D('',#118413,#91215,#91216) ;
#73347=AXIS2_PLACEMENT_3D('',#118415,#91217,#91218) ;
#73348=AXIS2_PLACEMENT_3D('',#118418,#91220,#91221) ;
#73349=AXIS2_PLACEMENT_3D('',#118419,#91222,#91223) ;
#73350=AXIS2_PLACEMENT_3D('',#118425,#91227,#91228) ;
#73351=AXIS2_PLACEMENT_3D('',#118427,#91229,#91230) ;
#73352=AXIS2_PLACEMENT_3D('',#118430,#91232,#91233) ;
#73353=AXIS2_PLACEMENT_3D('',#118431,#91234,#91235) ;
#73354=AXIS2_PLACEMENT_3D('',#118437,#91239,#91240) ;
#73355=AXIS2_PLACEMENT_3D('',#118439,#91241,#91242) ;
#73356=AXIS2_PLACEMENT_3D('',#118442,#91244,#91245) ;
#73357=AXIS2_PLACEMENT_3D('',#118443,#91246,#91247) ;
#73358=AXIS2_PLACEMENT_3D('',#118449,#91251,#91252) ;
#73359=AXIS2_PLACEMENT_3D('',#118451,#91253,#91254) ;
#73360=AXIS2_PLACEMENT_3D('',#118454,#91256,#91257) ;
#73361=AXIS2_PLACEMENT_3D('',#118455,#91258,#91259) ;
#73362=AXIS2_PLACEMENT_3D('',#118461,#91263,#91264) ;
#73363=AXIS2_PLACEMENT_3D('',#118463,#91265,#91266) ;
#73364=AXIS2_PLACEMENT_3D('',#118466,#91268,#91269) ;
#73365=AXIS2_PLACEMENT_3D('',#118467,#91270,#91271) ;
#73366=AXIS2_PLACEMENT_3D('',#118473,#91275,#91276) ;
#73367=AXIS2_PLACEMENT_3D('',#118475,#91277,#91278) ;
#73368=AXIS2_PLACEMENT_3D('',#118478,#91280,#91281) ;
#73369=AXIS2_PLACEMENT_3D('',#118479,#91282,#91283) ;
#73370=AXIS2_PLACEMENT_3D('',#118481,#91284,#91285) ;
#73371=AXIS2_PLACEMENT_3D('',#118484,#91287,#91288) ;
#73372=AXIS2_PLACEMENT_3D('',#118485,#91289,#91290) ;
#73373=AXIS2_PLACEMENT_3D('',#118487,#91291,#91292) ;
#73374=AXIS2_PLACEMENT_3D('',#118490,#91294,#91295) ;
#73375=AXIS2_PLACEMENT_3D('',#118491,#91296,#91297) ;
#73376=AXIS2_PLACEMENT_3D('',#118497,#91301,#91302) ;
#73377=AXIS2_PLACEMENT_3D('',#118499,#91303,#91304) ;
#73378=AXIS2_PLACEMENT_3D('',#118502,#91306,#91307) ;
#73379=AXIS2_PLACEMENT_3D('',#118503,#91308,#91309) ;
#73380=AXIS2_PLACEMENT_3D('',#118509,#91313,#91314) ;
#73381=AXIS2_PLACEMENT_3D('',#118511,#91315,#91316) ;
#73382=AXIS2_PLACEMENT_3D('',#118514,#91318,#91319) ;
#73383=AXIS2_PLACEMENT_3D('',#118515,#91320,#91321) ;
#73384=AXIS2_PLACEMENT_3D('',#118518,#91324,#91325) ;
#73385=AXIS2_PLACEMENT_3D('',#118521,#91326,#91327) ;
#73386=AXIS2_PLACEMENT_3D('',#118525,#91329,#91330) ;
#73387=AXIS2_PLACEMENT_3D('',#118533,#91334,#91335) ;
#73388=AXIS2_PLACEMENT_3D('',#118541,#91339,#91340) ;
#73389=AXIS2_PLACEMENT_3D('',#118545,#91342,#91343) ;
#73390=AXIS2_PLACEMENT_3D('',#118554,#91349,#91350) ;
#73391=AXIS2_PLACEMENT_3D('',#118559,#91352,#91353) ;
#73392=AXIS2_PLACEMENT_3D('',#118562,#91355,#91356) ;
#73393=AXIS2_PLACEMENT_3D('',#118563,#91357,#91358) ;
#73394=AXIS2_PLACEMENT_3D('',#118569,#91362,#91363) ;
#73395=AXIS2_PLACEMENT_3D('',#118571,#91364,#91365) ;
#73396=AXIS2_PLACEMENT_3D('',#118574,#91367,#91368) ;
#73397=AXIS2_PLACEMENT_3D('',#118575,#91369,#91370) ;
#73398=AXIS2_PLACEMENT_3D('',#118581,#91374,#91375) ;
#73399=AXIS2_PLACEMENT_3D('',#118583,#91376,#91377) ;
#73400=AXIS2_PLACEMENT_3D('',#118586,#91379,#91380) ;
#73401=AXIS2_PLACEMENT_3D('',#118587,#91381,#91382) ;
#73402=AXIS2_PLACEMENT_3D('',#118592,#91386,#91387) ;
#73403=AXIS2_PLACEMENT_3D('',#118595,#91389,#91390) ;
#73404=AXIS2_PLACEMENT_3D('',#118596,#91391,#91392) ;
#73405=AXIS2_PLACEMENT_3D('',#118599,#91395,#91396) ;
#73406=AXIS2_PLACEMENT_3D('',#118605,#91400,#91401) ;
#73407=AXIS2_PLACEMENT_3D('',#118607,#91402,#91403) ;
#73408=AXIS2_PLACEMENT_3D('',#118610,#91405,#91406) ;
#73409=AXIS2_PLACEMENT_3D('',#118611,#91407,#91408) ;
#73410=AXIS2_PLACEMENT_3D('',#118617,#91412,#91413) ;
#73411=AXIS2_PLACEMENT_3D('',#118619,#91414,#91415) ;
#73412=AXIS2_PLACEMENT_3D('',#118622,#91417,#91418) ;
#73413=AXIS2_PLACEMENT_3D('',#118623,#91419,#91420) ;
#73414=AXIS2_PLACEMENT_3D('',#118629,#91424,#91425) ;
#73415=AXIS2_PLACEMENT_3D('',#118631,#91426,#91427) ;
#73416=AXIS2_PLACEMENT_3D('',#118634,#91429,#91430) ;
#73417=AXIS2_PLACEMENT_3D('',#118635,#91431,#91432) ;
#73418=AXIS2_PLACEMENT_3D('',#118641,#91436,#91437) ;
#73419=AXIS2_PLACEMENT_3D('',#118643,#91438,#91439) ;
#73420=AXIS2_PLACEMENT_3D('',#118646,#91441,#91442) ;
#73421=AXIS2_PLACEMENT_3D('',#118647,#91443,#91444) ;
#73422=AXIS2_PLACEMENT_3D('',#118653,#91448,#91449) ;
#73423=AXIS2_PLACEMENT_3D('',#118655,#91450,#91451) ;
#73424=AXIS2_PLACEMENT_3D('',#118658,#91453,#91454) ;
#73425=AXIS2_PLACEMENT_3D('',#118659,#91455,#91456) ;
#73426=AXIS2_PLACEMENT_3D('',#118665,#91460,#91461) ;
#73427=AXIS2_PLACEMENT_3D('',#118667,#91462,#91463) ;
#73428=AXIS2_PLACEMENT_3D('',#118670,#91465,#91466) ;
#73429=AXIS2_PLACEMENT_3D('',#118671,#91467,#91468) ;
#73430=AXIS2_PLACEMENT_3D('',#118673,#91469,#91470) ;
#73431=AXIS2_PLACEMENT_3D('',#118676,#91472,#91473) ;
#73432=AXIS2_PLACEMENT_3D('',#118677,#91474,#91475) ;
#73433=AXIS2_PLACEMENT_3D('',#118679,#91476,#91477) ;
#73434=AXIS2_PLACEMENT_3D('',#118682,#91479,#91480) ;
#73435=AXIS2_PLACEMENT_3D('',#118683,#91481,#91482) ;
#73436=AXIS2_PLACEMENT_3D('',#118689,#91486,#91487) ;
#73437=AXIS2_PLACEMENT_3D('',#118691,#91488,#91489) ;
#73438=AXIS2_PLACEMENT_3D('',#118694,#91491,#91492) ;
#73439=AXIS2_PLACEMENT_3D('',#118695,#91493,#91494) ;
#73440=AXIS2_PLACEMENT_3D('',#118701,#91498,#91499) ;
#73441=AXIS2_PLACEMENT_3D('',#118703,#91500,#91501) ;
#73442=AXIS2_PLACEMENT_3D('',#118706,#91503,#91504) ;
#73443=AXIS2_PLACEMENT_3D('',#118707,#91505,#91506) ;
#73444=AXIS2_PLACEMENT_3D('',#118710,#91509,#91510) ;
#73445=AXIS2_PLACEMENT_3D('',#118713,#91511,#91512) ;
#73446=AXIS2_PLACEMENT_3D('',#118717,#91514,#91515) ;
#73447=AXIS2_PLACEMENT_3D('',#118725,#91519,#91520) ;
#73448=AXIS2_PLACEMENT_3D('',#118733,#91524,#91525) ;
#73449=AXIS2_PLACEMENT_3D('',#118737,#91527,#91528) ;
#73450=AXIS2_PLACEMENT_3D('',#118746,#91534,#91535) ;
#73451=AXIS2_PLACEMENT_3D('',#118751,#91537,#91538) ;
#73452=AXIS2_PLACEMENT_3D('',#118754,#91540,#91541) ;
#73453=AXIS2_PLACEMENT_3D('',#118755,#91542,#91543) ;
#73454=AXIS2_PLACEMENT_3D('',#118761,#91547,#91548) ;
#73455=AXIS2_PLACEMENT_3D('',#118763,#91549,#91550) ;
#73456=AXIS2_PLACEMENT_3D('',#118766,#91552,#91553) ;
#73457=AXIS2_PLACEMENT_3D('',#118767,#91554,#91555) ;
#73458=AXIS2_PLACEMENT_3D('',#118773,#91559,#91560) ;
#73459=AXIS2_PLACEMENT_3D('',#118775,#91561,#91562) ;
#73460=AXIS2_PLACEMENT_3D('',#118778,#91564,#91565) ;
#73461=AXIS2_PLACEMENT_3D('',#118779,#91566,#91567) ;
#73462=AXIS2_PLACEMENT_3D('',#118784,#91571,#91572) ;
#73463=AXIS2_PLACEMENT_3D('',#118787,#91574,#91575) ;
#73464=AXIS2_PLACEMENT_3D('',#118788,#91576,#91577) ;
#73465=AXIS2_PLACEMENT_3D('',#118791,#91580,#91581) ;
#73466=AXIS2_PLACEMENT_3D('',#118797,#91585,#91586) ;
#73467=AXIS2_PLACEMENT_3D('',#118799,#91587,#91588) ;
#73468=AXIS2_PLACEMENT_3D('',#118802,#91590,#91591) ;
#73469=AXIS2_PLACEMENT_3D('',#118803,#91592,#91593) ;
#73470=AXIS2_PLACEMENT_3D('',#118809,#91597,#91598) ;
#73471=AXIS2_PLACEMENT_3D('',#118811,#91599,#91600) ;
#73472=AXIS2_PLACEMENT_3D('',#118814,#91602,#91603) ;
#73473=AXIS2_PLACEMENT_3D('',#118815,#91604,#91605) ;
#73474=AXIS2_PLACEMENT_3D('',#118821,#91609,#91610) ;
#73475=AXIS2_PLACEMENT_3D('',#118823,#91611,#91612) ;
#73476=AXIS2_PLACEMENT_3D('',#118826,#91614,#91615) ;
#73477=AXIS2_PLACEMENT_3D('',#118827,#91616,#91617) ;
#73478=AXIS2_PLACEMENT_3D('',#118833,#91621,#91622) ;
#73479=AXIS2_PLACEMENT_3D('',#118835,#91623,#91624) ;
#73480=AXIS2_PLACEMENT_3D('',#118838,#91626,#91627) ;
#73481=AXIS2_PLACEMENT_3D('',#118839,#91628,#91629) ;
#73482=AXIS2_PLACEMENT_3D('',#118845,#91633,#91634) ;
#73483=AXIS2_PLACEMENT_3D('',#118847,#91635,#91636) ;
#73484=AXIS2_PLACEMENT_3D('',#118850,#91638,#91639) ;
#73485=AXIS2_PLACEMENT_3D('',#118851,#91640,#91641) ;
#73486=AXIS2_PLACEMENT_3D('',#118857,#91645,#91646) ;
#73487=AXIS2_PLACEMENT_3D('',#118859,#91647,#91648) ;
#73488=AXIS2_PLACEMENT_3D('',#118862,#91650,#91651) ;
#73489=AXIS2_PLACEMENT_3D('',#118863,#91652,#91653) ;
#73490=AXIS2_PLACEMENT_3D('',#118865,#91654,#91655) ;
#73491=AXIS2_PLACEMENT_3D('',#118868,#91657,#91658) ;
#73492=AXIS2_PLACEMENT_3D('',#118869,#91659,#91660) ;
#73493=AXIS2_PLACEMENT_3D('',#118871,#91661,#91662) ;
#73494=AXIS2_PLACEMENT_3D('',#118874,#91664,#91665) ;
#73495=AXIS2_PLACEMENT_3D('',#118875,#91666,#91667) ;
#73496=AXIS2_PLACEMENT_3D('',#118881,#91671,#91672) ;
#73497=AXIS2_PLACEMENT_3D('',#118883,#91673,#91674) ;
#73498=AXIS2_PLACEMENT_3D('',#118886,#91676,#91677) ;
#73499=AXIS2_PLACEMENT_3D('',#118887,#91678,#91679) ;
#73500=AXIS2_PLACEMENT_3D('',#118893,#91683,#91684) ;
#73501=AXIS2_PLACEMENT_3D('',#118895,#91685,#91686) ;
#73502=AXIS2_PLACEMENT_3D('',#118898,#91688,#91689) ;
#73503=AXIS2_PLACEMENT_3D('',#118899,#91690,#91691) ;
#73504=AXIS2_PLACEMENT_3D('',#118902,#91694,#91695) ;
#73505=AXIS2_PLACEMENT_3D('',#118905,#91696,#91697) ;
#73506=AXIS2_PLACEMENT_3D('',#118909,#91699,#91700) ;
#73507=AXIS2_PLACEMENT_3D('',#118917,#91704,#91705) ;
#73508=AXIS2_PLACEMENT_3D('',#118925,#91709,#91710) ;
#73509=AXIS2_PLACEMENT_3D('',#118929,#91712,#91713) ;
#73510=AXIS2_PLACEMENT_3D('',#118938,#91719,#91720) ;
#73511=AXIS2_PLACEMENT_3D('',#118943,#91722,#91723) ;
#73512=AXIS2_PLACEMENT_3D('',#118947,#91725,#91726) ;
#73513=AXIS2_PLACEMENT_3D('',#118951,#91728,#91729) ;
#73514=AXIS2_PLACEMENT_3D('',#118954,#91731,#91732) ;
#73515=AXIS2_PLACEMENT_3D('',#118955,#91733,#91734) ;
#73516=AXIS2_PLACEMENT_3D('',#118960,#91736,#91737) ;
#73517=AXIS2_PLACEMENT_3D('',#118964,#91739,#91740) ;
#73518=AXIS2_PLACEMENT_3D('',#118968,#91742,#91743) ;
#73519=AXIS2_PLACEMENT_3D('',#118971,#91745,#91746) ;
#73520=AXIS2_PLACEMENT_3D('',#118972,#91747,#91748) ;
#73521=AXIS2_PLACEMENT_3D('',#118977,#91750,#91751) ;
#73522=AXIS2_PLACEMENT_3D('',#118981,#91753,#91754) ;
#73523=AXIS2_PLACEMENT_3D('',#118985,#91756,#91757) ;
#73524=AXIS2_PLACEMENT_3D('',#118988,#91759,#91760) ;
#73525=AXIS2_PLACEMENT_3D('',#118989,#91761,#91762) ;
#73526=AXIS2_PLACEMENT_3D('',#118994,#91764,#91765) ;
#73527=AXIS2_PLACEMENT_3D('',#118998,#91767,#91768) ;
#73528=AXIS2_PLACEMENT_3D('',#119002,#91770,#91771) ;
#73529=AXIS2_PLACEMENT_3D('',#119005,#91773,#91774) ;
#73530=AXIS2_PLACEMENT_3D('',#119006,#91775,#91776) ;
#73531=AXIS2_PLACEMENT_3D('',#119011,#91778,#91779) ;
#73532=AXIS2_PLACEMENT_3D('',#119015,#91781,#91782) ;
#73533=AXIS2_PLACEMENT_3D('',#119019,#91784,#91785) ;
#73534=AXIS2_PLACEMENT_3D('',#119022,#91787,#91788) ;
#73535=AXIS2_PLACEMENT_3D('',#119023,#91789,#91790) ;
#73536=AXIS2_PLACEMENT_3D('',#119028,#91792,#91793) ;
#73537=AXIS2_PLACEMENT_3D('',#119032,#91795,#91796) ;
#73538=AXIS2_PLACEMENT_3D('',#119036,#91798,#91799) ;
#73539=AXIS2_PLACEMENT_3D('',#119039,#91801,#91802) ;
#73540=AXIS2_PLACEMENT_3D('',#119040,#91803,#91804) ;
#73541=AXIS2_PLACEMENT_3D('',#119045,#91806,#91807) ;
#73542=AXIS2_PLACEMENT_3D('',#119049,#91809,#91810) ;
#73543=AXIS2_PLACEMENT_3D('',#119053,#91812,#91813) ;
#73544=AXIS2_PLACEMENT_3D('',#119056,#91815,#91816) ;
#73545=AXIS2_PLACEMENT_3D('',#119057,#91817,#91818) ;
#73546=AXIS2_PLACEMENT_3D('',#119062,#91820,#91821) ;
#73547=AXIS2_PLACEMENT_3D('',#119066,#91823,#91824) ;
#73548=AXIS2_PLACEMENT_3D('',#119070,#91826,#91827) ;
#73549=AXIS2_PLACEMENT_3D('',#119073,#91829,#91830) ;
#73550=AXIS2_PLACEMENT_3D('',#119074,#91831,#91832) ;
#73551=AXIS2_PLACEMENT_3D('',#119079,#91834,#91835) ;
#73552=AXIS2_PLACEMENT_3D('',#119083,#91837,#91838) ;
#73553=AXIS2_PLACEMENT_3D('',#119087,#91840,#91841) ;
#73554=AXIS2_PLACEMENT_3D('',#119090,#91843,#91844) ;
#73555=AXIS2_PLACEMENT_3D('',#119091,#91845,#91846) ;
#73556=AXIS2_PLACEMENT_3D('',#119092,#91847,#91848) ;
#73557=AXIS2_PLACEMENT_3D('',#119093,#91849,#91850) ;
#73558=AXIS2_PLACEMENT_3D('',#119094,#91851,#91852) ;
#73559=AXIS2_PLACEMENT_3D('',#119095,#91853,#91854) ;
#73560=AXIS2_PLACEMENT_3D('',#119096,#91855,#91856) ;
#73561=AXIS2_PLACEMENT_3D('',#119097,#91857,#91858) ;
#73562=AXIS2_PLACEMENT_3D('',#119099,#91859,#91860) ;
#73563=AXIS2_PLACEMENT_3D('',#119100,#91861,#91862) ;
#73564=AXIS2_PLACEMENT_3D('',#119101,#91863,#91864) ;
#73565=AXIS2_PLACEMENT_3D('',#119102,#91865,#91866) ;
#73566=AXIS2_PLACEMENT_3D('',#119103,#91867,#91868) ;
#73567=AXIS2_PLACEMENT_3D('',#119104,#91869,#91870) ;
#73568=AXIS2_PLACEMENT_3D('',#119105,#91871,#91872) ;
#73569=AXIS2_PLACEMENT_3D('',#119106,#91873,#91874) ;
#73570=AXIS2_PLACEMENT_3D('',#119107,#91875,#91876) ;
#73571=AXIS2_PLACEMENT_3D('',#119118,#91878,#91879) ;
#73572=AXIS2_PLACEMENT_3D('',#119175,#91881,#91882) ;
#73573=AXIS2_PLACEMENT_3D('',#119176,#91883,#91884) ;
#73574=AXIS2_PLACEMENT_3D('',#119177,#91885,#91886) ;
#73575=AXIS2_PLACEMENT_3D('',#119178,#91887,#91888) ;
#73576=AXIS2_PLACEMENT_3D('',#119179,#91889,#91890) ;
#73577=AXIS2_PLACEMENT_3D('',#119180,#91891,#91892) ;
#73578=AXIS2_PLACEMENT_3D('',#119181,#91893,#91894) ;
#73579=AXIS2_PLACEMENT_3D('',#119182,#91895,#91896) ;
#73580=AXIS2_PLACEMENT_3D('',#119183,#91897,#91898) ;
#73581=AXIS2_PLACEMENT_3D('',#119184,#91899,#91900) ;
#73582=AXIS2_PLACEMENT_3D('',#119185,#91901,#91902) ;
#73583=AXIS2_PLACEMENT_3D('',#119186,#91903,#91904) ;
#73584=AXIS2_PLACEMENT_3D('',#119187,#91905,#91906) ;
#73585=AXIS2_PLACEMENT_3D('',#119188,#91907,#91908) ;
#73586=AXIS2_PLACEMENT_3D('',#119189,#91909,#91910) ;
#73587=AXIS2_PLACEMENT_3D('',#119190,#91911,#91912) ;
#73588=AXIS2_PLACEMENT_3D('',#119191,#91913,#91914) ;
#73589=AXIS2_PLACEMENT_3D('',#119192,#91915,#91916) ;
#73590=AXIS2_PLACEMENT_3D('',#119193,#91917,#91918) ;
#73591=AXIS2_PLACEMENT_3D('',#119194,#91919,#91920) ;
#73592=AXIS2_PLACEMENT_3D('',#119195,#91921,#91922) ;
#73593=AXIS2_PLACEMENT_3D('',#119196,#91923,#91924) ;
#73594=AXIS2_PLACEMENT_3D('',#119197,#91925,#91926) ;
#73595=AXIS2_PLACEMENT_3D('',#119200,#91928,#91929) ;
#73596=AXIS2_PLACEMENT_3D('',#119201,#91930,#91931) ;
#73597=AXIS2_PLACEMENT_3D('',#119202,#91932,#91933) ;
#73598=AXIS2_PLACEMENT_3D('',#119203,#91934,#91935) ;
#73599=AXIS2_PLACEMENT_3D('',#119204,#91936,#91937) ;
#73600=AXIS2_PLACEMENT_3D('',#119205,#91938,#91939) ;
#73601=AXIS2_PLACEMENT_3D('',#119206,#91940,#91941) ;
#73602=AXIS2_PLACEMENT_3D('',#119207,#91942,#91943) ;
#73603=AXIS2_PLACEMENT_3D('',#119208,#91944,#91945) ;
#73604=AXIS2_PLACEMENT_3D('',#119209,#91946,#91947) ;
#73605=AXIS2_PLACEMENT_3D('',#119210,#91948,#91949) ;
#73606=AXIS2_PLACEMENT_3D('',#119211,#91950,#91951) ;
#73607=AXIS2_PLACEMENT_3D('',#119212,#91952,#91953) ;
#73608=AXIS2_PLACEMENT_3D('',#119213,#91954,#91955) ;
#73609=AXIS2_PLACEMENT_3D('',#119214,#91956,#91957) ;
#73610=AXIS2_PLACEMENT_3D('',#119215,#91958,#91959) ;
#73611=AXIS2_PLACEMENT_3D('',#119217,#91960,#91961) ;
#73612=AXIS2_PLACEMENT_3D('',#119218,#91962,#91963) ;
#73613=AXIS2_PLACEMENT_3D('',#119219,#91964,#91965) ;
#73614=AXIS2_PLACEMENT_3D('',#119220,#91966,#91967) ;
#73615=AXIS2_PLACEMENT_3D('',#119221,#91968,#91969) ;
#73616=AXIS2_PLACEMENT_3D('',#119222,#91970,#91971) ;
#73617=AXIS2_PLACEMENT_3D('',#119223,#91972,#91973) ;
#73618=AXIS2_PLACEMENT_3D('',#119224,#91974,#91975) ;
#73619=AXIS2_PLACEMENT_3D('',#119225,#91976,#91977) ;
#73620=AXIS2_PLACEMENT_3D('',#119226,#91978,#91979) ;
#73621=AXIS2_PLACEMENT_3D('',#119227,#91980,#91981) ;
#73622=AXIS2_PLACEMENT_3D('',#119228,#91982,#91983) ;
#73623=AXIS2_PLACEMENT_3D('',#119229,#91984,#91985) ;
#73624=AXIS2_PLACEMENT_3D('',#119232,#91987,#91988) ;
#73625=AXIS2_PLACEMENT_3D('',#119233,#91989,#91990) ;
#73626=AXIS2_PLACEMENT_3D('',#119234,#91991,#91992) ;
#73627=AXIS2_PLACEMENT_3D('',#119235,#91993,#91994) ;
#73628=AXIS2_PLACEMENT_3D('',#119236,#91995,#91996) ;
#73629=AXIS2_PLACEMENT_3D('',#119237,#91997,#91998) ;
#73630=AXIS2_PLACEMENT_3D('',#119238,#91999,#92000) ;
#73631=AXIS2_PLACEMENT_3D('',#119239,#92001,#92002) ;
#73632=AXIS2_PLACEMENT_3D('',#119240,#92003,#92004) ;
#73633=AXIS2_PLACEMENT_3D('',#119241,#92005,#92006) ;
#73634=AXIS2_PLACEMENT_3D('',#119242,#92007,#92008) ;
#73635=AXIS2_PLACEMENT_3D('',#119243,#92009,#92010) ;
#73636=AXIS2_PLACEMENT_3D('',#119244,#92011,#92012) ;
#73637=AXIS2_PLACEMENT_3D('',#119246,#92013,#92014) ;
#73638=AXIS2_PLACEMENT_3D('',#119247,#92015,#92016) ;
#73639=AXIS2_PLACEMENT_3D('',#119248,#92017,#92018) ;
#73640=AXIS2_PLACEMENT_3D('',#119249,#92019,#92020) ;
#73641=AXIS2_PLACEMENT_3D('',#119250,#92021,#92022) ;
#73642=AXIS2_PLACEMENT_3D('',#119251,#92023,#92024) ;
#73643=AXIS2_PLACEMENT_3D('',#119252,#92025,#92026) ;
#73644=AXIS2_PLACEMENT_3D('',#119253,#92027,#92028) ;
#73645=AXIS2_PLACEMENT_3D('',#119254,#92029,#92030) ;
#73646=AXIS2_PLACEMENT_3D('',#119255,#92031,#92032) ;
#73647=AXIS2_PLACEMENT_3D('',#119256,#92033,#92034) ;
#73648=AXIS2_PLACEMENT_3D('',#119258,#92036,#92037) ;
#73649=AXIS2_PLACEMENT_3D('',#119259,#92038,#92039) ;
#73650=AXIS2_PLACEMENT_3D('',#119260,#92040,#92041) ;
#73651=AXIS2_PLACEMENT_3D('',#119261,#92042,#92043) ;
#73652=AXIS2_PLACEMENT_3D('',#119262,#92044,#92045) ;
#73653=AXIS2_PLACEMENT_3D('',#119263,#92046,#92047) ;
#73654=AXIS2_PLACEMENT_3D('',#119264,#92048,#92049) ;
#73655=AXIS2_PLACEMENT_3D('',#119265,#92050,#92051) ;
#73656=AXIS2_PLACEMENT_3D('',#119266,#92052,#92053) ;
#73657=AXIS2_PLACEMENT_3D('',#119267,#92054,#92055) ;
#73658=AXIS2_PLACEMENT_3D('',#119268,#92056,#92057) ;
#73659=AXIS2_PLACEMENT_3D('',#119269,#92058,#92059) ;
#73660=AXIS2_PLACEMENT_3D('',#119270,#92060,#92061) ;
#73661=AXIS2_PLACEMENT_3D('',#119271,#92062,#92063) ;
#73662=AXIS2_PLACEMENT_3D('',#119272,#92064,#92065) ;
#73663=AXIS2_PLACEMENT_3D('',#119273,#92066,#92067) ;
#73664=AXIS2_PLACEMENT_3D('',#119274,#92068,#92069) ;
#73665=AXIS2_PLACEMENT_3D('',#119275,#92070,#92071) ;
#73666=AXIS2_PLACEMENT_3D('',#119276,#92072,#92073) ;
#73667=AXIS2_PLACEMENT_3D('',#119277,#92074,#92075) ;
#73668=AXIS2_PLACEMENT_3D('',#119278,#92076,#92077) ;
#73669=AXIS2_PLACEMENT_3D('',#119279,#92078,#92079) ;
#73670=AXIS2_PLACEMENT_3D('',#119280,#92080,#92081) ;
#73671=AXIS2_PLACEMENT_3D('',#119281,#92082,#92083) ;
#73672=AXIS2_PLACEMENT_3D('',#119282,#92084,#92085) ;
#73673=AXIS2_PLACEMENT_3D('',#119283,#92086,#92087) ;
#73674=AXIS2_PLACEMENT_3D('',#119284,#92088,#92089) ;
#73675=AXIS2_PLACEMENT_3D('',#119285,#92090,#92091) ;
#73676=AXIS2_PLACEMENT_3D('',#119286,#92092,#92093) ;
#73677=AXIS2_PLACEMENT_3D('',#119287,#92094,#92095) ;
#73678=AXIS2_PLACEMENT_3D('',#119288,#92096,#92097) ;
#73679=AXIS2_PLACEMENT_3D('',#119289,#92098,#92099) ;
#73680=AXIS2_PLACEMENT_3D('',#119290,#92100,#92101) ;
#73681=AXIS2_PLACEMENT_3D('',#119291,#92102,#92103) ;
#73682=AXIS2_PLACEMENT_3D('',#119292,#92104,#92105) ;
#73683=AXIS2_PLACEMENT_3D('',#119293,#92106,#92107) ;
#73684=AXIS2_PLACEMENT_3D('',#119294,#92108,#92109) ;
#73685=AXIS2_PLACEMENT_3D('',#119295,#92110,#92111) ;
#73686=AXIS2_PLACEMENT_3D('',#119296,#92112,#92113) ;
#73687=AXIS2_PLACEMENT_3D('',#119297,#92114,#92115) ;
#73688=AXIS2_PLACEMENT_3D('',#119298,#92116,#92117) ;
#73689=AXIS2_PLACEMENT_3D('',#119299,#92118,#92119) ;
#73690=AXIS2_PLACEMENT_3D('',#119300,#92120,#92121) ;
#73691=AXIS2_PLACEMENT_3D('',#119301,#92122,#92123) ;
#73692=AXIS2_PLACEMENT_3D('',#119302,#92124,#92125) ;
#73693=AXIS2_PLACEMENT_3D('',#119303,#92126,#92127) ;
#73694=AXIS2_PLACEMENT_3D('',#119304,#92128,#92129) ;
#73695=AXIS2_PLACEMENT_3D('',#119305,#92130,#92131) ;
#73696=AXIS2_PLACEMENT_3D('',#119306,#92132,#92133) ;
#73697=AXIS2_PLACEMENT_3D('',#119307,#92134,#92135) ;
#73698=AXIS2_PLACEMENT_3D('',#119308,#92136,#92137) ;
#73699=AXIS2_PLACEMENT_3D('',#119309,#92138,#92139) ;
#73700=AXIS2_PLACEMENT_3D('',#119310,#92140,#92141) ;
#73701=AXIS2_PLACEMENT_3D('',#119311,#92142,#92143) ;
#73702=AXIS2_PLACEMENT_3D('',#119312,#92144,#92145) ;
#73703=AXIS2_PLACEMENT_3D('',#119313,#92146,#92147) ;
#73704=AXIS2_PLACEMENT_3D('',#119314,#92148,#92149) ;
#73705=AXIS2_PLACEMENT_3D('',#119315,#92150,#92151) ;
#73706=AXIS2_PLACEMENT_3D('',#119316,#92152,#92153) ;
#73707=AXIS2_PLACEMENT_3D('',#119317,#92154,#92155) ;
#73708=AXIS2_PLACEMENT_3D('',#119318,#92156,#92157) ;
#73709=AXIS2_PLACEMENT_3D('',#119319,#92158,#92159) ;
#73710=AXIS2_PLACEMENT_3D('',#119320,#92160,#92161) ;
#73711=AXIS2_PLACEMENT_3D('',#119321,#92162,#92163) ;
#73712=AXIS2_PLACEMENT_3D('',#119322,#92164,#92165) ;
#73713=AXIS2_PLACEMENT_3D('',#119323,#92166,#92167) ;
#73714=AXIS2_PLACEMENT_3D('',#119324,#92168,#92169) ;
#73715=AXIS2_PLACEMENT_3D('',#119325,#92170,#92171) ;
#73716=AXIS2_PLACEMENT_3D('',#119326,#92172,#92173) ;
#73717=AXIS2_PLACEMENT_3D('',#119327,#92174,#92175) ;
#73718=AXIS2_PLACEMENT_3D('',#119328,#92176,#92177) ;
#73719=AXIS2_PLACEMENT_3D('',#119329,#92178,#92179) ;
#73720=AXIS2_PLACEMENT_3D('',#119330,#92180,#92181) ;
#73721=AXIS2_PLACEMENT_3D('',#119331,#92182,#92183) ;
#73722=AXIS2_PLACEMENT_3D('',#119332,#92184,#92185) ;
#73723=AXIS2_PLACEMENT_3D('',#119333,#92186,#92187) ;
#73724=AXIS2_PLACEMENT_3D('',#119334,#92188,#92189) ;
#73725=AXIS2_PLACEMENT_3D('',#119335,#92190,#92191) ;
#73726=AXIS2_PLACEMENT_3D('',#119336,#92192,#92193) ;
#73727=AXIS2_PLACEMENT_3D('',#119337,#92194,#92195) ;
#73728=AXIS2_PLACEMENT_3D('',#119338,#92196,#92197) ;
#73729=AXIS2_PLACEMENT_3D('',#119339,#92198,#92199) ;
#73730=AXIS2_PLACEMENT_3D('',#119340,#92200,#92201) ;
#73731=AXIS2_PLACEMENT_3D('',#119341,#92202,#92203) ;
#73732=AXIS2_PLACEMENT_3D('',#119342,#92204,#92205) ;
#73733=AXIS2_PLACEMENT_3D('',#119343,#92206,#92207) ;
#73734=AXIS2_PLACEMENT_3D('',#119344,#92208,#92209) ;
#73735=AXIS2_PLACEMENT_3D('',#119345,#92210,#92211) ;
#73736=AXIS2_PLACEMENT_3D('',#119346,#92212,#92213) ;
#73737=AXIS2_PLACEMENT_3D('',#119347,#92214,#92215) ;
#73738=AXIS2_PLACEMENT_3D('',#119348,#92216,#92217) ;
#73739=AXIS2_PLACEMENT_3D('',#119349,#92218,#92219) ;
#73740=AXIS2_PLACEMENT_3D('',#119350,#92220,#92221) ;
#73741=AXIS2_PLACEMENT_3D('',#119351,#92222,#92223) ;
#73742=AXIS2_PLACEMENT_3D('',#119352,#92224,#92225) ;
#73743=AXIS2_PLACEMENT_3D('',#119353,#92226,#92227) ;
#73744=AXIS2_PLACEMENT_3D('',#119354,#92228,#92229) ;
#73745=AXIS2_PLACEMENT_3D('',#119355,#92230,#92231) ;
#73746=AXIS2_PLACEMENT_3D('',#119356,#92232,#92233) ;
#73747=AXIS2_PLACEMENT_3D('',#119357,#92234,#92235) ;
#73748=AXIS2_PLACEMENT_3D('',#119358,#92236,#92237) ;
#73749=AXIS2_PLACEMENT_3D('',#119359,#92238,#92239) ;
#73750=AXIS2_PLACEMENT_3D('',#119360,#92240,#92241) ;
#73751=AXIS2_PLACEMENT_3D('',#119361,#92242,#92243) ;
#73752=AXIS2_PLACEMENT_3D('',#119362,#92244,#92245) ;
#73753=AXIS2_PLACEMENT_3D('',#119363,#92246,#92247) ;
#73754=AXIS2_PLACEMENT_3D('',#119364,#92248,#92249) ;
#73755=AXIS2_PLACEMENT_3D('',#119365,#92250,#92251) ;
#73756=AXIS2_PLACEMENT_3D('',#119366,#92252,#92253) ;
#73757=AXIS2_PLACEMENT_3D('',#119367,#92254,#92255) ;
#73758=AXIS2_PLACEMENT_3D('',#119368,#92256,#92257) ;
#73759=AXIS2_PLACEMENT_3D('',#119369,#92258,#92259) ;
#73760=AXIS2_PLACEMENT_3D('',#119370,#92260,#92261) ;
#73761=AXIS2_PLACEMENT_3D('',#119371,#92262,#92263) ;
#73762=AXIS2_PLACEMENT_3D('',#119372,#92264,#92265) ;
#73763=AXIS2_PLACEMENT_3D('',#119373,#92266,#92267) ;
#73764=AXIS2_PLACEMENT_3D('',#119374,#92268,#92269) ;
#73765=AXIS2_PLACEMENT_3D('',#119375,#92270,#92271) ;
#73766=AXIS2_PLACEMENT_3D('',#119376,#92272,#92273) ;
#73767=AXIS2_PLACEMENT_3D('',#119377,#92274,#92275) ;
#73768=AXIS2_PLACEMENT_3D('',#119378,#92276,#92277) ;
#73769=AXIS2_PLACEMENT_3D('',#119379,#92278,#92279) ;
#73770=AXIS2_PLACEMENT_3D('',#119380,#92280,#92281) ;
#73771=AXIS2_PLACEMENT_3D('',#119381,#92282,#92283) ;
#73772=AXIS2_PLACEMENT_3D('',#119382,#92284,#92285) ;
#73773=AXIS2_PLACEMENT_3D('',#119383,#92286,#92287) ;
#73774=AXIS2_PLACEMENT_3D('',#119384,#92288,#92289) ;
#73775=AXIS2_PLACEMENT_3D('',#119385,#92290,#92291) ;
#73776=AXIS2_PLACEMENT_3D('',#119386,#92292,#92293) ;
#73777=AXIS2_PLACEMENT_3D('',#119387,#92294,#92295) ;
#73778=AXIS2_PLACEMENT_3D('',#119388,#92296,#92297) ;
#73779=AXIS2_PLACEMENT_3D('',#119389,#92298,#92299) ;
#73780=AXIS2_PLACEMENT_3D('',#119390,#92300,#92301) ;
#73781=AXIS2_PLACEMENT_3D('',#119391,#92302,#92303) ;
#73782=AXIS2_PLACEMENT_3D('',#119392,#92304,#92305) ;
#73783=AXIS2_PLACEMENT_3D('',#119393,#92306,#92307) ;
#73784=AXIS2_PLACEMENT_3D('',#119394,#92308,#92309) ;
#73785=AXIS2_PLACEMENT_3D('',#119395,#92310,#92311) ;
#73786=AXIS2_PLACEMENT_3D('',#119396,#92312,#92313) ;
#73787=AXIS2_PLACEMENT_3D('',#119397,#92314,#92315) ;
#73788=AXIS2_PLACEMENT_3D('',#119398,#92316,#92317) ;
#73789=AXIS2_PLACEMENT_3D('',#119399,#92318,#92319) ;
#73790=AXIS2_PLACEMENT_3D('',#119400,#92320,#92321) ;
#73791=AXIS2_PLACEMENT_3D('',#119401,#92322,#92323) ;
#73792=AXIS2_PLACEMENT_3D('',#119402,#92324,#92325) ;
#73793=AXIS2_PLACEMENT_3D('',#119403,#92326,#92327) ;
#73794=AXIS2_PLACEMENT_3D('',#119404,#92328,#92329) ;
#73795=AXIS2_PLACEMENT_3D('',#119405,#92330,#92331) ;
#73796=AXIS2_PLACEMENT_3D('',#119406,#92332,#92333) ;
#73797=AXIS2_PLACEMENT_3D('',#119407,#92334,#92335) ;
#73798=AXIS2_PLACEMENT_3D('',#119408,#92336,#92337) ;
#73799=AXIS2_PLACEMENT_3D('',#119409,#92338,#92339) ;
#73800=AXIS2_PLACEMENT_3D('',#119410,#92340,#92341) ;
#73801=AXIS2_PLACEMENT_3D('',#119411,#92342,#92343) ;
#73802=AXIS2_PLACEMENT_3D('',#119412,#92344,#92345) ;
#73803=AXIS2_PLACEMENT_3D('',#119413,#92346,#92347) ;
#73804=AXIS2_PLACEMENT_3D('',#119414,#92348,#92349) ;
#73805=AXIS2_PLACEMENT_3D('',#119415,#92350,#92351) ;
#73806=AXIS2_PLACEMENT_3D('',#119416,#92352,#92353) ;
#73807=AXIS2_PLACEMENT_3D('',#119417,#92354,#92355) ;
#73808=AXIS2_PLACEMENT_3D('',#119418,#92356,#92357) ;
#73809=AXIS2_PLACEMENT_3D('',#119419,#92358,#92359) ;
#73810=AXIS2_PLACEMENT_3D('',#119420,#92360,#92361) ;
#73811=AXIS2_PLACEMENT_3D('',#119421,#92362,#92363) ;
#73812=AXIS2_PLACEMENT_3D('',#119422,#92364,#92365) ;
#73813=AXIS2_PLACEMENT_3D('',#119423,#92366,#92367) ;
#73814=AXIS2_PLACEMENT_3D('',#119424,#92368,#92369) ;
#73815=AXIS2_PLACEMENT_3D('',#119425,#92370,#92371) ;
#73816=AXIS2_PLACEMENT_3D('',#119426,#92372,#92373) ;
#73817=AXIS2_PLACEMENT_3D('',#119427,#92374,#92375) ;
#73818=AXIS2_PLACEMENT_3D('',#119428,#92376,#92377) ;
#73819=AXIS2_PLACEMENT_3D('',#119429,#92378,#92379) ;
#73820=AXIS2_PLACEMENT_3D('',#119430,#92380,#92381) ;
#73821=AXIS2_PLACEMENT_3D('',#119431,#92382,#92383) ;
#73822=AXIS2_PLACEMENT_3D('',#119432,#92384,#92385) ;
#73823=AXIS2_PLACEMENT_3D('',#119433,#92386,#92387) ;
#73824=AXIS2_PLACEMENT_3D('',#119434,#92388,#92389) ;
#73825=AXIS2_PLACEMENT_3D('',#119435,#92390,#92391) ;
#73826=AXIS2_PLACEMENT_3D('',#119436,#92392,#92393) ;
#73827=AXIS2_PLACEMENT_3D('',#119437,#92394,#92395) ;
#73828=AXIS2_PLACEMENT_3D('',#119438,#92396,#92397) ;
#73829=AXIS2_PLACEMENT_3D('',#119439,#92398,#92399) ;
#73830=AXIS2_PLACEMENT_3D('',#119440,#92400,#92401) ;
#73831=AXIS2_PLACEMENT_3D('',#119441,#92402,#92403) ;
#73832=AXIS2_PLACEMENT_3D('',#119442,#92404,#92405) ;
#73833=AXIS2_PLACEMENT_3D('',#119443,#92406,#92407) ;
#73834=AXIS2_PLACEMENT_3D('',#119444,#92408,#92409) ;
#73835=AXIS2_PLACEMENT_3D('',#119445,#92410,#92411) ;
#73836=AXIS2_PLACEMENT_3D('',#119446,#92412,#92413) ;
#73837=AXIS2_PLACEMENT_3D('',#119447,#92414,#92415) ;
#73838=AXIS2_PLACEMENT_3D('',#119448,#92416,#92417) ;
#73839=AXIS2_PLACEMENT_3D('',#119449,#92418,#92419) ;
#73840=AXIS2_PLACEMENT_3D('',#119450,#92420,#92421) ;
#73841=AXIS2_PLACEMENT_3D('',#119451,#92422,#92423) ;
#73842=AXIS2_PLACEMENT_3D('',#119452,#92424,#92425) ;
#73843=AXIS2_PLACEMENT_3D('',#119453,#92426,#92427) ;
#73844=AXIS2_PLACEMENT_3D('',#119454,#92428,#92429) ;
#73845=AXIS2_PLACEMENT_3D('',#119455,#92430,#92431) ;
#73846=AXIS2_PLACEMENT_3D('',#119456,#92432,#92433) ;
#73847=AXIS2_PLACEMENT_3D('',#119457,#92434,#92435) ;
#73848=AXIS2_PLACEMENT_3D('',#119458,#92436,#92437) ;
#73849=AXIS2_PLACEMENT_3D('',#119459,#92438,#92439) ;
#73850=AXIS2_PLACEMENT_3D('',#119460,#92440,#92441) ;
#73851=AXIS2_PLACEMENT_3D('',#119461,#92442,#92443) ;
#73852=AXIS2_PLACEMENT_3D('',#119462,#92444,#92445) ;
#73853=AXIS2_PLACEMENT_3D('',#119463,#92446,#92447) ;
#73854=AXIS2_PLACEMENT_3D('',#119464,#92448,#92449) ;
#73855=AXIS2_PLACEMENT_3D('',#119465,#92450,#92451) ;
#73856=AXIS2_PLACEMENT_3D('',#119466,#92452,#92453) ;
#73857=AXIS2_PLACEMENT_3D('',#119467,#92454,#92455) ;
#73858=AXIS2_PLACEMENT_3D('',#119468,#92456,#92457) ;
#73859=AXIS2_PLACEMENT_3D('',#119469,#92458,#92459) ;
#73860=AXIS2_PLACEMENT_3D('',#119470,#92460,#92461) ;
#73861=AXIS2_PLACEMENT_3D('',#119471,#92462,#92463) ;
#73862=AXIS2_PLACEMENT_3D('',#119472,#92464,#92465) ;
#73863=AXIS2_PLACEMENT_3D('',#119473,#92466,#92467) ;
#73864=AXIS2_PLACEMENT_3D('',#119474,#92468,#92469) ;
#73865=AXIS2_PLACEMENT_3D('',#119475,#92470,#92471) ;
#73866=AXIS2_PLACEMENT_3D('',#119476,#92472,#92473) ;
#73867=AXIS2_PLACEMENT_3D('',#119477,#92474,#92475) ;
#73868=AXIS2_PLACEMENT_3D('',#119478,#92476,#92477) ;
#73869=AXIS2_PLACEMENT_3D('',#119479,#92478,#92479) ;
#73870=AXIS2_PLACEMENT_3D('',#119480,#92480,#92481) ;
#73871=AXIS2_PLACEMENT_3D('',#119481,#92482,#92483) ;
#73872=AXIS2_PLACEMENT_3D('',#119482,#92484,#92485) ;
#73873=AXIS2_PLACEMENT_3D('',#119483,#92486,#92487) ;
#73874=AXIS2_PLACEMENT_3D('',#119484,#92488,#92489) ;
#73875=AXIS2_PLACEMENT_3D('',#119485,#92490,#92491) ;
#73876=AXIS2_PLACEMENT_3D('',#119486,#92492,#92493) ;
#73877=AXIS2_PLACEMENT_3D('',#119487,#92494,#92495) ;
#73878=AXIS2_PLACEMENT_3D('',#119488,#92496,#92497) ;
#73879=AXIS2_PLACEMENT_3D('',#119489,#92498,#92499) ;
#73880=AXIS2_PLACEMENT_3D('',#119490,#92500,#92501) ;
#73881=AXIS2_PLACEMENT_3D('',#119491,#92502,#92503) ;
#73882=AXIS2_PLACEMENT_3D('',#119492,#92504,#92505) ;
#73883=AXIS2_PLACEMENT_3D('',#119493,#92506,#92507) ;
#73884=AXIS2_PLACEMENT_3D('',#119494,#92508,#92509) ;
#73885=AXIS2_PLACEMENT_3D('',#119495,#92510,#92511) ;
#73886=AXIS2_PLACEMENT_3D('',#119496,#92512,#92513) ;
#73887=AXIS2_PLACEMENT_3D('',#119497,#92514,#92515) ;
#73888=AXIS2_PLACEMENT_3D('',#119498,#92516,#92517) ;
#73889=AXIS2_PLACEMENT_3D('',#119499,#92518,#92519) ;
#73890=AXIS2_PLACEMENT_3D('',#119500,#92520,#92521) ;
#73891=AXIS2_PLACEMENT_3D('',#119501,#92522,#92523) ;
#73892=AXIS2_PLACEMENT_3D('',#119502,#92524,#92525) ;
#73893=AXIS2_PLACEMENT_3D('',#119503,#92526,#92527) ;
#73894=AXIS2_PLACEMENT_3D('',#119504,#92528,#92529) ;
#73895=AXIS2_PLACEMENT_3D('',#119505,#92530,#92531) ;
#73896=AXIS2_PLACEMENT_3D('',#119506,#92532,#92533) ;
#73897=AXIS2_PLACEMENT_3D('',#119507,#92534,#92535) ;
#73898=AXIS2_PLACEMENT_3D('',#119508,#92536,#92537) ;
#73899=AXIS2_PLACEMENT_3D('',#119509,#92538,#92539) ;
#73900=AXIS2_PLACEMENT_3D('',#119510,#92540,#92541) ;
#73901=AXIS2_PLACEMENT_3D('',#119511,#92542,#92543) ;
#73902=AXIS2_PLACEMENT_3D('',#119512,#92544,#92545) ;
#73903=AXIS2_PLACEMENT_3D('',#119513,#92546,#92547) ;
#73904=AXIS2_PLACEMENT_3D('',#119514,#92548,#92549) ;
#73905=AXIS2_PLACEMENT_3D('',#119515,#92550,#92551) ;
#73906=AXIS2_PLACEMENT_3D('',#119516,#92552,#92553) ;
#73907=AXIS2_PLACEMENT_3D('',#119517,#92554,#92555) ;
#73908=AXIS2_PLACEMENT_3D('',#119518,#92556,#92557) ;
#73909=AXIS2_PLACEMENT_3D('',#119519,#92558,#92559) ;
#73910=AXIS2_PLACEMENT_3D('',#119520,#92560,#92561) ;
#73911=AXIS2_PLACEMENT_3D('',#119521,#92562,#92563) ;
#73912=AXIS2_PLACEMENT_3D('',#119522,#92564,#92565) ;
#73913=AXIS2_PLACEMENT_3D('',#119523,#92566,#92567) ;
#73914=AXIS2_PLACEMENT_3D('',#119524,#92568,#92569) ;
#73915=AXIS2_PLACEMENT_3D('',#119525,#92570,#92571) ;
#73916=AXIS2_PLACEMENT_3D('',#119526,#92572,#92573) ;
#73917=AXIS2_PLACEMENT_3D('',#119527,#92574,#92575) ;
#73918=AXIS2_PLACEMENT_3D('',#119528,#92576,#92577) ;
#73919=AXIS2_PLACEMENT_3D('',#119529,#92578,#92579) ;
#73920=AXIS2_PLACEMENT_3D('',#119530,#92580,#92581) ;
#73921=AXIS2_PLACEMENT_3D('',#119531,#92582,#92583) ;
#73922=AXIS2_PLACEMENT_3D('',#119532,#92584,#92585) ;
#73923=AXIS2_PLACEMENT_3D('',#119533,#92586,#92587) ;
#73924=AXIS2_PLACEMENT_3D('',#119534,#92588,#92589) ;
#73925=AXIS2_PLACEMENT_3D('',#119535,#92590,#92591) ;
#73926=AXIS2_PLACEMENT_3D('',#119536,#92592,#92593) ;
#73927=AXIS2_PLACEMENT_3D('',#119537,#92594,#92595) ;
#73928=AXIS2_PLACEMENT_3D('',#119538,#92596,#92597) ;
#73929=AXIS2_PLACEMENT_3D('',#119539,#92598,#92599) ;
#73930=AXIS2_PLACEMENT_3D('',#119540,#92600,#92601) ;
#73931=AXIS2_PLACEMENT_3D('',#119541,#92602,#92603) ;
#73932=AXIS2_PLACEMENT_3D('',#119542,#92604,#92605) ;
#73933=AXIS2_PLACEMENT_3D('',#119543,#92606,#92607) ;
#73934=AXIS2_PLACEMENT_3D('',#119544,#92608,#92609) ;
#73935=AXIS2_PLACEMENT_3D('',#119545,#92610,#92611) ;
#73936=AXIS2_PLACEMENT_3D('',#119546,#92612,#92613) ;
#73937=AXIS2_PLACEMENT_3D('',#119547,#92614,#92615) ;
#73938=AXIS2_PLACEMENT_3D('',#119548,#92616,#92617) ;
#73939=AXIS2_PLACEMENT_3D('',#119549,#92618,#92619) ;
#73940=AXIS2_PLACEMENT_3D('',#119550,#92620,#92621) ;
#73941=AXIS2_PLACEMENT_3D('',#119551,#92622,#92623) ;
#73942=AXIS2_PLACEMENT_3D('',#119552,#92624,#92625) ;
#73943=AXIS2_PLACEMENT_3D('',#119553,#92626,#92627) ;
#73944=AXIS2_PLACEMENT_3D('',#119554,#92628,#92629) ;
#73945=AXIS2_PLACEMENT_3D('',#119555,#92630,#92631) ;
#73946=AXIS2_PLACEMENT_3D('',#119556,#92632,#92633) ;
#73947=AXIS2_PLACEMENT_3D('',#119557,#92634,#92635) ;
#73948=AXIS2_PLACEMENT_3D('',#119558,#92636,#92637) ;
#73949=AXIS2_PLACEMENT_3D('',#119559,#92638,#92639) ;
#73950=AXIS2_PLACEMENT_3D('',#119560,#92640,#92641) ;
#73951=AXIS2_PLACEMENT_3D('',#119561,#92642,#92643) ;
#73952=AXIS2_PLACEMENT_3D('',#119562,#92644,#92645) ;
#73953=AXIS2_PLACEMENT_3D('',#119563,#92646,#92647) ;
#73954=AXIS2_PLACEMENT_3D('',#119564,#92648,#92649) ;
#73955=AXIS2_PLACEMENT_3D('',#119565,#92650,#92651) ;
#73956=AXIS2_PLACEMENT_3D('',#119566,#92652,#92653) ;
#73957=AXIS2_PLACEMENT_3D('',#119567,#92654,#92655) ;
#73958=AXIS2_PLACEMENT_3D('',#119568,#92656,#92657) ;
#73959=AXIS2_PLACEMENT_3D('',#119569,#92658,#92659) ;
#73960=AXIS2_PLACEMENT_3D('',#119570,#92660,#92661) ;
#73961=AXIS2_PLACEMENT_3D('',#119571,#92662,#92663) ;
#73962=AXIS2_PLACEMENT_3D('',#119572,#92664,#92665) ;
#73963=AXIS2_PLACEMENT_3D('',#119573,#92666,#92667) ;
#73964=AXIS2_PLACEMENT_3D('',#119574,#92668,#92669) ;
#73965=AXIS2_PLACEMENT_3D('',#119575,#92670,#92671) ;
#73966=AXIS2_PLACEMENT_3D('',#119576,#92672,#92673) ;
#73967=AXIS2_PLACEMENT_3D('',#119577,#92674,#92675) ;
#73968=AXIS2_PLACEMENT_3D('',#119578,#92676,#92677) ;
#73969=AXIS2_PLACEMENT_3D('',#119579,#92678,#92679) ;
#73970=AXIS2_PLACEMENT_3D('',#119580,#92680,#92681) ;
#73971=AXIS2_PLACEMENT_3D('',#119581,#92682,#92683) ;
#73972=AXIS2_PLACEMENT_3D('',#119582,#92684,#92685) ;
#73973=AXIS2_PLACEMENT_3D('',#119583,#92686,#92687) ;
#73974=AXIS2_PLACEMENT_3D('',#119584,#92688,#92689) ;
#73975=AXIS2_PLACEMENT_3D('',#119585,#92690,#92691) ;
#73976=AXIS2_PLACEMENT_3D('',#119586,#92692,#92693) ;
#73977=AXIS2_PLACEMENT_3D('',#119587,#92694,#92695) ;
#73978=AXIS2_PLACEMENT_3D('',#119588,#92696,#92697) ;
#73979=AXIS2_PLACEMENT_3D('',#119589,#92698,#92699) ;
#73980=AXIS2_PLACEMENT_3D('',#119590,#92700,#92701) ;
#73981=AXIS2_PLACEMENT_3D('',#119591,#92702,#92703) ;
#73982=AXIS2_PLACEMENT_3D('',#119592,#92704,#92705) ;
#73983=AXIS2_PLACEMENT_3D('',#119593,#92706,#92707) ;
#73984=AXIS2_PLACEMENT_3D('',#119594,#92708,#92709) ;
#73985=AXIS2_PLACEMENT_3D('',#119595,#92710,#92711) ;
#73986=AXIS2_PLACEMENT_3D('',#119596,#92712,#92713) ;
#73987=AXIS2_PLACEMENT_3D('',#119597,#92714,#92715) ;
#73988=AXIS2_PLACEMENT_3D('',#119598,#92716,#92717) ;
#73989=AXIS2_PLACEMENT_3D('',#119599,#92718,#92719) ;
#73990=AXIS2_PLACEMENT_3D('',#119600,#92720,#92721) ;
#73991=AXIS2_PLACEMENT_3D('',#119601,#92722,#92723) ;
#73992=AXIS2_PLACEMENT_3D('',#119602,#92724,#92725) ;
#73993=AXIS2_PLACEMENT_3D('',#119603,#92726,#92727) ;
#73994=AXIS2_PLACEMENT_3D('',#119604,#92728,#92729) ;
#73995=AXIS2_PLACEMENT_3D('',#119605,#92730,#92731) ;
#73996=AXIS2_PLACEMENT_3D('',#119606,#92732,#92733) ;
#73997=AXIS2_PLACEMENT_3D('',#119607,#92734,#92735) ;
#73998=AXIS2_PLACEMENT_3D('',#119608,#92736,#92737) ;
#73999=AXIS2_PLACEMENT_3D('',#119609,#92738,#92739) ;
#74000=AXIS2_PLACEMENT_3D('',#119610,#92740,#92741) ;
#74001=AXIS2_PLACEMENT_3D('',#119611,#92742,#92743) ;
#74002=AXIS2_PLACEMENT_3D('',#119612,#92744,#92745) ;
#74003=AXIS2_PLACEMENT_3D('',#119613,#92746,#92747) ;
#74004=AXIS2_PLACEMENT_3D('',#119614,#92748,#92749) ;
#74005=AXIS2_PLACEMENT_3D('',#119615,#92750,#92751) ;
#74006=AXIS2_PLACEMENT_3D('',#119616,#92752,#92753) ;
#74007=AXIS2_PLACEMENT_3D('',#119617,#92754,#92755) ;
#74008=AXIS2_PLACEMENT_3D('',#119618,#92756,#92757) ;
#74009=AXIS2_PLACEMENT_3D('',#119619,#92758,#92759) ;
#74010=AXIS2_PLACEMENT_3D('',#119620,#92760,#92761) ;
#74011=AXIS2_PLACEMENT_3D('',#119621,#92762,#92763) ;
#74012=AXIS2_PLACEMENT_3D('',#119622,#92764,#92765) ;
#74013=AXIS2_PLACEMENT_3D('',#119623,#92766,#92767) ;
#74014=AXIS2_PLACEMENT_3D('',#119624,#92768,#92769) ;
#74015=AXIS2_PLACEMENT_3D('',#119625,#92770,#92771) ;
#74016=AXIS2_PLACEMENT_3D('',#119626,#92772,#92773) ;
#74017=AXIS2_PLACEMENT_3D('',#119627,#92774,#92775) ;
#74018=AXIS2_PLACEMENT_3D('',#119628,#92776,#92777) ;
#74019=AXIS2_PLACEMENT_3D('',#119629,#92778,#92779) ;
#74020=AXIS2_PLACEMENT_3D('',#119630,#92780,#92781) ;
#74021=AXIS2_PLACEMENT_3D('',#119631,#92782,#92783) ;
#74022=AXIS2_PLACEMENT_3D('',#119632,#92784,#92785) ;
#74023=AXIS2_PLACEMENT_3D('',#119633,#92786,#92787) ;
#74024=AXIS2_PLACEMENT_3D('',#119634,#92788,#92789) ;
#74025=AXIS2_PLACEMENT_3D('',#119635,#92790,#92791) ;
#74026=AXIS2_PLACEMENT_3D('',#119636,#92792,#92793) ;
#74027=AXIS2_PLACEMENT_3D('',#119637,#92794,#92795) ;
#74028=AXIS2_PLACEMENT_3D('',#119638,#92796,#92797) ;
#74029=AXIS2_PLACEMENT_3D('',#119639,#92798,#92799) ;
#74030=AXIS2_PLACEMENT_3D('',#119640,#92800,#92801) ;
#74031=AXIS2_PLACEMENT_3D('',#119641,#92802,#92803) ;
#74032=AXIS2_PLACEMENT_3D('',#119642,#92804,#92805) ;
#74033=AXIS2_PLACEMENT_3D('',#119643,#92806,#92807) ;
#74034=AXIS2_PLACEMENT_3D('',#119644,#92808,#92809) ;
#74035=AXIS2_PLACEMENT_3D('',#119645,#92810,#92811) ;
#74036=AXIS2_PLACEMENT_3D('',#119646,#92812,#92813) ;
#74037=AXIS2_PLACEMENT_3D('',#119647,#92814,#92815) ;
#74038=AXIS2_PLACEMENT_3D('',#119648,#92816,#92817) ;
#74039=AXIS2_PLACEMENT_3D('',#119649,#92818,#92819) ;
#74040=AXIS2_PLACEMENT_3D('',#119650,#92820,#92821) ;
#74041=AXIS2_PLACEMENT_3D('',#119651,#92822,#92823) ;
#74042=AXIS2_PLACEMENT_3D('',#119652,#92824,#92825) ;
#74043=AXIS2_PLACEMENT_3D('',#119653,#92826,#92827) ;
#74044=AXIS2_PLACEMENT_3D('',#119654,#92828,#92829) ;
#74045=AXIS2_PLACEMENT_3D('',#119655,#92830,#92831) ;
#74046=AXIS2_PLACEMENT_3D('',#119656,#92832,#92833) ;
#74047=AXIS2_PLACEMENT_3D('',#119657,#92834,#92835) ;
#74048=AXIS2_PLACEMENT_3D('',#119658,#92836,#92837) ;
#74049=AXIS2_PLACEMENT_3D('',#119659,#92838,#92839) ;
#74050=AXIS2_PLACEMENT_3D('',#119660,#92840,#92841) ;
#74051=AXIS2_PLACEMENT_3D('',#119661,#92842,#92843) ;
#74052=AXIS2_PLACEMENT_3D('',#119662,#92844,#92845) ;
#74053=AXIS2_PLACEMENT_3D('',#119663,#92846,#92847) ;
#74054=AXIS2_PLACEMENT_3D('',#119664,#92848,#92849) ;
#74055=AXIS2_PLACEMENT_3D('',#119665,#92850,#92851) ;
#74056=AXIS2_PLACEMENT_3D('',#119666,#92852,#92853) ;
#74057=AXIS2_PLACEMENT_3D('',#119667,#92854,#92855) ;
#74058=AXIS2_PLACEMENT_3D('',#119668,#92856,#92857) ;
#74059=AXIS2_PLACEMENT_3D('',#119669,#92858,#92859) ;
#74060=AXIS2_PLACEMENT_3D('',#119670,#92860,#92861) ;
#74061=AXIS2_PLACEMENT_3D('',#119671,#92862,#92863) ;
#74062=AXIS2_PLACEMENT_3D('',#119672,#92864,#92865) ;
#74063=AXIS2_PLACEMENT_3D('',#119673,#92866,#92867) ;
#74064=AXIS2_PLACEMENT_3D('',#119674,#92868,#92869) ;
#74065=AXIS2_PLACEMENT_3D('',#119675,#92870,#92871) ;
#74066=AXIS2_PLACEMENT_3D('',#119676,#92872,#92873) ;
#74067=AXIS2_PLACEMENT_3D('',#119677,#92874,#92875) ;
#74068=AXIS2_PLACEMENT_3D('',#119678,#92876,#92877) ;
#74069=AXIS2_PLACEMENT_3D('',#119679,#92878,#92879) ;
#74070=AXIS2_PLACEMENT_3D('',#119680,#92880,#92881) ;
#74071=AXIS2_PLACEMENT_3D('',#119681,#92882,#92883) ;
#74072=AXIS2_PLACEMENT_3D('',#119682,#92884,#92885) ;
#74073=AXIS2_PLACEMENT_3D('',#119683,#92886,#92887) ;
#74074=AXIS2_PLACEMENT_3D('',#119684,#92888,#92889) ;
#74075=AXIS2_PLACEMENT_3D('',#119685,#92890,#92891) ;
#74076=AXIS2_PLACEMENT_3D('',#119686,#92892,#92893) ;
#74077=AXIS2_PLACEMENT_3D('',#119687,#92894,#92895) ;
#74078=AXIS2_PLACEMENT_3D('',#119688,#92896,#92897) ;
#74079=AXIS2_PLACEMENT_3D('',#119689,#92898,#92899) ;
#74080=AXIS2_PLACEMENT_3D('',#119690,#92900,#92901) ;
#74081=AXIS2_PLACEMENT_3D('',#119691,#92902,#92903) ;
#74082=AXIS2_PLACEMENT_3D('',#119692,#92904,#92905) ;
#74083=AXIS2_PLACEMENT_3D('',#119693,#92906,#92907) ;
#74084=AXIS2_PLACEMENT_3D('',#119694,#92908,#92909) ;
#74085=AXIS2_PLACEMENT_3D('',#119695,#92910,#92911) ;
#74086=AXIS2_PLACEMENT_3D('',#119696,#92912,#92913) ;
#74087=AXIS2_PLACEMENT_3D('',#119697,#92914,#92915) ;
#74088=AXIS2_PLACEMENT_3D('',#119698,#92916,#92917) ;
#74089=AXIS2_PLACEMENT_3D('',#119699,#92918,#92919) ;
#74090=AXIS2_PLACEMENT_3D('',#119700,#92920,#92921) ;
#74091=AXIS2_PLACEMENT_3D('',#119701,#92922,#92923) ;
#74092=AXIS2_PLACEMENT_3D('',#119702,#92924,#92925) ;
#74093=AXIS2_PLACEMENT_3D('',#119703,#92926,#92927) ;
#74094=AXIS2_PLACEMENT_3D('',#119704,#92928,#92929) ;
#74095=AXIS2_PLACEMENT_3D('',#119705,#92930,#92931) ;
#74096=AXIS2_PLACEMENT_3D('',#119706,#92932,#92933) ;
#74097=AXIS2_PLACEMENT_3D('',#119707,#92934,#92935) ;
#74098=AXIS2_PLACEMENT_3D('',#119708,#92936,#92937) ;
#74099=AXIS2_PLACEMENT_3D('',#119709,#92938,#92939) ;
#74100=AXIS2_PLACEMENT_3D('',#119710,#92940,#92941) ;
#74101=AXIS2_PLACEMENT_3D('',#119711,#92942,#92943) ;
#74102=AXIS2_PLACEMENT_3D('',#119712,#92944,#92945) ;
#74103=AXIS2_PLACEMENT_3D('',#119713,#92946,#92947) ;
#74104=AXIS2_PLACEMENT_3D('',#119714,#92948,#92949) ;
#74105=AXIS2_PLACEMENT_3D('',#119715,#92950,#92951) ;
#74106=AXIS2_PLACEMENT_3D('',#119716,#92952,#92953) ;
#74107=AXIS2_PLACEMENT_3D('',#119717,#92954,#92955) ;
#74108=AXIS2_PLACEMENT_3D('',#119718,#92956,#92957) ;
#74109=AXIS2_PLACEMENT_3D('',#119719,#92958,#92959) ;
#74110=AXIS2_PLACEMENT_3D('',#119720,#92960,#92961) ;
#74111=AXIS2_PLACEMENT_3D('',#119721,#92962,#92963) ;
#74112=AXIS2_PLACEMENT_3D('',#119722,#92964,#92965) ;
#74113=AXIS2_PLACEMENT_3D('',#119723,#92966,#92967) ;
#74114=AXIS2_PLACEMENT_3D('',#119724,#92968,#92969) ;
#74115=AXIS2_PLACEMENT_3D('',#119725,#92970,#92971) ;
#74116=AXIS2_PLACEMENT_3D('',#119726,#92972,#92973) ;
#74117=AXIS2_PLACEMENT_3D('',#119727,#92974,#92975) ;
#74118=AXIS2_PLACEMENT_3D('',#119728,#92976,#92977) ;
#74119=AXIS2_PLACEMENT_3D('',#119729,#92978,#92979) ;
#74120=AXIS2_PLACEMENT_3D('',#119730,#92980,#92981) ;
#74121=AXIS2_PLACEMENT_3D('',#119731,#92982,#92983) ;
#74122=AXIS2_PLACEMENT_3D('',#119732,#92984,#92985) ;
#74123=AXIS2_PLACEMENT_3D('',#119733,#92986,#92987) ;
#74124=AXIS2_PLACEMENT_3D('',#119734,#92988,#92989) ;
#74125=AXIS2_PLACEMENT_3D('',#119735,#92990,#92991) ;
#74126=AXIS2_PLACEMENT_3D('',#119736,#92992,#92993) ;
#74127=AXIS2_PLACEMENT_3D('',#119737,#92994,#92995) ;
#74128=AXIS2_PLACEMENT_3D('',#119738,#92996,#92997) ;
#74129=AXIS2_PLACEMENT_3D('',#119739,#92998,#92999) ;
#74130=AXIS2_PLACEMENT_3D('',#119740,#93000,#93001) ;
#74131=AXIS2_PLACEMENT_3D('',#119741,#93002,#93003) ;
#74132=AXIS2_PLACEMENT_3D('',#119742,#93004,#93005) ;
#74133=AXIS2_PLACEMENT_3D('',#119743,#93006,#93007) ;
#74134=AXIS2_PLACEMENT_3D('',#119744,#93008,#93009) ;
#74135=AXIS2_PLACEMENT_3D('',#119745,#93010,#93011) ;
#74136=AXIS2_PLACEMENT_3D('',#119746,#93012,#93013) ;
#74137=AXIS2_PLACEMENT_3D('',#119747,#93014,#93015) ;
#74138=AXIS2_PLACEMENT_3D('',#119748,#93016,#93017) ;
#74139=AXIS2_PLACEMENT_3D('',#119749,#93018,#93019) ;
#74140=AXIS2_PLACEMENT_3D('',#119750,#93020,#93021) ;
#74141=AXIS2_PLACEMENT_3D('',#119751,#93022,#93023) ;
#74142=AXIS2_PLACEMENT_3D('',#119752,#93024,#93025) ;
#74143=AXIS2_PLACEMENT_3D('',#119753,#93026,#93027) ;
#74144=AXIS2_PLACEMENT_3D('',#119754,#93028,#93029) ;
#74145=AXIS2_PLACEMENT_3D('',#119755,#93030,#93031) ;
#74146=AXIS2_PLACEMENT_3D('',#119756,#93032,#93033) ;
#74147=AXIS2_PLACEMENT_3D('',#119757,#93034,#93035) ;
#74148=AXIS2_PLACEMENT_3D('',#119758,#93036,#93037) ;
#74149=AXIS2_PLACEMENT_3D('',#119759,#93038,#93039) ;
#74150=AXIS2_PLACEMENT_3D('',#119760,#93040,#93041) ;
#74151=AXIS2_PLACEMENT_3D('',#119761,#93042,#93043) ;
#74152=AXIS2_PLACEMENT_3D('',#119762,#93044,#93045) ;
#74153=AXIS2_PLACEMENT_3D('',#119763,#93046,#93047) ;
#74154=AXIS2_PLACEMENT_3D('',#119764,#93048,#93049) ;
#74155=AXIS2_PLACEMENT_3D('',#119765,#93050,#93051) ;
#74156=AXIS2_PLACEMENT_3D('',#119766,#93052,#93053) ;
#74157=AXIS2_PLACEMENT_3D('',#119767,#93054,#93055) ;
#74158=AXIS2_PLACEMENT_3D('',#119768,#93056,#93057) ;
#74159=AXIS2_PLACEMENT_3D('',#119769,#93058,#93059) ;
#74160=AXIS2_PLACEMENT_3D('',#119770,#93060,#93061) ;
#74161=AXIS2_PLACEMENT_3D('',#119771,#93062,#93063) ;
#74162=AXIS2_PLACEMENT_3D('',#119772,#93064,#93065) ;
#74163=AXIS2_PLACEMENT_3D('',#119773,#93066,#93067) ;
#74164=AXIS2_PLACEMENT_3D('',#119774,#93068,#93069) ;
#74165=AXIS2_PLACEMENT_3D('',#119775,#93070,#93071) ;
#74166=AXIS2_PLACEMENT_3D('',#119776,#93072,#93073) ;
#74167=AXIS2_PLACEMENT_3D('',#119777,#93074,#93075) ;
#74168=AXIS2_PLACEMENT_3D('',#119778,#93076,#93077) ;
#74169=AXIS2_PLACEMENT_3D('',#119779,#93078,#93079) ;
#74170=AXIS2_PLACEMENT_3D('',#119780,#93080,#93081) ;
#74171=AXIS2_PLACEMENT_3D('',#119781,#93082,#93083) ;
#74172=AXIS2_PLACEMENT_3D('',#119782,#93084,#93085) ;
#74173=AXIS2_PLACEMENT_3D('',#119783,#93086,#93087) ;
#74174=AXIS2_PLACEMENT_3D('',#119784,#93088,#93089) ;
#74175=AXIS2_PLACEMENT_3D('',#119785,#93090,#93091) ;
#74176=AXIS2_PLACEMENT_3D('',#119786,#93092,#93093) ;
#74177=AXIS2_PLACEMENT_3D('',#119787,#93094,#93095) ;
#74178=AXIS2_PLACEMENT_3D('',#119788,#93096,#93097) ;
#74179=AXIS2_PLACEMENT_3D('',#119789,#93098,#93099) ;
#74180=AXIS2_PLACEMENT_3D('',#119790,#93100,#93101) ;
#74181=AXIS2_PLACEMENT_3D('',#119791,#93102,#93103) ;
#74182=AXIS2_PLACEMENT_3D('',#119792,#93104,#93105) ;
#74183=AXIS2_PLACEMENT_3D('',#119793,#93106,#93107) ;
#74184=AXIS2_PLACEMENT_3D('',#119794,#93108,#93109) ;
#74185=AXIS2_PLACEMENT_3D('',#119795,#93110,#93111) ;
#74186=AXIS2_PLACEMENT_3D('',#119796,#93112,#93113) ;
#74187=AXIS2_PLACEMENT_3D('',#119797,#93114,#93115) ;
#74188=AXIS2_PLACEMENT_3D('',#119798,#93116,#93117) ;
#74189=AXIS2_PLACEMENT_3D('',#119799,#93118,#93119) ;
#74190=AXIS2_PLACEMENT_3D('',#119800,#93120,#93121) ;
#74191=AXIS2_PLACEMENT_3D('',#119801,#93122,#93123) ;
#74192=AXIS2_PLACEMENT_3D('',#119803,#93124,#93125) ;
#74193=AXIS2_PLACEMENT_3D('',#119804,#93126,#93127) ;
#74194=AXIS2_PLACEMENT_3D('',#119805,#93128,#93129) ;
#74195=AXIS2_PLACEMENT_3D('',#119806,#93130,#93131) ;
#74196=AXIS2_PLACEMENT_3D('',#119807,#93132,#93133) ;
#74197=AXIS2_PLACEMENT_3D('',#119808,#93134,#93135) ;
#74198=AXIS2_PLACEMENT_3D('',#119809,#93136,#93137) ;
#74199=AXIS2_PLACEMENT_3D('',#119810,#93138,#93139) ;
#74200=AXIS2_PLACEMENT_3D('',#119811,#93140,#93141) ;
#74201=AXIS2_PLACEMENT_3D('',#119822,#93143,#93144) ;
#74202=AXIS2_PLACEMENT_3D('',#119879,#93146,#93147) ;
#74203=AXIS2_PLACEMENT_3D('',#119880,#93148,#93149) ;
#74204=AXIS2_PLACEMENT_3D('',#119881,#93150,#93151) ;
#74205=AXIS2_PLACEMENT_3D('',#119882,#93152,#93153) ;
#74206=AXIS2_PLACEMENT_3D('',#119883,#93154,#93155) ;
#74207=AXIS2_PLACEMENT_3D('',#119884,#93156,#93157) ;
#74208=AXIS2_PLACEMENT_3D('',#119885,#93158,#93159) ;
#74209=AXIS2_PLACEMENT_3D('',#119886,#93160,#93161) ;
#74210=AXIS2_PLACEMENT_3D('',#119887,#93162,#93163) ;
#74211=AXIS2_PLACEMENT_3D('',#119888,#93164,#93165) ;
#74212=AXIS2_PLACEMENT_3D('',#119889,#93166,#93167) ;
#74213=AXIS2_PLACEMENT_3D('',#119890,#93168,#93169) ;
#74214=AXIS2_PLACEMENT_3D('',#119891,#93170,#93171) ;
#74215=AXIS2_PLACEMENT_3D('',#119892,#93172,#93173) ;
#74216=AXIS2_PLACEMENT_3D('',#119893,#93174,#93175) ;
#74217=AXIS2_PLACEMENT_3D('',#119894,#93176,#93177) ;
#74218=AXIS2_PLACEMENT_3D('',#119895,#93178,#93179) ;
#74219=AXIS2_PLACEMENT_3D('',#119896,#93180,#93181) ;
#74220=AXIS2_PLACEMENT_3D('',#119897,#93182,#93183) ;
#74221=AXIS2_PLACEMENT_3D('',#119898,#93184,#93185) ;
#74222=AXIS2_PLACEMENT_3D('',#119899,#93186,#93187) ;
#74223=AXIS2_PLACEMENT_3D('',#119900,#93188,#93189) ;
#74224=AXIS2_PLACEMENT_3D('',#119901,#93190,#93191) ;
#74225=AXIS2_PLACEMENT_3D('',#119904,#93193,#93194) ;
#74226=AXIS2_PLACEMENT_3D('',#119905,#93195,#93196) ;
#74227=AXIS2_PLACEMENT_3D('',#119906,#93197,#93198) ;
#74228=AXIS2_PLACEMENT_3D('',#119907,#93199,#93200) ;
#74229=AXIS2_PLACEMENT_3D('',#119908,#93201,#93202) ;
#74230=AXIS2_PLACEMENT_3D('',#119909,#93203,#93204) ;
#74231=AXIS2_PLACEMENT_3D('',#119910,#93205,#93206) ;
#74232=AXIS2_PLACEMENT_3D('',#119911,#93207,#93208) ;
#74233=AXIS2_PLACEMENT_3D('',#119912,#93209,#93210) ;
#74234=AXIS2_PLACEMENT_3D('',#119913,#93211,#93212) ;
#74235=AXIS2_PLACEMENT_3D('',#119914,#93213,#93214) ;
#74236=AXIS2_PLACEMENT_3D('',#119915,#93215,#93216) ;
#74237=AXIS2_PLACEMENT_3D('',#119916,#93217,#93218) ;
#74238=AXIS2_PLACEMENT_3D('',#119917,#93219,#93220) ;
#74239=AXIS2_PLACEMENT_3D('',#119918,#93221,#93222) ;
#74240=AXIS2_PLACEMENT_3D('',#119919,#93223,#93224) ;
#74241=AXIS2_PLACEMENT_3D('',#119921,#93225,#93226) ;
#74242=AXIS2_PLACEMENT_3D('',#119922,#93227,#93228) ;
#74243=AXIS2_PLACEMENT_3D('',#119923,#93229,#93230) ;
#74244=AXIS2_PLACEMENT_3D('',#119924,#93231,#93232) ;
#74245=AXIS2_PLACEMENT_3D('',#119925,#93233,#93234) ;
#74246=AXIS2_PLACEMENT_3D('',#119926,#93235,#93236) ;
#74247=AXIS2_PLACEMENT_3D('',#119927,#93237,#93238) ;
#74248=AXIS2_PLACEMENT_3D('',#119928,#93239,#93240) ;
#74249=AXIS2_PLACEMENT_3D('',#119929,#93241,#93242) ;
#74250=AXIS2_PLACEMENT_3D('',#119930,#93243,#93244) ;
#74251=AXIS2_PLACEMENT_3D('',#119931,#93245,#93246) ;
#74252=AXIS2_PLACEMENT_3D('',#119932,#93247,#93248) ;
#74253=AXIS2_PLACEMENT_3D('',#119933,#93249,#93250) ;
#74254=AXIS2_PLACEMENT_3D('',#119936,#93252,#93253) ;
#74255=AXIS2_PLACEMENT_3D('',#119937,#93254,#93255) ;
#74256=AXIS2_PLACEMENT_3D('',#119938,#93256,#93257) ;
#74257=AXIS2_PLACEMENT_3D('',#119939,#93258,#93259) ;
#74258=AXIS2_PLACEMENT_3D('',#119940,#93260,#93261) ;
#74259=AXIS2_PLACEMENT_3D('',#119941,#93262,#93263) ;
#74260=AXIS2_PLACEMENT_3D('',#119942,#93264,#93265) ;
#74261=AXIS2_PLACEMENT_3D('',#119943,#93266,#93267) ;
#74262=AXIS2_PLACEMENT_3D('',#119944,#93268,#93269) ;
#74263=AXIS2_PLACEMENT_3D('',#119945,#93270,#93271) ;
#74264=AXIS2_PLACEMENT_3D('',#119946,#93272,#93273) ;
#74265=AXIS2_PLACEMENT_3D('',#119947,#93274,#93275) ;
#74266=AXIS2_PLACEMENT_3D('',#119948,#93276,#93277) ;
#74267=AXIS2_PLACEMENT_3D('',#119950,#93278,#93279) ;
#74268=AXIS2_PLACEMENT_3D('',#119951,#93280,#93281) ;
#74269=AXIS2_PLACEMENT_3D('',#119952,#93282,#93283) ;
#74270=AXIS2_PLACEMENT_3D('',#119953,#93284,#93285) ;
#74271=AXIS2_PLACEMENT_3D('',#119954,#93286,#93287) ;
#74272=AXIS2_PLACEMENT_3D('',#119955,#93288,#93289) ;
#74273=AXIS2_PLACEMENT_3D('',#119956,#93290,#93291) ;
#74274=AXIS2_PLACEMENT_3D('',#119957,#93292,#93293) ;
#74275=AXIS2_PLACEMENT_3D('',#119958,#93294,#93295) ;
#74276=AXIS2_PLACEMENT_3D('',#119959,#93296,#93297) ;
#74277=AXIS2_PLACEMENT_3D('',#119960,#93298,#93299) ;
#74278=AXIS2_PLACEMENT_3D('',#119962,#93301,#93302) ;
#74279=AXIS2_PLACEMENT_3D('',#119963,#93303,#93304) ;
#74280=AXIS2_PLACEMENT_3D('',#119964,#93305,#93306) ;
#74281=AXIS2_PLACEMENT_3D('',#119965,#93307,#93308) ;
#74282=AXIS2_PLACEMENT_3D('',#119966,#93309,#93310) ;
#74283=AXIS2_PLACEMENT_3D('',#119967,#93311,#93312) ;
#74284=AXIS2_PLACEMENT_3D('',#119968,#93313,#93314) ;
#74285=AXIS2_PLACEMENT_3D('',#119969,#93315,#93316) ;
#74286=AXIS2_PLACEMENT_3D('',#119970,#93317,#93318) ;
#74287=AXIS2_PLACEMENT_3D('',#119971,#93319,#93320) ;
#74288=AXIS2_PLACEMENT_3D('',#119972,#93321,#93322) ;
#74289=AXIS2_PLACEMENT_3D('',#119973,#93323,#93324) ;
#74290=AXIS2_PLACEMENT_3D('',#119974,#93325,#93326) ;
#74291=AXIS2_PLACEMENT_3D('',#119975,#93327,#93328) ;
#74292=AXIS2_PLACEMENT_3D('',#119976,#93329,#93330) ;
#74293=AXIS2_PLACEMENT_3D('',#119977,#93331,#93332) ;
#74294=AXIS2_PLACEMENT_3D('',#119978,#93333,#93334) ;
#74295=AXIS2_PLACEMENT_3D('',#119979,#93335,#93336) ;
#74296=AXIS2_PLACEMENT_3D('',#119980,#93337,#93338) ;
#74297=AXIS2_PLACEMENT_3D('',#119981,#93339,#93340) ;
#74298=AXIS2_PLACEMENT_3D('',#119982,#93341,#93342) ;
#74299=AXIS2_PLACEMENT_3D('',#119983,#93343,#93344) ;
#74300=AXIS2_PLACEMENT_3D('',#119984,#93345,#93346) ;
#74301=AXIS2_PLACEMENT_3D('',#119985,#93347,#93348) ;
#74302=AXIS2_PLACEMENT_3D('',#119986,#93349,#93350) ;
#74303=AXIS2_PLACEMENT_3D('',#119987,#93351,#93352) ;
#74304=AXIS2_PLACEMENT_3D('',#119988,#93353,#93354) ;
#74305=AXIS2_PLACEMENT_3D('',#119989,#93355,#93356) ;
#74306=AXIS2_PLACEMENT_3D('',#119990,#93357,#93358) ;
#74307=AXIS2_PLACEMENT_3D('',#119991,#93359,#93360) ;
#74308=AXIS2_PLACEMENT_3D('',#119992,#93361,#93362) ;
#74309=AXIS2_PLACEMENT_3D('',#119993,#93363,#93364) ;
#74310=AXIS2_PLACEMENT_3D('',#119994,#93365,#93366) ;
#74311=AXIS2_PLACEMENT_3D('',#119995,#93367,#93368) ;
#74312=AXIS2_PLACEMENT_3D('',#119996,#93369,#93370) ;
#74313=AXIS2_PLACEMENT_3D('',#119997,#93371,#93372) ;
#74314=AXIS2_PLACEMENT_3D('',#119998,#93373,#93374) ;
#74315=AXIS2_PLACEMENT_3D('',#119999,#93375,#93376) ;
#74316=AXIS2_PLACEMENT_3D('',#120000,#93377,#93378) ;
#74317=AXIS2_PLACEMENT_3D('',#120001,#93379,#93380) ;
#74318=AXIS2_PLACEMENT_3D('',#120002,#93381,#93382) ;
#74319=AXIS2_PLACEMENT_3D('',#120003,#93383,#93384) ;
#74320=AXIS2_PLACEMENT_3D('',#120004,#93385,#93386) ;
#74321=AXIS2_PLACEMENT_3D('',#120005,#93387,#93388) ;
#74322=AXIS2_PLACEMENT_3D('',#120006,#93389,#93390) ;
#74323=AXIS2_PLACEMENT_3D('',#120007,#93391,#93392) ;
#74324=AXIS2_PLACEMENT_3D('',#120008,#93393,#93394) ;
#74325=AXIS2_PLACEMENT_3D('',#120009,#93395,#93396) ;
#74326=AXIS2_PLACEMENT_3D('',#120010,#93397,#93398) ;
#74327=AXIS2_PLACEMENT_3D('',#120011,#93399,#93400) ;
#74328=AXIS2_PLACEMENT_3D('',#120012,#93401,#93402) ;
#74329=AXIS2_PLACEMENT_3D('',#120013,#93403,#93404) ;
#74330=AXIS2_PLACEMENT_3D('',#120014,#93405,#93406) ;
#74331=AXIS2_PLACEMENT_3D('',#120015,#93407,#93408) ;
#74332=AXIS2_PLACEMENT_3D('',#120016,#93409,#93410) ;
#74333=AXIS2_PLACEMENT_3D('',#120017,#93411,#93412) ;
#74334=AXIS2_PLACEMENT_3D('',#120018,#93413,#93414) ;
#74335=AXIS2_PLACEMENT_3D('',#120019,#93415,#93416) ;
#74336=AXIS2_PLACEMENT_3D('',#120020,#93417,#93418) ;
#74337=AXIS2_PLACEMENT_3D('',#120021,#93419,#93420) ;
#74338=AXIS2_PLACEMENT_3D('',#120022,#93421,#93422) ;
#74339=AXIS2_PLACEMENT_3D('',#120023,#93423,#93424) ;
#74340=AXIS2_PLACEMENT_3D('',#120024,#93425,#93426) ;
#74341=AXIS2_PLACEMENT_3D('',#120025,#93427,#93428) ;
#74342=AXIS2_PLACEMENT_3D('',#120026,#93429,#93430) ;
#74343=AXIS2_PLACEMENT_3D('',#120027,#93431,#93432) ;
#74344=AXIS2_PLACEMENT_3D('',#120028,#93433,#93434) ;
#74345=AXIS2_PLACEMENT_3D('',#120030,#93435,#93436) ;
#74346=AXIS2_PLACEMENT_3D('',#120031,#93437,#93438) ;
#74347=AXIS2_PLACEMENT_3D('',#120032,#93439,#93440) ;
#74348=AXIS2_PLACEMENT_3D('',#120033,#93441,#93442) ;
#74349=AXIS2_PLACEMENT_3D('',#120034,#93443,#93444) ;
#74350=AXIS2_PLACEMENT_3D('',#120035,#93445,#93446) ;
#74351=AXIS2_PLACEMENT_3D('',#120036,#93447,#93448) ;
#74352=AXIS2_PLACEMENT_3D('',#120037,#93449,#93450) ;
#74353=AXIS2_PLACEMENT_3D('',#120038,#93451,#93452) ;
#74354=AXIS2_PLACEMENT_3D('',#120049,#93454,#93455) ;
#74355=AXIS2_PLACEMENT_3D('',#120106,#93457,#93458) ;
#74356=AXIS2_PLACEMENT_3D('',#120107,#93459,#93460) ;
#74357=AXIS2_PLACEMENT_3D('',#120108,#93461,#93462) ;
#74358=AXIS2_PLACEMENT_3D('',#120109,#93463,#93464) ;
#74359=AXIS2_PLACEMENT_3D('',#120110,#93465,#93466) ;
#74360=AXIS2_PLACEMENT_3D('',#120111,#93467,#93468) ;
#74361=AXIS2_PLACEMENT_3D('',#120112,#93469,#93470) ;
#74362=AXIS2_PLACEMENT_3D('',#120113,#93471,#93472) ;
#74363=AXIS2_PLACEMENT_3D('',#120114,#93473,#93474) ;
#74364=AXIS2_PLACEMENT_3D('',#120115,#93475,#93476) ;
#74365=AXIS2_PLACEMENT_3D('',#120116,#93477,#93478) ;
#74366=AXIS2_PLACEMENT_3D('',#120117,#93479,#93480) ;
#74367=AXIS2_PLACEMENT_3D('',#120118,#93481,#93482) ;
#74368=AXIS2_PLACEMENT_3D('',#120119,#93483,#93484) ;
#74369=AXIS2_PLACEMENT_3D('',#120120,#93485,#93486) ;
#74370=AXIS2_PLACEMENT_3D('',#120121,#93487,#93488) ;
#74371=AXIS2_PLACEMENT_3D('',#120122,#93489,#93490) ;
#74372=AXIS2_PLACEMENT_3D('',#120123,#93491,#93492) ;
#74373=AXIS2_PLACEMENT_3D('',#120124,#93493,#93494) ;
#74374=AXIS2_PLACEMENT_3D('',#120125,#93495,#93496) ;
#74375=AXIS2_PLACEMENT_3D('',#120126,#93497,#93498) ;
#74376=AXIS2_PLACEMENT_3D('',#120127,#93499,#93500) ;
#74377=AXIS2_PLACEMENT_3D('',#120128,#93501,#93502) ;
#74378=AXIS2_PLACEMENT_3D('',#120131,#93504,#93505) ;
#74379=AXIS2_PLACEMENT_3D('',#120132,#93506,#93507) ;
#74380=AXIS2_PLACEMENT_3D('',#120133,#93508,#93509) ;
#74381=AXIS2_PLACEMENT_3D('',#120134,#93510,#93511) ;
#74382=AXIS2_PLACEMENT_3D('',#120135,#93512,#93513) ;
#74383=AXIS2_PLACEMENT_3D('',#120136,#93514,#93515) ;
#74384=AXIS2_PLACEMENT_3D('',#120137,#93516,#93517) ;
#74385=AXIS2_PLACEMENT_3D('',#120138,#93518,#93519) ;
#74386=AXIS2_PLACEMENT_3D('',#120139,#93520,#93521) ;
#74387=AXIS2_PLACEMENT_3D('',#120140,#93522,#93523) ;
#74388=AXIS2_PLACEMENT_3D('',#120141,#93524,#93525) ;
#74389=AXIS2_PLACEMENT_3D('',#120142,#93526,#93527) ;
#74390=AXIS2_PLACEMENT_3D('',#120143,#93528,#93529) ;
#74391=AXIS2_PLACEMENT_3D('',#120144,#93530,#93531) ;
#74392=AXIS2_PLACEMENT_3D('',#120145,#93532,#93533) ;
#74393=AXIS2_PLACEMENT_3D('',#120146,#93534,#93535) ;
#74394=AXIS2_PLACEMENT_3D('',#120148,#93536,#93537) ;
#74395=AXIS2_PLACEMENT_3D('',#120149,#93538,#93539) ;
#74396=AXIS2_PLACEMENT_3D('',#120150,#93540,#93541) ;
#74397=AXIS2_PLACEMENT_3D('',#120151,#93542,#93543) ;
#74398=AXIS2_PLACEMENT_3D('',#120152,#93544,#93545) ;
#74399=AXIS2_PLACEMENT_3D('',#120153,#93546,#93547) ;
#74400=AXIS2_PLACEMENT_3D('',#120154,#93548,#93549) ;
#74401=AXIS2_PLACEMENT_3D('',#120155,#93550,#93551) ;
#74402=AXIS2_PLACEMENT_3D('',#120156,#93552,#93553) ;
#74403=AXIS2_PLACEMENT_3D('',#120157,#93554,#93555) ;
#74404=AXIS2_PLACEMENT_3D('',#120158,#93556,#93557) ;
#74405=AXIS2_PLACEMENT_3D('',#120159,#93558,#93559) ;
#74406=AXIS2_PLACEMENT_3D('',#120160,#93560,#93561) ;
#74407=AXIS2_PLACEMENT_3D('',#120163,#93563,#93564) ;
#74408=AXIS2_PLACEMENT_3D('',#120164,#93565,#93566) ;
#74409=AXIS2_PLACEMENT_3D('',#120165,#93567,#93568) ;
#74410=AXIS2_PLACEMENT_3D('',#120166,#93569,#93570) ;
#74411=AXIS2_PLACEMENT_3D('',#120167,#93571,#93572) ;
#74412=AXIS2_PLACEMENT_3D('',#120168,#93573,#93574) ;
#74413=AXIS2_PLACEMENT_3D('',#120169,#93575,#93576) ;
#74414=AXIS2_PLACEMENT_3D('',#120170,#93577,#93578) ;
#74415=AXIS2_PLACEMENT_3D('',#120171,#93579,#93580) ;
#74416=AXIS2_PLACEMENT_3D('',#120172,#93581,#93582) ;
#74417=AXIS2_PLACEMENT_3D('',#120173,#93583,#93584) ;
#74418=AXIS2_PLACEMENT_3D('',#120174,#93585,#93586) ;
#74419=AXIS2_PLACEMENT_3D('',#120175,#93587,#93588) ;
#74420=AXIS2_PLACEMENT_3D('',#120177,#93589,#93590) ;
#74421=AXIS2_PLACEMENT_3D('',#120178,#93591,#93592) ;
#74422=AXIS2_PLACEMENT_3D('',#120179,#93593,#93594) ;
#74423=AXIS2_PLACEMENT_3D('',#120180,#93595,#93596) ;
#74424=AXIS2_PLACEMENT_3D('',#120181,#93597,#93598) ;
#74425=AXIS2_PLACEMENT_3D('',#120182,#93599,#93600) ;
#74426=AXIS2_PLACEMENT_3D('',#120183,#93601,#93602) ;
#74427=AXIS2_PLACEMENT_3D('',#120184,#93603,#93604) ;
#74428=AXIS2_PLACEMENT_3D('',#120185,#93605,#93606) ;
#74429=AXIS2_PLACEMENT_3D('',#120186,#93607,#93608) ;
#74430=AXIS2_PLACEMENT_3D('',#120187,#93609,#93610) ;
#74431=AXIS2_PLACEMENT_3D('',#120189,#93612,#93613) ;
#74432=AXIS2_PLACEMENT_3D('',#120190,#93614,#93615) ;
#74433=AXIS2_PLACEMENT_3D('',#120191,#93616,#93617) ;
#74434=AXIS2_PLACEMENT_3D('',#120192,#93618,#93619) ;
#74435=AXIS2_PLACEMENT_3D('',#120193,#93620,#93621) ;
#74436=AXIS2_PLACEMENT_3D('',#120194,#93622,#93623) ;
#74437=AXIS2_PLACEMENT_3D('',#120195,#93624,#93625) ;
#74438=AXIS2_PLACEMENT_3D('',#120196,#93626,#93627) ;
#74439=AXIS2_PLACEMENT_3D('',#120197,#93628,#93629) ;
#74440=AXIS2_PLACEMENT_3D('',#120198,#93630,#93631) ;
#74441=AXIS2_PLACEMENT_3D('',#120199,#93632,#93633) ;
#74442=AXIS2_PLACEMENT_3D('',#120200,#93634,#93635) ;
#74443=AXIS2_PLACEMENT_3D('',#120201,#93636,#93637) ;
#74444=AXIS2_PLACEMENT_3D('',#120202,#93638,#93639) ;
#74445=AXIS2_PLACEMENT_3D('',#120203,#93640,#93641) ;
#74446=AXIS2_PLACEMENT_3D('',#120204,#93642,#93643) ;
#74447=AXIS2_PLACEMENT_3D('',#120205,#93644,#93645) ;
#74448=AXIS2_PLACEMENT_3D('',#120206,#93646,#93647) ;
#74449=AXIS2_PLACEMENT_3D('',#120207,#93648,#93649) ;
#74450=AXIS2_PLACEMENT_3D('',#120208,#93650,#93651) ;
#74451=AXIS2_PLACEMENT_3D('',#120209,#93652,#93653) ;
#74452=AXIS2_PLACEMENT_3D('',#120210,#93654,#93655) ;
#74453=AXIS2_PLACEMENT_3D('',#120211,#93656,#93657) ;
#74454=AXIS2_PLACEMENT_3D('',#120212,#93658,#93659) ;
#74455=AXIS2_PLACEMENT_3D('',#120213,#93660,#93661) ;
#74456=AXIS2_PLACEMENT_3D('',#120214,#93662,#93663) ;
#74457=AXIS2_PLACEMENT_3D('',#120215,#93664,#93665) ;
#74458=AXIS2_PLACEMENT_3D('',#120216,#93666,#93667) ;
#74459=AXIS2_PLACEMENT_3D('',#120217,#93668,#93669) ;
#74460=AXIS2_PLACEMENT_3D('',#120218,#93670,#93671) ;
#74461=AXIS2_PLACEMENT_3D('',#120219,#93672,#93673) ;
#74462=AXIS2_PLACEMENT_3D('',#120220,#93674,#93675) ;
#74463=AXIS2_PLACEMENT_3D('',#120221,#93676,#93677) ;
#74464=AXIS2_PLACEMENT_3D('',#120222,#93678,#93679) ;
#74465=AXIS2_PLACEMENT_3D('',#120223,#93680,#93681) ;
#74466=AXIS2_PLACEMENT_3D('',#120224,#93682,#93683) ;
#74467=AXIS2_PLACEMENT_3D('',#120225,#93684,#93685) ;
#74468=AXIS2_PLACEMENT_3D('',#120226,#93686,#93687) ;
#74469=AXIS2_PLACEMENT_3D('',#120227,#93688,#93689) ;
#74470=AXIS2_PLACEMENT_3D('',#120228,#93690,#93691) ;
#74471=AXIS2_PLACEMENT_3D('',#120229,#93692,#93693) ;
#74472=AXIS2_PLACEMENT_3D('',#120230,#93694,#93695) ;
#74473=AXIS2_PLACEMENT_3D('',#120231,#93696,#93697) ;
#74474=AXIS2_PLACEMENT_3D('',#120232,#93698,#93699) ;
#74475=AXIS2_PLACEMENT_3D('',#120233,#93700,#93701) ;
#74476=AXIS2_PLACEMENT_3D('',#120234,#93702,#93703) ;
#74477=AXIS2_PLACEMENT_3D('',#120235,#93704,#93705) ;
#74478=AXIS2_PLACEMENT_3D('',#120236,#93706,#93707) ;
#74479=AXIS2_PLACEMENT_3D('',#120237,#93708,#93709) ;
#74480=AXIS2_PLACEMENT_3D('',#120238,#93710,#93711) ;
#74481=AXIS2_PLACEMENT_3D('',#120239,#93712,#93713) ;
#74482=AXIS2_PLACEMENT_3D('',#120240,#93714,#93715) ;
#74483=AXIS2_PLACEMENT_3D('',#120241,#93716,#93717) ;
#74484=AXIS2_PLACEMENT_3D('',#120242,#93718,#93719) ;
#74485=AXIS2_PLACEMENT_3D('',#120243,#93720,#93721) ;
#74486=AXIS2_PLACEMENT_3D('',#120244,#93722,#93723) ;
#74487=AXIS2_PLACEMENT_3D('',#120245,#93724,#93725) ;
#74488=AXIS2_PLACEMENT_3D('',#120246,#93726,#93727) ;
#74489=AXIS2_PLACEMENT_3D('',#120247,#93728,#93729) ;
#74490=AXIS2_PLACEMENT_3D('',#120248,#93730,#93731) ;
#74491=AXIS2_PLACEMENT_3D('',#120249,#93732,#93733) ;
#74492=AXIS2_PLACEMENT_3D('',#120250,#93734,#93735) ;
#74493=AXIS2_PLACEMENT_3D('',#120251,#93736,#93737) ;
#74494=AXIS2_PLACEMENT_3D('',#120252,#93738,#93739) ;
#74495=AXIS2_PLACEMENT_3D('',#120253,#93740,#93741) ;
#74496=AXIS2_PLACEMENT_3D('',#120254,#93742,#93743) ;
#74497=AXIS2_PLACEMENT_3D('',#120255,#93744,#93745) ;
#74498=AXIS2_PLACEMENT_3D('',#120257,#93746,#93747) ;
#74499=AXIS2_PLACEMENT_3D('',#120258,#93748,#93749) ;
#74500=AXIS2_PLACEMENT_3D('',#120259,#93750,#93751) ;
#74501=AXIS2_PLACEMENT_3D('',#120260,#93752,#93753) ;
#74502=AXIS2_PLACEMENT_3D('',#120261,#93754,#93755) ;
#74503=AXIS2_PLACEMENT_3D('',#120262,#93756,#93757) ;
#74504=AXIS2_PLACEMENT_3D('',#120263,#93758,#93759) ;
#74505=AXIS2_PLACEMENT_3D('',#120264,#93760,#93761) ;
#74506=AXIS2_PLACEMENT_3D('',#120265,#93762,#93763) ;
#74507=AXIS2_PLACEMENT_3D('',#120276,#93765,#93766) ;
#74508=AXIS2_PLACEMENT_3D('',#120333,#93768,#93769) ;
#74509=AXIS2_PLACEMENT_3D('',#120334,#93770,#93771) ;
#74510=AXIS2_PLACEMENT_3D('',#120335,#93772,#93773) ;
#74511=AXIS2_PLACEMENT_3D('',#120336,#93774,#93775) ;
#74512=AXIS2_PLACEMENT_3D('',#120337,#93776,#93777) ;
#74513=AXIS2_PLACEMENT_3D('',#120338,#93778,#93779) ;
#74514=AXIS2_PLACEMENT_3D('',#120339,#93780,#93781) ;
#74515=AXIS2_PLACEMENT_3D('',#120340,#93782,#93783) ;
#74516=AXIS2_PLACEMENT_3D('',#120341,#93784,#93785) ;
#74517=AXIS2_PLACEMENT_3D('',#120342,#93786,#93787) ;
#74518=AXIS2_PLACEMENT_3D('',#120343,#93788,#93789) ;
#74519=AXIS2_PLACEMENT_3D('',#120344,#93790,#93791) ;
#74520=AXIS2_PLACEMENT_3D('',#120345,#93792,#93793) ;
#74521=AXIS2_PLACEMENT_3D('',#120346,#93794,#93795) ;
#74522=AXIS2_PLACEMENT_3D('',#120347,#93796,#93797) ;
#74523=AXIS2_PLACEMENT_3D('',#120348,#93798,#93799) ;
#74524=AXIS2_PLACEMENT_3D('',#120349,#93800,#93801) ;
#74525=AXIS2_PLACEMENT_3D('',#120350,#93802,#93803) ;
#74526=AXIS2_PLACEMENT_3D('',#120351,#93804,#93805) ;
#74527=AXIS2_PLACEMENT_3D('',#120352,#93806,#93807) ;
#74528=AXIS2_PLACEMENT_3D('',#120353,#93808,#93809) ;
#74529=AXIS2_PLACEMENT_3D('',#120354,#93810,#93811) ;
#74530=AXIS2_PLACEMENT_3D('',#120355,#93812,#93813) ;
#74531=AXIS2_PLACEMENT_3D('',#120358,#93815,#93816) ;
#74532=AXIS2_PLACEMENT_3D('',#120359,#93817,#93818) ;
#74533=AXIS2_PLACEMENT_3D('',#120360,#93819,#93820) ;
#74534=AXIS2_PLACEMENT_3D('',#120361,#93821,#93822) ;
#74535=AXIS2_PLACEMENT_3D('',#120362,#93823,#93824) ;
#74536=AXIS2_PLACEMENT_3D('',#120363,#93825,#93826) ;
#74537=AXIS2_PLACEMENT_3D('',#120364,#93827,#93828) ;
#74538=AXIS2_PLACEMENT_3D('',#120365,#93829,#93830) ;
#74539=AXIS2_PLACEMENT_3D('',#120366,#93831,#93832) ;
#74540=AXIS2_PLACEMENT_3D('',#120367,#93833,#93834) ;
#74541=AXIS2_PLACEMENT_3D('',#120368,#93835,#93836) ;
#74542=AXIS2_PLACEMENT_3D('',#120369,#93837,#93838) ;
#74543=AXIS2_PLACEMENT_3D('',#120370,#93839,#93840) ;
#74544=AXIS2_PLACEMENT_3D('',#120371,#93841,#93842) ;
#74545=AXIS2_PLACEMENT_3D('',#120372,#93843,#93844) ;
#74546=AXIS2_PLACEMENT_3D('',#120373,#93845,#93846) ;
#74547=AXIS2_PLACEMENT_3D('',#120375,#93847,#93848) ;
#74548=AXIS2_PLACEMENT_3D('',#120376,#93849,#93850) ;
#74549=AXIS2_PLACEMENT_3D('',#120377,#93851,#93852) ;
#74550=AXIS2_PLACEMENT_3D('',#120378,#93853,#93854) ;
#74551=AXIS2_PLACEMENT_3D('',#120379,#93855,#93856) ;
#74552=AXIS2_PLACEMENT_3D('',#120380,#93857,#93858) ;
#74553=AXIS2_PLACEMENT_3D('',#120381,#93859,#93860) ;
#74554=AXIS2_PLACEMENT_3D('',#120382,#93861,#93862) ;
#74555=AXIS2_PLACEMENT_3D('',#120383,#93863,#93864) ;
#74556=AXIS2_PLACEMENT_3D('',#120384,#93865,#93866) ;
#74557=AXIS2_PLACEMENT_3D('',#120385,#93867,#93868) ;
#74558=AXIS2_PLACEMENT_3D('',#120386,#93869,#93870) ;
#74559=AXIS2_PLACEMENT_3D('',#120387,#93871,#93872) ;
#74560=AXIS2_PLACEMENT_3D('',#120390,#93874,#93875) ;
#74561=AXIS2_PLACEMENT_3D('',#120391,#93876,#93877) ;
#74562=AXIS2_PLACEMENT_3D('',#120392,#93878,#93879) ;
#74563=AXIS2_PLACEMENT_3D('',#120393,#93880,#93881) ;
#74564=AXIS2_PLACEMENT_3D('',#120394,#93882,#93883) ;
#74565=AXIS2_PLACEMENT_3D('',#120395,#93884,#93885) ;
#74566=AXIS2_PLACEMENT_3D('',#120396,#93886,#93887) ;
#74567=AXIS2_PLACEMENT_3D('',#120397,#93888,#93889) ;
#74568=AXIS2_PLACEMENT_3D('',#120398,#93890,#93891) ;
#74569=AXIS2_PLACEMENT_3D('',#120399,#93892,#93893) ;
#74570=AXIS2_PLACEMENT_3D('',#120400,#93894,#93895) ;
#74571=AXIS2_PLACEMENT_3D('',#120401,#93896,#93897) ;
#74572=AXIS2_PLACEMENT_3D('',#120402,#93898,#93899) ;
#74573=AXIS2_PLACEMENT_3D('',#120404,#93900,#93901) ;
#74574=AXIS2_PLACEMENT_3D('',#120405,#93902,#93903) ;
#74575=AXIS2_PLACEMENT_3D('',#120406,#93904,#93905) ;
#74576=AXIS2_PLACEMENT_3D('',#120407,#93906,#93907) ;
#74577=AXIS2_PLACEMENT_3D('',#120408,#93908,#93909) ;
#74578=AXIS2_PLACEMENT_3D('',#120409,#93910,#93911) ;
#74579=AXIS2_PLACEMENT_3D('',#120410,#93912,#93913) ;
#74580=AXIS2_PLACEMENT_3D('',#120411,#93914,#93915) ;
#74581=AXIS2_PLACEMENT_3D('',#120412,#93916,#93917) ;
#74582=AXIS2_PLACEMENT_3D('',#120413,#93918,#93919) ;
#74583=AXIS2_PLACEMENT_3D('',#120414,#93920,#93921) ;
#74584=AXIS2_PLACEMENT_3D('',#120416,#93923,#93924) ;
#74585=AXIS2_PLACEMENT_3D('',#120417,#93925,#93926) ;
#74586=AXIS2_PLACEMENT_3D('',#120418,#93927,#93928) ;
#74587=AXIS2_PLACEMENT_3D('',#120419,#93929,#93930) ;
#74588=AXIS2_PLACEMENT_3D('',#120420,#93931,#93932) ;
#74589=AXIS2_PLACEMENT_3D('',#120421,#93933,#93934) ;
#74590=AXIS2_PLACEMENT_3D('',#120422,#93935,#93936) ;
#74591=AXIS2_PLACEMENT_3D('',#120423,#93937,#93938) ;
#74592=AXIS2_PLACEMENT_3D('',#120424,#93939,#93940) ;
#74593=AXIS2_PLACEMENT_3D('',#120425,#93941,#93942) ;
#74594=AXIS2_PLACEMENT_3D('',#120426,#93943,#93944) ;
#74595=AXIS2_PLACEMENT_3D('',#120427,#93945,#93946) ;
#74596=AXIS2_PLACEMENT_3D('',#120428,#93947,#93948) ;
#74597=AXIS2_PLACEMENT_3D('',#120429,#93949,#93950) ;
#74598=AXIS2_PLACEMENT_3D('',#120430,#93951,#93952) ;
#74599=AXIS2_PLACEMENT_3D('',#120431,#93953,#93954) ;
#74600=AXIS2_PLACEMENT_3D('',#120432,#93955,#93956) ;
#74601=AXIS2_PLACEMENT_3D('',#120433,#93957,#93958) ;
#74602=AXIS2_PLACEMENT_3D('',#120434,#93959,#93960) ;
#74603=AXIS2_PLACEMENT_3D('',#120435,#93961,#93962) ;
#74604=AXIS2_PLACEMENT_3D('',#120436,#93963,#93964) ;
#74605=AXIS2_PLACEMENT_3D('',#120437,#93965,#93966) ;
#74606=AXIS2_PLACEMENT_3D('',#120438,#93967,#93968) ;
#74607=AXIS2_PLACEMENT_3D('',#120439,#93969,#93970) ;
#74608=AXIS2_PLACEMENT_3D('',#120440,#93971,#93972) ;
#74609=AXIS2_PLACEMENT_3D('',#120441,#93973,#93974) ;
#74610=AXIS2_PLACEMENT_3D('',#120442,#93975,#93976) ;
#74611=AXIS2_PLACEMENT_3D('',#120443,#93977,#93978) ;
#74612=AXIS2_PLACEMENT_3D('',#120444,#93979,#93980) ;
#74613=AXIS2_PLACEMENT_3D('',#120445,#93981,#93982) ;
#74614=AXIS2_PLACEMENT_3D('',#120446,#93983,#93984) ;
#74615=AXIS2_PLACEMENT_3D('',#120447,#93985,#93986) ;
#74616=AXIS2_PLACEMENT_3D('',#120448,#93987,#93988) ;
#74617=AXIS2_PLACEMENT_3D('',#120449,#93989,#93990) ;
#74618=AXIS2_PLACEMENT_3D('',#120450,#93991,#93992) ;
#74619=AXIS2_PLACEMENT_3D('',#120451,#93993,#93994) ;
#74620=AXIS2_PLACEMENT_3D('',#120452,#93995,#93996) ;
#74621=AXIS2_PLACEMENT_3D('',#120453,#93997,#93998) ;
#74622=AXIS2_PLACEMENT_3D('',#120454,#93999,#94000) ;
#74623=AXIS2_PLACEMENT_3D('',#120455,#94001,#94002) ;
#74624=AXIS2_PLACEMENT_3D('',#120456,#94003,#94004) ;
#74625=AXIS2_PLACEMENT_3D('',#120457,#94005,#94006) ;
#74626=AXIS2_PLACEMENT_3D('',#120458,#94007,#94008) ;
#74627=AXIS2_PLACEMENT_3D('',#120459,#94009,#94010) ;
#74628=AXIS2_PLACEMENT_3D('',#120460,#94011,#94012) ;
#74629=AXIS2_PLACEMENT_3D('',#120461,#94013,#94014) ;
#74630=AXIS2_PLACEMENT_3D('',#120462,#94015,#94016) ;
#74631=AXIS2_PLACEMENT_3D('',#120463,#94017,#94018) ;
#74632=AXIS2_PLACEMENT_3D('',#120464,#94019,#94020) ;
#74633=AXIS2_PLACEMENT_3D('',#120465,#94021,#94022) ;
#74634=AXIS2_PLACEMENT_3D('',#120466,#94023,#94024) ;
#74635=AXIS2_PLACEMENT_3D('',#120467,#94025,#94026) ;
#74636=AXIS2_PLACEMENT_3D('',#120468,#94027,#94028) ;
#74637=AXIS2_PLACEMENT_3D('',#120469,#94029,#94030) ;
#74638=AXIS2_PLACEMENT_3D('',#120470,#94031,#94032) ;
#74639=AXIS2_PLACEMENT_3D('',#120471,#94033,#94034) ;
#74640=AXIS2_PLACEMENT_3D('',#120472,#94035,#94036) ;
#74641=AXIS2_PLACEMENT_3D('',#120473,#94037,#94038) ;
#74642=AXIS2_PLACEMENT_3D('',#120474,#94039,#94040) ;
#74643=AXIS2_PLACEMENT_3D('',#120475,#94041,#94042) ;
#74644=AXIS2_PLACEMENT_3D('',#120476,#94043,#94044) ;
#74645=AXIS2_PLACEMENT_3D('',#120477,#94045,#94046) ;
#74646=AXIS2_PLACEMENT_3D('',#120478,#94047,#94048) ;
#74647=AXIS2_PLACEMENT_3D('',#120479,#94049,#94050) ;
#74648=AXIS2_PLACEMENT_3D('',#120480,#94051,#94052) ;
#74649=AXIS2_PLACEMENT_3D('',#120481,#94053,#94054) ;
#74650=AXIS2_PLACEMENT_3D('',#120482,#94055,#94056) ;
#74651=AXIS2_PLACEMENT_3D('',#120484,#94057,#94058) ;
#74652=AXIS2_PLACEMENT_3D('',#120485,#94059,#94060) ;
#74653=AXIS2_PLACEMENT_3D('',#120486,#94061,#94062) ;
#74654=AXIS2_PLACEMENT_3D('',#120487,#94063,#94064) ;
#74655=AXIS2_PLACEMENT_3D('',#120488,#94065,#94066) ;
#74656=AXIS2_PLACEMENT_3D('',#120489,#94067,#94068) ;
#74657=AXIS2_PLACEMENT_3D('',#120490,#94069,#94070) ;
#74658=AXIS2_PLACEMENT_3D('',#120491,#94071,#94072) ;
#74659=AXIS2_PLACEMENT_3D('',#120492,#94073,#94074) ;
#74660=AXIS2_PLACEMENT_3D('',#120503,#94076,#94077) ;
#74661=AXIS2_PLACEMENT_3D('',#120560,#94079,#94080) ;
#74662=AXIS2_PLACEMENT_3D('',#120561,#94081,#94082) ;
#74663=AXIS2_PLACEMENT_3D('',#120562,#94083,#94084) ;
#74664=AXIS2_PLACEMENT_3D('',#120563,#94085,#94086) ;
#74665=AXIS2_PLACEMENT_3D('',#120564,#94087,#94088) ;
#74666=AXIS2_PLACEMENT_3D('',#120565,#94089,#94090) ;
#74667=AXIS2_PLACEMENT_3D('',#120566,#94091,#94092) ;
#74668=AXIS2_PLACEMENT_3D('',#120567,#94093,#94094) ;
#74669=AXIS2_PLACEMENT_3D('',#120568,#94095,#94096) ;
#74670=AXIS2_PLACEMENT_3D('',#120569,#94097,#94098) ;
#74671=AXIS2_PLACEMENT_3D('',#120570,#94099,#94100) ;
#74672=AXIS2_PLACEMENT_3D('',#120571,#94101,#94102) ;
#74673=AXIS2_PLACEMENT_3D('',#120572,#94103,#94104) ;
#74674=AXIS2_PLACEMENT_3D('',#120573,#94105,#94106) ;
#74675=AXIS2_PLACEMENT_3D('',#120574,#94107,#94108) ;
#74676=AXIS2_PLACEMENT_3D('',#120575,#94109,#94110) ;
#74677=AXIS2_PLACEMENT_3D('',#120576,#94111,#94112) ;
#74678=AXIS2_PLACEMENT_3D('',#120577,#94113,#94114) ;
#74679=AXIS2_PLACEMENT_3D('',#120578,#94115,#94116) ;
#74680=AXIS2_PLACEMENT_3D('',#120579,#94117,#94118) ;
#74681=AXIS2_PLACEMENT_3D('',#120580,#94119,#94120) ;
#74682=AXIS2_PLACEMENT_3D('',#120581,#94121,#94122) ;
#74683=AXIS2_PLACEMENT_3D('',#120582,#94123,#94124) ;
#74684=AXIS2_PLACEMENT_3D('',#120585,#94126,#94127) ;
#74685=AXIS2_PLACEMENT_3D('',#120586,#94128,#94129) ;
#74686=AXIS2_PLACEMENT_3D('',#120587,#94130,#94131) ;
#74687=AXIS2_PLACEMENT_3D('',#120588,#94132,#94133) ;
#74688=AXIS2_PLACEMENT_3D('',#120589,#94134,#94135) ;
#74689=AXIS2_PLACEMENT_3D('',#120590,#94136,#94137) ;
#74690=AXIS2_PLACEMENT_3D('',#120591,#94138,#94139) ;
#74691=AXIS2_PLACEMENT_3D('',#120592,#94140,#94141) ;
#74692=AXIS2_PLACEMENT_3D('',#120593,#94142,#94143) ;
#74693=AXIS2_PLACEMENT_3D('',#120594,#94144,#94145) ;
#74694=AXIS2_PLACEMENT_3D('',#120595,#94146,#94147) ;
#74695=AXIS2_PLACEMENT_3D('',#120596,#94148,#94149) ;
#74696=AXIS2_PLACEMENT_3D('',#120597,#94150,#94151) ;
#74697=AXIS2_PLACEMENT_3D('',#120598,#94152,#94153) ;
#74698=AXIS2_PLACEMENT_3D('',#120599,#94154,#94155) ;
#74699=AXIS2_PLACEMENT_3D('',#120600,#94156,#94157) ;
#74700=AXIS2_PLACEMENT_3D('',#120602,#94158,#94159) ;
#74701=AXIS2_PLACEMENT_3D('',#120603,#94160,#94161) ;
#74702=AXIS2_PLACEMENT_3D('',#120604,#94162,#94163) ;
#74703=AXIS2_PLACEMENT_3D('',#120605,#94164,#94165) ;
#74704=AXIS2_PLACEMENT_3D('',#120606,#94166,#94167) ;
#74705=AXIS2_PLACEMENT_3D('',#120607,#94168,#94169) ;
#74706=AXIS2_PLACEMENT_3D('',#120608,#94170,#94171) ;
#74707=AXIS2_PLACEMENT_3D('',#120609,#94172,#94173) ;
#74708=AXIS2_PLACEMENT_3D('',#120610,#94174,#94175) ;
#74709=AXIS2_PLACEMENT_3D('',#120611,#94176,#94177) ;
#74710=AXIS2_PLACEMENT_3D('',#120612,#94178,#94179) ;
#74711=AXIS2_PLACEMENT_3D('',#120613,#94180,#94181) ;
#74712=AXIS2_PLACEMENT_3D('',#120614,#94182,#94183) ;
#74713=AXIS2_PLACEMENT_3D('',#120617,#94185,#94186) ;
#74714=AXIS2_PLACEMENT_3D('',#120618,#94187,#94188) ;
#74715=AXIS2_PLACEMENT_3D('',#120619,#94189,#94190) ;
#74716=AXIS2_PLACEMENT_3D('',#120620,#94191,#94192) ;
#74717=AXIS2_PLACEMENT_3D('',#120621,#94193,#94194) ;
#74718=AXIS2_PLACEMENT_3D('',#120622,#94195,#94196) ;
#74719=AXIS2_PLACEMENT_3D('',#120623,#94197,#94198) ;
#74720=AXIS2_PLACEMENT_3D('',#120624,#94199,#94200) ;
#74721=AXIS2_PLACEMENT_3D('',#120625,#94201,#94202) ;
#74722=AXIS2_PLACEMENT_3D('',#120626,#94203,#94204) ;
#74723=AXIS2_PLACEMENT_3D('',#120627,#94205,#94206) ;
#74724=AXIS2_PLACEMENT_3D('',#120628,#94207,#94208) ;
#74725=AXIS2_PLACEMENT_3D('',#120629,#94209,#94210) ;
#74726=AXIS2_PLACEMENT_3D('',#120631,#94211,#94212) ;
#74727=AXIS2_PLACEMENT_3D('',#120632,#94213,#94214) ;
#74728=AXIS2_PLACEMENT_3D('',#120633,#94215,#94216) ;
#74729=AXIS2_PLACEMENT_3D('',#120634,#94217,#94218) ;
#74730=AXIS2_PLACEMENT_3D('',#120635,#94219,#94220) ;
#74731=AXIS2_PLACEMENT_3D('',#120636,#94221,#94222) ;
#74732=AXIS2_PLACEMENT_3D('',#120637,#94223,#94224) ;
#74733=AXIS2_PLACEMENT_3D('',#120638,#94225,#94226) ;
#74734=AXIS2_PLACEMENT_3D('',#120639,#94227,#94228) ;
#74735=AXIS2_PLACEMENT_3D('',#120640,#94229,#94230) ;
#74736=AXIS2_PLACEMENT_3D('',#120641,#94231,#94232) ;
#74737=AXIS2_PLACEMENT_3D('',#120643,#94234,#94235) ;
#74738=AXIS2_PLACEMENT_3D('',#120644,#94236,#94237) ;
#74739=AXIS2_PLACEMENT_3D('',#120645,#94238,#94239) ;
#74740=AXIS2_PLACEMENT_3D('',#120646,#94240,#94241) ;
#74741=AXIS2_PLACEMENT_3D('',#120647,#94242,#94243) ;
#74742=AXIS2_PLACEMENT_3D('',#120648,#94244,#94245) ;
#74743=AXIS2_PLACEMENT_3D('',#120649,#94246,#94247) ;
#74744=AXIS2_PLACEMENT_3D('',#120650,#94248,#94249) ;
#74745=AXIS2_PLACEMENT_3D('',#120651,#94250,#94251) ;
#74746=AXIS2_PLACEMENT_3D('',#120652,#94252,#94253) ;
#74747=AXIS2_PLACEMENT_3D('',#120653,#94254,#94255) ;
#74748=AXIS2_PLACEMENT_3D('',#120654,#94256,#94257) ;
#74749=AXIS2_PLACEMENT_3D('',#120655,#94258,#94259) ;
#74750=AXIS2_PLACEMENT_3D('',#120656,#94260,#94261) ;
#74751=AXIS2_PLACEMENT_3D('',#120657,#94262,#94263) ;
#74752=AXIS2_PLACEMENT_3D('',#120658,#94264,#94265) ;
#74753=AXIS2_PLACEMENT_3D('',#120659,#94266,#94267) ;
#74754=AXIS2_PLACEMENT_3D('',#120660,#94268,#94269) ;
#74755=AXIS2_PLACEMENT_3D('',#120661,#94270,#94271) ;
#74756=AXIS2_PLACEMENT_3D('',#120662,#94272,#94273) ;
#74757=AXIS2_PLACEMENT_3D('',#120663,#94274,#94275) ;
#74758=AXIS2_PLACEMENT_3D('',#120664,#94276,#94277) ;
#74759=AXIS2_PLACEMENT_3D('',#120665,#94278,#94279) ;
#74760=AXIS2_PLACEMENT_3D('',#120666,#94280,#94281) ;
#74761=AXIS2_PLACEMENT_3D('',#120667,#94282,#94283) ;
#74762=AXIS2_PLACEMENT_3D('',#120668,#94284,#94285) ;
#74763=AXIS2_PLACEMENT_3D('',#120669,#94286,#94287) ;
#74764=AXIS2_PLACEMENT_3D('',#120670,#94288,#94289) ;
#74765=AXIS2_PLACEMENT_3D('',#120671,#94290,#94291) ;
#74766=AXIS2_PLACEMENT_3D('',#120672,#94292,#94293) ;
#74767=AXIS2_PLACEMENT_3D('',#120673,#94294,#94295) ;
#74768=AXIS2_PLACEMENT_3D('',#120674,#94296,#94297) ;
#74769=AXIS2_PLACEMENT_3D('',#120675,#94298,#94299) ;
#74770=AXIS2_PLACEMENT_3D('',#120676,#94300,#94301) ;
#74771=AXIS2_PLACEMENT_3D('',#120677,#94302,#94303) ;
#74772=AXIS2_PLACEMENT_3D('',#120678,#94304,#94305) ;
#74773=AXIS2_PLACEMENT_3D('',#120679,#94306,#94307) ;
#74774=AXIS2_PLACEMENT_3D('',#120680,#94308,#94309) ;
#74775=AXIS2_PLACEMENT_3D('',#120681,#94310,#94311) ;
#74776=AXIS2_PLACEMENT_3D('',#120682,#94312,#94313) ;
#74777=AXIS2_PLACEMENT_3D('',#120683,#94314,#94315) ;
#74778=AXIS2_PLACEMENT_3D('',#120684,#94316,#94317) ;
#74779=AXIS2_PLACEMENT_3D('',#120685,#94318,#94319) ;
#74780=AXIS2_PLACEMENT_3D('',#120686,#94320,#94321) ;
#74781=AXIS2_PLACEMENT_3D('',#120687,#94322,#94323) ;
#74782=AXIS2_PLACEMENT_3D('',#120688,#94324,#94325) ;
#74783=AXIS2_PLACEMENT_3D('',#120689,#94326,#94327) ;
#74784=AXIS2_PLACEMENT_3D('',#120690,#94328,#94329) ;
#74785=AXIS2_PLACEMENT_3D('',#120691,#94330,#94331) ;
#74786=AXIS2_PLACEMENT_3D('',#120692,#94332,#94333) ;
#74787=AXIS2_PLACEMENT_3D('',#120693,#94334,#94335) ;
#74788=AXIS2_PLACEMENT_3D('',#120694,#94336,#94337) ;
#74789=AXIS2_PLACEMENT_3D('',#120695,#94338,#94339) ;
#74790=AXIS2_PLACEMENT_3D('',#120696,#94340,#94341) ;
#74791=AXIS2_PLACEMENT_3D('',#120697,#94342,#94343) ;
#74792=AXIS2_PLACEMENT_3D('',#120698,#94344,#94345) ;
#74793=AXIS2_PLACEMENT_3D('',#120699,#94346,#94347) ;
#74794=AXIS2_PLACEMENT_3D('',#120700,#94348,#94349) ;
#74795=AXIS2_PLACEMENT_3D('',#120701,#94350,#94351) ;
#74796=AXIS2_PLACEMENT_3D('',#120702,#94352,#94353) ;
#74797=AXIS2_PLACEMENT_3D('',#120703,#94354,#94355) ;
#74798=AXIS2_PLACEMENT_3D('',#120704,#94356,#94357) ;
#74799=AXIS2_PLACEMENT_3D('',#120705,#94358,#94359) ;
#74800=AXIS2_PLACEMENT_3D('',#120706,#94360,#94361) ;
#74801=AXIS2_PLACEMENT_3D('',#120707,#94362,#94363) ;
#74802=AXIS2_PLACEMENT_3D('',#120708,#94364,#94365) ;
#74803=AXIS2_PLACEMENT_3D('',#120709,#94366,#94367) ;
#74804=AXIS2_PLACEMENT_3D('',#120711,#94368,#94369) ;
#74805=AXIS2_PLACEMENT_3D('',#120712,#94370,#94371) ;
#74806=AXIS2_PLACEMENT_3D('',#120713,#94372,#94373) ;
#74807=AXIS2_PLACEMENT_3D('',#120714,#94374,#94375) ;
#74808=AXIS2_PLACEMENT_3D('',#120715,#94376,#94377) ;
#74809=AXIS2_PLACEMENT_3D('',#120716,#94378,#94379) ;
#74810=AXIS2_PLACEMENT_3D('',#120717,#94380,#94381) ;
#74811=AXIS2_PLACEMENT_3D('',#120718,#94382,#94383) ;
#74812=AXIS2_PLACEMENT_3D('',#120719,#94384,#94385) ;
#74813=AXIS2_PLACEMENT_3D('',#120730,#94387,#94388) ;
#74814=AXIS2_PLACEMENT_3D('',#120787,#94390,#94391) ;
#74815=AXIS2_PLACEMENT_3D('',#120788,#94392,#94393) ;
#74816=AXIS2_PLACEMENT_3D('',#120789,#94394,#94395) ;
#74817=AXIS2_PLACEMENT_3D('',#120790,#94396,#94397) ;
#74818=AXIS2_PLACEMENT_3D('',#120791,#94398,#94399) ;
#74819=AXIS2_PLACEMENT_3D('',#120792,#94400,#94401) ;
#74820=AXIS2_PLACEMENT_3D('',#120793,#94402,#94403) ;
#74821=AXIS2_PLACEMENT_3D('',#120794,#94404,#94405) ;
#74822=AXIS2_PLACEMENT_3D('',#120795,#94406,#94407) ;
#74823=AXIS2_PLACEMENT_3D('',#120796,#94408,#94409) ;
#74824=AXIS2_PLACEMENT_3D('',#120797,#94410,#94411) ;
#74825=AXIS2_PLACEMENT_3D('',#120798,#94412,#94413) ;
#74826=AXIS2_PLACEMENT_3D('',#120799,#94414,#94415) ;
#74827=AXIS2_PLACEMENT_3D('',#120800,#94416,#94417) ;
#74828=AXIS2_PLACEMENT_3D('',#120801,#94418,#94419) ;
#74829=AXIS2_PLACEMENT_3D('',#120802,#94420,#94421) ;
#74830=AXIS2_PLACEMENT_3D('',#120803,#94422,#94423) ;
#74831=AXIS2_PLACEMENT_3D('',#120804,#94424,#94425) ;
#74832=AXIS2_PLACEMENT_3D('',#120805,#94426,#94427) ;
#74833=AXIS2_PLACEMENT_3D('',#120806,#94428,#94429) ;
#74834=AXIS2_PLACEMENT_3D('',#120807,#94430,#94431) ;
#74835=AXIS2_PLACEMENT_3D('',#120808,#94432,#94433) ;
#74836=AXIS2_PLACEMENT_3D('',#120809,#94434,#94435) ;
#74837=AXIS2_PLACEMENT_3D('',#120812,#94437,#94438) ;
#74838=AXIS2_PLACEMENT_3D('',#120813,#94439,#94440) ;
#74839=AXIS2_PLACEMENT_3D('',#120814,#94441,#94442) ;
#74840=AXIS2_PLACEMENT_3D('',#120815,#94443,#94444) ;
#74841=AXIS2_PLACEMENT_3D('',#120816,#94445,#94446) ;
#74842=AXIS2_PLACEMENT_3D('',#120817,#94447,#94448) ;
#74843=AXIS2_PLACEMENT_3D('',#120818,#94449,#94450) ;
#74844=AXIS2_PLACEMENT_3D('',#120819,#94451,#94452) ;
#74845=AXIS2_PLACEMENT_3D('',#120820,#94453,#94454) ;
#74846=AXIS2_PLACEMENT_3D('',#120821,#94455,#94456) ;
#74847=AXIS2_PLACEMENT_3D('',#120822,#94457,#94458) ;
#74848=AXIS2_PLACEMENT_3D('',#120823,#94459,#94460) ;
#74849=AXIS2_PLACEMENT_3D('',#120824,#94461,#94462) ;
#74850=AXIS2_PLACEMENT_3D('',#120825,#94463,#94464) ;
#74851=AXIS2_PLACEMENT_3D('',#120826,#94465,#94466) ;
#74852=AXIS2_PLACEMENT_3D('',#120827,#94467,#94468) ;
#74853=AXIS2_PLACEMENT_3D('',#120829,#94469,#94470) ;
#74854=AXIS2_PLACEMENT_3D('',#120830,#94471,#94472) ;
#74855=AXIS2_PLACEMENT_3D('',#120831,#94473,#94474) ;
#74856=AXIS2_PLACEMENT_3D('',#120832,#94475,#94476) ;
#74857=AXIS2_PLACEMENT_3D('',#120833,#94477,#94478) ;
#74858=AXIS2_PLACEMENT_3D('',#120834,#94479,#94480) ;
#74859=AXIS2_PLACEMENT_3D('',#120835,#94481,#94482) ;
#74860=AXIS2_PLACEMENT_3D('',#120836,#94483,#94484) ;
#74861=AXIS2_PLACEMENT_3D('',#120837,#94485,#94486) ;
#74862=AXIS2_PLACEMENT_3D('',#120838,#94487,#94488) ;
#74863=AXIS2_PLACEMENT_3D('',#120839,#94489,#94490) ;
#74864=AXIS2_PLACEMENT_3D('',#120840,#94491,#94492) ;
#74865=AXIS2_PLACEMENT_3D('',#120841,#94493,#94494) ;
#74866=AXIS2_PLACEMENT_3D('',#120844,#94496,#94497) ;
#74867=AXIS2_PLACEMENT_3D('',#120845,#94498,#94499) ;
#74868=AXIS2_PLACEMENT_3D('',#120846,#94500,#94501) ;
#74869=AXIS2_PLACEMENT_3D('',#120847,#94502,#94503) ;
#74870=AXIS2_PLACEMENT_3D('',#120848,#94504,#94505) ;
#74871=AXIS2_PLACEMENT_3D('',#120849,#94506,#94507) ;
#74872=AXIS2_PLACEMENT_3D('',#120850,#94508,#94509) ;
#74873=AXIS2_PLACEMENT_3D('',#120851,#94510,#94511) ;
#74874=AXIS2_PLACEMENT_3D('',#120852,#94512,#94513) ;
#74875=AXIS2_PLACEMENT_3D('',#120853,#94514,#94515) ;
#74876=AXIS2_PLACEMENT_3D('',#120854,#94516,#94517) ;
#74877=AXIS2_PLACEMENT_3D('',#120855,#94518,#94519) ;
#74878=AXIS2_PLACEMENT_3D('',#120856,#94520,#94521) ;
#74879=AXIS2_PLACEMENT_3D('',#120858,#94522,#94523) ;
#74880=AXIS2_PLACEMENT_3D('',#120859,#94524,#94525) ;
#74881=AXIS2_PLACEMENT_3D('',#120860,#94526,#94527) ;
#74882=AXIS2_PLACEMENT_3D('',#120861,#94528,#94529) ;
#74883=AXIS2_PLACEMENT_3D('',#120862,#94530,#94531) ;
#74884=AXIS2_PLACEMENT_3D('',#120863,#94532,#94533) ;
#74885=AXIS2_PLACEMENT_3D('',#120864,#94534,#94535) ;
#74886=AXIS2_PLACEMENT_3D('',#120865,#94536,#94537) ;
#74887=AXIS2_PLACEMENT_3D('',#120866,#94538,#94539) ;
#74888=AXIS2_PLACEMENT_3D('',#120867,#94540,#94541) ;
#74889=AXIS2_PLACEMENT_3D('',#120868,#94542,#94543) ;
#74890=AXIS2_PLACEMENT_3D('',#120870,#94545,#94546) ;
#74891=AXIS2_PLACEMENT_3D('',#120871,#94547,#94548) ;
#74892=AXIS2_PLACEMENT_3D('',#120872,#94549,#94550) ;
#74893=AXIS2_PLACEMENT_3D('',#120873,#94551,#94552) ;
#74894=AXIS2_PLACEMENT_3D('',#120874,#94553,#94554) ;
#74895=AXIS2_PLACEMENT_3D('',#120875,#94555,#94556) ;
#74896=AXIS2_PLACEMENT_3D('',#120876,#94557,#94558) ;
#74897=AXIS2_PLACEMENT_3D('',#120877,#94559,#94560) ;
#74898=AXIS2_PLACEMENT_3D('',#120878,#94561,#94562) ;
#74899=AXIS2_PLACEMENT_3D('',#120879,#94563,#94564) ;
#74900=AXIS2_PLACEMENT_3D('',#120880,#94565,#94566) ;
#74901=AXIS2_PLACEMENT_3D('',#120881,#94567,#94568) ;
#74902=AXIS2_PLACEMENT_3D('',#120882,#94569,#94570) ;
#74903=AXIS2_PLACEMENT_3D('',#120883,#94571,#94572) ;
#74904=AXIS2_PLACEMENT_3D('',#120884,#94573,#94574) ;
#74905=AXIS2_PLACEMENT_3D('',#120885,#94575,#94576) ;
#74906=AXIS2_PLACEMENT_3D('',#120886,#94577,#94578) ;
#74907=AXIS2_PLACEMENT_3D('',#120887,#94579,#94580) ;
#74908=AXIS2_PLACEMENT_3D('',#120888,#94581,#94582) ;
#74909=AXIS2_PLACEMENT_3D('',#120889,#94583,#94584) ;
#74910=AXIS2_PLACEMENT_3D('',#120890,#94585,#94586) ;
#74911=AXIS2_PLACEMENT_3D('',#120891,#94587,#94588) ;
#74912=AXIS2_PLACEMENT_3D('',#120892,#94589,#94590) ;
#74913=AXIS2_PLACEMENT_3D('',#120893,#94591,#94592) ;
#74914=AXIS2_PLACEMENT_3D('',#120894,#94593,#94594) ;
#74915=AXIS2_PLACEMENT_3D('',#120895,#94595,#94596) ;
#74916=AXIS2_PLACEMENT_3D('',#120896,#94597,#94598) ;
#74917=AXIS2_PLACEMENT_3D('',#120897,#94599,#94600) ;
#74918=AXIS2_PLACEMENT_3D('',#120898,#94601,#94602) ;
#74919=AXIS2_PLACEMENT_3D('',#120899,#94603,#94604) ;
#74920=AXIS2_PLACEMENT_3D('',#120900,#94605,#94606) ;
#74921=AXIS2_PLACEMENT_3D('',#120901,#94607,#94608) ;
#74922=AXIS2_PLACEMENT_3D('',#120902,#94609,#94610) ;
#74923=AXIS2_PLACEMENT_3D('',#120903,#94611,#94612) ;
#74924=AXIS2_PLACEMENT_3D('',#120904,#94613,#94614) ;
#74925=AXIS2_PLACEMENT_3D('',#120905,#94615,#94616) ;
#74926=AXIS2_PLACEMENT_3D('',#120906,#94617,#94618) ;
#74927=AXIS2_PLACEMENT_3D('',#120907,#94619,#94620) ;
#74928=AXIS2_PLACEMENT_3D('',#120908,#94621,#94622) ;
#74929=AXIS2_PLACEMENT_3D('',#120909,#94623,#94624) ;
#74930=AXIS2_PLACEMENT_3D('',#120910,#94625,#94626) ;
#74931=AXIS2_PLACEMENT_3D('',#120911,#94627,#94628) ;
#74932=AXIS2_PLACEMENT_3D('',#120912,#94629,#94630) ;
#74933=AXIS2_PLACEMENT_3D('',#120913,#94631,#94632) ;
#74934=AXIS2_PLACEMENT_3D('',#120914,#94633,#94634) ;
#74935=AXIS2_PLACEMENT_3D('',#120915,#94635,#94636) ;
#74936=AXIS2_PLACEMENT_3D('',#120916,#94637,#94638) ;
#74937=AXIS2_PLACEMENT_3D('',#120917,#94639,#94640) ;
#74938=AXIS2_PLACEMENT_3D('',#120918,#94641,#94642) ;
#74939=AXIS2_PLACEMENT_3D('',#120919,#94643,#94644) ;
#74940=AXIS2_PLACEMENT_3D('',#120920,#94645,#94646) ;
#74941=AXIS2_PLACEMENT_3D('',#120921,#94647,#94648) ;
#74942=AXIS2_PLACEMENT_3D('',#120922,#94649,#94650) ;
#74943=AXIS2_PLACEMENT_3D('',#120923,#94651,#94652) ;
#74944=AXIS2_PLACEMENT_3D('',#120924,#94653,#94654) ;
#74945=AXIS2_PLACEMENT_3D('',#120925,#94655,#94656) ;
#74946=AXIS2_PLACEMENT_3D('',#120926,#94657,#94658) ;
#74947=AXIS2_PLACEMENT_3D('',#120927,#94659,#94660) ;
#74948=AXIS2_PLACEMENT_3D('',#120928,#94661,#94662) ;
#74949=AXIS2_PLACEMENT_3D('',#120929,#94663,#94664) ;
#74950=AXIS2_PLACEMENT_3D('',#120930,#94665,#94666) ;
#74951=AXIS2_PLACEMENT_3D('',#120931,#94667,#94668) ;
#74952=AXIS2_PLACEMENT_3D('',#120932,#94669,#94670) ;
#74953=AXIS2_PLACEMENT_3D('',#120933,#94671,#94672) ;
#74954=AXIS2_PLACEMENT_3D('',#120934,#94673,#94674) ;
#74955=AXIS2_PLACEMENT_3D('',#120935,#94675,#94676) ;
#74956=AXIS2_PLACEMENT_3D('',#120936,#94677,#94678) ;
#74957=AXIS2_PLACEMENT_3D('',#120938,#94679,#94680) ;
#74958=AXIS2_PLACEMENT_3D('',#120939,#94681,#94682) ;
#74959=AXIS2_PLACEMENT_3D('',#120940,#94683,#94684) ;
#74960=AXIS2_PLACEMENT_3D('',#120941,#94685,#94686) ;
#74961=AXIS2_PLACEMENT_3D('',#120942,#94687,#94688) ;
#74962=AXIS2_PLACEMENT_3D('',#120943,#94689,#94690) ;
#74963=AXIS2_PLACEMENT_3D('',#120944,#94691,#94692) ;
#74964=AXIS2_PLACEMENT_3D('',#120945,#94693,#94694) ;
#74965=AXIS2_PLACEMENT_3D('',#120946,#94695,#94696) ;
#74966=AXIS2_PLACEMENT_3D('',#120957,#94698,#94699) ;
#74967=AXIS2_PLACEMENT_3D('',#121014,#94701,#94702) ;
#74968=AXIS2_PLACEMENT_3D('',#121015,#94703,#94704) ;
#74969=AXIS2_PLACEMENT_3D('',#121016,#94705,#94706) ;
#74970=AXIS2_PLACEMENT_3D('',#121017,#94707,#94708) ;
#74971=AXIS2_PLACEMENT_3D('',#121018,#94709,#94710) ;
#74972=AXIS2_PLACEMENT_3D('',#121019,#94711,#94712) ;
#74973=AXIS2_PLACEMENT_3D('',#121020,#94713,#94714) ;
#74974=AXIS2_PLACEMENT_3D('',#121021,#94715,#94716) ;
#74975=AXIS2_PLACEMENT_3D('',#121022,#94717,#94718) ;
#74976=AXIS2_PLACEMENT_3D('',#121023,#94719,#94720) ;
#74977=AXIS2_PLACEMENT_3D('',#121024,#94721,#94722) ;
#74978=AXIS2_PLACEMENT_3D('',#121025,#94723,#94724) ;
#74979=AXIS2_PLACEMENT_3D('',#121026,#94725,#94726) ;
#74980=AXIS2_PLACEMENT_3D('',#121027,#94727,#94728) ;
#74981=AXIS2_PLACEMENT_3D('',#121028,#94729,#94730) ;
#74982=AXIS2_PLACEMENT_3D('',#121029,#94731,#94732) ;
#74983=AXIS2_PLACEMENT_3D('',#121030,#94733,#94734) ;
#74984=AXIS2_PLACEMENT_3D('',#121031,#94735,#94736) ;
#74985=AXIS2_PLACEMENT_3D('',#121032,#94737,#94738) ;
#74986=AXIS2_PLACEMENT_3D('',#121033,#94739,#94740) ;
#74987=AXIS2_PLACEMENT_3D('',#121034,#94741,#94742) ;
#74988=AXIS2_PLACEMENT_3D('',#121035,#94743,#94744) ;
#74989=AXIS2_PLACEMENT_3D('',#121036,#94745,#94746) ;
#74990=AXIS2_PLACEMENT_3D('',#121039,#94748,#94749) ;
#74991=AXIS2_PLACEMENT_3D('',#121040,#94750,#94751) ;
#74992=AXIS2_PLACEMENT_3D('',#121041,#94752,#94753) ;
#74993=AXIS2_PLACEMENT_3D('',#121042,#94754,#94755) ;
#74994=AXIS2_PLACEMENT_3D('',#121043,#94756,#94757) ;
#74995=AXIS2_PLACEMENT_3D('',#121044,#94758,#94759) ;
#74996=AXIS2_PLACEMENT_3D('',#121045,#94760,#94761) ;
#74997=AXIS2_PLACEMENT_3D('',#121046,#94762,#94763) ;
#74998=AXIS2_PLACEMENT_3D('',#121047,#94764,#94765) ;
#74999=AXIS2_PLACEMENT_3D('',#121048,#94766,#94767) ;
#75000=AXIS2_PLACEMENT_3D('',#121049,#94768,#94769) ;
#75001=AXIS2_PLACEMENT_3D('',#121050,#94770,#94771) ;
#75002=AXIS2_PLACEMENT_3D('',#121051,#94772,#94773) ;
#75003=AXIS2_PLACEMENT_3D('',#121052,#94774,#94775) ;
#75004=AXIS2_PLACEMENT_3D('',#121053,#94776,#94777) ;
#75005=AXIS2_PLACEMENT_3D('',#121054,#94778,#94779) ;
#75006=AXIS2_PLACEMENT_3D('',#121056,#94780,#94781) ;
#75007=AXIS2_PLACEMENT_3D('',#121057,#94782,#94783) ;
#75008=AXIS2_PLACEMENT_3D('',#121058,#94784,#94785) ;
#75009=AXIS2_PLACEMENT_3D('',#121059,#94786,#94787) ;
#75010=AXIS2_PLACEMENT_3D('',#121060,#94788,#94789) ;
#75011=AXIS2_PLACEMENT_3D('',#121061,#94790,#94791) ;
#75012=AXIS2_PLACEMENT_3D('',#121062,#94792,#94793) ;
#75013=AXIS2_PLACEMENT_3D('',#121063,#94794,#94795) ;
#75014=AXIS2_PLACEMENT_3D('',#121064,#94796,#94797) ;
#75015=AXIS2_PLACEMENT_3D('',#121065,#94798,#94799) ;
#75016=AXIS2_PLACEMENT_3D('',#121066,#94800,#94801) ;
#75017=AXIS2_PLACEMENT_3D('',#121067,#94802,#94803) ;
#75018=AXIS2_PLACEMENT_3D('',#121068,#94804,#94805) ;
#75019=AXIS2_PLACEMENT_3D('',#121071,#94807,#94808) ;
#75020=AXIS2_PLACEMENT_3D('',#121072,#94809,#94810) ;
#75021=AXIS2_PLACEMENT_3D('',#121073,#94811,#94812) ;
#75022=AXIS2_PLACEMENT_3D('',#121074,#94813,#94814) ;
#75023=AXIS2_PLACEMENT_3D('',#121075,#94815,#94816) ;
#75024=AXIS2_PLACEMENT_3D('',#121076,#94817,#94818) ;
#75025=AXIS2_PLACEMENT_3D('',#121077,#94819,#94820) ;
#75026=AXIS2_PLACEMENT_3D('',#121078,#94821,#94822) ;
#75027=AXIS2_PLACEMENT_3D('',#121079,#94823,#94824) ;
#75028=AXIS2_PLACEMENT_3D('',#121080,#94825,#94826) ;
#75029=AXIS2_PLACEMENT_3D('',#121081,#94827,#94828) ;
#75030=AXIS2_PLACEMENT_3D('',#121082,#94829,#94830) ;
#75031=AXIS2_PLACEMENT_3D('',#121083,#94831,#94832) ;
#75032=AXIS2_PLACEMENT_3D('',#121085,#94833,#94834) ;
#75033=AXIS2_PLACEMENT_3D('',#121086,#94835,#94836) ;
#75034=AXIS2_PLACEMENT_3D('',#121087,#94837,#94838) ;
#75035=AXIS2_PLACEMENT_3D('',#121088,#94839,#94840) ;
#75036=AXIS2_PLACEMENT_3D('',#121089,#94841,#94842) ;
#75037=AXIS2_PLACEMENT_3D('',#121090,#94843,#94844) ;
#75038=AXIS2_PLACEMENT_3D('',#121091,#94845,#94846) ;
#75039=AXIS2_PLACEMENT_3D('',#121092,#94847,#94848) ;
#75040=AXIS2_PLACEMENT_3D('',#121093,#94849,#94850) ;
#75041=AXIS2_PLACEMENT_3D('',#121094,#94851,#94852) ;
#75042=AXIS2_PLACEMENT_3D('',#121095,#94853,#94854) ;
#75043=AXIS2_PLACEMENT_3D('',#121097,#94856,#94857) ;
#75044=AXIS2_PLACEMENT_3D('',#121098,#94858,#94859) ;
#75045=AXIS2_PLACEMENT_3D('',#121099,#94860,#94861) ;
#75046=AXIS2_PLACEMENT_3D('',#121100,#94862,#94863) ;
#75047=AXIS2_PLACEMENT_3D('',#121101,#94864,#94865) ;
#75048=AXIS2_PLACEMENT_3D('',#121102,#94866,#94867) ;
#75049=AXIS2_PLACEMENT_3D('',#121103,#94868,#94869) ;
#75050=AXIS2_PLACEMENT_3D('',#121104,#94870,#94871) ;
#75051=AXIS2_PLACEMENT_3D('',#121105,#94872,#94873) ;
#75052=AXIS2_PLACEMENT_3D('',#121106,#94874,#94875) ;
#75053=AXIS2_PLACEMENT_3D('',#121107,#94876,#94877) ;
#75054=AXIS2_PLACEMENT_3D('',#121108,#94878,#94879) ;
#75055=AXIS2_PLACEMENT_3D('',#121109,#94880,#94881) ;
#75056=AXIS2_PLACEMENT_3D('',#121110,#94882,#94883) ;
#75057=AXIS2_PLACEMENT_3D('',#121111,#94884,#94885) ;
#75058=AXIS2_PLACEMENT_3D('',#121112,#94886,#94887) ;
#75059=AXIS2_PLACEMENT_3D('',#121113,#94888,#94889) ;
#75060=AXIS2_PLACEMENT_3D('',#121114,#94890,#94891) ;
#75061=AXIS2_PLACEMENT_3D('',#121115,#94892,#94893) ;
#75062=AXIS2_PLACEMENT_3D('',#121116,#94894,#94895) ;
#75063=AXIS2_PLACEMENT_3D('',#121117,#94896,#94897) ;
#75064=AXIS2_PLACEMENT_3D('',#121118,#94898,#94899) ;
#75065=AXIS2_PLACEMENT_3D('',#121119,#94900,#94901) ;
#75066=AXIS2_PLACEMENT_3D('',#121120,#94902,#94903) ;
#75067=AXIS2_PLACEMENT_3D('',#121121,#94904,#94905) ;
#75068=AXIS2_PLACEMENT_3D('',#121122,#94906,#94907) ;
#75069=AXIS2_PLACEMENT_3D('',#121123,#94908,#94909) ;
#75070=AXIS2_PLACEMENT_3D('',#121124,#94910,#94911) ;
#75071=AXIS2_PLACEMENT_3D('',#121125,#94912,#94913) ;
#75072=AXIS2_PLACEMENT_3D('',#121126,#94914,#94915) ;
#75073=AXIS2_PLACEMENT_3D('',#121127,#94916,#94917) ;
#75074=AXIS2_PLACEMENT_3D('',#121128,#94918,#94919) ;
#75075=AXIS2_PLACEMENT_3D('',#121129,#94920,#94921) ;
#75076=AXIS2_PLACEMENT_3D('',#121130,#94922,#94923) ;
#75077=AXIS2_PLACEMENT_3D('',#121131,#94924,#94925) ;
#75078=AXIS2_PLACEMENT_3D('',#121132,#94926,#94927) ;
#75079=AXIS2_PLACEMENT_3D('',#121133,#94928,#94929) ;
#75080=AXIS2_PLACEMENT_3D('',#121134,#94930,#94931) ;
#75081=AXIS2_PLACEMENT_3D('',#121135,#94932,#94933) ;
#75082=AXIS2_PLACEMENT_3D('',#121136,#94934,#94935) ;
#75083=AXIS2_PLACEMENT_3D('',#121137,#94936,#94937) ;
#75084=AXIS2_PLACEMENT_3D('',#121138,#94938,#94939) ;
#75085=AXIS2_PLACEMENT_3D('',#121139,#94940,#94941) ;
#75086=AXIS2_PLACEMENT_3D('',#121140,#94942,#94943) ;
#75087=AXIS2_PLACEMENT_3D('',#121141,#94944,#94945) ;
#75088=AXIS2_PLACEMENT_3D('',#121142,#94946,#94947) ;
#75089=AXIS2_PLACEMENT_3D('',#121143,#94948,#94949) ;
#75090=AXIS2_PLACEMENT_3D('',#121144,#94950,#94951) ;
#75091=AXIS2_PLACEMENT_3D('',#121145,#94952,#94953) ;
#75092=AXIS2_PLACEMENT_3D('',#121146,#94954,#94955) ;
#75093=AXIS2_PLACEMENT_3D('',#121147,#94956,#94957) ;
#75094=AXIS2_PLACEMENT_3D('',#121148,#94958,#94959) ;
#75095=AXIS2_PLACEMENT_3D('',#121149,#94960,#94961) ;
#75096=AXIS2_PLACEMENT_3D('',#121150,#94962,#94963) ;
#75097=AXIS2_PLACEMENT_3D('',#121151,#94964,#94965) ;
#75098=AXIS2_PLACEMENT_3D('',#121152,#94966,#94967) ;
#75099=AXIS2_PLACEMENT_3D('',#121153,#94968,#94969) ;
#75100=AXIS2_PLACEMENT_3D('',#121154,#94970,#94971) ;
#75101=AXIS2_PLACEMENT_3D('',#121155,#94972,#94973) ;
#75102=AXIS2_PLACEMENT_3D('',#121156,#94974,#94975) ;
#75103=AXIS2_PLACEMENT_3D('',#121157,#94976,#94977) ;
#75104=AXIS2_PLACEMENT_3D('',#121158,#94978,#94979) ;
#75105=AXIS2_PLACEMENT_3D('',#121159,#94980,#94981) ;
#75106=AXIS2_PLACEMENT_3D('',#121160,#94982,#94983) ;
#75107=AXIS2_PLACEMENT_3D('',#121161,#94984,#94985) ;
#75108=AXIS2_PLACEMENT_3D('',#121162,#94986,#94987) ;
#75109=AXIS2_PLACEMENT_3D('',#121163,#94988,#94989) ;
#75110=AXIS2_PLACEMENT_3D('',#121165,#94990,#94991) ;
#75111=AXIS2_PLACEMENT_3D('',#121166,#94992,#94993) ;
#75112=AXIS2_PLACEMENT_3D('',#121167,#94994,#94995) ;
#75113=AXIS2_PLACEMENT_3D('',#121168,#94996,#94997) ;
#75114=AXIS2_PLACEMENT_3D('',#121169,#94998,#94999) ;
#75115=AXIS2_PLACEMENT_3D('',#121170,#95000,#95001) ;
#75116=AXIS2_PLACEMENT_3D('',#121171,#95002,#95003) ;
#75117=AXIS2_PLACEMENT_3D('',#121172,#95004,#95005) ;
#75118=AXIS2_PLACEMENT_3D('',#121173,#95006,#95007) ;
#75119=AXIS2_PLACEMENT_3D('',#121184,#95009,#95010) ;
#75120=AXIS2_PLACEMENT_3D('',#121241,#95012,#95013) ;
#75121=AXIS2_PLACEMENT_3D('',#121242,#95014,#95015) ;
#75122=AXIS2_PLACEMENT_3D('',#121243,#95016,#95017) ;
#75123=AXIS2_PLACEMENT_3D('',#121244,#95018,#95019) ;
#75124=AXIS2_PLACEMENT_3D('',#121245,#95020,#95021) ;
#75125=AXIS2_PLACEMENT_3D('',#121246,#95022,#95023) ;
#75126=AXIS2_PLACEMENT_3D('',#121247,#95024,#95025) ;
#75127=AXIS2_PLACEMENT_3D('',#121248,#95026,#95027) ;
#75128=AXIS2_PLACEMENT_3D('',#121249,#95028,#95029) ;
#75129=AXIS2_PLACEMENT_3D('',#121250,#95030,#95031) ;
#75130=AXIS2_PLACEMENT_3D('',#121251,#95032,#95033) ;
#75131=AXIS2_PLACEMENT_3D('',#121252,#95034,#95035) ;
#75132=AXIS2_PLACEMENT_3D('',#121253,#95036,#95037) ;
#75133=AXIS2_PLACEMENT_3D('',#121254,#95038,#95039) ;
#75134=AXIS2_PLACEMENT_3D('',#121255,#95040,#95041) ;
#75135=AXIS2_PLACEMENT_3D('',#121256,#95042,#95043) ;
#75136=AXIS2_PLACEMENT_3D('',#121257,#95044,#95045) ;
#75137=AXIS2_PLACEMENT_3D('',#121258,#95046,#95047) ;
#75138=AXIS2_PLACEMENT_3D('',#121259,#95048,#95049) ;
#75139=AXIS2_PLACEMENT_3D('',#121260,#95050,#95051) ;
#75140=AXIS2_PLACEMENT_3D('',#121261,#95052,#95053) ;
#75141=AXIS2_PLACEMENT_3D('',#121262,#95054,#95055) ;
#75142=AXIS2_PLACEMENT_3D('',#121263,#95056,#95057) ;
#75143=AXIS2_PLACEMENT_3D('',#121266,#95059,#95060) ;
#75144=AXIS2_PLACEMENT_3D('',#121267,#95061,#95062) ;
#75145=AXIS2_PLACEMENT_3D('',#121268,#95063,#95064) ;
#75146=AXIS2_PLACEMENT_3D('',#121269,#95065,#95066) ;
#75147=AXIS2_PLACEMENT_3D('',#121270,#95067,#95068) ;
#75148=AXIS2_PLACEMENT_3D('',#121271,#95069,#95070) ;
#75149=AXIS2_PLACEMENT_3D('',#121272,#95071,#95072) ;
#75150=AXIS2_PLACEMENT_3D('',#121273,#95073,#95074) ;
#75151=AXIS2_PLACEMENT_3D('',#121274,#95075,#95076) ;
#75152=AXIS2_PLACEMENT_3D('',#121275,#95077,#95078) ;
#75153=AXIS2_PLACEMENT_3D('',#121276,#95079,#95080) ;
#75154=AXIS2_PLACEMENT_3D('',#121277,#95081,#95082) ;
#75155=AXIS2_PLACEMENT_3D('',#121278,#95083,#95084) ;
#75156=AXIS2_PLACEMENT_3D('',#121279,#95085,#95086) ;
#75157=AXIS2_PLACEMENT_3D('',#121280,#95087,#95088) ;
#75158=AXIS2_PLACEMENT_3D('',#121281,#95089,#95090) ;
#75159=AXIS2_PLACEMENT_3D('',#121283,#95091,#95092) ;
#75160=AXIS2_PLACEMENT_3D('',#121284,#95093,#95094) ;
#75161=AXIS2_PLACEMENT_3D('',#121285,#95095,#95096) ;
#75162=AXIS2_PLACEMENT_3D('',#121286,#95097,#95098) ;
#75163=AXIS2_PLACEMENT_3D('',#121287,#95099,#95100) ;
#75164=AXIS2_PLACEMENT_3D('',#121288,#95101,#95102) ;
#75165=AXIS2_PLACEMENT_3D('',#121289,#95103,#95104) ;
#75166=AXIS2_PLACEMENT_3D('',#121290,#95105,#95106) ;
#75167=AXIS2_PLACEMENT_3D('',#121291,#95107,#95108) ;
#75168=AXIS2_PLACEMENT_3D('',#121292,#95109,#95110) ;
#75169=AXIS2_PLACEMENT_3D('',#121293,#95111,#95112) ;
#75170=AXIS2_PLACEMENT_3D('',#121294,#95113,#95114) ;
#75171=AXIS2_PLACEMENT_3D('',#121295,#95115,#95116) ;
#75172=AXIS2_PLACEMENT_3D('',#121298,#95118,#95119) ;
#75173=AXIS2_PLACEMENT_3D('',#121299,#95120,#95121) ;
#75174=AXIS2_PLACEMENT_3D('',#121300,#95122,#95123) ;
#75175=AXIS2_PLACEMENT_3D('',#121301,#95124,#95125) ;
#75176=AXIS2_PLACEMENT_3D('',#121302,#95126,#95127) ;
#75177=AXIS2_PLACEMENT_3D('',#121303,#95128,#95129) ;
#75178=AXIS2_PLACEMENT_3D('',#121304,#95130,#95131) ;
#75179=AXIS2_PLACEMENT_3D('',#121305,#95132,#95133) ;
#75180=AXIS2_PLACEMENT_3D('',#121306,#95134,#95135) ;
#75181=AXIS2_PLACEMENT_3D('',#121307,#95136,#95137) ;
#75182=AXIS2_PLACEMENT_3D('',#121308,#95138,#95139) ;
#75183=AXIS2_PLACEMENT_3D('',#121309,#95140,#95141) ;
#75184=AXIS2_PLACEMENT_3D('',#121310,#95142,#95143) ;
#75185=AXIS2_PLACEMENT_3D('',#121312,#95144,#95145) ;
#75186=AXIS2_PLACEMENT_3D('',#121313,#95146,#95147) ;
#75187=AXIS2_PLACEMENT_3D('',#121314,#95148,#95149) ;
#75188=AXIS2_PLACEMENT_3D('',#121315,#95150,#95151) ;
#75189=AXIS2_PLACEMENT_3D('',#121316,#95152,#95153) ;
#75190=AXIS2_PLACEMENT_3D('',#121317,#95154,#95155) ;
#75191=AXIS2_PLACEMENT_3D('',#121318,#95156,#95157) ;
#75192=AXIS2_PLACEMENT_3D('',#121319,#95158,#95159) ;
#75193=AXIS2_PLACEMENT_3D('',#121320,#95160,#95161) ;
#75194=AXIS2_PLACEMENT_3D('',#121321,#95162,#95163) ;
#75195=AXIS2_PLACEMENT_3D('',#121322,#95164,#95165) ;
#75196=AXIS2_PLACEMENT_3D('',#121324,#95167,#95168) ;
#75197=AXIS2_PLACEMENT_3D('',#121325,#95169,#95170) ;
#75198=AXIS2_PLACEMENT_3D('',#121326,#95171,#95172) ;
#75199=AXIS2_PLACEMENT_3D('',#121327,#95173,#95174) ;
#75200=AXIS2_PLACEMENT_3D('',#121328,#95175,#95176) ;
#75201=AXIS2_PLACEMENT_3D('',#121329,#95177,#95178) ;
#75202=AXIS2_PLACEMENT_3D('',#121330,#95179,#95180) ;
#75203=AXIS2_PLACEMENT_3D('',#121331,#95181,#95182) ;
#75204=AXIS2_PLACEMENT_3D('',#121332,#95183,#95184) ;
#75205=AXIS2_PLACEMENT_3D('',#121333,#95185,#95186) ;
#75206=AXIS2_PLACEMENT_3D('',#121334,#95187,#95188) ;
#75207=AXIS2_PLACEMENT_3D('',#121335,#95189,#95190) ;
#75208=AXIS2_PLACEMENT_3D('',#121336,#95191,#95192) ;
#75209=AXIS2_PLACEMENT_3D('',#121337,#95193,#95194) ;
#75210=AXIS2_PLACEMENT_3D('',#121338,#95195,#95196) ;
#75211=AXIS2_PLACEMENT_3D('',#121339,#95197,#95198) ;
#75212=AXIS2_PLACEMENT_3D('',#121340,#95199,#95200) ;
#75213=AXIS2_PLACEMENT_3D('',#121341,#95201,#95202) ;
#75214=AXIS2_PLACEMENT_3D('',#121342,#95203,#95204) ;
#75215=AXIS2_PLACEMENT_3D('',#121343,#95205,#95206) ;
#75216=AXIS2_PLACEMENT_3D('',#121344,#95207,#95208) ;
#75217=AXIS2_PLACEMENT_3D('',#121345,#95209,#95210) ;
#75218=AXIS2_PLACEMENT_3D('',#121346,#95211,#95212) ;
#75219=AXIS2_PLACEMENT_3D('',#121347,#95213,#95214) ;
#75220=AXIS2_PLACEMENT_3D('',#121348,#95215,#95216) ;
#75221=AXIS2_PLACEMENT_3D('',#121349,#95217,#95218) ;
#75222=AXIS2_PLACEMENT_3D('',#121350,#95219,#95220) ;
#75223=AXIS2_PLACEMENT_3D('',#121351,#95221,#95222) ;
#75224=AXIS2_PLACEMENT_3D('',#121352,#95223,#95224) ;
#75225=AXIS2_PLACEMENT_3D('',#121353,#95225,#95226) ;
#75226=AXIS2_PLACEMENT_3D('',#121354,#95227,#95228) ;
#75227=AXIS2_PLACEMENT_3D('',#121355,#95229,#95230) ;
#75228=AXIS2_PLACEMENT_3D('',#121356,#95231,#95232) ;
#75229=AXIS2_PLACEMENT_3D('',#121357,#95233,#95234) ;
#75230=AXIS2_PLACEMENT_3D('',#121358,#95235,#95236) ;
#75231=AXIS2_PLACEMENT_3D('',#121359,#95237,#95238) ;
#75232=AXIS2_PLACEMENT_3D('',#121360,#95239,#95240) ;
#75233=AXIS2_PLACEMENT_3D('',#121361,#95241,#95242) ;
#75234=AXIS2_PLACEMENT_3D('',#121362,#95243,#95244) ;
#75235=AXIS2_PLACEMENT_3D('',#121363,#95245,#95246) ;
#75236=AXIS2_PLACEMENT_3D('',#121364,#95247,#95248) ;
#75237=AXIS2_PLACEMENT_3D('',#121365,#95249,#95250) ;
#75238=AXIS2_PLACEMENT_3D('',#121366,#95251,#95252) ;
#75239=AXIS2_PLACEMENT_3D('',#121367,#95253,#95254) ;
#75240=AXIS2_PLACEMENT_3D('',#121368,#95255,#95256) ;
#75241=AXIS2_PLACEMENT_3D('',#121369,#95257,#95258) ;
#75242=AXIS2_PLACEMENT_3D('',#121370,#95259,#95260) ;
#75243=AXIS2_PLACEMENT_3D('',#121371,#95261,#95262) ;
#75244=AXIS2_PLACEMENT_3D('',#121372,#95263,#95264) ;
#75245=AXIS2_PLACEMENT_3D('',#121373,#95265,#95266) ;
#75246=AXIS2_PLACEMENT_3D('',#121374,#95267,#95268) ;
#75247=AXIS2_PLACEMENT_3D('',#121375,#95269,#95270) ;
#75248=AXIS2_PLACEMENT_3D('',#121376,#95271,#95272) ;
#75249=AXIS2_PLACEMENT_3D('',#121377,#95273,#95274) ;
#75250=AXIS2_PLACEMENT_3D('',#121378,#95275,#95276) ;
#75251=AXIS2_PLACEMENT_3D('',#121379,#95277,#95278) ;
#75252=AXIS2_PLACEMENT_3D('',#121380,#95279,#95280) ;
#75253=AXIS2_PLACEMENT_3D('',#121381,#95281,#95282) ;
#75254=AXIS2_PLACEMENT_3D('',#121382,#95283,#95284) ;
#75255=AXIS2_PLACEMENT_3D('',#121383,#95285,#95286) ;
#75256=AXIS2_PLACEMENT_3D('',#121384,#95287,#95288) ;
#75257=AXIS2_PLACEMENT_3D('',#121385,#95289,#95290) ;
#75258=AXIS2_PLACEMENT_3D('',#121386,#95291,#95292) ;
#75259=AXIS2_PLACEMENT_3D('',#121387,#95293,#95294) ;
#75260=AXIS2_PLACEMENT_3D('',#121388,#95295,#95296) ;
#75261=AXIS2_PLACEMENT_3D('',#121389,#95297,#95298) ;
#75262=AXIS2_PLACEMENT_3D('',#121390,#95299,#95300) ;
#75263=AXIS2_PLACEMENT_3D('',#121392,#95301,#95302) ;
#75264=AXIS2_PLACEMENT_3D('',#121393,#95303,#95304) ;
#75265=AXIS2_PLACEMENT_3D('',#121394,#95305,#95306) ;
#75266=AXIS2_PLACEMENT_3D('',#121395,#95307,#95308) ;
#75267=AXIS2_PLACEMENT_3D('',#121396,#95309,#95310) ;
#75268=AXIS2_PLACEMENT_3D('',#121397,#95311,#95312) ;
#75269=AXIS2_PLACEMENT_3D('',#121398,#95313,#95314) ;
#75270=AXIS2_PLACEMENT_3D('',#121399,#95315,#95316) ;
#75271=AXIS2_PLACEMENT_3D('',#121400,#95317,#95318) ;
#75272=AXIS2_PLACEMENT_3D('',#121411,#95320,#95321) ;
#75273=AXIS2_PLACEMENT_3D('',#121468,#95323,#95324) ;
#75274=AXIS2_PLACEMENT_3D('',#121469,#95325,#95326) ;
#75275=AXIS2_PLACEMENT_3D('',#121470,#95327,#95328) ;
#75276=AXIS2_PLACEMENT_3D('',#121471,#95329,#95330) ;
#75277=AXIS2_PLACEMENT_3D('',#121472,#95331,#95332) ;
#75278=AXIS2_PLACEMENT_3D('',#121473,#95333,#95334) ;
#75279=AXIS2_PLACEMENT_3D('',#121474,#95335,#95336) ;
#75280=AXIS2_PLACEMENT_3D('',#121475,#95337,#95338) ;
#75281=AXIS2_PLACEMENT_3D('',#121476,#95339,#95340) ;
#75282=AXIS2_PLACEMENT_3D('',#121477,#95341,#95342) ;
#75283=AXIS2_PLACEMENT_3D('',#121478,#95343,#95344) ;
#75284=AXIS2_PLACEMENT_3D('',#121479,#95345,#95346) ;
#75285=AXIS2_PLACEMENT_3D('',#121480,#95347,#95348) ;
#75286=AXIS2_PLACEMENT_3D('',#121481,#95349,#95350) ;
#75287=AXIS2_PLACEMENT_3D('',#121482,#95351,#95352) ;
#75288=AXIS2_PLACEMENT_3D('',#121483,#95353,#95354) ;
#75289=AXIS2_PLACEMENT_3D('',#121484,#95355,#95356) ;
#75290=AXIS2_PLACEMENT_3D('',#121485,#95357,#95358) ;
#75291=AXIS2_PLACEMENT_3D('',#121486,#95359,#95360) ;
#75292=AXIS2_PLACEMENT_3D('',#121487,#95361,#95362) ;
#75293=AXIS2_PLACEMENT_3D('',#121488,#95363,#95364) ;
#75294=AXIS2_PLACEMENT_3D('',#121489,#95365,#95366) ;
#75295=AXIS2_PLACEMENT_3D('',#121490,#95367,#95368) ;
#75296=AXIS2_PLACEMENT_3D('',#121493,#95370,#95371) ;
#75297=AXIS2_PLACEMENT_3D('',#121494,#95372,#95373) ;
#75298=AXIS2_PLACEMENT_3D('',#121495,#95374,#95375) ;
#75299=AXIS2_PLACEMENT_3D('',#121496,#95376,#95377) ;
#75300=AXIS2_PLACEMENT_3D('',#121497,#95378,#95379) ;
#75301=AXIS2_PLACEMENT_3D('',#121498,#95380,#95381) ;
#75302=AXIS2_PLACEMENT_3D('',#121499,#95382,#95383) ;
#75303=AXIS2_PLACEMENT_3D('',#121500,#95384,#95385) ;
#75304=AXIS2_PLACEMENT_3D('',#121501,#95386,#95387) ;
#75305=AXIS2_PLACEMENT_3D('',#121502,#95388,#95389) ;
#75306=AXIS2_PLACEMENT_3D('',#121503,#95390,#95391) ;
#75307=AXIS2_PLACEMENT_3D('',#121504,#95392,#95393) ;
#75308=AXIS2_PLACEMENT_3D('',#121505,#95394,#95395) ;
#75309=AXIS2_PLACEMENT_3D('',#121506,#95396,#95397) ;
#75310=AXIS2_PLACEMENT_3D('',#121507,#95398,#95399) ;
#75311=AXIS2_PLACEMENT_3D('',#121508,#95400,#95401) ;
#75312=AXIS2_PLACEMENT_3D('',#121510,#95402,#95403) ;
#75313=AXIS2_PLACEMENT_3D('',#121511,#95404,#95405) ;
#75314=AXIS2_PLACEMENT_3D('',#121512,#95406,#95407) ;
#75315=AXIS2_PLACEMENT_3D('',#121513,#95408,#95409) ;
#75316=AXIS2_PLACEMENT_3D('',#121514,#95410,#95411) ;
#75317=AXIS2_PLACEMENT_3D('',#121515,#95412,#95413) ;
#75318=AXIS2_PLACEMENT_3D('',#121516,#95414,#95415) ;
#75319=AXIS2_PLACEMENT_3D('',#121517,#95416,#95417) ;
#75320=AXIS2_PLACEMENT_3D('',#121518,#95418,#95419) ;
#75321=AXIS2_PLACEMENT_3D('',#121519,#95420,#95421) ;
#75322=AXIS2_PLACEMENT_3D('',#121520,#95422,#95423) ;
#75323=AXIS2_PLACEMENT_3D('',#121521,#95424,#95425) ;
#75324=AXIS2_PLACEMENT_3D('',#121522,#95426,#95427) ;
#75325=AXIS2_PLACEMENT_3D('',#121525,#95429,#95430) ;
#75326=AXIS2_PLACEMENT_3D('',#121526,#95431,#95432) ;
#75327=AXIS2_PLACEMENT_3D('',#121527,#95433,#95434) ;
#75328=AXIS2_PLACEMENT_3D('',#121528,#95435,#95436) ;
#75329=AXIS2_PLACEMENT_3D('',#121529,#95437,#95438) ;
#75330=AXIS2_PLACEMENT_3D('',#121530,#95439,#95440) ;
#75331=AXIS2_PLACEMENT_3D('',#121531,#95441,#95442) ;
#75332=AXIS2_PLACEMENT_3D('',#121532,#95443,#95444) ;
#75333=AXIS2_PLACEMENT_3D('',#121533,#95445,#95446) ;
#75334=AXIS2_PLACEMENT_3D('',#121534,#95447,#95448) ;
#75335=AXIS2_PLACEMENT_3D('',#121535,#95449,#95450) ;
#75336=AXIS2_PLACEMENT_3D('',#121536,#95451,#95452) ;
#75337=AXIS2_PLACEMENT_3D('',#121537,#95453,#95454) ;
#75338=AXIS2_PLACEMENT_3D('',#121539,#95455,#95456) ;
#75339=AXIS2_PLACEMENT_3D('',#121540,#95457,#95458) ;
#75340=AXIS2_PLACEMENT_3D('',#121541,#95459,#95460) ;
#75341=AXIS2_PLACEMENT_3D('',#121542,#95461,#95462) ;
#75342=AXIS2_PLACEMENT_3D('',#121543,#95463,#95464) ;
#75343=AXIS2_PLACEMENT_3D('',#121544,#95465,#95466) ;
#75344=AXIS2_PLACEMENT_3D('',#121545,#95467,#95468) ;
#75345=AXIS2_PLACEMENT_3D('',#121546,#95469,#95470) ;
#75346=AXIS2_PLACEMENT_3D('',#121547,#95471,#95472) ;
#75347=AXIS2_PLACEMENT_3D('',#121548,#95473,#95474) ;
#75348=AXIS2_PLACEMENT_3D('',#121549,#95475,#95476) ;
#75349=AXIS2_PLACEMENT_3D('',#121551,#95478,#95479) ;
#75350=AXIS2_PLACEMENT_3D('',#121552,#95480,#95481) ;
#75351=AXIS2_PLACEMENT_3D('',#121553,#95482,#95483) ;
#75352=AXIS2_PLACEMENT_3D('',#121554,#95484,#95485) ;
#75353=AXIS2_PLACEMENT_3D('',#121555,#95486,#95487) ;
#75354=AXIS2_PLACEMENT_3D('',#121556,#95488,#95489) ;
#75355=AXIS2_PLACEMENT_3D('',#121557,#95490,#95491) ;
#75356=AXIS2_PLACEMENT_3D('',#121558,#95492,#95493) ;
#75357=AXIS2_PLACEMENT_3D('',#121559,#95494,#95495) ;
#75358=AXIS2_PLACEMENT_3D('',#121560,#95496,#95497) ;
#75359=AXIS2_PLACEMENT_3D('',#121561,#95498,#95499) ;
#75360=AXIS2_PLACEMENT_3D('',#121562,#95500,#95501) ;
#75361=AXIS2_PLACEMENT_3D('',#121563,#95502,#95503) ;
#75362=AXIS2_PLACEMENT_3D('',#121564,#95504,#95505) ;
#75363=AXIS2_PLACEMENT_3D('',#121565,#95506,#95507) ;
#75364=AXIS2_PLACEMENT_3D('',#121566,#95508,#95509) ;
#75365=AXIS2_PLACEMENT_3D('',#121567,#95510,#95511) ;
#75366=AXIS2_PLACEMENT_3D('',#121568,#95512,#95513) ;
#75367=AXIS2_PLACEMENT_3D('',#121569,#95514,#95515) ;
#75368=AXIS2_PLACEMENT_3D('',#121570,#95516,#95517) ;
#75369=AXIS2_PLACEMENT_3D('',#121571,#95518,#95519) ;
#75370=AXIS2_PLACEMENT_3D('',#121572,#95520,#95521) ;
#75371=AXIS2_PLACEMENT_3D('',#121573,#95522,#95523) ;
#75372=AXIS2_PLACEMENT_3D('',#121574,#95524,#95525) ;
#75373=AXIS2_PLACEMENT_3D('',#121575,#95526,#95527) ;
#75374=AXIS2_PLACEMENT_3D('',#121576,#95528,#95529) ;
#75375=AXIS2_PLACEMENT_3D('',#121577,#95530,#95531) ;
#75376=AXIS2_PLACEMENT_3D('',#121578,#95532,#95533) ;
#75377=AXIS2_PLACEMENT_3D('',#121579,#95534,#95535) ;
#75378=AXIS2_PLACEMENT_3D('',#121580,#95536,#95537) ;
#75379=AXIS2_PLACEMENT_3D('',#121581,#95538,#95539) ;
#75380=AXIS2_PLACEMENT_3D('',#121582,#95540,#95541) ;
#75381=AXIS2_PLACEMENT_3D('',#121583,#95542,#95543) ;
#75382=AXIS2_PLACEMENT_3D('',#121584,#95544,#95545) ;
#75383=AXIS2_PLACEMENT_3D('',#121585,#95546,#95547) ;
#75384=AXIS2_PLACEMENT_3D('',#121586,#95548,#95549) ;
#75385=AXIS2_PLACEMENT_3D('',#121587,#95550,#95551) ;
#75386=AXIS2_PLACEMENT_3D('',#121588,#95552,#95553) ;
#75387=AXIS2_PLACEMENT_3D('',#121589,#95554,#95555) ;
#75388=AXIS2_PLACEMENT_3D('',#121590,#95556,#95557) ;
#75389=AXIS2_PLACEMENT_3D('',#121591,#95558,#95559) ;
#75390=AXIS2_PLACEMENT_3D('',#121592,#95560,#95561) ;
#75391=AXIS2_PLACEMENT_3D('',#121593,#95562,#95563) ;
#75392=AXIS2_PLACEMENT_3D('',#121594,#95564,#95565) ;
#75393=AXIS2_PLACEMENT_3D('',#121595,#95566,#95567) ;
#75394=AXIS2_PLACEMENT_3D('',#121596,#95568,#95569) ;
#75395=AXIS2_PLACEMENT_3D('',#121597,#95570,#95571) ;
#75396=AXIS2_PLACEMENT_3D('',#121598,#95572,#95573) ;
#75397=AXIS2_PLACEMENT_3D('',#121599,#95574,#95575) ;
#75398=AXIS2_PLACEMENT_3D('',#121600,#95576,#95577) ;
#75399=AXIS2_PLACEMENT_3D('',#121601,#95578,#95579) ;
#75400=AXIS2_PLACEMENT_3D('',#121602,#95580,#95581) ;
#75401=AXIS2_PLACEMENT_3D('',#121603,#95582,#95583) ;
#75402=AXIS2_PLACEMENT_3D('',#121604,#95584,#95585) ;
#75403=AXIS2_PLACEMENT_3D('',#121605,#95586,#95587) ;
#75404=AXIS2_PLACEMENT_3D('',#121606,#95588,#95589) ;
#75405=AXIS2_PLACEMENT_3D('',#121607,#95590,#95591) ;
#75406=AXIS2_PLACEMENT_3D('',#121608,#95592,#95593) ;
#75407=AXIS2_PLACEMENT_3D('',#121609,#95594,#95595) ;
#75408=AXIS2_PLACEMENT_3D('',#121610,#95596,#95597) ;
#75409=AXIS2_PLACEMENT_3D('',#121611,#95598,#95599) ;
#75410=AXIS2_PLACEMENT_3D('',#121620,#95604,#95605) ;
#75411=AXIS2_PLACEMENT_3D('',#121629,#95610,#95611) ;
#75412=AXIS2_PLACEMENT_3D('',#121638,#95616,#95617) ;
#75413=AXIS2_PLACEMENT_3D('',#121647,#95622,#95623) ;
#75414=AXIS2_PLACEMENT_3D('',#121656,#95628,#95629) ;
#75415=AXIS2_PLACEMENT_3D('',#121660,#95631,#95632) ;
#75416=AXIS2_PLACEMENT_3D('',#121662,#95633,#95634) ;
#75417=AXIS2_PLACEMENT_3D('',#121666,#95637,#95638) ;
#75418=AXIS2_PLACEMENT_3D('',#121670,#95640,#95641) ;
#75419=AXIS2_PLACEMENT_3D('',#121672,#95642,#95643) ;
#75420=AXIS2_PLACEMENT_3D('',#121676,#95646,#95647) ;
#75421=AXIS2_PLACEMENT_3D('',#121677,#95648,#95649) ;
#75422=AXIS2_PLACEMENT_3D('',#121678,#95650,#95651) ;
#75423=AXIS2_PLACEMENT_3D('',#121679,#95652,#95653) ;
#75424=AXIS2_PLACEMENT_3D('',#121680,#95654,#95655) ;
#75425=AXIS2_PLACEMENT_3D('',#121681,#95656,#95657) ;
#75426=AXIS2_PLACEMENT_3D('',#121682,#95658,#95659) ;
#75427=AXIS2_PLACEMENT_3D('',#121691,#95664,#95665) ;
#75428=AXIS2_PLACEMENT_3D('',#121697,#95669,#95670) ;
#75429=AXIS2_PLACEMENT_3D('',#121703,#95674,#95675) ;
#75430=AXIS2_PLACEMENT_3D('',#121712,#95680,#95681) ;
#75431=AXIS2_PLACEMENT_3D('',#121721,#95686,#95687) ;
#75432=AXIS2_PLACEMENT_3D('',#121727,#95691,#95692) ;
#75433=AXIS2_PLACEMENT_3D('',#121733,#95696,#95697) ;
#75434=AXIS2_PLACEMENT_3D('',#121742,#95702,#95703) ;
#75435=AXIS2_PLACEMENT_3D('',#121751,#95708,#95709) ;
#75436=AXIS2_PLACEMENT_3D('',#121760,#95714,#95715) ;
#75437=AXIS2_PLACEMENT_3D('',#121769,#95720,#95721) ;
#75438=AXIS2_PLACEMENT_3D('',#121778,#95726,#95727) ;
#75439=AXIS2_PLACEMENT_3D('',#121782,#95729,#95730) ;
#75440=AXIS2_PLACEMENT_3D('',#121784,#95731,#95732) ;
#75441=AXIS2_PLACEMENT_3D('',#121788,#95735,#95736) ;
#75442=AXIS2_PLACEMENT_3D('',#121792,#95738,#95739) ;
#75443=AXIS2_PLACEMENT_3D('',#121794,#95740,#95741) ;
#75444=AXIS2_PLACEMENT_3D('',#121798,#95744,#95745) ;
#75445=AXIS2_PLACEMENT_3D('',#121799,#95746,#95747) ;
#75446=AXIS2_PLACEMENT_3D('',#121800,#95748,#95749) ;
#75447=AXIS2_PLACEMENT_3D('',#121801,#95750,#95751) ;
#75448=AXIS2_PLACEMENT_3D('',#121802,#95752,#95753) ;
#75449=AXIS2_PLACEMENT_3D('',#121803,#95754,#95755) ;
#75450=AXIS2_PLACEMENT_3D('',#121804,#95756,#95757) ;
#75451=AXIS2_PLACEMENT_3D('',#121813,#95762,#95763) ;
#75452=AXIS2_PLACEMENT_3D('',#121819,#95767,#95768) ;
#75453=AXIS2_PLACEMENT_3D('',#121825,#95772,#95773) ;
#75454=AXIS2_PLACEMENT_3D('',#121834,#95778,#95779) ;
#75455=AXIS2_PLACEMENT_3D('',#121843,#95784,#95785) ;
#75456=AXIS2_PLACEMENT_3D('',#121849,#95789,#95790) ;
#75457=AXIS2_PLACEMENT_3D('',#121855,#95794,#95795) ;
#75458=AXIS2_PLACEMENT_3D('',#121864,#95800,#95801) ;
#75459=AXIS2_PLACEMENT_3D('',#121873,#95806,#95807) ;
#75460=AXIS2_PLACEMENT_3D('',#121882,#95812,#95813) ;
#75461=AXIS2_PLACEMENT_3D('',#121891,#95818,#95819) ;
#75462=AXIS2_PLACEMENT_3D('',#121900,#95824,#95825) ;
#75463=AXIS2_PLACEMENT_3D('',#121904,#95827,#95828) ;
#75464=AXIS2_PLACEMENT_3D('',#121906,#95829,#95830) ;
#75465=AXIS2_PLACEMENT_3D('',#121910,#95833,#95834) ;
#75466=AXIS2_PLACEMENT_3D('',#121914,#95836,#95837) ;
#75467=AXIS2_PLACEMENT_3D('',#121916,#95838,#95839) ;
#75468=AXIS2_PLACEMENT_3D('',#121920,#95842,#95843) ;
#75469=AXIS2_PLACEMENT_3D('',#121921,#95844,#95845) ;
#75470=AXIS2_PLACEMENT_3D('',#121922,#95846,#95847) ;
#75471=AXIS2_PLACEMENT_3D('',#121923,#95848,#95849) ;
#75472=AXIS2_PLACEMENT_3D('',#121924,#95850,#95851) ;
#75473=AXIS2_PLACEMENT_3D('',#121925,#95852,#95853) ;
#75474=AXIS2_PLACEMENT_3D('',#121926,#95854,#95855) ;
#75475=AXIS2_PLACEMENT_3D('',#121935,#95860,#95861) ;
#75476=AXIS2_PLACEMENT_3D('',#121941,#95865,#95866) ;
#75477=AXIS2_PLACEMENT_3D('',#121947,#95870,#95871) ;
#75478=AXIS2_PLACEMENT_3D('',#121956,#95876,#95877) ;
#75479=AXIS2_PLACEMENT_3D('',#121965,#95882,#95883) ;
#75480=AXIS2_PLACEMENT_3D('',#121971,#95887,#95888) ;
#75481=AXIS2_PLACEMENT_3D('',#121977,#95892,#95893) ;
#75482=AXIS2_PLACEMENT_3D('',#121986,#95898,#95899) ;
#75483=AXIS2_PLACEMENT_3D('',#121995,#95904,#95905) ;
#75484=AXIS2_PLACEMENT_3D('',#122004,#95910,#95911) ;
#75485=AXIS2_PLACEMENT_3D('',#122013,#95916,#95917) ;
#75486=AXIS2_PLACEMENT_3D('',#122022,#95922,#95923) ;
#75487=AXIS2_PLACEMENT_3D('',#122026,#95925,#95926) ;
#75488=AXIS2_PLACEMENT_3D('',#122028,#95927,#95928) ;
#75489=AXIS2_PLACEMENT_3D('',#122032,#95931,#95932) ;
#75490=AXIS2_PLACEMENT_3D('',#122036,#95934,#95935) ;
#75491=AXIS2_PLACEMENT_3D('',#122038,#95936,#95937) ;
#75492=AXIS2_PLACEMENT_3D('',#122042,#95940,#95941) ;
#75493=AXIS2_PLACEMENT_3D('',#122043,#95942,#95943) ;
#75494=AXIS2_PLACEMENT_3D('',#122044,#95944,#95945) ;
#75495=AXIS2_PLACEMENT_3D('',#122045,#95946,#95947) ;
#75496=AXIS2_PLACEMENT_3D('',#122046,#95948,#95949) ;
#75497=AXIS2_PLACEMENT_3D('',#122047,#95950,#95951) ;
#75498=AXIS2_PLACEMENT_3D('',#122048,#95952,#95953) ;
#75499=AXIS2_PLACEMENT_3D('',#122057,#95958,#95959) ;
#75500=AXIS2_PLACEMENT_3D('',#122063,#95963,#95964) ;
#75501=AXIS2_PLACEMENT_3D('',#122069,#95968,#95969) ;
#75502=AXIS2_PLACEMENT_3D('',#122078,#95974,#95975) ;
#75503=AXIS2_PLACEMENT_3D('',#122087,#95980,#95981) ;
#75504=AXIS2_PLACEMENT_3D('',#122093,#95985,#95986) ;
#75505=AXIS2_PLACEMENT_3D('',#122099,#95990,#95991) ;
#75506=AXIS2_PLACEMENT_3D('',#122108,#95996,#95997) ;
#75507=AXIS2_PLACEMENT_3D('',#122117,#96002,#96003) ;
#75508=AXIS2_PLACEMENT_3D('',#122126,#96008,#96009) ;
#75509=AXIS2_PLACEMENT_3D('',#122135,#96014,#96015) ;
#75510=AXIS2_PLACEMENT_3D('',#122144,#96020,#96021) ;
#75511=AXIS2_PLACEMENT_3D('',#122148,#96023,#96024) ;
#75512=AXIS2_PLACEMENT_3D('',#122150,#96025,#96026) ;
#75513=AXIS2_PLACEMENT_3D('',#122154,#96029,#96030) ;
#75514=AXIS2_PLACEMENT_3D('',#122158,#96032,#96033) ;
#75515=AXIS2_PLACEMENT_3D('',#122160,#96034,#96035) ;
#75516=AXIS2_PLACEMENT_3D('',#122164,#96038,#96039) ;
#75517=AXIS2_PLACEMENT_3D('',#122165,#96040,#96041) ;
#75518=AXIS2_PLACEMENT_3D('',#122166,#96042,#96043) ;
#75519=AXIS2_PLACEMENT_3D('',#122167,#96044,#96045) ;
#75520=AXIS2_PLACEMENT_3D('',#122168,#96046,#96047) ;
#75521=AXIS2_PLACEMENT_3D('',#122169,#96048,#96049) ;
#75522=AXIS2_PLACEMENT_3D('',#122170,#96050,#96051) ;
#75523=AXIS2_PLACEMENT_3D('',#122179,#96056,#96057) ;
#75524=AXIS2_PLACEMENT_3D('',#122185,#96061,#96062) ;
#75525=AXIS2_PLACEMENT_3D('',#122191,#96066,#96067) ;
#75526=AXIS2_PLACEMENT_3D('',#122200,#96072,#96073) ;
#75527=AXIS2_PLACEMENT_3D('',#122209,#96078,#96079) ;
#75528=AXIS2_PLACEMENT_3D('',#122215,#96083,#96084) ;
#75529=AXIS2_PLACEMENT_3D('',#122221,#96088,#96089) ;
#75530=AXIS2_PLACEMENT_3D('',#122230,#96094,#96095) ;
#75531=AXIS2_PLACEMENT_3D('',#122239,#96100,#96101) ;
#75532=AXIS2_PLACEMENT_3D('',#122248,#96106,#96107) ;
#75533=AXIS2_PLACEMENT_3D('',#122257,#96112,#96113) ;
#75534=AXIS2_PLACEMENT_3D('',#122266,#96118,#96119) ;
#75535=AXIS2_PLACEMENT_3D('',#122270,#96121,#96122) ;
#75536=AXIS2_PLACEMENT_3D('',#122272,#96123,#96124) ;
#75537=AXIS2_PLACEMENT_3D('',#122276,#96127,#96128) ;
#75538=AXIS2_PLACEMENT_3D('',#122280,#96130,#96131) ;
#75539=AXIS2_PLACEMENT_3D('',#122282,#96132,#96133) ;
#75540=AXIS2_PLACEMENT_3D('',#122286,#96136,#96137) ;
#75541=AXIS2_PLACEMENT_3D('',#122287,#96138,#96139) ;
#75542=AXIS2_PLACEMENT_3D('',#122288,#96140,#96141) ;
#75543=AXIS2_PLACEMENT_3D('',#122289,#96142,#96143) ;
#75544=AXIS2_PLACEMENT_3D('',#122290,#96144,#96145) ;
#75545=AXIS2_PLACEMENT_3D('',#122291,#96146,#96147) ;
#75546=AXIS2_PLACEMENT_3D('',#122292,#96148,#96149) ;
#75547=AXIS2_PLACEMENT_3D('',#122301,#96154,#96155) ;
#75548=AXIS2_PLACEMENT_3D('',#122307,#96159,#96160) ;
#75549=AXIS2_PLACEMENT_3D('',#122313,#96164,#96165) ;
#75550=AXIS2_PLACEMENT_3D('',#122322,#96170,#96171) ;
#75551=AXIS2_PLACEMENT_3D('',#122331,#96176,#96177) ;
#75552=AXIS2_PLACEMENT_3D('',#122337,#96181,#96182) ;
#75553=AXIS2_PLACEMENT_3D('',#122343,#96186,#96187) ;
#75554=AXIS2_PLACEMENT_3D('',#122352,#96192,#96193) ;
#75555=AXIS2_PLACEMENT_3D('',#122361,#96198,#96199) ;
#75556=AXIS2_PLACEMENT_3D('',#122370,#96204,#96205) ;
#75557=AXIS2_PLACEMENT_3D('',#122379,#96210,#96211) ;
#75558=AXIS2_PLACEMENT_3D('',#122388,#96216,#96217) ;
#75559=AXIS2_PLACEMENT_3D('',#122392,#96219,#96220) ;
#75560=AXIS2_PLACEMENT_3D('',#122394,#96221,#96222) ;
#75561=AXIS2_PLACEMENT_3D('',#122398,#96225,#96226) ;
#75562=AXIS2_PLACEMENT_3D('',#122402,#96228,#96229) ;
#75563=AXIS2_PLACEMENT_3D('',#122404,#96230,#96231) ;
#75564=AXIS2_PLACEMENT_3D('',#122408,#96234,#96235) ;
#75565=AXIS2_PLACEMENT_3D('',#122409,#96236,#96237) ;
#75566=AXIS2_PLACEMENT_3D('',#122410,#96238,#96239) ;
#75567=AXIS2_PLACEMENT_3D('',#122411,#96240,#96241) ;
#75568=AXIS2_PLACEMENT_3D('',#122412,#96242,#96243) ;
#75569=AXIS2_PLACEMENT_3D('',#122413,#96244,#96245) ;
#75570=AXIS2_PLACEMENT_3D('',#122414,#96246,#96247) ;
#75571=AXIS2_PLACEMENT_3D('',#122423,#96252,#96253) ;
#75572=AXIS2_PLACEMENT_3D('',#122429,#96257,#96258) ;
#75573=AXIS2_PLACEMENT_3D('',#122435,#96262,#96263) ;
#75574=AXIS2_PLACEMENT_3D('',#122444,#96268,#96269) ;
#75575=AXIS2_PLACEMENT_3D('',#122453,#96274,#96275) ;
#75576=AXIS2_PLACEMENT_3D('',#122459,#96279,#96280) ;
#75577=AXIS2_PLACEMENT_3D('',#122465,#96284,#96285) ;
#75578=AXIS2_PLACEMENT_3D('',#122474,#96290,#96291) ;
#75579=AXIS2_PLACEMENT_3D('',#122483,#96296,#96297) ;
#75580=AXIS2_PLACEMENT_3D('',#122492,#96302,#96303) ;
#75581=AXIS2_PLACEMENT_3D('',#122501,#96308,#96309) ;
#75582=AXIS2_PLACEMENT_3D('',#122510,#96314,#96315) ;
#75583=AXIS2_PLACEMENT_3D('',#122514,#96317,#96318) ;
#75584=AXIS2_PLACEMENT_3D('',#122516,#96319,#96320) ;
#75585=AXIS2_PLACEMENT_3D('',#122520,#96323,#96324) ;
#75586=AXIS2_PLACEMENT_3D('',#122524,#96326,#96327) ;
#75587=AXIS2_PLACEMENT_3D('',#122526,#96328,#96329) ;
#75588=AXIS2_PLACEMENT_3D('',#122530,#96332,#96333) ;
#75589=AXIS2_PLACEMENT_3D('',#122531,#96334,#96335) ;
#75590=AXIS2_PLACEMENT_3D('',#122532,#96336,#96337) ;
#75591=AXIS2_PLACEMENT_3D('',#122533,#96338,#96339) ;
#75592=AXIS2_PLACEMENT_3D('',#122534,#96340,#96341) ;
#75593=AXIS2_PLACEMENT_3D('',#122535,#96342,#96343) ;
#75594=AXIS2_PLACEMENT_3D('',#122536,#96344,#96345) ;
#75595=AXIS2_PLACEMENT_3D('',#122545,#96350,#96351) ;
#75596=AXIS2_PLACEMENT_3D('',#122551,#96355,#96356) ;
#75597=AXIS2_PLACEMENT_3D('',#122557,#96360,#96361) ;
#75598=AXIS2_PLACEMENT_3D('',#122566,#96366,#96367) ;
#75599=AXIS2_PLACEMENT_3D('',#122575,#96372,#96373) ;
#75600=AXIS2_PLACEMENT_3D('',#122581,#96377,#96378) ;
#75601=AXIS2_PLACEMENT_3D('',#122587,#96382,#96383) ;
#75602=AXIS2_PLACEMENT_3D('',#122596,#96388,#96389) ;
#75603=AXIS2_PLACEMENT_3D('',#122605,#96394,#96395) ;
#75604=AXIS2_PLACEMENT_3D('',#122614,#96400,#96401) ;
#75605=AXIS2_PLACEMENT_3D('',#122623,#96406,#96407) ;
#75606=AXIS2_PLACEMENT_3D('',#122632,#96412,#96413) ;
#75607=AXIS2_PLACEMENT_3D('',#122636,#96415,#96416) ;
#75608=AXIS2_PLACEMENT_3D('',#122638,#96417,#96418) ;
#75609=AXIS2_PLACEMENT_3D('',#122642,#96421,#96422) ;
#75610=AXIS2_PLACEMENT_3D('',#122646,#96424,#96425) ;
#75611=AXIS2_PLACEMENT_3D('',#122648,#96426,#96427) ;
#75612=AXIS2_PLACEMENT_3D('',#122652,#96430,#96431) ;
#75613=AXIS2_PLACEMENT_3D('',#122653,#96432,#96433) ;
#75614=AXIS2_PLACEMENT_3D('',#122654,#96434,#96435) ;
#75615=AXIS2_PLACEMENT_3D('',#122655,#96436,#96437) ;
#75616=AXIS2_PLACEMENT_3D('',#122656,#96438,#96439) ;
#75617=AXIS2_PLACEMENT_3D('',#122657,#96440,#96441) ;
#75618=AXIS2_PLACEMENT_3D('',#122658,#96442,#96443) ;
#75619=AXIS2_PLACEMENT_3D('',#122667,#96448,#96449) ;
#75620=AXIS2_PLACEMENT_3D('',#122673,#96453,#96454) ;
#75621=AXIS2_PLACEMENT_3D('',#122679,#96458,#96459) ;
#75622=AXIS2_PLACEMENT_3D('',#122688,#96464,#96465) ;
#75623=AXIS2_PLACEMENT_3D('',#122697,#96470,#96471) ;
#75624=AXIS2_PLACEMENT_3D('',#122703,#96475,#96476) ;
#75625=AXIS2_PLACEMENT_3D('',#122709,#96480,#96481) ;
#75626=AXIS2_PLACEMENT_3D('',#122718,#96486,#96487) ;
#75627=AXIS2_PLACEMENT_3D('',#122727,#96492,#96493) ;
#75628=AXIS2_PLACEMENT_3D('',#122736,#96498,#96499) ;
#75629=AXIS2_PLACEMENT_3D('',#122745,#96504,#96505) ;
#75630=AXIS2_PLACEMENT_3D('',#122754,#96510,#96511) ;
#75631=AXIS2_PLACEMENT_3D('',#122763,#96516,#96517) ;
#75632=AXIS2_PLACEMENT_3D('',#122772,#96522,#96523) ;
#75633=AXIS2_PLACEMENT_3D('',#122781,#96528,#96529) ;
#75634=AXIS2_PLACEMENT_3D('',#122790,#96534,#96535) ;
#75635=AXIS2_PLACEMENT_3D('',#122799,#96540,#96541) ;
#75636=AXIS2_PLACEMENT_3D('',#122808,#96546,#96547) ;
#75637=AXIS2_PLACEMENT_3D('',#122817,#96552,#96553) ;
#75638=AXIS2_PLACEMENT_3D('',#122826,#96558,#96559) ;
#75639=AXIS2_PLACEMENT_3D('',#122835,#96564,#96565) ;
#75640=AXIS2_PLACEMENT_3D('',#122844,#96570,#96571) ;
#75641=AXIS2_PLACEMENT_3D('',#122853,#96576,#96577) ;
#75642=AXIS2_PLACEMENT_3D('',#122862,#96582,#96583) ;
#75643=AXIS2_PLACEMENT_3D('',#122871,#96588,#96589) ;
#75644=AXIS2_PLACEMENT_3D('',#122880,#96594,#96595) ;
#75645=AXIS2_PLACEMENT_3D('',#122889,#96600,#96601) ;
#75646=AXIS2_PLACEMENT_3D('',#122898,#96606,#96607) ;
#75647=AXIS2_PLACEMENT_3D('',#122907,#96612,#96613) ;
#75648=AXIS2_PLACEMENT_3D('',#122916,#96618,#96619) ;
#75649=AXIS2_PLACEMENT_3D('',#122925,#96624,#96625) ;
#75650=AXIS2_PLACEMENT_3D('',#122934,#96630,#96631) ;
#75651=AXIS2_PLACEMENT_3D('',#122943,#96636,#96637) ;
#75652=AXIS2_PLACEMENT_3D('',#122952,#96642,#96643) ;
#75653=AXIS2_PLACEMENT_3D('',#122961,#96648,#96649) ;
#75654=AXIS2_PLACEMENT_3D('',#122970,#96654,#96655) ;
#75655=AXIS2_PLACEMENT_3D('',#122979,#96660,#96661) ;
#75656=AXIS2_PLACEMENT_3D('',#122988,#96666,#96667) ;
#75657=AXIS2_PLACEMENT_3D('',#122997,#96672,#96673) ;
#75658=AXIS2_PLACEMENT_3D('',#123006,#96678,#96679) ;
#75659=AXIS2_PLACEMENT_3D('',#123015,#96684,#96685) ;
#75660=AXIS2_PLACEMENT_3D('',#123024,#96690,#96691) ;
#75661=AXIS2_PLACEMENT_3D('',#123033,#96696,#96697) ;
#75662=AXIS2_PLACEMENT_3D('',#123034,#96698,#96699) ;
#75663=AXIS2_PLACEMENT_3D('',#123035,#96700,#96701) ;
#75664=AXIS2_PLACEMENT_3D('',#123036,#96702,#96703) ;
#75665=AXIS2_PLACEMENT_3D('',#123037,#96704,#96705) ;
#75666=AXIS2_PLACEMENT_3D('',#123038,#96706,#96707) ;
#75667=AXIS2_PLACEMENT_3D('',#123039,#96708,#96709) ;
#75668=AXIS2_PLACEMENT_3D('',#123040,#96710,#96711) ;
#75669=AXIS2_PLACEMENT_3D('',#123041,#96712,#96713) ;
#75670=AXIS2_PLACEMENT_3D('',#123042,#96714,#96715) ;
#75671=AXIS2_PLACEMENT_3D('',#123043,#96716,#96717) ;
#75672=AXIS2_PLACEMENT_3D('',#123044,#96718,#96719) ;
#75673=AXIS2_PLACEMENT_3D('',#123045,#96720,#96721) ;
#75674=AXIS2_PLACEMENT_3D('',#123046,#96722,#96723) ;
#75675=AXIS2_PLACEMENT_3D('',#123047,#96724,#96725) ;
#75676=AXIS2_PLACEMENT_3D('',#123048,#96726,#96727) ;
#75677=AXIS2_PLACEMENT_3D('',#123049,#96728,#96729) ;
#75678=AXIS2_PLACEMENT_3D('',#123050,#96730,#96731) ;
#75679=AXIS2_PLACEMENT_3D('',#123051,#96732,#96733) ;
#75680=AXIS2_PLACEMENT_3D('',#123052,#96734,#96735) ;
#75681=AXIS2_PLACEMENT_3D('',#123053,#96736,#96737) ;
#75682=AXIS2_PLACEMENT_3D('',#123054,#96738,#96739) ;
#75683=AXIS2_PLACEMENT_3D('',#123055,#96740,#96741) ;
#75684=AXIS2_PLACEMENT_3D('',#123056,#96742,#96743) ;
#75685=AXIS2_PLACEMENT_3D('',#123057,#96744,#96745) ;
#75686=AXIS2_PLACEMENT_3D('',#123058,#96746,#96747) ;
#75687=AXIS2_PLACEMENT_3D('',#123059,#96748,#96749) ;
#75688=AXIS2_PLACEMENT_3D('',#123060,#96750,#96751) ;
#75689=AXIS2_PLACEMENT_3D('',#123061,#96752,#96753) ;
#75690=AXIS2_PLACEMENT_3D('',#123062,#96754,#96755) ;
#75691=AXIS2_PLACEMENT_3D('',#123063,#96756,#96757) ;
#75692=AXIS2_PLACEMENT_3D('',#123064,#96758,#96759) ;
#75693=AXIS2_PLACEMENT_3D('',#123065,#96760,#96761) ;
#75694=AXIS2_PLACEMENT_3D('',#123066,#96762,#96763) ;
#75695=AXIS2_PLACEMENT_3D('',#123067,#96764,#96765) ;
#75696=AXIS2_PLACEMENT_3D('',#123068,#96766,#96767) ;
#75697=AXIS2_PLACEMENT_3D('',#123069,#96768,#96769) ;
#75698=AXIS2_PLACEMENT_3D('',#123070,#96770,#96771) ;
#75699=AXIS2_PLACEMENT_3D('',#123071,#96772,#96773) ;
#75700=AXIS2_PLACEMENT_3D('',#123072,#96774,#96775) ;
#75701=AXIS2_PLACEMENT_3D('',#123073,#96776,#96777) ;
#75702=AXIS2_PLACEMENT_3D('',#123074,#96778,#96779) ;
#75703=AXIS2_PLACEMENT_3D('',#123075,#96780,#96781) ;
#75704=AXIS2_PLACEMENT_3D('',#123076,#96782,#96783) ;
#75705=AXIS2_PLACEMENT_3D('',#123077,#96784,#96785) ;
#75706=AXIS2_PLACEMENT_3D('',#123078,#96786,#96787) ;
#75707=AXIS2_PLACEMENT_3D('',#123079,#96788,#96789) ;
#75708=AXIS2_PLACEMENT_3D('',#123080,#96790,#96791) ;
#75709=AXIS2_PLACEMENT_3D('',#123081,#96792,#96793) ;
#75710=AXIS2_PLACEMENT_3D('',#123082,#96794,#96795) ;
#75711=AXIS2_PLACEMENT_3D('',#123083,#96796,#96797) ;
#75712=AXIS2_PLACEMENT_3D('',#123084,#96798,#96799) ;
#75713=AXIS2_PLACEMENT_3D('',#123085,#96800,#96801) ;
#75714=AXIS2_PLACEMENT_3D('',#123086,#96802,#96803) ;
#75715=AXIS2_PLACEMENT_3D('',#123087,#96804,#96805) ;
#75716=AXIS2_PLACEMENT_3D('',#123088,#96806,#96807) ;
#75717=AXIS2_PLACEMENT_3D('',#123089,#96808,#96809) ;
#75718=AXIS2_PLACEMENT_3D('',#123090,#96810,#96811) ;
#75719=AXIS2_PLACEMENT_3D('',#123091,#96812,#96813) ;
#75720=AXIS2_PLACEMENT_3D('',#123092,#96814,#96815) ;
#75721=AXIS2_PLACEMENT_3D('',#123093,#96816,#96817) ;
#75722=AXIS2_PLACEMENT_3D('',#123094,#96818,#96819) ;
#75723=AXIS2_PLACEMENT_3D('',#123095,#96820,#96821) ;
#75724=AXIS2_PLACEMENT_3D('',#123096,#96822,#96823) ;
#75725=AXIS2_PLACEMENT_3D('',#123097,#96824,#96825) ;
#75726=AXIS2_PLACEMENT_3D('',#123098,#96826,#96827) ;
#75727=AXIS2_PLACEMENT_3D('',#123099,#96828,#96829) ;
#75728=AXIS2_PLACEMENT_3D('',#123100,#96830,#96831) ;
#75729=AXIS2_PLACEMENT_3D('',#123101,#96832,#96833) ;
#75730=AXIS2_PLACEMENT_3D('',#123102,#96834,#96835) ;
#75731=AXIS2_PLACEMENT_3D('',#123103,#96836,#96837) ;
#75732=AXIS2_PLACEMENT_3D('',#123104,#96838,#96839) ;
#75733=AXIS2_PLACEMENT_3D('',#123105,#96840,#96841) ;
#75734=AXIS2_PLACEMENT_3D('',#123106,#96842,#96843) ;
#75735=AXIS2_PLACEMENT_3D('',#123107,#96844,#96845) ;
#75736=AXIS2_PLACEMENT_3D('',#123108,#96846,#96847) ;
#75737=AXIS2_PLACEMENT_3D('',#123109,#96848,#96849) ;
#75738=AXIS2_PLACEMENT_3D('',#123110,#96850,#96851) ;
#75739=AXIS2_PLACEMENT_3D('',#123111,#96852,#96853) ;
#75740=AXIS2_PLACEMENT_3D('',#123112,#96854,#96855) ;
#75741=AXIS2_PLACEMENT_3D('',#123113,#96856,#96857) ;
#75742=AXIS2_PLACEMENT_3D('',#123114,#96858,#96859) ;
#75743=AXIS2_PLACEMENT_3D('',#123115,#96860,#96861) ;
#75744=AXIS2_PLACEMENT_3D('',#123116,#96862,#96863) ;
#75745=AXIS2_PLACEMENT_3D('',#123117,#96864,#96865) ;
#75746=AXIS2_PLACEMENT_3D('',#123118,#96866,#96867) ;
#75747=AXIS2_PLACEMENT_3D('',#123119,#96868,#96869) ;
#75748=AXIS2_PLACEMENT_3D('',#123120,#96870,#96871) ;
#75749=AXIS2_PLACEMENT_3D('',#123121,#96872,#96873) ;
#75750=AXIS2_PLACEMENT_3D('',#123122,#96874,#96875) ;
#75751=AXIS2_PLACEMENT_3D('',#123123,#96876,#96877) ;
#75752=AXIS2_PLACEMENT_3D('',#123124,#96878,#96879) ;
#75753=AXIS2_PLACEMENT_3D('',#123125,#96880,#96881) ;
#75754=AXIS2_PLACEMENT_3D('',#123126,#96882,#96883) ;
#75755=AXIS2_PLACEMENT_3D('',#123127,#96884,#96885) ;
#75756=AXIS2_PLACEMENT_3D('',#123128,#96886,#96887) ;
#75757=AXIS2_PLACEMENT_3D('',#123129,#96888,#96889) ;
#75758=AXIS2_PLACEMENT_3D('',#123130,#96890,#96891) ;
#75759=AXIS2_PLACEMENT_3D('',#123131,#96892,#96893) ;
#75760=AXIS2_PLACEMENT_3D('',#123132,#96894,#96895) ;
#75761=AXIS2_PLACEMENT_3D('',#123133,#96896,#96897) ;
#75762=AXIS2_PLACEMENT_3D('',#123134,#96898,#96899) ;
#75763=AXIS2_PLACEMENT_3D('',#123135,#96900,#96901) ;
#75764=AXIS2_PLACEMENT_3D('',#123136,#96902,#96903) ;
#75765=AXIS2_PLACEMENT_3D('',#123137,#96904,#96905) ;
#75766=AXIS2_PLACEMENT_3D('',#123138,#96906,#96907) ;
#75767=AXIS2_PLACEMENT_3D('',#123139,#96908,#96909) ;
#75768=AXIS2_PLACEMENT_3D('',#123140,#96910,#96911) ;
#75769=AXIS2_PLACEMENT_3D('',#123141,#96912,#96913) ;
#75770=AXIS2_PLACEMENT_3D('',#123142,#96914,#96915) ;
#75771=AXIS2_PLACEMENT_3D('',#123143,#96916,#96917) ;
#75772=AXIS2_PLACEMENT_3D('',#123144,#96918,#96919) ;
#75773=AXIS2_PLACEMENT_3D('',#123145,#96920,#96921) ;
#75774=AXIS2_PLACEMENT_3D('',#123146,#96922,#96923) ;
#75775=AXIS2_PLACEMENT_3D('',#123147,#96924,#96925) ;
#75776=AXIS2_PLACEMENT_3D('',#123148,#96926,#96927) ;
#75777=AXIS2_PLACEMENT_3D('',#123149,#96928,#96929) ;
#75778=AXIS2_PLACEMENT_3D('',#123150,#96930,#96931) ;
#75779=AXIS2_PLACEMENT_3D('',#123151,#96932,#96933) ;
#75780=AXIS2_PLACEMENT_3D('',#123152,#96934,#96935) ;
#75781=AXIS2_PLACEMENT_3D('',#123153,#96936,#96937) ;
#75782=AXIS2_PLACEMENT_3D('',#123154,#96938,#96939) ;
#75783=AXIS2_PLACEMENT_3D('',#123155,#96940,#96941) ;
#75784=AXIS2_PLACEMENT_3D('',#123156,#96942,#96943) ;
#75785=AXIS2_PLACEMENT_3D('',#123157,#96944,#96945) ;
#75786=AXIS2_PLACEMENT_3D('',#123158,#96946,#96947) ;
#75787=AXIS2_PLACEMENT_3D('',#123159,#96948,#96949) ;
#75788=AXIS2_PLACEMENT_3D('',#123160,#96950,#96951) ;
#75789=AXIS2_PLACEMENT_3D('',#123161,#96952,#96953) ;
#75790=AXIS2_PLACEMENT_3D('',#123162,#96954,#96955) ;
#75791=AXIS2_PLACEMENT_3D('',#123163,#96956,#96957) ;
#75792=AXIS2_PLACEMENT_3D('',#123164,#96958,#96959) ;
#75793=AXIS2_PLACEMENT_3D('',#123165,#96960,#96961) ;
#75794=AXIS2_PLACEMENT_3D('',#123166,#96962,#96963) ;
#75795=AXIS2_PLACEMENT_3D('',#123167,#96964,#96965) ;
#75796=AXIS2_PLACEMENT_3D('',#123168,#96966,#96967) ;
#75797=AXIS2_PLACEMENT_3D('',#123169,#96968,#96969) ;
#75798=AXIS2_PLACEMENT_3D('',#123170,#96970,#96971) ;
#75799=AXIS2_PLACEMENT_3D('',#123171,#96972,#96973) ;
#75800=AXIS2_PLACEMENT_3D('',#123172,#96974,#96975) ;
#75801=AXIS2_PLACEMENT_3D('',#123173,#96976,#96977) ;
#75802=AXIS2_PLACEMENT_3D('',#123174,#96978,#96979) ;
#75803=AXIS2_PLACEMENT_3D('',#123175,#96980,#96981) ;
#75804=AXIS2_PLACEMENT_3D('',#123176,#96982,#96983) ;
#75805=AXIS2_PLACEMENT_3D('',#123177,#96984,#96985) ;
#75806=AXIS2_PLACEMENT_3D('',#123178,#96986,#96987) ;
#75807=AXIS2_PLACEMENT_3D('',#123179,#96988,#96989) ;
#75808=AXIS2_PLACEMENT_3D('',#123180,#96990,#96991) ;
#75809=AXIS2_PLACEMENT_3D('',#123181,#96992,#96993) ;
#75810=AXIS2_PLACEMENT_3D('',#123182,#96994,#96995) ;
#75811=AXIS2_PLACEMENT_3D('',#123183,#96996,#96997) ;
#75812=AXIS2_PLACEMENT_3D('',#123184,#96998,#96999) ;
#75813=AXIS2_PLACEMENT_3D('',#123185,#97000,#97001) ;
#75814=AXIS2_PLACEMENT_3D('',#123186,#97002,#97003) ;
#75815=AXIS2_PLACEMENT_3D('',#123187,#97004,#97005) ;
#75816=AXIS2_PLACEMENT_3D('',#123188,#97006,#97007) ;
#75817=AXIS2_PLACEMENT_3D('',#123189,#97008,#97009) ;
#75818=AXIS2_PLACEMENT_3D('',#123190,#97010,#97011) ;
#75819=AXIS2_PLACEMENT_3D('',#123191,#97012,#97013) ;
#75820=AXIS2_PLACEMENT_3D('',#123192,#97014,#97015) ;
#75821=AXIS2_PLACEMENT_3D('',#123193,#97016,#97017) ;
#75822=AXIS2_PLACEMENT_3D('',#123194,#97018,#97019) ;
#75823=AXIS2_PLACEMENT_3D('',#123195,#97020,#97021) ;
#75824=AXIS2_PLACEMENT_3D('',#123196,#97022,#97023) ;
#75825=AXIS2_PLACEMENT_3D('',#123197,#97024,#97025) ;
#75826=AXIS2_PLACEMENT_3D('',#123198,#97026,#97027) ;
#75827=AXIS2_PLACEMENT_3D('',#123199,#97028,#97029) ;
#75828=AXIS2_PLACEMENT_3D('',#123200,#97030,#97031) ;
#75829=AXIS2_PLACEMENT_3D('',#123201,#97032,#97033) ;
#75830=AXIS2_PLACEMENT_3D('',#123202,#97034,#97035) ;
#75831=AXIS2_PLACEMENT_3D('',#123203,#97036,#97037) ;
#75832=AXIS2_PLACEMENT_3D('',#123204,#97038,#97039) ;
#75833=AXIS2_PLACEMENT_3D('',#123205,#97040,#97041) ;
#75834=AXIS2_PLACEMENT_3D('',#123206,#97042,#97043) ;
#75835=AXIS2_PLACEMENT_3D('',#123207,#97044,#97045) ;
#75836=AXIS2_PLACEMENT_3D('',#123208,#97046,#97047) ;
#75837=AXIS2_PLACEMENT_3D('',#123209,#97048,#97049) ;
#75838=AXIS2_PLACEMENT_3D('',#123210,#97050,#97051) ;
#75839=AXIS2_PLACEMENT_3D('',#123211,#97052,#97053) ;
#75840=AXIS2_PLACEMENT_3D('',#123212,#97054,#97055) ;
#75841=AXIS2_PLACEMENT_3D('',#123213,#97056,#97057) ;
#75842=AXIS2_PLACEMENT_3D('',#123214,#97058,#97059) ;
#75843=AXIS2_PLACEMENT_3D('',#123215,#97060,#97061) ;
#75844=AXIS2_PLACEMENT_3D('',#123216,#97062,#97063) ;
#75845=AXIS2_PLACEMENT_3D('',#123217,#97064,#97065) ;
#75846=AXIS2_PLACEMENT_3D('',#123218,#97066,#97067) ;
#75847=AXIS2_PLACEMENT_3D('',#123219,#97068,#97069) ;
#75848=AXIS2_PLACEMENT_3D('',#123220,#97070,#97071) ;
#75849=AXIS2_PLACEMENT_3D('',#123221,#97072,#97073) ;
#75850=AXIS2_PLACEMENT_3D('',#123222,#97074,#97075) ;
#75851=AXIS2_PLACEMENT_3D('',#123223,#97076,#97077) ;
#75852=AXIS2_PLACEMENT_3D('',#123224,#97078,#97079) ;
#75853=AXIS2_PLACEMENT_3D('',#123225,#97080,#97081) ;
#75854=AXIS2_PLACEMENT_3D('',#123226,#97082,#97083) ;
#75855=AXIS2_PLACEMENT_3D('',#123227,#97084,#97085) ;
#75856=AXIS2_PLACEMENT_3D('',#123228,#97086,#97087) ;
#75857=AXIS2_PLACEMENT_3D('',#123229,#97088,#97089) ;
#75858=AXIS2_PLACEMENT_3D('',#123230,#97090,#97091) ;
#75859=AXIS2_PLACEMENT_3D('',#123231,#97092,#97093) ;
#75860=AXIS2_PLACEMENT_3D('',#123232,#97094,#97095) ;
#75861=AXIS2_PLACEMENT_3D('',#123233,#97096,#97097) ;
#75862=AXIS2_PLACEMENT_3D('',#123234,#97098,#97099) ;
#75863=AXIS2_PLACEMENT_3D('',#123235,#97100,#97101) ;
#75864=AXIS2_PLACEMENT_3D('',#123236,#97102,#97103) ;
#75865=AXIS2_PLACEMENT_3D('',#123237,#97104,#97105) ;
#75866=AXIS2_PLACEMENT_3D('',#123238,#97106,#97107) ;
#75867=AXIS2_PLACEMENT_3D('',#123239,#97108,#97109) ;
#75868=AXIS2_PLACEMENT_3D('',#123240,#97110,#97111) ;
#75869=AXIS2_PLACEMENT_3D('',#123241,#97112,#97113) ;
#75870=AXIS2_PLACEMENT_3D('',#123242,#97114,#97115) ;
#75871=AXIS2_PLACEMENT_3D('',#123243,#97116,#97117) ;
#75872=AXIS2_PLACEMENT_3D('',#123244,#97118,#97119) ;
#75873=AXIS2_PLACEMENT_3D('',#123245,#97120,#97121) ;
#75874=AXIS2_PLACEMENT_3D('',#123246,#97122,#97123) ;
#75875=AXIS2_PLACEMENT_3D('',#123247,#97124,#97125) ;
#75876=AXIS2_PLACEMENT_3D('',#123248,#97126,#97127) ;
#75877=AXIS2_PLACEMENT_3D('',#123249,#97128,#97129) ;
#75878=AXIS2_PLACEMENT_3D('',#123250,#97130,#97131) ;
#75879=AXIS2_PLACEMENT_3D('',#123251,#97132,#97133) ;
#75880=AXIS2_PLACEMENT_3D('',#123252,#97134,#97135) ;
#75881=AXIS2_PLACEMENT_3D('',#123253,#97136,#97137) ;
#75882=AXIS2_PLACEMENT_3D('',#123254,#97138,#97139) ;
#75883=AXIS2_PLACEMENT_3D('',#123255,#97140,#97141) ;
#75884=AXIS2_PLACEMENT_3D('',#123256,#97142,#97143) ;
#75885=AXIS2_PLACEMENT_3D('',#123257,#97144,#97145) ;
#75886=AXIS2_PLACEMENT_3D('',#123258,#97146,#97147) ;
#75887=AXIS2_PLACEMENT_3D('',#123259,#97148,#97149) ;
#75888=AXIS2_PLACEMENT_3D('',#123260,#97150,#97151) ;
#75889=AXIS2_PLACEMENT_3D('',#123261,#97152,#97153) ;
#75890=AXIS2_PLACEMENT_3D('',#123262,#97154,#97155) ;
#75891=AXIS2_PLACEMENT_3D('',#123263,#97156,#97157) ;
#75892=AXIS2_PLACEMENT_3D('',#123264,#97158,#97159) ;
#75893=AXIS2_PLACEMENT_3D('',#123265,#97160,#97161) ;
#75894=AXIS2_PLACEMENT_3D('',#123266,#97162,#97163) ;
#75895=AXIS2_PLACEMENT_3D('',#123267,#97164,#97165) ;
#75896=AXIS2_PLACEMENT_3D('',#123268,#97166,#97167) ;
#75897=AXIS2_PLACEMENT_3D('',#123269,#97168,#97169) ;
#75898=AXIS2_PLACEMENT_3D('',#123270,#97170,#97171) ;
#75899=AXIS2_PLACEMENT_3D('',#123271,#97172,#97173) ;
#75900=AXIS2_PLACEMENT_3D('',#123272,#97174,#97175) ;
#75901=AXIS2_PLACEMENT_3D('',#123273,#97176,#97177) ;
#75902=AXIS2_PLACEMENT_3D('',#123274,#97178,#97179) ;
#75903=AXIS2_PLACEMENT_3D('',#123275,#97180,#97181) ;
#75904=AXIS2_PLACEMENT_3D('',#123276,#97182,#97183) ;
#75905=AXIS2_PLACEMENT_3D('',#123277,#97184,#97185) ;
#75906=AXIS2_PLACEMENT_3D('',#123278,#97186,#97187) ;
#75907=AXIS2_PLACEMENT_3D('',#123279,#97188,#97189) ;
#75908=AXIS2_PLACEMENT_3D('',#123280,#97190,#97191) ;
#75909=AXIS2_PLACEMENT_3D('',#123281,#97192,#97193) ;
#75910=AXIS2_PLACEMENT_3D('',#123282,#97194,#97195) ;
#75911=AXIS2_PLACEMENT_3D('',#123283,#97196,#97197) ;
#75912=AXIS2_PLACEMENT_3D('',#123284,#97198,#97199) ;
#75913=AXIS2_PLACEMENT_3D('',#123285,#97200,#97201) ;
#75914=AXIS2_PLACEMENT_3D('',#123286,#97202,#97203) ;
#75915=AXIS2_PLACEMENT_3D('',#123287,#97204,#97205) ;
#75916=AXIS2_PLACEMENT_3D('',#123288,#97206,#97207) ;
#75917=AXIS2_PLACEMENT_3D('',#123289,#97208,#97209) ;
#75918=AXIS2_PLACEMENT_3D('',#123290,#97210,#97211) ;
#75919=AXIS2_PLACEMENT_3D('',#123291,#97212,#97213) ;
#75920=AXIS2_PLACEMENT_3D('',#123292,#97214,#97215) ;
#75921=AXIS2_PLACEMENT_3D('',#123293,#97216,#97217) ;
#75922=AXIS2_PLACEMENT_3D('',#123294,#97218,#97219) ;
#75923=AXIS2_PLACEMENT_3D('',#123295,#97220,#97221) ;
#75924=AXIS2_PLACEMENT_3D('',#123296,#97222,#97223) ;
#75925=AXIS2_PLACEMENT_3D('',#123297,#97224,#97225) ;
#75926=AXIS2_PLACEMENT_3D('',#123298,#97226,#97227) ;
#75927=AXIS2_PLACEMENT_3D('',#123299,#97228,#97229) ;
#75928=AXIS2_PLACEMENT_3D('',#123300,#97230,#97231) ;
#75929=AXIS2_PLACEMENT_3D('',#123301,#97232,#97233) ;
#75930=AXIS2_PLACEMENT_3D('',#123302,#97234,#97235) ;
#75931=AXIS2_PLACEMENT_3D('',#123303,#97236,#97237) ;
#75932=AXIS2_PLACEMENT_3D('',#123304,#97238,#97239) ;
#75933=AXIS2_PLACEMENT_3D('',#123305,#97240,#97241) ;
#75934=AXIS2_PLACEMENT_3D('',#123306,#97242,#97243) ;
#75935=AXIS2_PLACEMENT_3D('',#123307,#97244,#97245) ;
#75936=AXIS2_PLACEMENT_3D('',#123308,#97246,#97247) ;
#75937=AXIS2_PLACEMENT_3D('',#123309,#97248,#97249) ;
#75938=AXIS2_PLACEMENT_3D('',#123310,#97250,#97251) ;
#75939=AXIS2_PLACEMENT_3D('',#123311,#97252,#97253) ;
#75940=AXIS2_PLACEMENT_3D('',#123312,#97254,#97255) ;
#75941=AXIS2_PLACEMENT_3D('',#123313,#97256,#97257) ;
#75942=AXIS2_PLACEMENT_3D('',#123314,#97258,#97259) ;
#75943=AXIS2_PLACEMENT_3D('',#123315,#97260,#97261) ;
#75944=AXIS2_PLACEMENT_3D('',#123316,#97262,#97263) ;
#75945=AXIS2_PLACEMENT_3D('',#123317,#97264,#97265) ;
#75946=AXIS2_PLACEMENT_3D('',#123318,#97266,#97267) ;
#75947=AXIS2_PLACEMENT_3D('',#123319,#97268,#97269) ;
#75948=AXIS2_PLACEMENT_3D('',#123320,#97270,#97271) ;
#75949=AXIS2_PLACEMENT_3D('',#123321,#97272,#97273) ;
#75950=AXIS2_PLACEMENT_3D('',#123322,#97274,#97275) ;
#75951=AXIS2_PLACEMENT_3D('',#123323,#97276,#97277) ;
#75952=AXIS2_PLACEMENT_3D('',#123324,#97278,#97279) ;
#75953=AXIS2_PLACEMENT_3D('',#123325,#97280,#97281) ;
#75954=AXIS2_PLACEMENT_3D('',#123326,#97282,#97283) ;
#75955=AXIS2_PLACEMENT_3D('',#123327,#97284,#97285) ;
#75956=AXIS2_PLACEMENT_3D('',#123328,#97286,#97287) ;
#75957=AXIS2_PLACEMENT_3D('',#123329,#97288,#97289) ;
#75958=AXIS2_PLACEMENT_3D('',#123330,#97290,#97291) ;
#75959=AXIS2_PLACEMENT_3D('',#123331,#97292,#97293) ;
#75960=AXIS2_PLACEMENT_3D('',#123332,#97294,#97295) ;
#75961=AXIS2_PLACEMENT_3D('',#123333,#97296,#97297) ;
#75962=AXIS2_PLACEMENT_3D('',#123334,#97298,#97299) ;
#75963=AXIS2_PLACEMENT_3D('',#123335,#97300,#97301) ;
#75964=AXIS2_PLACEMENT_3D('',#123336,#97302,#97303) ;
#75965=AXIS2_PLACEMENT_3D('',#123337,#97304,#97305) ;
#75966=AXIS2_PLACEMENT_3D('',#123338,#97306,#97307) ;
#75967=AXIS2_PLACEMENT_3D('',#123339,#97308,#97309) ;
#75968=AXIS2_PLACEMENT_3D('',#123340,#97310,#97311) ;
#75969=AXIS2_PLACEMENT_3D('',#123341,#97312,#97313) ;
#75970=AXIS2_PLACEMENT_3D('',#123342,#97314,#97315) ;
#75971=AXIS2_PLACEMENT_3D('',#123343,#97316,#97317) ;
#75972=AXIS2_PLACEMENT_3D('',#123344,#97318,#97319) ;
#75973=AXIS2_PLACEMENT_3D('',#123345,#97320,#97321) ;
#75974=AXIS2_PLACEMENT_3D('',#123346,#97322,#97323) ;
#75975=AXIS2_PLACEMENT_3D('',#123347,#97324,#97325) ;
#75976=AXIS2_PLACEMENT_3D('',#123348,#97326,#97327) ;
#75977=AXIS2_PLACEMENT_3D('',#123349,#97328,#97329) ;
#75978=AXIS2_PLACEMENT_3D('',#123350,#97330,#97331) ;
#75979=AXIS2_PLACEMENT_3D('',#123351,#97332,#97333) ;
#75980=AXIS2_PLACEMENT_3D('',#123352,#97334,#97335) ;
#75981=AXIS2_PLACEMENT_3D('',#123353,#97336,#97337) ;
#75982=AXIS2_PLACEMENT_3D('',#123354,#97338,#97339) ;
#75983=AXIS2_PLACEMENT_3D('',#123355,#97340,#97341) ;
#75984=AXIS2_PLACEMENT_3D('',#123356,#97342,#97343) ;
#75985=AXIS2_PLACEMENT_3D('',#123357,#97344,#97345) ;
#75986=AXIS2_PLACEMENT_3D('',#123358,#97346,#97347) ;
#75987=AXIS2_PLACEMENT_3D('',#123359,#97348,#97349) ;
#75988=AXIS2_PLACEMENT_3D('',#123360,#97350,#97351) ;
#75989=AXIS2_PLACEMENT_3D('',#123361,#97352,#97353) ;
#75990=AXIS2_PLACEMENT_3D('',#123362,#97354,#97355) ;
#75991=AXIS2_PLACEMENT_3D('',#123363,#97356,#97357) ;
#75992=AXIS2_PLACEMENT_3D('',#123364,#97358,#97359) ;
#75993=AXIS2_PLACEMENT_3D('',#123365,#97360,#97361) ;
#75994=AXIS2_PLACEMENT_3D('',#123366,#97362,#97363) ;
#75995=AXIS2_PLACEMENT_3D('',#123367,#97364,#97365) ;
#75996=AXIS2_PLACEMENT_3D('',#123368,#97366,#97367) ;
#75997=AXIS2_PLACEMENT_3D('',#123369,#97368,#97369) ;
#75998=AXIS2_PLACEMENT_3D('',#123370,#97370,#97371) ;
#75999=AXIS2_PLACEMENT_3D('',#123371,#97372,#97373) ;
#76000=AXIS2_PLACEMENT_3D('',#123372,#97374,#97375) ;
#76001=AXIS2_PLACEMENT_3D('',#123373,#97376,#97377) ;
#76002=AXIS2_PLACEMENT_3D('',#123374,#97378,#97379) ;
#76003=AXIS2_PLACEMENT_3D('',#123375,#97380,#97381) ;
#76004=AXIS2_PLACEMENT_3D('',#123376,#97382,#97383) ;
#76005=AXIS2_PLACEMENT_3D('',#123377,#97384,#97385) ;
#76006=AXIS2_PLACEMENT_3D('',#123378,#97386,#97387) ;
#76007=AXIS2_PLACEMENT_3D('',#123379,#97388,#97389) ;
#76008=AXIS2_PLACEMENT_3D('',#123380,#97390,#97391) ;
#76009=AXIS2_PLACEMENT_3D('',#123381,#97392,#97393) ;
#76010=AXIS2_PLACEMENT_3D('',#123382,#97394,#97395) ;
#76011=AXIS2_PLACEMENT_3D('',#123383,#97396,#97397) ;
#76012=AXIS2_PLACEMENT_3D('',#123384,#97398,#97399) ;
#76013=AXIS2_PLACEMENT_3D('',#123385,#97400,#97401) ;
#76014=AXIS2_PLACEMENT_3D('',#123386,#97402,#97403) ;
#76015=AXIS2_PLACEMENT_3D('',#123387,#97404,#97405) ;
#76016=AXIS2_PLACEMENT_3D('',#123388,#97406,#97407) ;
#76017=AXIS2_PLACEMENT_3D('',#123389,#97408,#97409) ;
#76018=AXIS2_PLACEMENT_3D('',#123390,#97410,#97411) ;
#76019=AXIS2_PLACEMENT_3D('',#123391,#97412,#97413) ;
#76020=AXIS2_PLACEMENT_3D('',#123392,#97414,#97415) ;
#76021=AXIS2_PLACEMENT_3D('',#123393,#97416,#97417) ;
#76022=AXIS2_PLACEMENT_3D('',#123394,#97418,#97419) ;
#76023=AXIS2_PLACEMENT_3D('',#123395,#97420,#97421) ;
#76024=AXIS2_PLACEMENT_3D('',#123396,#97422,#97423) ;
#76025=AXIS2_PLACEMENT_3D('',#123397,#97424,#97425) ;
#76026=AXIS2_PLACEMENT_3D('',#123398,#97426,#97427) ;
#76027=AXIS2_PLACEMENT_3D('',#123399,#97428,#97429) ;
#76028=AXIS2_PLACEMENT_3D('',#123400,#97430,#97431) ;
#76029=AXIS2_PLACEMENT_3D('',#123401,#97432,#97433) ;
#76030=AXIS2_PLACEMENT_3D('',#123402,#97434,#97435) ;
#76031=AXIS2_PLACEMENT_3D('',#123403,#97436,#97437) ;
#76032=AXIS2_PLACEMENT_3D('',#123404,#97438,#97439) ;
#76033=AXIS2_PLACEMENT_3D('',#123405,#97440,#97441) ;
#76034=AXIS2_PLACEMENT_3D('',#123406,#97442,#97443) ;
#76035=AXIS2_PLACEMENT_3D('',#123407,#97444,#97445) ;
#76036=AXIS2_PLACEMENT_3D('',#123408,#97446,#97447) ;
#76037=AXIS2_PLACEMENT_3D('',#123409,#97448,#97449) ;
#76038=AXIS2_PLACEMENT_3D('',#123410,#97450,#97451) ;
#76039=AXIS2_PLACEMENT_3D('',#123411,#97452,#97453) ;
#76040=AXIS2_PLACEMENT_3D('',#123412,#97454,#97455) ;
#76041=AXIS2_PLACEMENT_3D('',#123413,#97456,#97457) ;
#76042=AXIS2_PLACEMENT_3D('',#123414,#97458,#97459) ;
#76043=AXIS2_PLACEMENT_3D('',#123415,#97460,#97461) ;
#76044=AXIS2_PLACEMENT_3D('',#123416,#97462,#97463) ;
#76045=AXIS2_PLACEMENT_3D('',#123417,#97464,#97465) ;
#76046=AXIS2_PLACEMENT_3D('',#123418,#97466,#97467) ;
#76047=AXIS2_PLACEMENT_3D('',#123419,#97468,#97469) ;
#76048=AXIS2_PLACEMENT_3D('',#123420,#97470,#97471) ;
#76049=AXIS2_PLACEMENT_3D('',#123421,#97472,#97473) ;
#76050=AXIS2_PLACEMENT_3D('',#123422,#97474,#97475) ;
#76051=AXIS2_PLACEMENT_3D('',#123423,#97476,#97477) ;
#76052=AXIS2_PLACEMENT_3D('',#123424,#97478,#97479) ;
#76053=AXIS2_PLACEMENT_3D('',#123425,#97480,#97481) ;
#76054=AXIS2_PLACEMENT_3D('',#123426,#97482,#97483) ;
#76055=AXIS2_PLACEMENT_3D('',#123427,#97484,#97485) ;
#76056=AXIS2_PLACEMENT_3D('',#123428,#97486,#97487) ;
#76057=AXIS2_PLACEMENT_3D('',#123429,#97488,#97489) ;
#76058=AXIS2_PLACEMENT_3D('',#123430,#97490,#97491) ;
#76059=AXIS2_PLACEMENT_3D('',#123431,#97492,#97493) ;
#76060=AXIS2_PLACEMENT_3D('',#123432,#97494,#97495) ;
#76061=AXIS2_PLACEMENT_3D('',#123433,#97496,#97497) ;
#76062=AXIS2_PLACEMENT_3D('',#123434,#97498,#97499) ;
#76063=AXIS2_PLACEMENT_3D('',#123435,#97500,#97501) ;
#76064=AXIS2_PLACEMENT_3D('',#123436,#97502,#97503) ;
#76065=AXIS2_PLACEMENT_3D('',#123437,#97504,#97505) ;
#76066=AXIS2_PLACEMENT_3D('',#123438,#97506,#97507) ;
#76067=AXIS2_PLACEMENT_3D('',#123439,#97508,#97509) ;
#76068=AXIS2_PLACEMENT_3D('',#123440,#97510,#97511) ;
#76069=AXIS2_PLACEMENT_3D('',#123441,#97512,#97513) ;
#76070=AXIS2_PLACEMENT_3D('',#123442,#97514,#97515) ;
#76071=AXIS2_PLACEMENT_3D('',#123443,#97516,#97517) ;
#76072=AXIS2_PLACEMENT_3D('',#123444,#97518,#97519) ;
#76073=AXIS2_PLACEMENT_3D('',#123445,#97520,#97521) ;
#76074=AXIS2_PLACEMENT_3D('',#123446,#97522,#97523) ;
#76075=AXIS2_PLACEMENT_3D('',#123447,#97524,#97525) ;
#76076=AXIS2_PLACEMENT_3D('',#123448,#97526,#97527) ;
#76077=AXIS2_PLACEMENT_3D('',#123449,#97528,#97529) ;
#76078=AXIS2_PLACEMENT_3D('',#123450,#97530,#97531) ;
#76079=AXIS2_PLACEMENT_3D('',#123451,#97532,#97533) ;
#76080=AXIS2_PLACEMENT_3D('',#123452,#97534,#97535) ;
#76081=AXIS2_PLACEMENT_3D('',#123453,#97536,#97537) ;
#76082=AXIS2_PLACEMENT_3D('',#123454,#97538,#97539) ;
#76083=AXIS2_PLACEMENT_3D('',#123455,#97540,#97541) ;
#76084=AXIS2_PLACEMENT_3D('',#123456,#97542,#97543) ;
#76085=AXIS2_PLACEMENT_3D('',#123457,#97544,#97545) ;
#76086=AXIS2_PLACEMENT_3D('',#123458,#97546,#97547) ;
#76087=AXIS2_PLACEMENT_3D('',#123459,#97548,#97549) ;
#76088=AXIS2_PLACEMENT_3D('',#123460,#97550,#97551) ;
#76089=AXIS2_PLACEMENT_3D('',#123461,#97552,#97553) ;
#76090=AXIS2_PLACEMENT_3D('',#123462,#97554,#97555) ;
#76091=AXIS2_PLACEMENT_3D('',#123463,#97556,#97557) ;
#76092=AXIS2_PLACEMENT_3D('',#123464,#97558,#97559) ;
#76093=AXIS2_PLACEMENT_3D('',#123465,#97560,#97561) ;
#76094=AXIS2_PLACEMENT_3D('',#123466,#97562,#97563) ;
#76095=AXIS2_PLACEMENT_3D('',#123467,#97564,#97565) ;
#76096=AXIS2_PLACEMENT_3D('',#123468,#97566,#97567) ;
#76097=AXIS2_PLACEMENT_3D('',#123469,#97568,#97569) ;
#76098=AXIS2_PLACEMENT_3D('',#123470,#97570,#97571) ;
#76099=AXIS2_PLACEMENT_3D('',#123471,#97572,#97573) ;
#76100=AXIS2_PLACEMENT_3D('',#123472,#97574,#97575) ;
#76101=AXIS2_PLACEMENT_3D('',#123473,#97576,#97577) ;
#76102=AXIS2_PLACEMENT_3D('',#123474,#97578,#97579) ;
#76103=AXIS2_PLACEMENT_3D('',#123475,#97580,#97581) ;
#76104=AXIS2_PLACEMENT_3D('',#123476,#97582,#97583) ;
#76105=AXIS2_PLACEMENT_3D('',#123477,#97584,#97585) ;
#76106=AXIS2_PLACEMENT_3D('',#123478,#97586,#97587) ;
#76107=AXIS2_PLACEMENT_3D('',#123479,#97588,#97589) ;
#76108=AXIS2_PLACEMENT_3D('',#123480,#97590,#97591) ;
#76109=AXIS2_PLACEMENT_3D('',#123481,#97592,#97593) ;
#76110=AXIS2_PLACEMENT_3D('',#123482,#97594,#97595) ;
#76111=AXIS2_PLACEMENT_3D('',#123483,#97596,#97597) ;
#76112=AXIS2_PLACEMENT_3D('',#123484,#97598,#97599) ;
#76113=AXIS2_PLACEMENT_3D('',#123485,#97600,#97601) ;
#76114=AXIS2_PLACEMENT_3D('',#123486,#97602,#97603) ;
#76115=AXIS2_PLACEMENT_3D('',#123487,#97604,#97605) ;
#76116=AXIS2_PLACEMENT_3D('',#123488,#97606,#97607) ;
#76117=AXIS2_PLACEMENT_3D('',#123489,#97608,#97609) ;
#76118=AXIS2_PLACEMENT_3D('',#123490,#97610,#97611) ;
#76119=AXIS2_PLACEMENT_3D('',#123491,#97612,#97613) ;
#76120=AXIS2_PLACEMENT_3D('',#123492,#97614,#97615) ;
#76121=AXIS2_PLACEMENT_3D('',#123493,#97616,#97617) ;
#76122=AXIS2_PLACEMENT_3D('',#123494,#97618,#97619) ;
#76123=AXIS2_PLACEMENT_3D('',#123495,#97620,#97621) ;
#76124=AXIS2_PLACEMENT_3D('',#123496,#97622,#97623) ;
#76125=AXIS2_PLACEMENT_3D('',#123497,#97624,#97625) ;
#76126=AXIS2_PLACEMENT_3D('',#123498,#97626,#97627) ;
#76127=AXIS2_PLACEMENT_3D('',#123499,#97628,#97629) ;
#76128=AXIS2_PLACEMENT_3D('',#123500,#97630,#97631) ;
#76129=AXIS2_PLACEMENT_3D('',#123501,#97632,#97633) ;
#76130=AXIS2_PLACEMENT_3D('',#123502,#97634,#97635) ;
#76131=AXIS2_PLACEMENT_3D('',#123503,#97636,#97637) ;
#76132=AXIS2_PLACEMENT_3D('',#123504,#97638,#97639) ;
#76133=AXIS2_PLACEMENT_3D('',#123505,#97640,#97641) ;
#76134=AXIS2_PLACEMENT_3D('',#123506,#97642,#97643) ;
#76135=AXIS2_PLACEMENT_3D('',#123507,#97644,#97645) ;
#76136=AXIS2_PLACEMENT_3D('',#123508,#97646,#97647) ;
#76137=AXIS2_PLACEMENT_3D('',#123509,#97648,#97649) ;
#76138=AXIS2_PLACEMENT_3D('',#123510,#97650,#97651) ;
#76139=AXIS2_PLACEMENT_3D('',#123511,#97652,#97653) ;
#76140=AXIS2_PLACEMENT_3D('',#123512,#97654,#97655) ;
#76141=AXIS2_PLACEMENT_3D('',#123513,#97656,#97657) ;
#76142=AXIS2_PLACEMENT_3D('',#123514,#97658,#97659) ;
#76143=AXIS2_PLACEMENT_3D('',#123515,#97660,#97661) ;
#76144=AXIS2_PLACEMENT_3D('',#123516,#97662,#97663) ;
#76145=AXIS2_PLACEMENT_3D('',#123517,#97664,#97665) ;
#76146=AXIS2_PLACEMENT_3D('',#123518,#97666,#97667) ;
#76147=AXIS2_PLACEMENT_3D('',#123519,#97668,#97669) ;
#76148=AXIS2_PLACEMENT_3D('',#123520,#97670,#97671) ;
#76149=AXIS2_PLACEMENT_3D('',#123521,#97672,#97673) ;
#76150=AXIS2_PLACEMENT_3D('',#123522,#97674,#97675) ;
#76151=AXIS2_PLACEMENT_3D('',#123523,#97676,#97677) ;
#76152=AXIS2_PLACEMENT_3D('',#123524,#97678,#97679) ;
#76153=AXIS2_PLACEMENT_3D('',#123525,#97680,#97681) ;
#76154=AXIS2_PLACEMENT_3D('',#123526,#97682,#97683) ;
#76155=AXIS2_PLACEMENT_3D('',#123527,#97684,#97685) ;
#76156=AXIS2_PLACEMENT_3D('',#123528,#97686,#97687) ;
#76157=AXIS2_PLACEMENT_3D('',#123529,#97688,#97689) ;
#76158=AXIS2_PLACEMENT_3D('',#123530,#97690,#97691) ;
#76159=AXIS2_PLACEMENT_3D('',#123531,#97692,#97693) ;
#76160=AXIS2_PLACEMENT_3D('',#123532,#97694,#97695) ;
#76161=AXIS2_PLACEMENT_3D('',#123533,#97696,#97697) ;
#76162=AXIS2_PLACEMENT_3D('',#123534,#97698,#97699) ;
#76163=AXIS2_PLACEMENT_3D('',#123535,#97700,#97701) ;
#76164=AXIS2_PLACEMENT_3D('',#123536,#97702,#97703) ;
#76165=AXIS2_PLACEMENT_3D('',#123537,#97704,#97705) ;
#76166=AXIS2_PLACEMENT_3D('',#123538,#97706,#97707) ;
#76167=AXIS2_PLACEMENT_3D('',#123539,#97708,#97709) ;
#76168=AXIS2_PLACEMENT_3D('',#123540,#97710,#97711) ;
#76169=AXIS2_PLACEMENT_3D('',#123541,#97712,#97713) ;
#76170=AXIS2_PLACEMENT_3D('',#123542,#97714,#97715) ;
#76171=AXIS2_PLACEMENT_3D('',#123543,#97716,#97717) ;
#76172=AXIS2_PLACEMENT_3D('',#123544,#97718,#97719) ;
#76173=AXIS2_PLACEMENT_3D('',#123545,#97720,#97721) ;
#76174=AXIS2_PLACEMENT_3D('',#123546,#97722,#97723) ;
#76175=AXIS2_PLACEMENT_3D('',#123547,#97724,#97725) ;
#76176=AXIS2_PLACEMENT_3D('',#123548,#97726,#97727) ;
#76177=AXIS2_PLACEMENT_3D('',#123549,#97728,#97729) ;
#76178=AXIS2_PLACEMENT_3D('',#123550,#97730,#97731) ;
#76179=AXIS2_PLACEMENT_3D('',#123551,#97732,#97733) ;
#76180=AXIS2_PLACEMENT_3D('',#123552,#97734,#97735) ;
#76181=AXIS2_PLACEMENT_3D('',#123553,#97736,#97737) ;
#76182=AXIS2_PLACEMENT_3D('',#123554,#97738,#97739) ;
#76183=AXIS2_PLACEMENT_3D('',#123555,#97740,#97741) ;
#76184=AXIS2_PLACEMENT_3D('',#123556,#97742,#97743) ;
#76185=AXIS2_PLACEMENT_3D('',#123557,#97744,#97745) ;
#76186=AXIS2_PLACEMENT_3D('',#123558,#97746,#97747) ;
#76187=AXIS2_PLACEMENT_3D('',#123559,#97748,#97749) ;
#76188=AXIS2_PLACEMENT_3D('',#123560,#97750,#97751) ;
#76189=AXIS2_PLACEMENT_3D('',#123561,#97752,#97753) ;
#76190=AXIS2_PLACEMENT_3D('',#123562,#97754,#97755) ;
#76191=AXIS2_PLACEMENT_3D('',#123563,#97756,#97757) ;
#76192=AXIS2_PLACEMENT_3D('',#123564,#97758,#97759) ;
#76193=AXIS2_PLACEMENT_3D('',#123565,#97760,#97761) ;
#76194=AXIS2_PLACEMENT_3D('',#123566,#97762,#97763) ;
#76195=AXIS2_PLACEMENT_3D('',#123567,#97764,#97765) ;
#76196=AXIS2_PLACEMENT_3D('',#123568,#97766,#97767) ;
#76197=AXIS2_PLACEMENT_3D('',#123569,#97768,#97769) ;
#76198=AXIS2_PLACEMENT_3D('',#123570,#97770,#97771) ;
#76199=AXIS2_PLACEMENT_3D('',#123571,#97772,#97773) ;
#76200=AXIS2_PLACEMENT_3D('',#123572,#97774,#97775) ;
#76201=AXIS2_PLACEMENT_3D('',#123573,#97776,#97777) ;
#76202=AXIS2_PLACEMENT_3D('',#123574,#97778,#97779) ;
#76203=AXIS2_PLACEMENT_3D('',#123575,#97780,#97781) ;
#76204=AXIS2_PLACEMENT_3D('',#123576,#97782,#97783) ;
#76205=AXIS2_PLACEMENT_3D('',#123577,#97784,#97785) ;
#76206=AXIS2_PLACEMENT_3D('',#123578,#97786,#97787) ;
#76207=AXIS2_PLACEMENT_3D('',#123579,#97788,#97789) ;
#76208=AXIS2_PLACEMENT_3D('',#123580,#97790,#97791) ;
#76209=AXIS2_PLACEMENT_3D('',#123581,#97792,#97793) ;
#76210=AXIS2_PLACEMENT_3D('',#123582,#97794,#97795) ;
#76211=AXIS2_PLACEMENT_3D('',#123583,#97796,#97797) ;
#76212=AXIS2_PLACEMENT_3D('',#123584,#97798,#97799) ;
#76213=AXIS2_PLACEMENT_3D('',#123585,#97800,#97801) ;
#76214=AXIS2_PLACEMENT_3D('',#123586,#97802,#97803) ;
#76215=AXIS2_PLACEMENT_3D('',#123587,#97804,#97805) ;
#76216=AXIS2_PLACEMENT_3D('',#123588,#97806,#97807) ;
#76217=AXIS2_PLACEMENT_3D('',#123589,#97808,#97809) ;
#76218=AXIS2_PLACEMENT_3D('',#123590,#97810,#97811) ;
#76219=AXIS2_PLACEMENT_3D('',#123591,#97812,#97813) ;
#76220=AXIS2_PLACEMENT_3D('',#123592,#97814,#97815) ;
#76221=AXIS2_PLACEMENT_3D('',#123593,#97816,#97817) ;
#76222=AXIS2_PLACEMENT_3D('',#123594,#97818,#97819) ;
#76223=AXIS2_PLACEMENT_3D('',#123595,#97820,#97821) ;
#76224=AXIS2_PLACEMENT_3D('',#123596,#97822,#97823) ;
#76225=AXIS2_PLACEMENT_3D('',#123597,#97824,#97825) ;
#76226=AXIS2_PLACEMENT_3D('',#123598,#97826,#97827) ;
#76227=AXIS2_PLACEMENT_3D('',#123599,#97828,#97829) ;
#76228=AXIS2_PLACEMENT_3D('',#123600,#97830,#97831) ;
#76229=AXIS2_PLACEMENT_3D('',#123601,#97832,#97833) ;
#76230=AXIS2_PLACEMENT_3D('',#123602,#97834,#97835) ;
#76231=AXIS2_PLACEMENT_3D('',#123603,#97836,#97837) ;
#76232=AXIS2_PLACEMENT_3D('',#123604,#97838,#97839) ;
#76233=AXIS2_PLACEMENT_3D('',#123605,#97840,#97841) ;
#76234=AXIS2_PLACEMENT_3D('',#123606,#97842,#97843) ;
#76235=AXIS2_PLACEMENT_3D('',#123607,#97844,#97845) ;
#76236=AXIS2_PLACEMENT_3D('',#123608,#97846,#97847) ;
#76237=AXIS2_PLACEMENT_3D('',#123609,#97848,#97849) ;
#76238=AXIS2_PLACEMENT_3D('',#123610,#97850,#97851) ;
#76239=AXIS2_PLACEMENT_3D('',#123611,#97852,#97853) ;
#76240=AXIS2_PLACEMENT_3D('',#123612,#97854,#97855) ;
#76241=AXIS2_PLACEMENT_3D('',#123613,#97856,#97857) ;
#76242=AXIS2_PLACEMENT_3D('',#123614,#97858,#97859) ;
#76243=AXIS2_PLACEMENT_3D('',#123615,#97860,#97861) ;
#76244=AXIS2_PLACEMENT_3D('',#123616,#97862,#97863) ;
#76245=AXIS2_PLACEMENT_3D('',#123617,#97864,#97865) ;
#76246=AXIS2_PLACEMENT_3D('',#123618,#97866,#97867) ;
#76247=AXIS2_PLACEMENT_3D('',#123619,#97868,#97869) ;
#76248=AXIS2_PLACEMENT_3D('',#123620,#97870,#97871) ;
#76249=AXIS2_PLACEMENT_3D('',#123621,#97872,#97873) ;
#76250=AXIS2_PLACEMENT_3D('',#123622,#97874,#97875) ;
#76251=AXIS2_PLACEMENT_3D('',#123623,#97876,#97877) ;
#76252=AXIS2_PLACEMENT_3D('',#123624,#97878,#97879) ;
#76253=AXIS2_PLACEMENT_3D('',#123625,#97880,#97881) ;
#76254=AXIS2_PLACEMENT_3D('',#123626,#97882,#97883) ;
#76255=AXIS2_PLACEMENT_3D('',#123627,#97884,#97885) ;
#76256=AXIS2_PLACEMENT_3D('',#123628,#97886,#97887) ;
#76257=AXIS2_PLACEMENT_3D('',#123629,#97888,#97889) ;
#76258=AXIS2_PLACEMENT_3D('',#123630,#97890,#97891) ;
#76259=AXIS2_PLACEMENT_3D('',#123631,#97892,#97893) ;
#76260=AXIS2_PLACEMENT_3D('',#123632,#97894,#97895) ;
#76261=AXIS2_PLACEMENT_3D('',#123633,#97896,#97897) ;
#76262=AXIS2_PLACEMENT_3D('',#123634,#97898,#97899) ;
#76263=AXIS2_PLACEMENT_3D('',#123635,#97900,#97901) ;
#76264=AXIS2_PLACEMENT_3D('',#123636,#97902,#97903) ;
#76265=AXIS2_PLACEMENT_3D('',#123637,#97904,#97905) ;
#76266=AXIS2_PLACEMENT_3D('',#123638,#97906,#97907) ;
#76267=AXIS2_PLACEMENT_3D('',#123639,#97908,#97909) ;
#76268=AXIS2_PLACEMENT_3D('',#123640,#97910,#97911) ;
#76269=AXIS2_PLACEMENT_3D('',#123641,#97912,#97913) ;
#76270=AXIS2_PLACEMENT_3D('',#123642,#97914,#97915) ;
#76271=AXIS2_PLACEMENT_3D('',#123643,#97916,#97917) ;
#76272=AXIS2_PLACEMENT_3D('',#123644,#97918,#97919) ;
#76273=AXIS2_PLACEMENT_3D('',#123645,#97920,#97921) ;
#76274=AXIS2_PLACEMENT_3D('',#123646,#97922,#97923) ;
#76275=AXIS2_PLACEMENT_3D('',#123647,#97924,#97925) ;
#76276=AXIS2_PLACEMENT_3D('',#123648,#97926,#97927) ;
#76277=AXIS2_PLACEMENT_3D('',#123649,#97928,#97929) ;
#76278=AXIS2_PLACEMENT_3D('',#123650,#97930,#97931) ;
#76279=AXIS2_PLACEMENT_3D('',#123651,#97932,#97933) ;
#76280=AXIS2_PLACEMENT_3D('',#123652,#97934,#97935) ;
#76281=AXIS2_PLACEMENT_3D('',#123653,#97936,#97937) ;
#76282=AXIS2_PLACEMENT_3D('',#123654,#97938,#97939) ;
#76283=AXIS2_PLACEMENT_3D('',#123655,#97940,#97941) ;
#76284=AXIS2_PLACEMENT_3D('',#123656,#97942,#97943) ;
#76285=AXIS2_PLACEMENT_3D('',#123657,#97944,#97945) ;
#76286=AXIS2_PLACEMENT_3D('',#123658,#97946,#97947) ;
#76287=AXIS2_PLACEMENT_3D('',#123659,#97948,#97949) ;
#76288=AXIS2_PLACEMENT_3D('',#123660,#97950,#97951) ;
#76289=AXIS2_PLACEMENT_3D('',#123661,#97952,#97953) ;
#76290=AXIS2_PLACEMENT_3D('',#123662,#97954,#97955) ;
#76291=AXIS2_PLACEMENT_3D('',#123663,#97956,#97957) ;
#76292=AXIS2_PLACEMENT_3D('',#123664,#97958,#97959) ;
#76293=AXIS2_PLACEMENT_3D('',#123665,#97960,#97961) ;
#76294=AXIS2_PLACEMENT_3D('',#123666,#97962,#97963) ;
#76295=AXIS2_PLACEMENT_3D('',#123667,#97964,#97965) ;
#76296=AXIS2_PLACEMENT_3D('',#123668,#97966,#97967) ;
#76297=AXIS2_PLACEMENT_3D('',#123669,#97968,#97969) ;
#76298=AXIS2_PLACEMENT_3D('',#123670,#97970,#97971) ;
#76299=AXIS2_PLACEMENT_3D('',#123671,#97972,#97973) ;
#76300=AXIS2_PLACEMENT_3D('',#123672,#97974,#97975) ;
#76301=AXIS2_PLACEMENT_3D('',#123673,#97976,#97977) ;
#76302=AXIS2_PLACEMENT_3D('',#123674,#97978,#97979) ;
#76303=AXIS2_PLACEMENT_3D('',#123675,#97980,#97981) ;
#76304=AXIS2_PLACEMENT_3D('',#123676,#97982,#97983) ;
#76305=AXIS2_PLACEMENT_3D('',#123677,#97984,#97985) ;
#76306=AXIS2_PLACEMENT_3D('',#123678,#97986,#97987) ;
#76307=AXIS2_PLACEMENT_3D('',#123679,#97988,#97989) ;
#76308=AXIS2_PLACEMENT_3D('',#123680,#97990,#97991) ;
#76309=AXIS2_PLACEMENT_3D('',#123681,#97992,#97993) ;
#76310=AXIS2_PLACEMENT_3D('',#123682,#97994,#97995) ;
#76311=AXIS2_PLACEMENT_3D('',#123683,#97996,#97997) ;
#76312=AXIS2_PLACEMENT_3D('',#123684,#97998,#97999) ;
#76313=AXIS2_PLACEMENT_3D('',#123685,#98000,#98001) ;
#76314=AXIS2_PLACEMENT_3D('',#123686,#98002,#98003) ;
#76315=AXIS2_PLACEMENT_3D('',#123687,#98004,#98005) ;
#76316=AXIS2_PLACEMENT_3D('',#123688,#98006,#98007) ;
#76317=AXIS2_PLACEMENT_3D('',#123689,#98008,#98009) ;
#76318=AXIS2_PLACEMENT_3D('',#123690,#98010,#98011) ;
#76319=AXIS2_PLACEMENT_3D('',#123691,#98012,#98013) ;
#76320=AXIS2_PLACEMENT_3D('',#123692,#98014,#98015) ;
#76321=AXIS2_PLACEMENT_3D('',#123693,#98016,#98017) ;
#76322=AXIS2_PLACEMENT_3D('',#123694,#98018,#98019) ;
#76323=AXIS2_PLACEMENT_3D('',#123695,#98020,#98021) ;
#76324=AXIS2_PLACEMENT_3D('',#123696,#98022,#98023) ;
#76325=AXIS2_PLACEMENT_3D('',#123697,#98024,#98025) ;
#76326=AXIS2_PLACEMENT_3D('',#123698,#98026,#98027) ;
#76327=AXIS2_PLACEMENT_3D('',#123699,#98028,#98029) ;
#76328=AXIS2_PLACEMENT_3D('',#123700,#98030,#98031) ;
#76329=AXIS2_PLACEMENT_3D('',#123701,#98032,#98033) ;
#76330=AXIS2_PLACEMENT_3D('',#123702,#98034,#98035) ;
#76331=AXIS2_PLACEMENT_3D('',#123703,#98036,#98037) ;
#76332=AXIS2_PLACEMENT_3D('',#123704,#98038,#98039) ;
#76333=AXIS2_PLACEMENT_3D('',#123705,#98040,#98041) ;
#76334=AXIS2_PLACEMENT_3D('',#123706,#98042,#98043) ;
#76335=AXIS2_PLACEMENT_3D('',#123707,#98044,#98045) ;
#76336=AXIS2_PLACEMENT_3D('',#123708,#98046,#98047) ;
#76337=AXIS2_PLACEMENT_3D('',#123709,#98048,#98049) ;
#76338=AXIS2_PLACEMENT_3D('',#123710,#98050,#98051) ;
#76339=AXIS2_PLACEMENT_3D('',#123711,#98052,#98053) ;
#76340=AXIS2_PLACEMENT_3D('',#123712,#98054,#98055) ;
#76341=AXIS2_PLACEMENT_3D('',#123713,#98056,#98057) ;
#76342=AXIS2_PLACEMENT_3D('',#123714,#98058,#98059) ;
#76343=AXIS2_PLACEMENT_3D('',#123715,#98060,#98061) ;
#76344=AXIS2_PLACEMENT_3D('',#123716,#98062,#98063) ;
#76345=AXIS2_PLACEMENT_3D('',#123717,#98064,#98065) ;
#76346=AXIS2_PLACEMENT_3D('',#123718,#98066,#98067) ;
#76347=AXIS2_PLACEMENT_3D('',#123719,#98068,#98069) ;
#76348=AXIS2_PLACEMENT_3D('',#123720,#98070,#98071) ;
#76349=AXIS2_PLACEMENT_3D('',#123721,#98072,#98073) ;
#76350=AXIS2_PLACEMENT_3D('',#123722,#98074,#98075) ;
#76351=AXIS2_PLACEMENT_3D('',#123723,#98076,#98077) ;
#76352=AXIS2_PLACEMENT_3D('',#123724,#98078,#98079) ;
#76353=AXIS2_PLACEMENT_3D('',#123725,#98080,#98081) ;
#76354=AXIS2_PLACEMENT_3D('',#123726,#98082,#98083) ;
#76355=AXIS2_PLACEMENT_3D('',#123727,#98084,#98085) ;
#76356=AXIS2_PLACEMENT_3D('',#123728,#98086,#98087) ;
#76357=AXIS2_PLACEMENT_3D('',#123729,#98088,#98089) ;
#76358=AXIS2_PLACEMENT_3D('',#123730,#98090,#98091) ;
#76359=AXIS2_PLACEMENT_3D('',#123731,#98092,#98093) ;
#76360=AXIS2_PLACEMENT_3D('',#123732,#98094,#98095) ;
#76361=AXIS2_PLACEMENT_3D('',#123733,#98096,#98097) ;
#76362=AXIS2_PLACEMENT_3D('',#123734,#98098,#98099) ;
#76363=AXIS2_PLACEMENT_3D('',#123735,#98100,#98101) ;
#76364=AXIS2_PLACEMENT_3D('',#123736,#98102,#98103) ;
#76365=AXIS2_PLACEMENT_3D('',#123737,#98104,#98105) ;
#76366=AXIS2_PLACEMENT_3D('',#123738,#98106,#98107) ;
#76367=AXIS2_PLACEMENT_3D('',#123739,#98108,#98109) ;
#76368=AXIS2_PLACEMENT_3D('',#123740,#98110,#98111) ;
#76369=AXIS2_PLACEMENT_3D('',#123741,#98112,#98113) ;
#76370=AXIS2_PLACEMENT_3D('',#123742,#98114,#98115) ;
#76371=AXIS2_PLACEMENT_3D('',#123743,#98116,#98117) ;
#76372=AXIS2_PLACEMENT_3D('',#123744,#98118,#98119) ;
#76373=AXIS2_PLACEMENT_3D('',#123745,#98120,#98121) ;
#76374=AXIS2_PLACEMENT_3D('',#123746,#98122,#98123) ;
#76375=AXIS2_PLACEMENT_3D('',#123747,#98124,#98125) ;
#76376=AXIS2_PLACEMENT_3D('',#123748,#98126,#98127) ;
#76377=AXIS2_PLACEMENT_3D('',#123749,#98128,#98129) ;
#76378=AXIS2_PLACEMENT_3D('',#123750,#98130,#98131) ;
#76379=AXIS2_PLACEMENT_3D('',#123751,#98132,#98133) ;
#76380=AXIS2_PLACEMENT_3D('',#123752,#98134,#98135) ;
#76381=AXIS2_PLACEMENT_3D('',#123753,#98136,#98137) ;
#76382=AXIS2_PLACEMENT_3D('',#123754,#98138,#98139) ;
#76383=AXIS2_PLACEMENT_3D('',#123755,#98140,#98141) ;
#76384=AXIS2_PLACEMENT_3D('',#123756,#98142,#98143) ;
#76385=AXIS2_PLACEMENT_3D('',#123757,#98144,#98145) ;
#76386=AXIS2_PLACEMENT_3D('',#123758,#98146,#98147) ;
#76387=AXIS2_PLACEMENT_3D('',#123759,#98148,#98149) ;
#76388=AXIS2_PLACEMENT_3D('',#123760,#98150,#98151) ;
#76389=AXIS2_PLACEMENT_3D('',#123761,#98152,#98153) ;
#76390=AXIS2_PLACEMENT_3D('',#123762,#98154,#98155) ;
#76391=AXIS2_PLACEMENT_3D('',#123763,#98156,#98157) ;
#76392=AXIS2_PLACEMENT_3D('',#123764,#98158,#98159) ;
#76393=AXIS2_PLACEMENT_3D('',#123765,#98160,#98161) ;
#76394=AXIS2_PLACEMENT_3D('',#123766,#98162,#98163) ;
#76395=AXIS2_PLACEMENT_3D('',#123767,#98164,#98165) ;
#76396=AXIS2_PLACEMENT_3D('',#123768,#98166,#98167) ;
#76397=AXIS2_PLACEMENT_3D('',#123769,#98168,#98169) ;
#76398=AXIS2_PLACEMENT_3D('',#123770,#98170,#98171) ;
#76399=AXIS2_PLACEMENT_3D('',#123771,#98172,#98173) ;
#76400=AXIS2_PLACEMENT_3D('',#123772,#98174,#98175) ;
#76401=AXIS2_PLACEMENT_3D('',#123773,#98176,#98177) ;
#76402=AXIS2_PLACEMENT_3D('',#123774,#98178,#98179) ;
#76403=AXIS2_PLACEMENT_3D('',#123775,#98180,#98181) ;
#76404=AXIS2_PLACEMENT_3D('',#123776,#98182,#98183) ;
#76405=AXIS2_PLACEMENT_3D('',#123777,#98184,#98185) ;
#76406=AXIS2_PLACEMENT_3D('',#123778,#98186,#98187) ;
#76407=AXIS2_PLACEMENT_3D('',#123779,#98188,#98189) ;
#76408=AXIS2_PLACEMENT_3D('',#123780,#98190,#98191) ;
#76409=AXIS2_PLACEMENT_3D('',#123781,#98192,#98193) ;
#76410=AXIS2_PLACEMENT_3D('',#123782,#98194,#98195) ;
#76411=AXIS2_PLACEMENT_3D('',#123783,#98196,#98197) ;
#76412=AXIS2_PLACEMENT_3D('',#123784,#98198,#98199) ;
#76413=AXIS2_PLACEMENT_3D('',#123785,#98200,#98201) ;
#76414=AXIS2_PLACEMENT_3D('',#123786,#98202,#98203) ;
#76415=AXIS2_PLACEMENT_3D('',#123787,#98204,#98205) ;
#76416=AXIS2_PLACEMENT_3D('',#123788,#98206,#98207) ;
#76417=AXIS2_PLACEMENT_3D('',#123789,#98208,#98209) ;
#76418=AXIS2_PLACEMENT_3D('',#123790,#98210,#98211) ;
#76419=AXIS2_PLACEMENT_3D('',#123791,#98212,#98213) ;
#76420=AXIS2_PLACEMENT_3D('',#123792,#98214,#98215) ;
#76421=AXIS2_PLACEMENT_3D('',#123793,#98216,#98217) ;
#76422=AXIS2_PLACEMENT_3D('',#123794,#98218,#98219) ;
#76423=AXIS2_PLACEMENT_3D('',#123795,#98220,#98221) ;
#76424=AXIS2_PLACEMENT_3D('',#123796,#98222,#98223) ;
#76425=AXIS2_PLACEMENT_3D('',#123797,#98224,#98225) ;
#76426=AXIS2_PLACEMENT_3D('',#123798,#98226,#98227) ;
#76427=AXIS2_PLACEMENT_3D('',#123799,#98228,#98229) ;
#76428=AXIS2_PLACEMENT_3D('',#123800,#98230,#98231) ;
#76429=AXIS2_PLACEMENT_3D('',#123801,#98232,#98233) ;
#76430=AXIS2_PLACEMENT_3D('',#123802,#98234,#98235) ;
#76431=AXIS2_PLACEMENT_3D('',#123803,#98236,#98237) ;
#76432=AXIS2_PLACEMENT_3D('',#123804,#98238,#98239) ;
#76433=AXIS2_PLACEMENT_3D('',#123805,#98240,#98241) ;
#76434=AXIS2_PLACEMENT_3D('',#123806,#98242,#98243) ;
#76435=AXIS2_PLACEMENT_3D('',#123807,#98244,#98245) ;
#76436=AXIS2_PLACEMENT_3D('',#123808,#98246,#98247) ;
#76437=AXIS2_PLACEMENT_3D('',#123809,#98248,#98249) ;
#76438=AXIS2_PLACEMENT_3D('',#123810,#98250,#98251) ;
#76439=AXIS2_PLACEMENT_3D('',#123811,#98252,#98253) ;
#76440=AXIS2_PLACEMENT_3D('',#123812,#98254,#98255) ;
#76441=AXIS2_PLACEMENT_3D('',#123813,#98256,#98257) ;
#76442=AXIS2_PLACEMENT_3D('',#123814,#98258,#98259) ;
#76443=AXIS2_PLACEMENT_3D('',#123815,#98260,#98261) ;
#76444=AXIS2_PLACEMENT_3D('',#123816,#98262,#98263) ;
#76445=AXIS2_PLACEMENT_3D('',#123817,#98264,#98265) ;
#76446=AXIS2_PLACEMENT_3D('',#123818,#98266,#98267) ;
#76447=AXIS2_PLACEMENT_3D('',#123819,#98268,#98269) ;
#76448=AXIS2_PLACEMENT_3D('',#123820,#98270,#98271) ;
#76449=AXIS2_PLACEMENT_3D('',#123821,#98272,#98273) ;
#76450=AXIS2_PLACEMENT_3D('',#123822,#98274,#98275) ;
#76451=AXIS2_PLACEMENT_3D('',#123823,#98276,#98277) ;
#76452=AXIS2_PLACEMENT_3D('',#123824,#98278,#98279) ;
#76453=AXIS2_PLACEMENT_3D('',#123825,#98280,#98281) ;
#76454=AXIS2_PLACEMENT_3D('',#123826,#98282,#98283) ;
#76455=AXIS2_PLACEMENT_3D('',#123827,#98284,#98285) ;
#76456=AXIS2_PLACEMENT_3D('',#123828,#98286,#98287) ;
#76457=AXIS2_PLACEMENT_3D('',#123829,#98288,#98289) ;
#76458=AXIS2_PLACEMENT_3D('',#123830,#98290,#98291) ;
#76459=AXIS2_PLACEMENT_3D('',#123831,#98292,#98293) ;
#76460=AXIS2_PLACEMENT_3D('',#123832,#98294,#98295) ;
#76461=AXIS2_PLACEMENT_3D('',#123833,#98296,#98297) ;
#76462=AXIS2_PLACEMENT_3D('',#123834,#98298,#98299) ;
#76463=AXIS2_PLACEMENT_3D('',#123835,#98300,#98301) ;
#76464=AXIS2_PLACEMENT_3D('',#123836,#98302,#98303) ;
#76465=AXIS2_PLACEMENT_3D('',#123837,#98304,#98305) ;
#76466=AXIS2_PLACEMENT_3D('',#123838,#98306,#98307) ;
#76467=AXIS2_PLACEMENT_3D('',#123839,#98308,#98309) ;
#76468=AXIS2_PLACEMENT_3D('',#123840,#98310,#98311) ;
#76469=AXIS2_PLACEMENT_3D('',#123841,#98312,#98313) ;
#76470=AXIS2_PLACEMENT_3D('',#123842,#98314,#98315) ;
#76471=AXIS2_PLACEMENT_3D('',#123843,#98316,#98317) ;
#76472=AXIS2_PLACEMENT_3D('',#123844,#98318,#98319) ;
#76473=AXIS2_PLACEMENT_3D('',#123845,#98320,#98321) ;
#76474=AXIS2_PLACEMENT_3D('',#123846,#98322,#98323) ;
#76475=AXIS2_PLACEMENT_3D('',#123847,#98324,#98325) ;
#76476=AXIS2_PLACEMENT_3D('',#123848,#98326,#98327) ;
#76477=AXIS2_PLACEMENT_3D('',#123849,#98328,#98329) ;
#76478=AXIS2_PLACEMENT_3D('',#123850,#98330,#98331) ;
#76479=AXIS2_PLACEMENT_3D('',#123851,#98332,#98333) ;
#76480=AXIS2_PLACEMENT_3D('',#123852,#98334,#98335) ;
#76481=AXIS2_PLACEMENT_3D('',#123853,#98336,#98337) ;
#76482=AXIS2_PLACEMENT_3D('',#123854,#98338,#98339) ;
#76483=AXIS2_PLACEMENT_3D('',#123855,#98340,#98341) ;
#76484=AXIS2_PLACEMENT_3D('',#123856,#98342,#98343) ;
#76485=AXIS2_PLACEMENT_3D('',#123857,#98344,#98345) ;
#76486=AXIS2_PLACEMENT_3D('',#123858,#98346,#98347) ;
#76487=AXIS2_PLACEMENT_3D('',#123859,#98348,#98349) ;
#76488=AXIS2_PLACEMENT_3D('',#123860,#98350,#98351) ;
#76489=AXIS2_PLACEMENT_3D('',#123861,#98352,#98353) ;
#76490=AXIS2_PLACEMENT_3D('',#123862,#98354,#98355) ;
#76491=AXIS2_PLACEMENT_3D('',#123863,#98356,#98357) ;
#76492=AXIS2_PLACEMENT_3D('',#123864,#98358,#98359) ;
#76493=AXIS2_PLACEMENT_3D('',#123865,#98360,#98361) ;
#76494=AXIS2_PLACEMENT_3D('',#123866,#98362,#98363) ;
#76495=AXIS2_PLACEMENT_3D('',#123867,#98364,#98365) ;
#76496=AXIS2_PLACEMENT_3D('',#123868,#98366,#98367) ;
#76497=AXIS2_PLACEMENT_3D('',#123869,#98368,#98369) ;
#76498=AXIS2_PLACEMENT_3D('',#123870,#98370,#98371) ;
#76499=AXIS2_PLACEMENT_3D('',#123871,#98372,#98373) ;
#76500=AXIS2_PLACEMENT_3D('',#123872,#98374,#98375) ;
#76501=AXIS2_PLACEMENT_3D('',#123873,#98376,#98377) ;
#76502=AXIS2_PLACEMENT_3D('',#123874,#98378,#98379) ;
#76503=AXIS2_PLACEMENT_3D('',#123875,#98380,#98381) ;
#76504=AXIS2_PLACEMENT_3D('',#123876,#98382,#98383) ;
#76505=AXIS2_PLACEMENT_3D('',#123877,#98384,#98385) ;
#76506=AXIS2_PLACEMENT_3D('',#123878,#98386,#98387) ;
#76507=AXIS2_PLACEMENT_3D('',#123879,#98388,#98389) ;
#76508=AXIS2_PLACEMENT_3D('',#123880,#98390,#98391) ;
#76509=AXIS2_PLACEMENT_3D('',#123881,#98392,#98393) ;
#76510=AXIS2_PLACEMENT_3D('',#123882,#98394,#98395) ;
#76511=AXIS2_PLACEMENT_3D('',#123883,#98396,#98397) ;
#76512=AXIS2_PLACEMENT_3D('',#123884,#98398,#98399) ;
#76513=AXIS2_PLACEMENT_3D('',#123885,#98400,#98401) ;
#76514=AXIS2_PLACEMENT_3D('',#123886,#98402,#98403) ;
#76515=AXIS2_PLACEMENT_3D('',#123887,#98404,#98405) ;
#76516=AXIS2_PLACEMENT_3D('',#123888,#98406,#98407) ;
#76517=AXIS2_PLACEMENT_3D('',#123889,#98408,#98409) ;
#76518=AXIS2_PLACEMENT_3D('',#123890,#98410,#98411) ;
#76519=AXIS2_PLACEMENT_3D('',#123891,#98412,#98413) ;
#76520=AXIS2_PLACEMENT_3D('',#123892,#98414,#98415) ;
#76521=AXIS2_PLACEMENT_3D('',#123893,#98416,#98417) ;
#76522=AXIS2_PLACEMENT_3D('',#123894,#98418,#98419) ;
#76523=AXIS2_PLACEMENT_3D('',#123895,#98420,#98421) ;
#76524=AXIS2_PLACEMENT_3D('',#123896,#98422,#98423) ;
#76525=AXIS2_PLACEMENT_3D('',#123897,#98424,#98425) ;
#76526=AXIS2_PLACEMENT_3D('',#123898,#98426,#98427) ;
#76527=AXIS2_PLACEMENT_3D('',#123899,#98428,#98429) ;
#76528=AXIS2_PLACEMENT_3D('',#123900,#98430,#98431) ;
#76529=AXIS2_PLACEMENT_3D('',#123901,#98432,#98433) ;
#76530=AXIS2_PLACEMENT_3D('',#123902,#98434,#98435) ;
#76531=AXIS2_PLACEMENT_3D('',#123903,#98436,#98437) ;
#76532=AXIS2_PLACEMENT_3D('',#123904,#98438,#98439) ;
#76533=AXIS2_PLACEMENT_3D('',#123905,#98440,#98441) ;
#76534=AXIS2_PLACEMENT_3D('',#123906,#98442,#98443) ;
#76535=AXIS2_PLACEMENT_3D('',#123907,#98444,#98445) ;
#76536=AXIS2_PLACEMENT_3D('',#123908,#98446,#98447) ;
#76537=AXIS2_PLACEMENT_3D('',#123909,#98448,#98449) ;
#76538=AXIS2_PLACEMENT_3D('',#123910,#98450,#98451) ;
#76539=AXIS2_PLACEMENT_3D('',#123911,#98452,#98453) ;
#76540=AXIS2_PLACEMENT_3D('',#123912,#98454,#98455) ;
#76541=AXIS2_PLACEMENT_3D('',#123913,#98456,#98457) ;
#76542=AXIS2_PLACEMENT_3D('',#123914,#98458,#98459) ;
#76543=AXIS2_PLACEMENT_3D('',#123915,#98460,#98461) ;
#76544=AXIS2_PLACEMENT_3D('',#123916,#98462,#98463) ;
#76545=AXIS2_PLACEMENT_3D('',#123917,#98464,#98465) ;
#76546=AXIS2_PLACEMENT_3D('',#123918,#98466,#98467) ;
#76547=AXIS2_PLACEMENT_3D('',#123919,#98468,#98469) ;
#76548=AXIS2_PLACEMENT_3D('',#123920,#98470,#98471) ;
#76549=AXIS2_PLACEMENT_3D('',#123921,#98472,#98473) ;
#76550=AXIS2_PLACEMENT_3D('',#123922,#98474,#98475) ;
#76551=AXIS2_PLACEMENT_3D('',#123923,#98476,#98477) ;
#76552=AXIS2_PLACEMENT_3D('',#123924,#98478,#98479) ;
#76553=AXIS2_PLACEMENT_3D('',#123925,#98480,#98481) ;
#76554=AXIS2_PLACEMENT_3D('',#123926,#98482,#98483) ;
#76555=AXIS2_PLACEMENT_3D('',#123927,#98484,#98485) ;
#76556=AXIS2_PLACEMENT_3D('',#123928,#98486,#98487) ;
#76557=AXIS2_PLACEMENT_3D('',#123929,#98488,#98489) ;
#76558=AXIS2_PLACEMENT_3D('',#123930,#98490,#98491) ;
#76559=AXIS2_PLACEMENT_3D('',#123931,#98492,#98493) ;
#76560=AXIS2_PLACEMENT_3D('',#123932,#98494,#98495) ;
#76561=AXIS2_PLACEMENT_3D('',#123933,#98496,#98497) ;
#76562=AXIS2_PLACEMENT_3D('',#123934,#98498,#98499) ;
#76563=AXIS2_PLACEMENT_3D('',#123935,#98500,#98501) ;
#76564=AXIS2_PLACEMENT_3D('',#123936,#98502,#98503) ;
#76565=AXIS2_PLACEMENT_3D('',#123937,#98504,#98505) ;
#76566=AXIS2_PLACEMENT_3D('',#123938,#98506,#98507) ;
#76567=AXIS2_PLACEMENT_3D('',#123939,#98508,#98509) ;
#76568=AXIS2_PLACEMENT_3D('',#123940,#98510,#98511) ;
#76569=AXIS2_PLACEMENT_3D('',#123941,#98512,#98513) ;
#76570=AXIS2_PLACEMENT_3D('',#123942,#98514,#98515) ;
#76571=AXIS2_PLACEMENT_3D('',#123943,#98516,#98517) ;
#76572=AXIS2_PLACEMENT_3D('',#123944,#98518,#98519) ;
#76573=AXIS2_PLACEMENT_3D('',#123945,#98520,#98521) ;
#76574=AXIS2_PLACEMENT_3D('',#123946,#98522,#98523) ;
#76575=AXIS2_PLACEMENT_3D('',#123947,#98524,#98525) ;
#76576=AXIS2_PLACEMENT_3D('',#123948,#98526,#98527) ;
#76577=AXIS2_PLACEMENT_3D('',#123949,#98528,#98529) ;
#76578=AXIS2_PLACEMENT_3D('',#123950,#98530,#98531) ;
#76579=AXIS2_PLACEMENT_3D('',#123951,#98532,#98533) ;
#76580=AXIS2_PLACEMENT_3D('',#123952,#98534,#98535) ;
#76581=AXIS2_PLACEMENT_3D('',#123953,#98536,#98537) ;
#76582=AXIS2_PLACEMENT_3D('',#123954,#98538,#98539) ;
#76583=AXIS2_PLACEMENT_3D('',#123955,#98540,#98541) ;
#76584=AXIS2_PLACEMENT_3D('',#123956,#98542,#98543) ;
#76585=AXIS2_PLACEMENT_3D('',#123957,#98544,#98545) ;
#76586=AXIS2_PLACEMENT_3D('',#123958,#98546,#98547) ;
#76587=AXIS2_PLACEMENT_3D('',#123959,#98548,#98549) ;
#76588=AXIS2_PLACEMENT_3D('',#123960,#98550,#98551) ;
#76589=AXIS2_PLACEMENT_3D('',#123961,#98552,#98553) ;
#76590=AXIS2_PLACEMENT_3D('',#123962,#98554,#98555) ;
#76591=AXIS2_PLACEMENT_3D('',#123963,#98556,#98557) ;
#76592=AXIS2_PLACEMENT_3D('',#123964,#98558,#98559) ;
#76593=AXIS2_PLACEMENT_3D('',#123965,#98560,#98561) ;
#76594=AXIS2_PLACEMENT_3D('',#123966,#98562,#98563) ;
#76595=AXIS2_PLACEMENT_3D('',#123967,#98564,#98565) ;
#76596=AXIS2_PLACEMENT_3D('',#123968,#98566,#98567) ;
#76597=AXIS2_PLACEMENT_3D('',#123969,#98568,#98569) ;
#76598=AXIS2_PLACEMENT_3D('',#123970,#98570,#98571) ;
#76599=AXIS2_PLACEMENT_3D('',#123971,#98572,#98573) ;
#76600=AXIS2_PLACEMENT_3D('',#123972,#98574,#98575) ;
#76601=AXIS2_PLACEMENT_3D('',#123973,#98576,#98577) ;
#76602=AXIS2_PLACEMENT_3D('',#123974,#98578,#98579) ;
#76603=AXIS2_PLACEMENT_3D('',#123975,#98580,#98581) ;
#76604=AXIS2_PLACEMENT_3D('',#123976,#98582,#98583) ;
#76605=AXIS2_PLACEMENT_3D('',#123977,#98584,#98585) ;
#76606=AXIS2_PLACEMENT_3D('',#123978,#98586,#98587) ;
#76607=AXIS2_PLACEMENT_3D('',#123979,#98588,#98589) ;
#76608=AXIS2_PLACEMENT_3D('',#123980,#98590,#98591) ;
#76609=AXIS2_PLACEMENT_3D('',#123981,#98592,#98593) ;
#76610=AXIS2_PLACEMENT_3D('',#123982,#98594,#98595) ;
#76611=AXIS2_PLACEMENT_3D('',#123983,#98596,#98597) ;
#76612=AXIS2_PLACEMENT_3D('',#123984,#98598,#98599) ;
#76613=AXIS2_PLACEMENT_3D('',#123985,#98600,#98601) ;
#76614=AXIS2_PLACEMENT_3D('',#123986,#98602,#98603) ;
#76615=AXIS2_PLACEMENT_3D('',#123987,#98604,#98605) ;
#76616=AXIS2_PLACEMENT_3D('',#123988,#98606,#98607) ;
#76617=AXIS2_PLACEMENT_3D('',#123989,#98608,#98609) ;
#76618=AXIS2_PLACEMENT_3D('',#123990,#98610,#98611) ;
#76619=AXIS2_PLACEMENT_3D('',#123991,#98612,#98613) ;
#76620=AXIS2_PLACEMENT_3D('',#123992,#98614,#98615) ;
#76621=AXIS2_PLACEMENT_3D('',#123993,#98616,#98617) ;
#76622=AXIS2_PLACEMENT_3D('',#123994,#98618,#98619) ;
#76623=AXIS2_PLACEMENT_3D('',#123995,#98620,#98621) ;
#76624=AXIS2_PLACEMENT_3D('',#123996,#98622,#98623) ;
#76625=AXIS2_PLACEMENT_3D('',#123997,#98624,#98625) ;
#76626=AXIS2_PLACEMENT_3D('',#123998,#98626,#98627) ;
#76627=AXIS2_PLACEMENT_3D('',#123999,#98628,#98629) ;
#76628=AXIS2_PLACEMENT_3D('',#124000,#98630,#98631) ;
#76629=AXIS2_PLACEMENT_3D('',#124001,#98632,#98633) ;
#76630=AXIS2_PLACEMENT_3D('',#124002,#98634,#98635) ;
#76631=AXIS2_PLACEMENT_3D('',#124003,#98636,#98637) ;
#76632=AXIS2_PLACEMENT_3D('',#124004,#98638,#98639) ;
#76633=AXIS2_PLACEMENT_3D('',#124005,#98640,#98641) ;
#76634=AXIS2_PLACEMENT_3D('',#124006,#98642,#98643) ;
#76635=AXIS2_PLACEMENT_3D('',#124007,#98644,#98645) ;
#76636=AXIS2_PLACEMENT_3D('',#124008,#98646,#98647) ;
#76637=AXIS2_PLACEMENT_3D('',#124009,#98648,#98649) ;
#76638=AXIS2_PLACEMENT_3D('',#124010,#98650,#98651) ;
#76639=AXIS2_PLACEMENT_3D('',#124011,#98652,#98653) ;
#76640=AXIS2_PLACEMENT_3D('',#124012,#98654,#98655) ;
#76641=AXIS2_PLACEMENT_3D('',#124013,#98656,#98657) ;
#76642=AXIS2_PLACEMENT_3D('',#124014,#98658,#98659) ;
#76643=AXIS2_PLACEMENT_3D('',#124015,#98660,#98661) ;
#76644=AXIS2_PLACEMENT_3D('',#124016,#98662,#98663) ;
#76645=AXIS2_PLACEMENT_3D('',#124017,#98664,#98665) ;
#76646=AXIS2_PLACEMENT_3D('',#124018,#98666,#98667) ;
#76647=AXIS2_PLACEMENT_3D('',#124019,#98668,#98669) ;
#76648=AXIS2_PLACEMENT_3D('',#124020,#98670,#98671) ;
#76649=AXIS2_PLACEMENT_3D('',#124021,#98672,#98673) ;
#76650=AXIS2_PLACEMENT_3D('',#124022,#98674,#98675) ;
#76651=AXIS2_PLACEMENT_3D('',#124023,#98676,#98677) ;
#76652=AXIS2_PLACEMENT_3D('',#124024,#98678,#98679) ;
#76653=AXIS2_PLACEMENT_3D('',#124025,#98680,#98681) ;
#76654=AXIS2_PLACEMENT_3D('',#124026,#98682,#98683) ;
#76655=AXIS2_PLACEMENT_3D('',#124027,#98684,#98685) ;
#76656=AXIS2_PLACEMENT_3D('',#124028,#98686,#98687) ;
#76657=AXIS2_PLACEMENT_3D('',#124029,#98688,#98689) ;
#76658=AXIS2_PLACEMENT_3D('',#124030,#98690,#98691) ;
#76659=AXIS2_PLACEMENT_3D('',#124031,#98692,#98693) ;
#76660=AXIS2_PLACEMENT_3D('',#124032,#98694,#98695) ;
#76661=AXIS2_PLACEMENT_3D('',#124033,#98696,#98697) ;
#76662=AXIS2_PLACEMENT_3D('',#124034,#98698,#98699) ;
#76663=AXIS2_PLACEMENT_3D('',#124035,#98700,#98701) ;
#76664=AXIS2_PLACEMENT_3D('',#124036,#98702,#98703) ;
#76665=AXIS2_PLACEMENT_3D('',#124037,#98704,#98705) ;
#76666=AXIS2_PLACEMENT_3D('',#124038,#98706,#98707) ;
#76667=AXIS2_PLACEMENT_3D('',#124039,#98708,#98709) ;
#76668=AXIS2_PLACEMENT_3D('',#124040,#98710,#98711) ;
#86968=DIRECTION('axis',(0.,0.,1.)) ;
#86969=DIRECTION('refdir',(1.,0.,0.)) ;
#86970=DIRECTION('center_axis',(1.,0.,0.)) ;
#86971=DIRECTION('ref_axis',(0.,0.,-1.)) ;
#86972=DIRECTION('center_axis',(1.,0.,0.)) ;
#86973=DIRECTION('ref_axis',(0.,0.,-1.)) ;
#86974=DIRECTION('center_axis',(0.,-1.,-1.22464679914735E-16)) ;
#86975=DIRECTION('ref_axis',(0.,-1.22464679914735E-16,1.)) ;
#86976=DIRECTION('center_axis',(-1.,0.,0.)) ;
#86977=DIRECTION('ref_axis',(0.,0.,-1.)) ;
#86978=DIRECTION('center_axis',(-1.,0.,0.)) ;
#86979=DIRECTION('ref_axis',(0.,0.,-1.)) ;
#86980=DIRECTION('center_axis',(-1.,0.,0.)) ;
#86981=DIRECTION('ref_axis',(0.,0.,1.)) ;
#86982=DIRECTION('center_axis',(-1.,0.,0.)) ;
#86983=DIRECTION('ref_axis',(0.,0.,1.)) ;
#86984=DIRECTION('center_axis',(0.,1.,-1.22464679914735E-16)) ;
#86985=DIRECTION('ref_axis',(0.,-1.22464679914735E-16,-1.)) ;
#86986=DIRECTION('center_axis',(1.,0.,0.)) ;
#86987=DIRECTION('ref_axis',(0.,0.,1.)) ;
#86988=DIRECTION('center_axis',(0.,1.,0.)) ;
#86989=DIRECTION('ref_axis',(0.,0.,1.)) ;
#86990=DIRECTION('center_axis',(-1.,0.,0.)) ;
#86991=DIRECTION('ref_axis',(0.,0.,-1.)) ;
#86992=DIRECTION('center_axis',(0.,0.707106781186532,0.707106781186563)) ;
#86993=DIRECTION('ref_axis',(0.,-0.707106781186563,0.707106781186532)) ;
#86994=DIRECTION('center_axis',(0.,0.,-1.)) ;
#86995=DIRECTION('ref_axis',(-1.,0.,0.)) ;
#86996=DIRECTION('center_axis',(2.16840434497101E-16,-1.,1.30104260698261E-16)) ;
#86997=DIRECTION('ref_axis',(1.,2.16840434497101E-16,-1.09476442525376E-47)) ;
#86998=DIRECTION('center_axis',(-2.25262403289994E-12,-0.707106781186411,
-0.707106781186684)) ;
#86999=DIRECTION('ref_axis',(2.77642807980434E-11,0.707106781186684,-0.707106781186411)) ;
#87000=DIRECTION('center_axis',(-5.42101086242752E-16,1.,0.)) ;
#87001=DIRECTION('ref_axis',(1.,5.42101086242752E-16,0.)) ;
#87002=DIRECTION('',(-2.16840434497101E-16,1.,-1.30104260698261E-16)) ;
#87003=DIRECTION('center_axis',(0.,1.,0.)) ;
#87004=DIRECTION('ref_axis',(0.,0.,1.)) ;
#87005=DIRECTION('',(2.16840434497101E-16,-1.,1.30104260698261E-16)) ;
#87006=DIRECTION('',(2.16840434497101E-16,-1.,1.30104260698261E-16)) ;
#87007=DIRECTION('center_axis',(1.,0.,0.)) ;
#87008=DIRECTION('ref_axis',(0.,0.,-1.)) ;
#87009=DIRECTION('center_axis',(1.,0.,0.)) ;
#87010=DIRECTION('ref_axis',(0.,0.,-1.)) ;
#87011=DIRECTION('center_axis',(0.,-1.,-1.22464679914735E-16)) ;
#87012=DIRECTION('ref_axis',(0.,-1.22464679914735E-16,1.)) ;
#87013=DIRECTION('center_axis',(-1.,0.,0.)) ;
#87014=DIRECTION('ref_axis',(0.,0.,-1.)) ;
#87015=DIRECTION('center_axis',(-1.,0.,0.)) ;
#87016=DIRECTION('ref_axis',(0.,0.,-1.)) ;
#87017=DIRECTION('center_axis',(-1.,0.,0.)) ;
#87018=DIRECTION('ref_axis',(0.,0.,1.)) ;
#87019=DIRECTION('center_axis',(-1.,0.,0.)) ;
#87020=DIRECTION('ref_axis',(0.,0.,1.)) ;
#87021=DIRECTION('center_axis',(0.,1.,-1.22464679914735E-16)) ;
#87022=DIRECTION('ref_axis',(0.,-1.22464679914735E-16,-1.)) ;
#87023=DIRECTION('center_axis',(1.,0.,0.)) ;
#87024=DIRECTION('ref_axis',(0.,0.,1.)) ;
#87025=DIRECTION('center_axis',(0.,1.,0.)) ;
#87026=DIRECTION('ref_axis',(0.,0.,1.)) ;
#87027=DIRECTION('center_axis',(-1.,0.,0.)) ;
#87028=DIRECTION('ref_axis',(0.,0.,-1.)) ;
#87029=DIRECTION('center_axis',(0.,0.707106781186558,0.707106781186537)) ;
#87030=DIRECTION('ref_axis',(0.,-0.707106781186537,0.707106781186558)) ;
#87031=DIRECTION('center_axis',(0.,0.,-1.)) ;
#87032=DIRECTION('ref_axis',(-1.,0.,0.)) ;
#87033=DIRECTION('center_axis',(2.16840434497101E-16,-1.,1.30104260698261E-16)) ;
#87034=DIRECTION('ref_axis',(1.,2.16840434497101E-16,-1.09476442525376E-47)) ;
#87035=DIRECTION('center_axis',(-2.85488809725132E-13,-0.707106781186525,
-0.70710678118657)) ;
#87036=DIRECTION('ref_axis',(7.82804041694617E-11,0.70710678118657,-0.707106781186525)) ;
#87037=DIRECTION('center_axis',(-5.42101086242752E-16,1.,0.)) ;
#87038=DIRECTION('ref_axis',(1.,5.42101086242752E-16,0.)) ;
#87039=DIRECTION('',(-2.16840434497101E-16,1.,-1.30104260698261E-16)) ;
#87040=DIRECTION('center_axis',(0.,1.,0.)) ;
#87041=DIRECTION('ref_axis',(0.,0.,1.)) ;
#87042=DIRECTION('',(2.16840434497101E-16,-1.,1.30104260698261E-16)) ;
#87043=DIRECTION('',(2.16840434497101E-16,-1.,1.30104260698261E-16)) ;
#87044=DIRECTION('center_axis',(1.,0.,0.)) ;
#87045=DIRECTION('ref_axis',(0.,0.,-1.)) ;
#87046=DIRECTION('center_axis',(1.,0.,0.)) ;
#87047=DIRECTION('ref_axis',(0.,0.,-1.)) ;
#87048=DIRECTION('center_axis',(0.,-1.,-1.22464679914735E-16)) ;
#87049=DIRECTION('ref_axis',(0.,-1.22464679914735E-16,1.)) ;
#87050=DIRECTION('center_axis',(-1.,0.,0.)) ;
#87051=DIRECTION('ref_axis',(0.,0.,-1.)) ;
#87052=DIRECTION('center_axis',(-1.,0.,0.)) ;
#87053=DIRECTION('ref_axis',(0.,0.,-1.)) ;
#87054=DIRECTION('center_axis',(-1.,0.,0.)) ;
#87055=DIRECTION('ref_axis',(0.,0.,1.)) ;
#87056=DIRECTION('center_axis',(-1.,0.,0.)) ;
#87057=DIRECTION('ref_axis',(0.,0.,1.)) ;
#87058=DIRECTION('center_axis',(0.,1.,-1.22464679914735E-16)) ;
#87059=DIRECTION('ref_axis',(0.,-1.22464679914735E-16,-1.)) ;
#87060=DIRECTION('center_axis',(1.,0.,0.)) ;
#87061=DIRECTION('ref_axis',(0.,0.,1.)) ;
#87062=DIRECTION('center_axis',(0.,1.,0.)) ;
#87063=DIRECTION('ref_axis',(0.,0.,1.)) ;
#87064=DIRECTION('center_axis',(-1.,0.,0.)) ;
#87065=DIRECTION('ref_axis',(0.,0.,-1.)) ;
#87066=DIRECTION('center_axis',(0.,0.707106781186558,0.707106781186537)) ;
#87067=DIRECTION('ref_axis',(0.,-0.707106781186537,0.707106781186558)) ;
#87068=DIRECTION('center_axis',(0.,0.,-1.)) ;
#87069=DIRECTION('ref_axis',(-1.,0.,0.)) ;
#87070=DIRECTION('center_axis',(2.16840434497101E-16,-1.,1.30104260698261E-16)) ;
#87071=DIRECTION('ref_axis',(1.,2.16840434497101E-16,-1.09476442525376E-47)) ;
#87072=DIRECTION('center_axis',(-4.61475062295438E-13,-0.707106781186512,
-0.707106781186583)) ;
#87073=DIRECTION('ref_axis',(8.02352901261504E-11,0.707106781186583,-0.707106781186512)) ;
#87074=DIRECTION('center_axis',(-5.42101086242752E-16,1.,0.)) ;
#87075=DIRECTION('ref_axis',(1.,5.42101086242752E-16,0.)) ;
#87076=DIRECTION('',(-2.16840434497101E-16,1.,-1.30104260698261E-16)) ;
#87077=DIRECTION('center_axis',(0.,1.,0.)) ;
#87078=DIRECTION('ref_axis',(0.,0.,1.)) ;
#87079=DIRECTION('',(2.16840434497101E-16,-1.,1.30104260698261E-16)) ;
#87080=DIRECTION('',(2.16840434497101E-16,-1.,1.30104260698261E-16)) ;
#87081=DIRECTION('center_axis',(1.,0.,0.)) ;
#87082=DIRECTION('ref_axis',(0.,0.,-1.)) ;
#87083=DIRECTION('center_axis',(1.,0.,0.)) ;
#87084=DIRECTION('ref_axis',(0.,0.,-1.)) ;
#87085=DIRECTION('center_axis',(0.,-1.,-1.22464679914735E-16)) ;
#87086=DIRECTION('ref_axis',(0.,-1.22464679914735E-16,1.)) ;
#87087=DIRECTION('center_axis',(-1.,0.,0.)) ;
#87088=DIRECTION('ref_axis',(0.,0.,-1.)) ;
#87089=DIRECTION('center_axis',(-1.,0.,0.)) ;
#87090=DIRECTION('ref_axis',(0.,0.,-1.)) ;
#87091=DIRECTION('center_axis',(-1.,0.,0.)) ;
#87092=DIRECTION('ref_axis',(0.,0.,1.)) ;
#87093=DIRECTION('center_axis',(-1.,0.,0.)) ;
#87094=DIRECTION('ref_axis',(0.,0.,1.)) ;
#87095=DIRECTION('center_axis',(0.,1.,-1.22464679914735E-16)) ;
#87096=DIRECTION('ref_axis',(0.,-1.22464679914735E-16,-1.)) ;
#87097=DIRECTION('center_axis',(1.,0.,0.)) ;
#87098=DIRECTION('ref_axis',(0.,0.,1.)) ;
#87099=DIRECTION('center_axis',(0.,1.,0.)) ;
#87100=DIRECTION('ref_axis',(0.,0.,1.)) ;
#87101=DIRECTION('center_axis',(-1.,0.,0.)) ;
#87102=DIRECTION('ref_axis',(0.,0.,-1.)) ;
#87103=DIRECTION('center_axis',(0.,0.707106781186558,0.707106781186537)) ;
#87104=DIRECTION('ref_axis',(0.,-0.707106781186537,0.707106781186558)) ;
#87105=DIRECTION('center_axis',(0.,0.,-1.)) ;
#87106=DIRECTION('ref_axis',(-1.,0.,0.)) ;
#87107=DIRECTION('center_axis',(2.16840434497101E-16,-1.,1.30104260698261E-16)) ;
#87108=DIRECTION('ref_axis',(1.,2.16840434497101E-16,-1.09476442525376E-47)) ;
#87109=DIRECTION('center_axis',(-5.4946818858058E-13,-0.707106781186505,
-0.70710678118659)) ;
#87110=DIRECTION('ref_axis',(1.03835885983909E-10,0.70710678118659,-0.707106781186505)) ;
#87111=DIRECTION('center_axis',(-5.42101086242752E-16,1.,0.)) ;
#87112=DIRECTION('ref_axis',(1.,5.42101086242752E-16,0.)) ;
#87113=DIRECTION('',(-2.16840434497101E-16,1.,-1.30104260698261E-16)) ;
#87114=DIRECTION('center_axis',(0.,1.,0.)) ;
#87115=DIRECTION('ref_axis',(0.,0.,1.)) ;
#87116=DIRECTION('',(2.16840434497101E-16,-1.,1.30104260698261E-16)) ;
#87117=DIRECTION('',(2.16840434497101E-16,-1.,1.30104260698261E-16)) ;
#87118=DIRECTION('center_axis',(1.,0.,0.)) ;
#87119=DIRECTION('ref_axis',(0.,0.,-1.)) ;
#87120=DIRECTION('center_axis',(1.,0.,0.)) ;
#87121=DIRECTION('ref_axis',(0.,0.,-1.)) ;
#87122=DIRECTION('center_axis',(0.,-1.,-1.22464679914735E-16)) ;
#87123=DIRECTION('ref_axis',(0.,-1.22464679914735E-16,1.)) ;
#87124=DIRECTION('center_axis',(-1.,0.,0.)) ;
#87125=DIRECTION('ref_axis',(0.,0.,-1.)) ;
#87126=DIRECTION('center_axis',(-1.,0.,0.)) ;
#87127=DIRECTION('ref_axis',(0.,0.,-1.)) ;
#87128=DIRECTION('center_axis',(-1.,0.,0.)) ;
#87129=DIRECTION('ref_axis',(0.,0.,1.)) ;
#87130=DIRECTION('center_axis',(-1.,0.,0.)) ;
#87131=DIRECTION('ref_axis',(0.,0.,1.)) ;
#87132=DIRECTION('center_axis',(0.,1.,-1.22464679914735E-16)) ;
#87133=DIRECTION('ref_axis',(0.,-1.22464679914735E-16,-1.)) ;
#87134=DIRECTION('center_axis',(1.,0.,0.)) ;
#87135=DIRECTION('ref_axis',(0.,0.,1.)) ;
#87136=DIRECTION('center_axis',(0.,1.,0.)) ;
#87137=DIRECTION('ref_axis',(0.,0.,1.)) ;
#87138=DIRECTION('center_axis',(-1.,0.,0.)) ;
#87139=DIRECTION('ref_axis',(0.,0.,-1.)) ;
#87140=DIRECTION('center_axis',(0.,0.707106781186558,0.707106781186537)) ;
#87141=DIRECTION('ref_axis',(0.,-0.707106781186537,0.707106781186558)) ;
#87142=DIRECTION('center_axis',(0.,0.,-1.)) ;
#87143=DIRECTION('ref_axis',(-1.,0.,0.)) ;
#87144=DIRECTION('center_axis',(2.16840434497101E-16,-1.,1.30104260698261E-16)) ;
#87145=DIRECTION('ref_axis',(1.,2.16840434497101E-16,-1.09476442525376E-47)) ;
#87146=DIRECTION('center_axis',(-4.61475062295467E-13,-0.707106781186512,
-0.707106781186583)) ;
#87147=DIRECTION('ref_axis',(8.2666922773353E-11,0.707106781186583,-0.707106781186512)) ;
#87148=DIRECTION('center_axis',(-5.42101086242752E-16,1.,0.)) ;
#87149=DIRECTION('ref_axis',(1.,5.42101086242752E-16,0.)) ;
#87150=DIRECTION('',(-2.16840434497101E-16,1.,-1.30104260698261E-16)) ;
#87151=DIRECTION('center_axis',(0.,1.,0.)) ;
#87152=DIRECTION('ref_axis',(0.,0.,1.)) ;
#87153=DIRECTION('',(2.16840434497101E-16,-1.,1.30104260698261E-16)) ;
#87154=DIRECTION('',(2.16840434497101E-16,-1.,1.30104260698261E-16)) ;
#87155=DIRECTION('center_axis',(1.,0.,0.)) ;
#87156=DIRECTION('ref_axis',(0.,0.,-1.)) ;
#87157=DIRECTION('center_axis',(1.,0.,0.)) ;
#87158=DIRECTION('ref_axis',(0.,0.,-1.)) ;
#87159=DIRECTION('center_axis',(0.,-1.,-1.22464679914735E-16)) ;
#87160=DIRECTION('ref_axis',(0.,-1.22464679914735E-16,1.)) ;
#87161=DIRECTION('center_axis',(-1.,0.,0.)) ;
#87162=DIRECTION('ref_axis',(0.,0.,-1.)) ;
#87163=DIRECTION('center_axis',(-1.,0.,0.)) ;
#87164=DIRECTION('ref_axis',(0.,0.,-1.)) ;
#87165=DIRECTION('center_axis',(-1.,0.,0.)) ;
#87166=DIRECTION('ref_axis',(0.,0.,1.)) ;
#87167=DIRECTION('center_axis',(-1.,0.,0.)) ;
#87168=DIRECTION('ref_axis',(0.,0.,1.)) ;
#87169=DIRECTION('center_axis',(0.,1.,-1.22464679914735E-16)) ;
#87170=DIRECTION('ref_axis',(0.,-1.22464679914735E-16,-1.)) ;
#87171=DIRECTION('center_axis',(1.,0.,0.)) ;
#87172=DIRECTION('ref_axis',(0.,0.,1.)) ;
#87173=DIRECTION('center_axis',(0.,1.,0.)) ;
#87174=DIRECTION('ref_axis',(0.,0.,1.)) ;
#87175=DIRECTION('center_axis',(-1.,0.,0.)) ;
#87176=DIRECTION('ref_axis',(0.,0.,-1.)) ;
#87177=DIRECTION('center_axis',(0.,0.707106781186545,0.70710678118655)) ;
#87178=DIRECTION('ref_axis',(0.,-0.70710678118655,0.707106781186545)) ;
#87179=DIRECTION('center_axis',(0.,0.,-1.)) ;
#87180=DIRECTION('ref_axis',(-1.,0.,0.)) ;
#87181=DIRECTION('center_axis',(2.16840434497101E-16,-1.,1.30104260698261E-16)) ;
#87182=DIRECTION('ref_axis',(1.,2.16840434497101E-16,-1.09476442525376E-47)) ;
#87183=DIRECTION('center_axis',(-6.37461314865721E-13,-0.707106781186499,
-0.707106781186596)) ;
#87184=DIRECTION('ref_axis',(-7.23831307879934E-11,0.707106781186596,-0.707106781186499)) ;
#87185=DIRECTION('center_axis',(-5.42101086242752E-16,1.,0.)) ;
#87186=DIRECTION('ref_axis',(1.,5.42101086242752E-16,0.)) ;
#87187=DIRECTION('',(-2.16840434497101E-16,1.,-1.30104260698261E-16)) ;
#87188=DIRECTION('center_axis',(0.,1.,0.)) ;
#87189=DIRECTION('ref_axis',(0.,0.,1.)) ;
#87190=DIRECTION('',(2.16840434497101E-16,-1.,1.30104260698261E-16)) ;
#87191=DIRECTION('',(2.16840434497101E-16,-1.,1.30104260698261E-16)) ;
#87192=DIRECTION('center_axis',(1.,0.,0.)) ;
#87193=DIRECTION('ref_axis',(0.,0.,-1.)) ;
#87194=DIRECTION('center_axis',(1.,0.,0.)) ;
#87195=DIRECTION('ref_axis',(0.,0.,-1.)) ;
#87196=DIRECTION('center_axis',(0.,-1.,-1.22464679914735E-16)) ;
#87197=DIRECTION('ref_axis',(0.,-1.22464679914735E-16,1.)) ;
#87198=DIRECTION('center_axis',(-1.,0.,0.)) ;
#87199=DIRECTION('ref_axis',(0.,0.,-1.)) ;
#87200=DIRECTION('center_axis',(-1.,0.,0.)) ;
#87201=DIRECTION('ref_axis',(0.,0.,-1.)) ;
#87202=DIRECTION('center_axis',(-1.,0.,0.)) ;
#87203=DIRECTION('ref_axis',(0.,0.,1.)) ;
#87204=DIRECTION('center_axis',(-1.,0.,0.)) ;
#87205=DIRECTION('ref_axis',(0.,0.,1.)) ;
#87206=DIRECTION('center_axis',(0.,1.,-1.22464679914735E-16)) ;
#87207=DIRECTION('ref_axis',(0.,-1.22464679914735E-16,-1.)) ;
#87208=DIRECTION('center_axis',(1.,0.,0.)) ;
#87209=DIRECTION('ref_axis',(0.,0.,1.)) ;
#87210=DIRECTION('center_axis',(0.,1.,0.)) ;
#87211=DIRECTION('ref_axis',(0.,0.,1.)) ;
#87212=DIRECTION('center_axis',(-1.,0.,0.)) ;
#87213=DIRECTION('ref_axis',(0.,0.,-1.)) ;
#87214=DIRECTION('center_axis',(0.,0.707106781186545,0.70710678118655)) ;
#87215=DIRECTION('ref_axis',(0.,-0.70710678118655,0.707106781186545)) ;
#87216=DIRECTION('center_axis',(0.,0.,-1.)) ;
#87217=DIRECTION('ref_axis',(-1.,0.,0.)) ;
#87218=DIRECTION('center_axis',(2.16840434497101E-16,-1.,1.30104260698261E-16)) ;
#87219=DIRECTION('ref_axis',(1.,2.16840434497101E-16,-1.09476442525376E-47)) ;
#87220=DIRECTION('center_axis',(-2.04144052981523E-12,-0.707106781186384,
-0.707106781186711)) ;
#87221=DIRECTION('ref_axis',(3.79286005912221E-12,0.707106781186711,-0.707106781186384)) ;
#87222=DIRECTION('center_axis',(-5.42101086242752E-16,1.,0.)) ;
#87223=DIRECTION('ref_axis',(1.,5.42101086242752E-16,0.)) ;
#87224=DIRECTION('',(-2.16840434497101E-16,1.,-1.30104260698261E-16)) ;
#87225=DIRECTION('center_axis',(0.,1.,0.)) ;
#87226=DIRECTION('ref_axis',(0.,0.,1.)) ;
#87227=DIRECTION('',(2.16840434497101E-16,-1.,1.30104260698261E-16)) ;
#87228=DIRECTION('',(2.16840434497101E-16,-1.,1.30104260698261E-16)) ;
#87229=DIRECTION('center_axis',(1.,0.,0.)) ;
#87230=DIRECTION('ref_axis',(0.,0.,-1.)) ;
#87231=DIRECTION('center_axis',(1.,0.,0.)) ;
#87232=DIRECTION('ref_axis',(0.,0.,-1.)) ;
#87233=DIRECTION('center_axis',(0.,-1.,-1.22464679914735E-16)) ;
#87234=DIRECTION('ref_axis',(0.,-1.22464679914735E-16,1.)) ;
#87235=DIRECTION('center_axis',(-1.,0.,0.)) ;
#87236=DIRECTION('ref_axis',(0.,0.,-1.)) ;
#87237=DIRECTION('center_axis',(-1.,0.,0.)) ;
#87238=DIRECTION('ref_axis',(0.,0.,-1.)) ;
#87239=DIRECTION('center_axis',(-1.,0.,0.)) ;
#87240=DIRECTION('ref_axis',(0.,0.,1.)) ;
#87241=DIRECTION('center_axis',(-1.,0.,0.)) ;
#87242=DIRECTION('ref_axis',(0.,0.,1.)) ;
#87243=DIRECTION('center_axis',(0.,1.,-1.22464679914735E-16)) ;
#87244=DIRECTION('ref_axis',(0.,-1.22464679914735E-16,-1.)) ;
#87245=DIRECTION('center_axis',(1.,0.,0.)) ;
#87246=DIRECTION('ref_axis',(0.,0.,1.)) ;
#87247=DIRECTION('center_axis',(0.,1.,0.)) ;
#87248=DIRECTION('ref_axis',(0.,0.,1.)) ;
#87249=DIRECTION('center_axis',(-1.,0.,0.)) ;
#87250=DIRECTION('ref_axis',(0.,0.,-1.)) ;
#87251=DIRECTION('center_axis',(0.,0.707106781186545,0.70710678118655)) ;
#87252=DIRECTION('ref_axis',(0.,-0.70710678118655,0.707106781186545)) ;
#87253=DIRECTION('center_axis',(0.,0.,-1.)) ;
#87254=DIRECTION('ref_axis',(-1.,0.,0.)) ;
#87255=DIRECTION('center_axis',(2.16840434497101E-16,-1.,1.30104260698261E-16)) ;
#87256=DIRECTION('ref_axis',(1.,2.16840434497101E-16,-1.09476442525376E-47)) ;
#87257=DIRECTION('center_axis',(-1.65035996854789E-12,-0.707106781186426,
-0.707106781186669)) ;
#87258=DIRECTION('ref_axis',(-9.42995735618098E-12,0.707106781186669,-0.707106781186426)) ;
#87259=DIRECTION('center_axis',(-5.42101086242752E-16,1.,0.)) ;
#87260=DIRECTION('ref_axis',(1.,5.42101086242752E-16,0.)) ;
#87261=DIRECTION('',(-2.16840434497101E-16,1.,-1.30104260698261E-16)) ;
#87262=DIRECTION('center_axis',(0.,1.,0.)) ;
#87263=DIRECTION('ref_axis',(0.,0.,1.)) ;
#87264=DIRECTION('',(2.16840434497101E-16,-1.,1.30104260698261E-16)) ;
#87265=DIRECTION('',(2.16840434497101E-16,-1.,1.30104260698261E-16)) ;
#87266=DIRECTION('center_axis',(1.,0.,0.)) ;
#87267=DIRECTION('ref_axis',(0.,0.,-1.)) ;
#87268=DIRECTION('center_axis',(1.,0.,0.)) ;
#87269=DIRECTION('ref_axis',(0.,0.,-1.)) ;
#87270=DIRECTION('center_axis',(0.,-1.,-1.22464679914735E-16)) ;
#87271=DIRECTION('ref_axis',(0.,-1.22464679914735E-16,1.)) ;
#87272=DIRECTION('center_axis',(-1.,0.,0.)) ;
#87273=DIRECTION('ref_axis',(0.,0.,-1.)) ;
#87274=DIRECTION('center_axis',(-1.,0.,0.)) ;
#87275=DIRECTION('ref_axis',(0.,0.,-1.)) ;
#87276=DIRECTION('center_axis',(1.,0.,0.)) ;
#87277=DIRECTION('ref_axis',(0.,0.,-1.)) ;
#87278=DIRECTION('center_axis',(-1.,0.,0.)) ;
#87279=DIRECTION('ref_axis',(0.,0.,-1.)) ;
#87280=DIRECTION('center_axis',(0.,0.,1.)) ;
#87281=DIRECTION('ref_axis',(1.,0.,0.)) ;
#87282=DIRECTION('center_axis',(1.,0.,0.)) ;
#87283=DIRECTION('ref_axis',(0.,0.,-1.)) ;
#87284=DIRECTION('center_axis',(0.,0.707106781186548,-0.707106781186548)) ;
#87285=DIRECTION('ref_axis',(0.,0.707106781186548,0.707106781186548)) ;
#87286=DIRECTION('center_axis',(1.,0.,0.)) ;
#87287=DIRECTION('ref_axis',(0.,0.,-1.)) ;
#87288=DIRECTION('center_axis',(-1.,0.,0.)) ;
#87289=DIRECTION('ref_axis',(0.,0.,-1.)) ;
#87290=DIRECTION('center_axis',(0.,0.,1.)) ;
#87291=DIRECTION('ref_axis',(1.,0.,0.)) ;
#87292=DIRECTION('center_axis',(1.,0.,0.)) ;
#87293=DIRECTION('ref_axis',(0.,0.,-1.)) ;
#87294=DIRECTION('center_axis',(0.,0.707106781186548,-0.707106781186548)) ;
#87295=DIRECTION('ref_axis',(0.,0.707106781186548,0.707106781186548)) ;
#87296=DIRECTION('center_axis',(1.,0.,0.)) ;
#87297=DIRECTION('ref_axis',(0.,0.,-1.)) ;
#87298=DIRECTION('center_axis',(-1.,0.,0.)) ;
#87299=DIRECTION('ref_axis',(0.,0.,-1.)) ;
#87300=DIRECTION('center_axis',(0.,0.,1.)) ;
#87301=DIRECTION('ref_axis',(1.,0.,0.)) ;
#87302=DIRECTION('center_axis',(1.,0.,0.)) ;
#87303=DIRECTION('ref_axis',(0.,0.,-1.)) ;
#87304=DIRECTION('center_axis',(0.,0.707106781186548,-0.707106781186548)) ;
#87305=DIRECTION('ref_axis',(0.,0.707106781186548,0.707106781186548)) ;
#87306=DIRECTION('center_axis',(1.,0.,0.)) ;
#87307=DIRECTION('ref_axis',(0.,0.,-1.)) ;
#87308=DIRECTION('center_axis',(-1.,0.,0.)) ;
#87309=DIRECTION('ref_axis',(0.,0.,-1.)) ;
#87310=DIRECTION('center_axis',(0.,0.,1.)) ;
#87311=DIRECTION('ref_axis',(1.,0.,0.)) ;
#87312=DIRECTION('center_axis',(1.,0.,0.)) ;
#87313=DIRECTION('ref_axis',(0.,0.,-1.)) ;
#87314=DIRECTION('center_axis',(0.,0.707106781186539,-0.707106781186556)) ;
#87315=DIRECTION('ref_axis',(0.,0.707106781186556,0.707106781186539)) ;
#87316=DIRECTION('center_axis',(1.,0.,0.)) ;
#87317=DIRECTION('ref_axis',(0.,0.,-1.)) ;
#87318=DIRECTION('center_axis',(-1.,0.,0.)) ;
#87319=DIRECTION('ref_axis',(0.,0.,-1.)) ;
#87320=DIRECTION('center_axis',(0.,0.,1.)) ;
#87321=DIRECTION('ref_axis',(1.,0.,0.)) ;
#87322=DIRECTION('center_axis',(1.,0.,0.)) ;
#87323=DIRECTION('ref_axis',(0.,0.,-1.)) ;
#87324=DIRECTION('center_axis',(0.,0.707106781186539,-0.707106781186556)) ;
#87325=DIRECTION('ref_axis',(0.,0.707106781186556,0.707106781186539)) ;
#87326=DIRECTION('center_axis',(1.,0.,0.)) ;
#87327=DIRECTION('ref_axis',(0.,0.,-1.)) ;
#87328=DIRECTION('center_axis',(-1.,0.,0.)) ;
#87329=DIRECTION('ref_axis',(0.,0.,-1.)) ;
#87330=DIRECTION('center_axis',(0.,0.,1.)) ;
#87331=DIRECTION('ref_axis',(1.,0.,0.)) ;
#87332=DIRECTION('center_axis',(1.,0.,0.)) ;
#87333=DIRECTION('ref_axis',(0.,0.,-1.)) ;
#87334=DIRECTION('center_axis',(0.,0.707106781186539,-0.707106781186556)) ;
#87335=DIRECTION('ref_axis',(0.,0.707106781186556,0.707106781186539)) ;
#87336=DIRECTION('center_axis',(1.,0.,0.)) ;
#87337=DIRECTION('ref_axis',(0.,0.,-1.)) ;
#87338=DIRECTION('center_axis',(-1.,0.,0.)) ;
#87339=DIRECTION('ref_axis',(0.,0.,-1.)) ;
#87340=DIRECTION('center_axis',(0.,0.,1.)) ;
#87341=DIRECTION('ref_axis',(1.,0.,0.)) ;
#87342=DIRECTION('center_axis',(1.,0.,0.)) ;
#87343=DIRECTION('ref_axis',(0.,0.,-1.)) ;
#87344=DIRECTION('center_axis',(0.,0.707106781186539,-0.707106781186556)) ;
#87345=DIRECTION('ref_axis',(0.,0.707106781186556,0.707106781186539)) ;
#87346=DIRECTION('center_axis',(1.,0.,0.)) ;
#87347=DIRECTION('ref_axis',(0.,0.,-1.)) ;
#87348=DIRECTION('center_axis',(-1.,0.,0.)) ;
#87349=DIRECTION('ref_axis',(0.,0.,-1.)) ;
#87350=DIRECTION('center_axis',(0.,0.,1.)) ;
#87351=DIRECTION('ref_axis',(1.,0.,0.)) ;
#87352=DIRECTION('center_axis',(1.,0.,0.)) ;
#87353=DIRECTION('ref_axis',(0.,0.,-1.)) ;
#87354=DIRECTION('center_axis',(-6.13317366673346E-15,0.707106781186539,
-0.707106781186556)) ;
#87355=DIRECTION('ref_axis',(3.80912633391397E-29,0.707106781186556,0.707106781186539)) ;
#87356=DIRECTION('center_axis',(1.,0.,0.)) ;
#87357=DIRECTION('ref_axis',(0.,0.,-1.)) ;
#87358=DIRECTION('center_axis',(-1.,0.,0.)) ;
#87359=DIRECTION('ref_axis',(0.,0.,-1.)) ;
#87360=DIRECTION('center_axis',(0.,0.,1.)) ;
#87361=DIRECTION('ref_axis',(1.,0.,0.)) ;
#87362=DIRECTION('center_axis',(1.,0.,0.)) ;
#87363=DIRECTION('ref_axis',(0.,0.,-1.)) ;
#87364=DIRECTION('center_axis',(-6.13317366673346E-15,0.707106781186539,
-0.707106781186556)) ;
#87365=DIRECTION('ref_axis',(3.80912633391397E-29,0.707106781186556,0.707106781186539)) ;
#87366=DIRECTION('center_axis',(-1.,0.,0.)) ;
#87367=DIRECTION('ref_axis',(0.,0.,1.)) ;
#87368=DIRECTION('center_axis',(-1.,0.,0.)) ;
#87369=DIRECTION('ref_axis',(0.,0.,1.)) ;
#87370=DIRECTION('center_axis',(0.,1.,-1.22464679914735E-16)) ;
#87371=DIRECTION('ref_axis',(0.,-1.22464679914735E-16,-1.)) ;
#87372=DIRECTION('center_axis',(1.,0.,0.)) ;
#87373=DIRECTION('ref_axis',(0.,0.,1.)) ;
#87374=DIRECTION('center_axis',(0.,1.,0.)) ;
#87375=DIRECTION('ref_axis',(0.,0.,1.)) ;
#87376=DIRECTION('center_axis',(-1.,0.,0.)) ;
#87377=DIRECTION('ref_axis',(0.,0.,-1.)) ;
#87378=DIRECTION('center_axis',(0.,0.70710678118655,0.707106781186545)) ;
#87379=DIRECTION('ref_axis',(0.,-0.707106781186545,0.70710678118655)) ;
#87380=DIRECTION('center_axis',(0.,0.,-1.)) ;
#87381=DIRECTION('ref_axis',(-1.,0.,0.)) ;
#87382=DIRECTION('center_axis',(2.16840434497101E-16,-1.,1.30104260698261E-16)) ;
#87383=DIRECTION('ref_axis',(1.,2.16840434497101E-16,-1.09476442525376E-47)) ;
#87384=DIRECTION('center_axis',(6.64836954154425E-14,-0.707106781186552,
-0.707106781186543)) ;
#87385=DIRECTION('ref_axis',(-1.70648371771735E-11,0.707106781186543,-0.707106781186552)) ;
#87386=DIRECTION('center_axis',(-5.42101086242752E-16,1.,0.)) ;
#87387=DIRECTION('ref_axis',(1.,5.42101086242752E-16,0.)) ;
#87388=DIRECTION('',(-2.16840434497101E-16,1.,-1.30104260698261E-16)) ;
#87389=DIRECTION('center_axis',(0.,1.,0.)) ;
#87390=DIRECTION('ref_axis',(0.,0.,1.)) ;
#87391=DIRECTION('',(2.16840434497101E-16,-1.,1.30104260698261E-16)) ;
#87392=DIRECTION('',(2.16840434497101E-16,-1.,1.30104260698261E-16)) ;
#87393=DIRECTION('center_axis',(-1.,0.,0.)) ;
#87394=DIRECTION('ref_axis',(0.,0.,1.)) ;
#87395=DIRECTION('',(1.,0.,0.)) ;
#87396=DIRECTION('center_axis',(-1.,0.,0.)) ;
#87397=DIRECTION('ref_axis',(0.,0.,1.)) ;
#87398=DIRECTION('',(1.,0.,0.)) ;
#87399=DIRECTION('center_axis',(-1.,0.,0.)) ;
#87400=DIRECTION('ref_axis',(0.,0.,1.)) ;
#87401=DIRECTION('',(1.,0.,0.)) ;
#87402=DIRECTION('center_axis',(-1.,0.,0.)) ;
#87403=DIRECTION('ref_axis',(0.,0.,1.)) ;
#87404=DIRECTION('',(1.,0.,0.)) ;
#87405=DIRECTION('center_axis',(-1.,0.,0.)) ;
#87406=DIRECTION('ref_axis',(0.,0.,1.)) ;
#87407=DIRECTION('',(1.,0.,0.)) ;
#87408=DIRECTION('center_axis',(-1.,0.,0.)) ;
#87409=DIRECTION('ref_axis',(0.,0.,1.)) ;
#87410=DIRECTION('',(1.,0.,0.)) ;
#87411=DIRECTION('center_axis',(-1.,0.,0.)) ;
#87412=DIRECTION('ref_axis',(0.,0.,1.)) ;
#87413=DIRECTION('',(1.,0.,0.)) ;
#87414=DIRECTION('center_axis',(-1.,0.,0.)) ;
#87415=DIRECTION('ref_axis',(0.,0.,1.)) ;
#87416=DIRECTION('',(1.,0.,0.)) ;
#87417=DIRECTION('center_axis',(-1.,0.,0.)) ;
#87418=DIRECTION('ref_axis',(0.,0.,1.)) ;
#87419=DIRECTION('',(1.,0.,0.)) ;
#87420=DIRECTION('center_axis',(1.,0.,0.)) ;
#87421=DIRECTION('ref_axis',(0.,0.,-1.)) ;
#87422=DIRECTION('center_axis',(-1.,0.,0.)) ;
#87423=DIRECTION('ref_axis',(0.,0.,-1.)) ;
#87424=DIRECTION('',(1.,0.,0.)) ;
#87425=DIRECTION('',(1.,0.,0.)) ;
#87426=DIRECTION('center_axis',(1.,0.,0.)) ;
#87427=DIRECTION('ref_axis',(0.,0.,-1.)) ;
#87428=DIRECTION('center_axis',(-1.,0.,0.)) ;
#87429=DIRECTION('ref_axis',(0.,0.,-1.)) ;
#87430=DIRECTION('',(1.,0.,0.)) ;
#87431=DIRECTION('',(1.,0.,0.)) ;
#87432=DIRECTION('center_axis',(1.,0.,0.)) ;
#87433=DIRECTION('ref_axis',(0.,0.,-1.)) ;
#87434=DIRECTION('center_axis',(-1.,0.,0.)) ;
#87435=DIRECTION('ref_axis',(0.,0.,-1.)) ;
#87436=DIRECTION('',(1.,0.,0.)) ;
#87437=DIRECTION('',(1.,0.,0.)) ;
#87438=DIRECTION('center_axis',(1.,0.,0.)) ;
#87439=DIRECTION('ref_axis',(0.,0.,-1.)) ;
#87440=DIRECTION('center_axis',(-1.,0.,0.)) ;
#87441=DIRECTION('ref_axis',(0.,0.,-1.)) ;
#87442=DIRECTION('',(1.,0.,0.)) ;
#87443=DIRECTION('',(1.,0.,0.)) ;
#87444=DIRECTION('center_axis',(1.,0.,0.)) ;
#87445=DIRECTION('ref_axis',(0.,0.,-1.)) ;
#87446=DIRECTION('center_axis',(-1.,0.,0.)) ;
#87447=DIRECTION('ref_axis',(0.,0.,-1.)) ;
#87448=DIRECTION('',(1.,0.,0.)) ;
#87449=DIRECTION('',(1.,0.,0.)) ;
#87450=DIRECTION('center_axis',(1.,0.,0.)) ;
#87451=DIRECTION('ref_axis',(0.,0.,-1.)) ;
#87452=DIRECTION('center_axis',(-1.,0.,0.)) ;
#87453=DIRECTION('ref_axis',(0.,0.,-1.)) ;
#87454=DIRECTION('',(1.,0.,0.)) ;
#87455=DIRECTION('',(1.,0.,0.)) ;
#87456=DIRECTION('center_axis',(1.,0.,0.)) ;
#87457=DIRECTION('ref_axis',(0.,0.,-1.)) ;
#87458=DIRECTION('center_axis',(-1.,0.,0.)) ;
#87459=DIRECTION('ref_axis',(0.,0.,-1.)) ;
#87460=DIRECTION('',(1.,0.,0.)) ;
#87461=DIRECTION('',(1.,0.,0.)) ;
#87462=DIRECTION('center_axis',(1.,0.,0.)) ;
#87463=DIRECTION('ref_axis',(0.,0.,-1.)) ;
#87464=DIRECTION('center_axis',(-1.,0.,0.)) ;
#87465=DIRECTION('ref_axis',(0.,0.,-1.)) ;
#87466=DIRECTION('',(1.,0.,0.)) ;
#87467=DIRECTION('',(1.,0.,0.)) ;
#87468=DIRECTION('center_axis',(1.,0.,0.)) ;
#87469=DIRECTION('ref_axis',(0.,0.,-1.)) ;
#87470=DIRECTION('center_axis',(-1.,0.,0.)) ;
#87471=DIRECTION('ref_axis',(0.,0.,-1.)) ;
#87472=DIRECTION('',(1.,0.,0.)) ;
#87473=DIRECTION('',(1.,0.,0.)) ;
#87474=DIRECTION('center_axis',(1.,0.,0.)) ;
#87475=DIRECTION('ref_axis',(0.,0.,-1.)) ;
#87476=DIRECTION('center_axis',(1.,0.,0.)) ;
#87477=DIRECTION('ref_axis',(0.,0.,-1.)) ;
#87478=DIRECTION('center_axis',(0.,-1.,-1.22464679914735E-16)) ;
#87479=DIRECTION('ref_axis',(0.,-1.22464679914735E-16,1.)) ;
#87480=DIRECTION('center_axis',(-1.,0.,0.)) ;
#87481=DIRECTION('ref_axis',(0.,0.,-1.)) ;
#87482=DIRECTION('center_axis',(-1.,0.,0.)) ;
#87483=DIRECTION('ref_axis',(0.,0.,-1.)) ;
#87484=DIRECTION('center_axis',(1.,0.,0.)) ;
#87485=DIRECTION('ref_axis',(0.,0.,-1.)) ;
#87486=DIRECTION('center_axis',(-1.,0.,0.)) ;
#87487=DIRECTION('ref_axis',(0.,0.,-1.)) ;
#87488=DIRECTION('center_axis',(0.,0.,1.)) ;
#87489=DIRECTION('ref_axis',(1.,0.,0.)) ;
#87490=DIRECTION('center_axis',(1.,0.,0.)) ;
#87491=DIRECTION('ref_axis',(0.,0.,-1.)) ;
#87492=DIRECTION('center_axis',(0.,0.707106781186548,-0.707106781186548)) ;
#87493=DIRECTION('ref_axis',(0.,0.707106781186548,0.707106781186548)) ;
#87494=DIRECTION('center_axis',(-1.,0.,0.)) ;
#87495=DIRECTION('ref_axis',(0.,0.,1.)) ;
#87496=DIRECTION('center_axis',(-1.,0.,0.)) ;
#87497=DIRECTION('ref_axis',(0.,0.,1.)) ;
#87498=DIRECTION('center_axis',(0.,1.,-1.22464679914735E-16)) ;
#87499=DIRECTION('ref_axis',(0.,-1.22464679914735E-16,-1.)) ;
#87500=DIRECTION('center_axis',(1.,0.,0.)) ;
#87501=DIRECTION('ref_axis',(0.,0.,1.)) ;
#87502=DIRECTION('center_axis',(0.,1.,0.)) ;
#87503=DIRECTION('ref_axis',(0.,0.,1.)) ;
#87504=DIRECTION('center_axis',(-1.,0.,0.)) ;
#87505=DIRECTION('ref_axis',(0.,0.,-1.)) ;
#87506=DIRECTION('center_axis',(0.,0.70710678118655,0.707106781186545)) ;
#87507=DIRECTION('ref_axis',(0.,-0.707106781186545,0.70710678118655)) ;
#87508=DIRECTION('center_axis',(0.,0.,-1.)) ;
#87509=DIRECTION('ref_axis',(-1.,0.,0.)) ;
#87510=DIRECTION('center_axis',(2.16840434497101E-16,-1.,1.30104260698261E-16)) ;
#87511=DIRECTION('ref_axis',(1.,2.16840434497101E-16,-1.09476442525376E-47)) ;
#87512=DIRECTION('center_axis',(-1.95540280633655E-15,-0.707106781186549,
-0.707106781186546)) ;
#87513=DIRECTION('ref_axis',(-2.18299406319968E-11,0.707106781186546,-0.707106781186549)) ;
#87514=DIRECTION('center_axis',(-5.42101086242752E-16,1.,0.)) ;
#87515=DIRECTION('ref_axis',(1.,5.42101086242752E-16,0.)) ;
#87516=DIRECTION('',(-2.16840434497101E-16,1.,-1.30104260698261E-16)) ;
#87517=DIRECTION('center_axis',(0.,1.,0.)) ;
#87518=DIRECTION('ref_axis',(0.,0.,1.)) ;
#87519=DIRECTION('',(2.16840434497101E-16,-1.,1.30104260698261E-16)) ;
#87520=DIRECTION('',(2.16840434497101E-16,-1.,1.30104260698261E-16)) ;
#87521=DIRECTION('center_axis',(-1.,0.,0.)) ;
#87522=DIRECTION('ref_axis',(0.,0.,1.)) ;
#87523=DIRECTION('',(1.,0.,0.)) ;
#87524=DIRECTION('center_axis',(1.,0.,0.)) ;
#87525=DIRECTION('ref_axis',(0.,0.,-1.)) ;
#87526=DIRECTION('center_axis',(-1.,0.,0.)) ;
#87527=DIRECTION('ref_axis',(0.,0.,-1.)) ;
#87528=DIRECTION('',(1.,0.,0.)) ;
#87529=DIRECTION('',(1.,0.,0.)) ;
#87530=DIRECTION('center_axis',(-1.,-2.16840434497101E-16,0.)) ;
#87531=DIRECTION('ref_axis',(2.16840434497101E-16,-1.,0.)) ;
#87532=DIRECTION('',(-2.16840434497101E-16,1.,1.30104260698261E-16)) ;
#87533=DIRECTION('center_axis',(1.,2.16840434497101E-16,0.)) ;
#87534=DIRECTION('ref_axis',(2.16840434497101E-16,-1.,0.)) ;
#87535=DIRECTION('',(0.,0.,-1.)) ;
#87536=DIRECTION('center_axis',(1.,2.16840434497101E-16,0.)) ;
#87537=DIRECTION('ref_axis',(2.16840434497101E-16,-1.,0.)) ;
#87538=DIRECTION('center_axis',(-1.,-2.16840434497101E-16,0.)) ;
#87539=DIRECTION('ref_axis',(2.16840434497101E-16,-1.,0.)) ;
#87540=DIRECTION('',(0.,0.,-1.)) ;
#87541=DIRECTION('',(2.16840434497101E-16,-1.,5.10212787052002E-17)) ;
#87542=DIRECTION('',(0.,0.,1.)) ;
#87543=DIRECTION('',(-2.16840434497101E-16,1.,-1.020425574104E-16)) ;
#87544=DIRECTION('',(0.,0.,-1.)) ;
#87545=DIRECTION('center_axis',(-1.,-2.16840434497101E-16,0.)) ;
#87546=DIRECTION('ref_axis',(2.16840434497101E-16,-1.,0.)) ;
#87547=DIRECTION('center_axis',(-1.,-2.16840434497101E-16,0.)) ;
#87548=DIRECTION('ref_axis',(2.16840434497101E-16,-1.,0.)) ;
#87549=DIRECTION('',(-2.16840434497101E-16,1.,1.30104260698261E-16)) ;
#87550=DIRECTION('center_axis',(1.,2.16840434497101E-16,0.)) ;
#87551=DIRECTION('ref_axis',(2.16840434497101E-16,-1.,0.)) ;
#87552=DIRECTION('',(0.,0.,-1.)) ;
#87553=DIRECTION('center_axis',(1.,2.16840434497101E-16,0.)) ;
#87554=DIRECTION('ref_axis',(2.16840434497101E-16,-1.,0.)) ;
#87555=DIRECTION('center_axis',(-1.,-2.16840434497101E-16,0.)) ;
#87556=DIRECTION('ref_axis',(2.16840434497101E-16,-1.,0.)) ;
#87557=DIRECTION('',(0.,0.,-1.)) ;
#87558=DIRECTION('',(2.16840434497101E-16,-1.,5.10212787052002E-17)) ;
#87559=DIRECTION('',(0.,0.,1.)) ;
#87560=DIRECTION('',(-2.16840434497101E-16,1.,-1.020425574104E-16)) ;
#87561=DIRECTION('',(0.,0.,-1.)) ;
#87562=DIRECTION('center_axis',(-1.,-2.16840434497101E-16,0.)) ;
#87563=DIRECTION('ref_axis',(2.16840434497101E-16,-1.,0.)) ;
#87564=DIRECTION('center_axis',(-1.,-2.16840434497101E-16,0.)) ;
#87565=DIRECTION('ref_axis',(2.16840434497101E-16,-1.,0.)) ;
#87566=DIRECTION('',(-2.16840434497101E-16,1.,1.30104260698261E-16)) ;
#87567=DIRECTION('center_axis',(1.,2.16840434497101E-16,0.)) ;
#87568=DIRECTION('ref_axis',(2.16840434497101E-16,-1.,0.)) ;
#87569=DIRECTION('',(0.,0.,-1.)) ;
#87570=DIRECTION('center_axis',(1.,2.16840434497101E-16,0.)) ;
#87571=DIRECTION('ref_axis',(2.16840434497101E-16,-1.,0.)) ;
#87572=DIRECTION('center_axis',(-1.,-2.16840434497101E-16,0.)) ;
#87573=DIRECTION('ref_axis',(2.16840434497101E-16,-1.,0.)) ;
#87574=DIRECTION('',(0.,0.,-1.)) ;
#87575=DIRECTION('',(2.16840434497101E-16,-1.,5.10212787052002E-17)) ;
#87576=DIRECTION('',(0.,0.,1.)) ;
#87577=DIRECTION('',(-2.16840434497101E-16,1.,-1.020425574104E-16)) ;
#87578=DIRECTION('',(0.,0.,-1.)) ;
#87579=DIRECTION('center_axis',(-1.,-2.16840434497101E-16,0.)) ;
#87580=DIRECTION('ref_axis',(2.16840434497101E-16,-1.,0.)) ;
#87581=DIRECTION('center_axis',(-1.,-2.16840434497101E-16,0.)) ;
#87582=DIRECTION('ref_axis',(2.16840434497101E-16,-1.,0.)) ;
#87583=DIRECTION('',(-2.16840434497101E-16,1.,1.30104260698261E-16)) ;
#87584=DIRECTION('center_axis',(1.,2.16840434497101E-16,0.)) ;
#87585=DIRECTION('ref_axis',(2.16840434497101E-16,-1.,0.)) ;
#87586=DIRECTION('',(0.,0.,-1.)) ;
#87587=DIRECTION('center_axis',(1.,2.16840434497101E-16,0.)) ;
#87588=DIRECTION('ref_axis',(2.16840434497101E-16,-1.,0.)) ;
#87589=DIRECTION('center_axis',(-1.,-2.16840434497101E-16,0.)) ;
#87590=DIRECTION('ref_axis',(2.16840434497101E-16,-1.,0.)) ;
#87591=DIRECTION('',(0.,0.,-1.)) ;
#87592=DIRECTION('',(2.16840434497101E-16,-1.,5.10212787052002E-17)) ;
#87593=DIRECTION('',(0.,0.,1.)) ;
#87594=DIRECTION('',(-2.16840434497101E-16,1.,-1.020425574104E-16)) ;
#87595=DIRECTION('',(0.,0.,-1.)) ;
#87596=DIRECTION('center_axis',(-1.,-2.16840434497101E-16,0.)) ;
#87597=DIRECTION('ref_axis',(2.16840434497101E-16,-1.,0.)) ;
#87598=DIRECTION('center_axis',(-1.,-2.16840434497101E-16,0.)) ;
#87599=DIRECTION('ref_axis',(2.16840434497101E-16,-1.,0.)) ;
#87600=DIRECTION('',(-2.16840434497101E-16,1.,1.30104260698261E-16)) ;
#87601=DIRECTION('center_axis',(1.,2.16840434497101E-16,0.)) ;
#87602=DIRECTION('ref_axis',(2.16840434497101E-16,-1.,0.)) ;
#87603=DIRECTION('',(0.,0.,-1.)) ;
#87604=DIRECTION('center_axis',(1.,2.16840434497101E-16,0.)) ;
#87605=DIRECTION('ref_axis',(2.16840434497101E-16,-1.,0.)) ;
#87606=DIRECTION('center_axis',(-1.,-2.16840434497101E-16,0.)) ;
#87607=DIRECTION('ref_axis',(2.16840434497101E-16,-1.,0.)) ;
#87608=DIRECTION('',(0.,0.,-1.)) ;
#87609=DIRECTION('',(2.16840434497101E-16,-1.,5.10212787052002E-17)) ;
#87610=DIRECTION('',(0.,0.,1.)) ;
#87611=DIRECTION('',(-2.16840434497101E-16,1.,-1.020425574104E-16)) ;
#87612=DIRECTION('',(0.,0.,-1.)) ;
#87613=DIRECTION('center_axis',(-1.,-2.16840434497101E-16,0.)) ;
#87614=DIRECTION('ref_axis',(2.16840434497101E-16,-1.,0.)) ;
#87615=DIRECTION('center_axis',(-1.,-2.16840434497101E-16,0.)) ;
#87616=DIRECTION('ref_axis',(2.16840434497101E-16,-1.,0.)) ;
#87617=DIRECTION('',(-2.16840434497101E-16,1.,1.30104260698261E-16)) ;
#87618=DIRECTION('center_axis',(1.,2.16840434497101E-16,0.)) ;
#87619=DIRECTION('ref_axis',(2.16840434497101E-16,-1.,0.)) ;
#87620=DIRECTION('',(0.,0.,-1.)) ;
#87621=DIRECTION('center_axis',(1.,2.16840434497101E-16,0.)) ;
#87622=DIRECTION('ref_axis',(2.16840434497101E-16,-1.,0.)) ;
#87623=DIRECTION('center_axis',(-1.,-2.16840434497101E-16,0.)) ;
#87624=DIRECTION('ref_axis',(2.16840434497101E-16,-1.,0.)) ;
#87625=DIRECTION('',(0.,0.,-1.)) ;
#87626=DIRECTION('',(2.16840434497101E-16,-1.,5.10212787052002E-17)) ;
#87627=DIRECTION('',(0.,0.,1.)) ;
#87628=DIRECTION('',(-2.16840434497101E-16,1.,-1.020425574104E-16)) ;
#87629=DIRECTION('',(0.,0.,-1.)) ;
#87630=DIRECTION('center_axis',(-1.,-2.16840434497101E-16,0.)) ;
#87631=DIRECTION('ref_axis',(2.16840434497101E-16,-1.,0.)) ;
#87632=DIRECTION('center_axis',(-1.,-2.16840434497101E-16,0.)) ;
#87633=DIRECTION('ref_axis',(2.16840434497101E-16,-1.,0.)) ;
#87634=DIRECTION('',(-2.16840434497101E-16,1.,1.30104260698261E-16)) ;
#87635=DIRECTION('center_axis',(1.,2.16840434497101E-16,0.)) ;
#87636=DIRECTION('ref_axis',(2.16840434497101E-16,-1.,0.)) ;
#87637=DIRECTION('',(0.,0.,-1.)) ;
#87638=DIRECTION('center_axis',(1.,2.16840434497101E-16,0.)) ;
#87639=DIRECTION('ref_axis',(2.16840434497101E-16,-1.,0.)) ;
#87640=DIRECTION('center_axis',(-1.,-2.16840434497101E-16,0.)) ;
#87641=DIRECTION('ref_axis',(2.16840434497101E-16,-1.,0.)) ;
#87642=DIRECTION('',(0.,0.,-1.)) ;
#87643=DIRECTION('',(2.16840434497101E-16,-1.,5.10212787052002E-17)) ;
#87644=DIRECTION('',(0.,0.,1.)) ;
#87645=DIRECTION('',(-2.16840434497101E-16,1.,-1.020425574104E-16)) ;
#87646=DIRECTION('',(0.,0.,-1.)) ;
#87647=DIRECTION('center_axis',(-1.,-2.16840434497101E-16,0.)) ;
#87648=DIRECTION('ref_axis',(2.16840434497101E-16,-1.,0.)) ;
#87649=DIRECTION('center_axis',(-1.,-2.16840434497101E-16,0.)) ;
#87650=DIRECTION('ref_axis',(2.16840434497101E-16,-1.,0.)) ;
#87651=DIRECTION('',(-2.16840434497101E-16,1.,1.30104260698261E-16)) ;
#87652=DIRECTION('center_axis',(1.,2.16840434497101E-16,0.)) ;
#87653=DIRECTION('ref_axis',(2.16840434497101E-16,-1.,0.)) ;
#87654=DIRECTION('',(0.,0.,-1.)) ;
#87655=DIRECTION('center_axis',(1.,2.16840434497101E-16,0.)) ;
#87656=DIRECTION('ref_axis',(2.16840434497101E-16,-1.,0.)) ;
#87657=DIRECTION('center_axis',(-1.,-2.16840434497101E-16,0.)) ;
#87658=DIRECTION('ref_axis',(2.16840434497101E-16,-1.,0.)) ;
#87659=DIRECTION('',(0.,0.,-1.)) ;
#87660=DIRECTION('',(2.16840434497101E-16,-1.,5.10212787052002E-17)) ;
#87661=DIRECTION('',(0.,0.,1.)) ;
#87662=DIRECTION('',(-2.16840434497101E-16,1.,-1.020425574104E-16)) ;
#87663=DIRECTION('',(0.,0.,-1.)) ;
#87664=DIRECTION('center_axis',(-1.,-2.16840434497101E-16,0.)) ;
#87665=DIRECTION('ref_axis',(2.16840434497101E-16,-1.,0.)) ;
#87666=DIRECTION('center_axis',(-1.,-2.16840434497101E-16,0.)) ;
#87667=DIRECTION('ref_axis',(2.16840434497101E-16,-1.,0.)) ;
#87668=DIRECTION('',(-2.16840434497101E-16,1.,1.30104260698261E-16)) ;
#87669=DIRECTION('center_axis',(1.,2.16840434497101E-16,0.)) ;
#87670=DIRECTION('ref_axis',(2.16840434497101E-16,-1.,0.)) ;
#87671=DIRECTION('',(0.,0.,-1.)) ;
#87672=DIRECTION('center_axis',(1.,2.16840434497101E-16,0.)) ;
#87673=DIRECTION('ref_axis',(2.16840434497101E-16,-1.,0.)) ;
#87674=DIRECTION('center_axis',(-1.,-2.16840434497101E-16,0.)) ;
#87675=DIRECTION('ref_axis',(2.16840434497101E-16,-1.,0.)) ;
#87676=DIRECTION('',(0.,0.,-1.)) ;
#87677=DIRECTION('',(2.16840434497101E-16,-1.,5.10212787052002E-17)) ;
#87678=DIRECTION('',(0.,0.,1.)) ;
#87679=DIRECTION('',(-2.16840434497101E-16,1.,-1.020425574104E-16)) ;
#87680=DIRECTION('',(0.,0.,-1.)) ;
#87681=DIRECTION('center_axis',(-1.,-2.16840434497101E-16,0.)) ;
#87682=DIRECTION('ref_axis',(2.16840434497101E-16,-1.,0.)) ;
#87683=DIRECTION('center_axis',(6.27714964143733E-33,-5.10212787052002E-17,
-1.)) ;
#87684=DIRECTION('ref_axis',(0.,1.,-5.10212787052002E-17)) ;
#87685=DIRECTION('center_axis',(-6.27714964143733E-33,5.10212787052002E-17,
1.)) ;
#87686=DIRECTION('ref_axis',(3.20268201330022E-49,1.,-5.10212787052002E-17)) ;
#87687=DIRECTION('',(1.2303003375722E-16,-1.,5.10212787052002E-17)) ;
#87688=DIRECTION('',(1.,0.,6.27714964143733E-33)) ;
#87689=DIRECTION('',(-2.16840434497101E-16,1.,-5.10212787052002E-17)) ;
#87690=DIRECTION('',(-1.,-1.53063836115601E-16,1.53236300070382E-33)) ;
#87691=DIRECTION('center_axis',(-1.25542992828747E-32,1.020425574104E-16,
1.)) ;
#87692=DIRECTION('ref_axis',(0.,-1.,1.020425574104E-16)) ;
#87693=DIRECTION('center_axis',(1.25542992828747E-32,-1.020425574104E-16,
-1.)) ;
#87694=DIRECTION('ref_axis',(-1.28107280532009E-48,-1.,1.020425574104E-16)) ;
#87695=DIRECTION('',(1.,1.53063836115601E-16,-3.06472600140763E-33)) ;
#87696=DIRECTION('',(2.16840434497101E-16,-1.,1.020425574104E-16)) ;
#87697=DIRECTION('',(-1.,0.,-1.25542992828747E-32)) ;
#87698=DIRECTION('',(-1.2303003375722E-16,1.,-1.020425574104E-16)) ;
#87699=DIRECTION('center_axis',(6.27714964143733E-33,-5.10212787052002E-17,
-1.)) ;
#87700=DIRECTION('ref_axis',(0.,1.,-5.10212787052002E-17)) ;
#87701=DIRECTION('center_axis',(-6.27714964143733E-33,5.10212787052002E-17,
1.)) ;
#87702=DIRECTION('ref_axis',(3.20268201330022E-49,1.,-5.10212787052002E-17)) ;
#87703=DIRECTION('',(1.2303003375722E-16,-1.,5.10212787052002E-17)) ;
#87704=DIRECTION('',(1.,0.,6.27714964143733E-33)) ;
#87705=DIRECTION('',(-2.16840434497101E-16,1.,-5.10212787052002E-17)) ;
#87706=DIRECTION('',(-1.,-1.53063836115601E-16,1.53236300070382E-33)) ;
#87707=DIRECTION('center_axis',(-1.25542992828747E-32,1.020425574104E-16,
1.)) ;
#87708=DIRECTION('ref_axis',(0.,-1.,1.020425574104E-16)) ;
#87709=DIRECTION('center_axis',(1.25542992828747E-32,-1.020425574104E-16,
-1.)) ;
#87710=DIRECTION('ref_axis',(-1.28107280532009E-48,-1.,1.020425574104E-16)) ;
#87711=DIRECTION('',(1.,1.53063836115601E-16,-3.06472600140763E-33)) ;
#87712=DIRECTION('',(2.16840434497101E-16,-1.,1.020425574104E-16)) ;
#87713=DIRECTION('',(-1.,0.,-1.25542992828747E-32)) ;
#87714=DIRECTION('',(-1.2303003375722E-16,1.,-1.020425574104E-16)) ;
#87715=DIRECTION('center_axis',(6.27714964143733E-33,-5.10212787052002E-17,
-1.)) ;
#87716=DIRECTION('ref_axis',(0.,1.,-5.10212787052002E-17)) ;
#87717=DIRECTION('center_axis',(-6.27714964143733E-33,5.10212787052002E-17,
1.)) ;
#87718=DIRECTION('ref_axis',(3.20268201330022E-49,1.,-5.10212787052002E-17)) ;
#87719=DIRECTION('',(1.2303003375722E-16,-1.,5.10212787052002E-17)) ;
#87720=DIRECTION('',(1.,0.,6.27714964143733E-33)) ;
#87721=DIRECTION('',(-2.16840434497101E-16,1.,-5.10212787052002E-17)) ;
#87722=DIRECTION('',(-1.,-1.53063836115601E-16,1.53236300070382E-33)) ;
#87723=DIRECTION('center_axis',(-1.25542992828747E-32,1.020425574104E-16,
1.)) ;
#87724=DIRECTION('ref_axis',(0.,-1.,1.020425574104E-16)) ;
#87725=DIRECTION('center_axis',(1.25542992828747E-32,-1.020425574104E-16,
-1.)) ;
#87726=DIRECTION('ref_axis',(-1.28107280532009E-48,-1.,1.020425574104E-16)) ;
#87727=DIRECTION('',(1.,1.53063836115601E-16,-3.06472600140763E-33)) ;
#87728=DIRECTION('',(2.16840434497101E-16,-1.,1.020425574104E-16)) ;
#87729=DIRECTION('',(-1.,0.,-1.25542992828747E-32)) ;
#87730=DIRECTION('',(-1.2303003375722E-16,1.,-1.020425574104E-16)) ;
#87731=DIRECTION('center_axis',(6.27714964143733E-33,-5.10212787052002E-17,
-1.)) ;
#87732=DIRECTION('ref_axis',(0.,1.,-5.10212787052002E-17)) ;
#87733=DIRECTION('center_axis',(-6.27714964143733E-33,5.10212787052002E-17,
1.)) ;
#87734=DIRECTION('ref_axis',(3.20268201330022E-49,1.,-5.10212787052002E-17)) ;
#87735=DIRECTION('',(1.2303003375722E-16,-1.,5.10212787052002E-17)) ;
#87736=DIRECTION('',(1.,0.,6.27714964143733E-33)) ;
#87737=DIRECTION('',(-2.16840434497101E-16,1.,-5.10212787052002E-17)) ;
#87738=DIRECTION('',(-1.,-1.53063836115601E-16,1.53236300070382E-33)) ;
#87739=DIRECTION('center_axis',(-1.25542992828747E-32,1.020425574104E-16,
1.)) ;
#87740=DIRECTION('ref_axis',(0.,-1.,1.020425574104E-16)) ;
#87741=DIRECTION('center_axis',(1.25542992828747E-32,-1.020425574104E-16,
-1.)) ;
#87742=DIRECTION('ref_axis',(-1.28107280532009E-48,-1.,1.020425574104E-16)) ;
#87743=DIRECTION('',(1.,1.53063836115601E-16,-3.06472600140763E-33)) ;
#87744=DIRECTION('',(2.16840434497101E-16,-1.,1.020425574104E-16)) ;
#87745=DIRECTION('',(-1.,0.,-1.25542992828747E-32)) ;
#87746=DIRECTION('',(-1.2303003375722E-16,1.,-1.020425574104E-16)) ;
#87747=DIRECTION('center_axis',(6.27714964143733E-33,-5.10212787052002E-17,
-1.)) ;
#87748=DIRECTION('ref_axis',(0.,1.,-5.10212787052002E-17)) ;
#87749=DIRECTION('center_axis',(-6.27714964143733E-33,5.10212787052002E-17,
1.)) ;
#87750=DIRECTION('ref_axis',(3.20268201330022E-49,1.,-5.10212787052002E-17)) ;
#87751=DIRECTION('',(1.2303003375722E-16,-1.,5.10212787052002E-17)) ;
#87752=DIRECTION('',(1.,0.,6.27714964143733E-33)) ;
#87753=DIRECTION('',(-2.16840434497101E-16,1.,-5.10212787052002E-17)) ;
#87754=DIRECTION('',(-1.,-1.53063836115601E-16,1.53236300070382E-33)) ;
#87755=DIRECTION('center_axis',(-1.25542992828747E-32,1.020425574104E-16,
1.)) ;
#87756=DIRECTION('ref_axis',(0.,-1.,1.020425574104E-16)) ;
#87757=DIRECTION('center_axis',(1.25542992828747E-32,-1.020425574104E-16,
-1.)) ;
#87758=DIRECTION('ref_axis',(-1.28107280532009E-48,-1.,1.020425574104E-16)) ;
#87759=DIRECTION('',(1.,1.53063836115601E-16,-3.06472600140763E-33)) ;
#87760=DIRECTION('',(2.16840434497101E-16,-1.,1.020425574104E-16)) ;
#87761=DIRECTION('',(-1.,0.,-1.25542992828747E-32)) ;
#87762=DIRECTION('',(-1.2303003375722E-16,1.,-1.020425574104E-16)) ;
#87763=DIRECTION('center_axis',(6.27714964143733E-33,-5.10212787052002E-17,
-1.)) ;
#87764=DIRECTION('ref_axis',(0.,1.,-5.10212787052002E-17)) ;
#87765=DIRECTION('center_axis',(-6.27714964143733E-33,5.10212787052002E-17,
1.)) ;
#87766=DIRECTION('ref_axis',(3.20268201330022E-49,1.,-5.10212787052002E-17)) ;
#87767=DIRECTION('',(1.2303003375722E-16,-1.,5.10212787052002E-17)) ;
#87768=DIRECTION('',(1.,0.,6.27714964143733E-33)) ;
#87769=DIRECTION('',(-2.16840434497101E-16,1.,-5.10212787052002E-17)) ;
#87770=DIRECTION('',(-1.,-1.53063836115601E-16,1.53236300070382E-33)) ;
#87771=DIRECTION('center_axis',(-1.25542992828747E-32,1.020425574104E-16,
1.)) ;
#87772=DIRECTION('ref_axis',(0.,-1.,1.020425574104E-16)) ;
#87773=DIRECTION('center_axis',(1.25542992828747E-32,-1.020425574104E-16,
-1.)) ;
#87774=DIRECTION('ref_axis',(-1.28107280532009E-48,-1.,1.020425574104E-16)) ;
#87775=DIRECTION('',(1.,1.53063836115601E-16,-3.06472600140763E-33)) ;
#87776=DIRECTION('',(2.16840434497101E-16,-1.,1.020425574104E-16)) ;
#87777=DIRECTION('',(-1.,0.,-1.25542992828747E-32)) ;
#87778=DIRECTION('',(-1.2303003375722E-16,1.,-1.020425574104E-16)) ;
#87779=DIRECTION('center_axis',(6.27714964143733E-33,-5.10212787052002E-17,
-1.)) ;
#87780=DIRECTION('ref_axis',(0.,1.,-5.10212787052002E-17)) ;
#87781=DIRECTION('center_axis',(-6.27714964143733E-33,5.10212787052002E-17,
1.)) ;
#87782=DIRECTION('ref_axis',(3.20268201330022E-49,1.,-5.10212787052002E-17)) ;
#87783=DIRECTION('',(1.2303003375722E-16,-1.,5.10212787052002E-17)) ;
#87784=DIRECTION('',(1.,0.,6.27714964143733E-33)) ;
#87785=DIRECTION('',(-2.16840434497101E-16,1.,-5.10212787052002E-17)) ;
#87786=DIRECTION('',(-1.,-1.53063836115601E-16,1.53236300070382E-33)) ;
#87787=DIRECTION('center_axis',(-1.25542992828747E-32,1.020425574104E-16,
1.)) ;
#87788=DIRECTION('ref_axis',(0.,-1.,1.020425574104E-16)) ;
#87789=DIRECTION('center_axis',(1.25542992828747E-32,-1.020425574104E-16,
-1.)) ;
#87790=DIRECTION('ref_axis',(-1.28107280532009E-48,-1.,1.020425574104E-16)) ;
#87791=DIRECTION('',(1.,1.53063836115601E-16,-3.06472600140763E-33)) ;
#87792=DIRECTION('',(2.16840434497101E-16,-1.,1.020425574104E-16)) ;
#87793=DIRECTION('',(-1.,0.,-1.25542992828747E-32)) ;
#87794=DIRECTION('',(-1.2303003375722E-16,1.,-1.020425574104E-16)) ;
#87795=DIRECTION('center_axis',(6.27714964143733E-33,-5.10212787052002E-17,
-1.)) ;
#87796=DIRECTION('ref_axis',(0.,1.,-5.10212787052002E-17)) ;
#87797=DIRECTION('center_axis',(-6.27714964143733E-33,5.10212787052002E-17,
1.)) ;
#87798=DIRECTION('ref_axis',(3.20268201330022E-49,1.,-5.10212787052002E-17)) ;
#87799=DIRECTION('',(1.2303003375722E-16,-1.,5.10212787052002E-17)) ;
#87800=DIRECTION('',(1.,0.,6.27714964143733E-33)) ;
#87801=DIRECTION('',(-2.16840434497101E-16,1.,-5.10212787052002E-17)) ;
#87802=DIRECTION('',(-1.,-1.53063836115601E-16,1.53236300070382E-33)) ;
#87803=DIRECTION('center_axis',(-1.25542992828747E-32,1.020425574104E-16,
1.)) ;
#87804=DIRECTION('ref_axis',(0.,-1.,1.020425574104E-16)) ;
#87805=DIRECTION('center_axis',(1.25542992828747E-32,-1.020425574104E-16,
-1.)) ;
#87806=DIRECTION('ref_axis',(-1.28107280532009E-48,-1.,1.020425574104E-16)) ;
#87807=DIRECTION('',(1.,1.53063836115601E-16,-3.06472600140763E-33)) ;
#87808=DIRECTION('',(2.16840434497101E-16,-1.,1.020425574104E-16)) ;
#87809=DIRECTION('',(-1.,0.,-1.25542992828747E-32)) ;
#87810=DIRECTION('',(-1.2303003375722E-16,1.,-1.020425574104E-16)) ;
#87811=DIRECTION('center_axis',(6.27714964143733E-33,-5.10212787052002E-17,
-1.)) ;
#87812=DIRECTION('ref_axis',(0.,1.,-5.10212787052002E-17)) ;
#87813=DIRECTION('center_axis',(-6.27714964143733E-33,5.10212787052002E-17,
1.)) ;
#87814=DIRECTION('ref_axis',(3.20268201330022E-49,1.,-5.10212787052002E-17)) ;
#87815=DIRECTION('',(1.2303003375722E-16,-1.,5.10212787052002E-17)) ;
#87816=DIRECTION('',(1.,0.,6.27714964143733E-33)) ;
#87817=DIRECTION('',(-2.16840434497101E-16,1.,-5.10212787052002E-17)) ;
#87818=DIRECTION('',(-1.,-1.53063836115601E-16,1.53236300070382E-33)) ;
#87819=DIRECTION('center_axis',(-1.25542992828747E-32,1.020425574104E-16,
1.)) ;
#87820=DIRECTION('ref_axis',(0.,-1.,1.020425574104E-16)) ;
#87821=DIRECTION('center_axis',(1.25542992828747E-32,-1.020425574104E-16,
-1.)) ;
#87822=DIRECTION('ref_axis',(-1.28107280532009E-48,-1.,1.020425574104E-16)) ;
#87823=DIRECTION('',(1.,1.53063836115601E-16,-3.06472600140763E-33)) ;
#87824=DIRECTION('',(2.16840434497101E-16,-1.,1.020425574104E-16)) ;
#87825=DIRECTION('',(-1.,0.,-1.25542992828747E-32)) ;
#87826=DIRECTION('',(-1.2303003375722E-16,1.,-1.020425574104E-16)) ;
#87827=DIRECTION('center_axis',(0.,0.,1.)) ;
#87828=DIRECTION('ref_axis',(1.,0.,0.)) ;
#87829=DIRECTION('',(0.,0.,1.)) ;
#87830=DIRECTION('center_axis',(0.,0.,1.)) ;
#87831=DIRECTION('ref_axis',(1.,0.,0.)) ;
#87832=DIRECTION('',(0.,0.,1.)) ;
#87833=DIRECTION('center_axis',(0.,0.,-1.)) ;
#87834=DIRECTION('ref_axis',(1.,0.,0.)) ;
#87835=DIRECTION('center_axis',(0.,0.,1.)) ;
#87836=DIRECTION('ref_axis',(1.,0.,0.)) ;
#87837=DIRECTION('',(0.,0.,1.)) ;
#87838=DIRECTION('center_axis',(0.,0.,1.)) ;
#87839=DIRECTION('ref_axis',(1.,0.,0.)) ;
#87840=DIRECTION('',(0.,0.,1.)) ;
#87841=DIRECTION('center_axis',(0.,0.,-1.)) ;
#87842=DIRECTION('ref_axis',(1.,0.,0.)) ;
#87843=DIRECTION('center_axis',(0.,0.,1.)) ;
#87844=DIRECTION('ref_axis',(1.,0.,0.)) ;
#87845=DIRECTION('',(0.,0.,1.)) ;
#87846=DIRECTION('center_axis',(0.,0.,1.)) ;
#87847=DIRECTION('ref_axis',(1.,0.,0.)) ;
#87848=DIRECTION('',(0.,0.,1.)) ;
#87849=DIRECTION('center_axis',(0.,0.,-1.)) ;
#87850=DIRECTION('ref_axis',(1.,0.,0.)) ;
#87851=DIRECTION('center_axis',(0.,0.,1.)) ;
#87852=DIRECTION('ref_axis',(1.,0.,0.)) ;
#87853=DIRECTION('',(0.,0.,1.)) ;
#87854=DIRECTION('center_axis',(0.,0.,1.)) ;
#87855=DIRECTION('ref_axis',(1.,0.,0.)) ;
#87856=DIRECTION('',(0.,0.,1.)) ;
#87857=DIRECTION('center_axis',(0.,0.,-1.)) ;
#87858=DIRECTION('ref_axis',(1.,0.,0.)) ;
#87859=DIRECTION('center_axis',(0.,0.,1.)) ;
#87860=DIRECTION('ref_axis',(1.,0.,0.)) ;
#87861=DIRECTION('',(0.,0.,1.)) ;
#87862=DIRECTION('center_axis',(0.,0.,1.)) ;
#87863=DIRECTION('ref_axis',(1.,0.,0.)) ;
#87864=DIRECTION('',(0.,0.,1.)) ;
#87865=DIRECTION('center_axis',(0.,0.,-1.)) ;
#87866=DIRECTION('ref_axis',(1.,0.,0.)) ;
#87867=DIRECTION('center_axis',(0.,0.,1.)) ;
#87868=DIRECTION('ref_axis',(1.,0.,0.)) ;
#87869=DIRECTION('',(0.,0.,1.)) ;
#87870=DIRECTION('center_axis',(0.,0.,1.)) ;
#87871=DIRECTION('ref_axis',(1.,0.,0.)) ;
#87872=DIRECTION('',(0.,0.,1.)) ;
#87873=DIRECTION('center_axis',(0.,0.,-1.)) ;
#87874=DIRECTION('ref_axis',(1.,0.,0.)) ;
#87875=DIRECTION('center_axis',(0.,0.,1.)) ;
#87876=DIRECTION('ref_axis',(1.,0.,0.)) ;
#87877=DIRECTION('',(0.,0.,1.)) ;
#87878=DIRECTION('center_axis',(0.,0.,1.)) ;
#87879=DIRECTION('ref_axis',(1.,0.,0.)) ;
#87880=DIRECTION('',(0.,0.,1.)) ;
#87881=DIRECTION('center_axis',(0.,0.,-1.)) ;
#87882=DIRECTION('ref_axis',(1.,0.,0.)) ;
#87883=DIRECTION('center_axis',(0.,0.,1.)) ;
#87884=DIRECTION('ref_axis',(1.,0.,0.)) ;
#87885=DIRECTION('',(0.,0.,1.)) ;
#87886=DIRECTION('center_axis',(0.,0.,1.)) ;
#87887=DIRECTION('ref_axis',(1.,0.,0.)) ;
#87888=DIRECTION('',(0.,0.,1.)) ;
#87889=DIRECTION('center_axis',(0.,0.,-1.)) ;
#87890=DIRECTION('ref_axis',(1.,0.,0.)) ;
#87891=DIRECTION('center_axis',(0.,0.,1.)) ;
#87892=DIRECTION('ref_axis',(1.,0.,0.)) ;
#87893=DIRECTION('',(0.,0.,1.)) ;
#87894=DIRECTION('center_axis',(0.,0.,1.)) ;
#87895=DIRECTION('ref_axis',(1.,0.,0.)) ;
#87896=DIRECTION('',(0.,0.,1.)) ;
#87897=DIRECTION('center_axis',(0.,0.,-1.)) ;
#87898=DIRECTION('ref_axis',(1.,0.,0.)) ;
#87899=DIRECTION('center_axis',(-1.,-2.16840434497101E-16,0.)) ;
#87900=DIRECTION('ref_axis',(2.16840434497101E-16,-1.,0.)) ;
#87901=DIRECTION('',(-2.16840434497101E-16,1.,1.30104260698261E-16)) ;
#87902=DIRECTION('center_axis',(1.,2.16840434497101E-16,0.)) ;
#87903=DIRECTION('ref_axis',(2.16840434497101E-16,-1.,0.)) ;
#87904=DIRECTION('',(0.,0.,-1.)) ;
#87905=DIRECTION('center_axis',(1.,2.16840434497101E-16,0.)) ;
#87906=DIRECTION('ref_axis',(2.16840434497101E-16,-1.,0.)) ;
#87907=DIRECTION('center_axis',(-1.,-2.16840434497101E-16,0.)) ;
#87908=DIRECTION('ref_axis',(2.16840434497101E-16,-1.,0.)) ;
#87909=DIRECTION('',(0.,0.,-1.)) ;
#87910=DIRECTION('',(2.16840434497101E-16,-1.,5.10212787052002E-17)) ;
#87911=DIRECTION('',(0.,0.,1.)) ;
#87912=DIRECTION('',(-2.16840434497101E-16,1.,-1.020425574104E-16)) ;
#87913=DIRECTION('',(0.,0.,-1.)) ;
#87914=DIRECTION('center_axis',(-1.,-2.16840434497101E-16,0.)) ;
#87915=DIRECTION('ref_axis',(2.16840434497101E-16,-1.,0.)) ;
#87916=DIRECTION('center_axis',(6.27714964143733E-33,-5.10212787052002E-17,
-1.)) ;
#87917=DIRECTION('ref_axis',(0.,1.,-5.10212787052002E-17)) ;
#87918=DIRECTION('center_axis',(-6.27714964143733E-33,5.10212787052002E-17,
1.)) ;
#87919=DIRECTION('ref_axis',(3.20268201330022E-49,1.,-5.10212787052002E-17)) ;
#87920=DIRECTION('',(1.2303003375722E-16,-1.,5.10212787052002E-17)) ;
#87921=DIRECTION('',(1.,0.,6.27714964143733E-33)) ;
#87922=DIRECTION('',(-2.16840434497101E-16,1.,-5.10212787052002E-17)) ;
#87923=DIRECTION('',(-1.,-1.53063836115601E-16,1.53236300070382E-33)) ;
#87924=DIRECTION('center_axis',(-1.25542992828747E-32,1.020425574104E-16,
1.)) ;
#87925=DIRECTION('ref_axis',(0.,-1.,1.020425574104E-16)) ;
#87926=DIRECTION('center_axis',(1.25542992828747E-32,-1.020425574104E-16,
-1.)) ;
#87927=DIRECTION('ref_axis',(-1.28107280532009E-48,-1.,1.020425574104E-16)) ;
#87928=DIRECTION('',(1.,1.53063836115601E-16,-3.06472600140763E-33)) ;
#87929=DIRECTION('',(2.16840434497101E-16,-1.,1.020425574104E-16)) ;
#87930=DIRECTION('',(-1.,0.,-1.25542992828747E-32)) ;
#87931=DIRECTION('',(-1.2303003375722E-16,1.,-1.020425574104E-16)) ;
#87932=DIRECTION('center_axis',(0.,0.,1.)) ;
#87933=DIRECTION('ref_axis',(1.,0.,0.)) ;
#87934=DIRECTION('',(0.,0.,1.)) ;
#87935=DIRECTION('center_axis',(0.,0.,1.)) ;
#87936=DIRECTION('ref_axis',(1.,0.,0.)) ;
#87937=DIRECTION('',(0.,0.,1.)) ;
#87938=DIRECTION('center_axis',(0.,0.,-1.)) ;
#87939=DIRECTION('ref_axis',(1.,0.,0.)) ;
#87940=DIRECTION('center_axis',(0.,0.,1.)) ;
#87941=DIRECTION('ref_axis',(1.,0.,0.)) ;
#87942=DIRECTION('',(0.,0.,1.)) ;
#87943=DIRECTION('center_axis',(0.,0.,1.)) ;
#87944=DIRECTION('ref_axis',(1.,0.,0.)) ;
#87945=DIRECTION('',(0.,0.,1.)) ;
#87946=DIRECTION('center_axis',(0.,0.,-1.)) ;
#87947=DIRECTION('ref_axis',(1.,0.,0.)) ;
#87948=DIRECTION('center_axis',(0.,-1.,0.)) ;
#87949=DIRECTION('ref_axis',(0.,0.,-1.)) ;
#87950=DIRECTION('center_axis',(0.,-1.,0.)) ;
#87951=DIRECTION('ref_axis',(0.,0.,-1.)) ;
#87952=DIRECTION('',(-1.,0.,-6.27714964143733E-33)) ;
#87953=DIRECTION('',(0.,0.,1.)) ;
#87954=DIRECTION('',(1.,0.,0.)) ;
#87955=DIRECTION('',(-1.,0.,0.)) ;
#87956=DIRECTION('',(1.,0.,1.25542992828747E-32)) ;
#87957=DIRECTION('center_axis',(0.,-1.,0.)) ;
#87958=DIRECTION('ref_axis',(0.,0.,-1.)) ;
#87959=DIRECTION('',(0.,0.,-1.)) ;
#87960=DIRECTION('center_axis',(0.,-1.,0.)) ;
#87961=DIRECTION('ref_axis',(0.,0.,-1.)) ;
#87962=DIRECTION('',(-1.,0.,-6.27714964143733E-33)) ;
#87963=DIRECTION('',(1.,0.,1.25542992828747E-32)) ;
#87964=DIRECTION('center_axis',(0.,-1.,0.)) ;
#87965=DIRECTION('ref_axis',(0.,0.,-1.)) ;
#87966=DIRECTION('',(0.,0.,-1.)) ;
#87967=DIRECTION('center_axis',(0.,-1.,0.)) ;
#87968=DIRECTION('ref_axis',(0.,0.,-1.)) ;
#87969=DIRECTION('',(-1.,0.,-6.27714964143733E-33)) ;
#87970=DIRECTION('',(1.,0.,1.25542992828747E-32)) ;
#87971=DIRECTION('center_axis',(0.,-1.,0.)) ;
#87972=DIRECTION('ref_axis',(0.,0.,-1.)) ;
#87973=DIRECTION('',(0.,0.,-1.)) ;
#87974=DIRECTION('center_axis',(0.,-1.,0.)) ;
#87975=DIRECTION('ref_axis',(0.,0.,-1.)) ;
#87976=DIRECTION('',(-1.,0.,-6.27714964143733E-33)) ;
#87977=DIRECTION('',(1.,0.,1.25542992828747E-32)) ;
#87978=DIRECTION('center_axis',(0.,-1.,0.)) ;
#87979=DIRECTION('ref_axis',(0.,0.,-1.)) ;
#87980=DIRECTION('',(0.,0.,-1.)) ;
#87981=DIRECTION('center_axis',(0.,-1.,0.)) ;
#87982=DIRECTION('ref_axis',(0.,0.,-1.)) ;
#87983=DIRECTION('',(-1.,0.,-6.27714964143733E-33)) ;
#87984=DIRECTION('',(1.,0.,1.25542992828747E-32)) ;
#87985=DIRECTION('center_axis',(0.,-1.,0.)) ;
#87986=DIRECTION('ref_axis',(0.,0.,-1.)) ;
#87987=DIRECTION('',(0.,0.,-1.)) ;
#87988=DIRECTION('center_axis',(0.,-1.,0.)) ;
#87989=DIRECTION('ref_axis',(0.,0.,-1.)) ;
#87990=DIRECTION('',(-1.,0.,-6.27714964143733E-33)) ;
#87991=DIRECTION('',(1.,0.,1.25542992828747E-32)) ;
#87992=DIRECTION('center_axis',(0.,-1.,0.)) ;
#87993=DIRECTION('ref_axis',(0.,0.,-1.)) ;
#87994=DIRECTION('',(0.,0.,-1.)) ;
#87995=DIRECTION('center_axis',(0.,-1.,0.)) ;
#87996=DIRECTION('ref_axis',(0.,0.,-1.)) ;
#87997=DIRECTION('',(-1.,0.,-6.27714964143733E-33)) ;
#87998=DIRECTION('',(1.,0.,1.25542992828747E-32)) ;
#87999=DIRECTION('center_axis',(0.,-1.,0.)) ;
#88000=DIRECTION('ref_axis',(0.,0.,-1.)) ;
#88001=DIRECTION('',(0.,0.,-1.)) ;
#88002=DIRECTION('center_axis',(0.,-1.,0.)) ;
#88003=DIRECTION('ref_axis',(0.,0.,-1.)) ;
#88004=DIRECTION('',(-1.,0.,-6.27714964143733E-33)) ;
#88005=DIRECTION('',(1.,0.,1.25542992828747E-32)) ;
#88006=DIRECTION('center_axis',(0.,-1.,0.)) ;
#88007=DIRECTION('ref_axis',(0.,0.,-1.)) ;
#88008=DIRECTION('',(0.,0.,-1.)) ;
#88009=DIRECTION('center_axis',(0.,-1.,0.)) ;
#88010=DIRECTION('ref_axis',(0.,0.,-1.)) ;
#88011=DIRECTION('',(-1.,0.,-6.27714964143733E-33)) ;
#88012=DIRECTION('',(1.,0.,1.25542992828747E-32)) ;
#88013=DIRECTION('center_axis',(0.,-1.,0.)) ;
#88014=DIRECTION('ref_axis',(0.,0.,-1.)) ;
#88015=DIRECTION('',(0.,0.,-1.)) ;
#88016=DIRECTION('center_axis',(0.,-1.,0.)) ;
#88017=DIRECTION('ref_axis',(0.,0.,-1.)) ;
#88018=DIRECTION('',(-1.,0.,-6.27714964143733E-33)) ;
#88019=DIRECTION('',(1.,0.,1.25542992828747E-32)) ;
#88020=DIRECTION('center_axis',(0.,-1.,0.)) ;
#88021=DIRECTION('ref_axis',(0.,0.,-1.)) ;
#88022=DIRECTION('',(0.,0.,-1.)) ;
#88023=DIRECTION('center_axis',(0.,0.,1.)) ;
#88024=DIRECTION('ref_axis',(1.,0.,0.)) ;
#88025=DIRECTION('center_axis',(0.,0.,-1.)) ;
#88026=DIRECTION('ref_axis',(1.,0.,0.)) ;
#88027=DIRECTION('',(0.,0.,1.)) ;
#88028=DIRECTION('center_axis',(0.,0.,1.)) ;
#88029=DIRECTION('ref_axis',(1.,0.,0.)) ;
#88030=DIRECTION('center_axis',(-1.,-1.2303003375722E-16,0.)) ;
#88031=DIRECTION('ref_axis',(1.2303003375722E-16,-1.,0.)) ;
#88032=DIRECTION('center_axis',(-1.,-1.2303003375722E-16,0.)) ;
#88033=DIRECTION('ref_axis',(1.2303003375722E-16,-1.,0.)) ;
#88034=DIRECTION('',(1.2303003375722E-16,-1.,1.020425574104E-16)) ;
#88035=DIRECTION('',(-1.2303003375722E-16,1.,-5.10212787052002E-17)) ;
#88036=DIRECTION('center_axis',(-1.,-1.2303003375722E-16,0.)) ;
#88037=DIRECTION('ref_axis',(1.2303003375722E-16,-1.,0.)) ;
#88038=DIRECTION('',(0.,0.,1.)) ;
#88039=DIRECTION('center_axis',(-1.,-1.2303003375722E-16,0.)) ;
#88040=DIRECTION('ref_axis',(1.2303003375722E-16,-1.,0.)) ;
#88041=DIRECTION('',(1.2303003375722E-16,-1.,1.020425574104E-16)) ;
#88042=DIRECTION('',(-1.2303003375722E-16,1.,-5.10212787052002E-17)) ;
#88043=DIRECTION('center_axis',(-1.,-1.2303003375722E-16,0.)) ;
#88044=DIRECTION('ref_axis',(1.2303003375722E-16,-1.,0.)) ;
#88045=DIRECTION('',(0.,0.,1.)) ;
#88046=DIRECTION('center_axis',(-1.,-1.2303003375722E-16,0.)) ;
#88047=DIRECTION('ref_axis',(1.2303003375722E-16,-1.,0.)) ;
#88048=DIRECTION('',(1.2303003375722E-16,-1.,1.020425574104E-16)) ;
#88049=DIRECTION('',(-1.2303003375722E-16,1.,-5.10212787052002E-17)) ;
#88050=DIRECTION('center_axis',(-1.,-1.2303003375722E-16,0.)) ;
#88051=DIRECTION('ref_axis',(1.2303003375722E-16,-1.,0.)) ;
#88052=DIRECTION('',(0.,0.,1.)) ;
#88053=DIRECTION('center_axis',(-1.,-1.2303003375722E-16,0.)) ;
#88054=DIRECTION('ref_axis',(1.2303003375722E-16,-1.,0.)) ;
#88055=DIRECTION('',(1.2303003375722E-16,-1.,1.020425574104E-16)) ;
#88056=DIRECTION('',(-1.2303003375722E-16,1.,-5.10212787052002E-17)) ;
#88057=DIRECTION('center_axis',(-1.,-1.2303003375722E-16,0.)) ;
#88058=DIRECTION('ref_axis',(1.2303003375722E-16,-1.,0.)) ;
#88059=DIRECTION('',(0.,0.,1.)) ;
#88060=DIRECTION('center_axis',(-1.,-1.2303003375722E-16,0.)) ;
#88061=DIRECTION('ref_axis',(1.2303003375722E-16,-1.,0.)) ;
#88062=DIRECTION('',(1.2303003375722E-16,-1.,1.020425574104E-16)) ;
#88063=DIRECTION('',(-1.2303003375722E-16,1.,-5.10212787052002E-17)) ;
#88064=DIRECTION('center_axis',(-1.,-1.2303003375722E-16,0.)) ;
#88065=DIRECTION('ref_axis',(1.2303003375722E-16,-1.,0.)) ;
#88066=DIRECTION('',(0.,0.,1.)) ;
#88067=DIRECTION('center_axis',(-1.,-1.2303003375722E-16,0.)) ;
#88068=DIRECTION('ref_axis',(1.2303003375722E-16,-1.,0.)) ;
#88069=DIRECTION('',(1.2303003375722E-16,-1.,1.020425574104E-16)) ;
#88070=DIRECTION('',(-1.2303003375722E-16,1.,-5.10212787052002E-17)) ;
#88071=DIRECTION('center_axis',(-1.,-1.2303003375722E-16,0.)) ;
#88072=DIRECTION('ref_axis',(1.2303003375722E-16,-1.,0.)) ;
#88073=DIRECTION('',(0.,0.,1.)) ;
#88074=DIRECTION('center_axis',(-1.,-1.2303003375722E-16,0.)) ;
#88075=DIRECTION('ref_axis',(1.2303003375722E-16,-1.,0.)) ;
#88076=DIRECTION('',(1.2303003375722E-16,-1.,1.020425574104E-16)) ;
#88077=DIRECTION('',(-1.2303003375722E-16,1.,-5.10212787052002E-17)) ;
#88078=DIRECTION('center_axis',(-1.,-1.2303003375722E-16,0.)) ;
#88079=DIRECTION('ref_axis',(1.2303003375722E-16,-1.,0.)) ;
#88080=DIRECTION('',(0.,0.,1.)) ;
#88081=DIRECTION('center_axis',(-1.,-1.2303003375722E-16,0.)) ;
#88082=DIRECTION('ref_axis',(1.2303003375722E-16,-1.,0.)) ;
#88083=DIRECTION('',(1.2303003375722E-16,-1.,1.020425574104E-16)) ;
#88084=DIRECTION('',(-1.2303003375722E-16,1.,-5.10212787052002E-17)) ;
#88085=DIRECTION('center_axis',(-1.,-1.2303003375722E-16,0.)) ;
#88086=DIRECTION('ref_axis',(1.2303003375722E-16,-1.,0.)) ;
#88087=DIRECTION('',(0.,0.,1.)) ;
#88088=DIRECTION('center_axis',(-1.,-1.2303003375722E-16,0.)) ;
#88089=DIRECTION('ref_axis',(1.2303003375722E-16,-1.,0.)) ;
#88090=DIRECTION('',(1.2303003375722E-16,-1.,1.020425574104E-16)) ;
#88091=DIRECTION('',(-1.2303003375722E-16,1.,-5.10212787052002E-17)) ;
#88092=DIRECTION('center_axis',(-1.,-1.2303003375722E-16,0.)) ;
#88093=DIRECTION('ref_axis',(1.2303003375722E-16,-1.,0.)) ;
#88094=DIRECTION('',(0.,0.,1.)) ;
#88095=DIRECTION('center_axis',(-1.,-1.2303003375722E-16,0.)) ;
#88096=DIRECTION('ref_axis',(1.2303003375722E-16,-1.,0.)) ;
#88097=DIRECTION('',(1.2303003375722E-16,-1.,1.020425574104E-16)) ;
#88098=DIRECTION('',(-1.2303003375722E-16,1.,0.)) ;
#88099=DIRECTION('',(0.,0.,1.)) ;
#88100=DIRECTION('',(1.2303003375722E-16,-1.,0.)) ;
#88101=DIRECTION('',(-1.2303003375722E-16,1.,-5.10212787052002E-17)) ;
#88102=DIRECTION('center_axis',(-1.,-1.2303003375722E-16,0.)) ;
#88103=DIRECTION('ref_axis',(1.2303003375722E-16,-1.,0.)) ;
#88104=DIRECTION('',(0.,0.,1.)) ;
#88105=DIRECTION('center_axis',(0.,0.,1.)) ;
#88106=DIRECTION('ref_axis',(1.,0.,0.)) ;
#88107=DIRECTION('',(0.,0.,1.)) ;
#88108=DIRECTION('center_axis',(0.,0.,1.)) ;
#88109=DIRECTION('ref_axis',(1.,0.,0.)) ;
#88110=DIRECTION('center_axis',(0.,0.,-1.)) ;
#88111=DIRECTION('ref_axis',(1.,0.,0.)) ;
#88112=DIRECTION('center_axis',(-1.59148942750166E-16,1.,0.)) ;
#88113=DIRECTION('ref_axis',(-1.,-1.59148942750166E-16,0.)) ;
#88114=DIRECTION('',(0.,0.,1.)) ;
#88115=DIRECTION('',(-1.,-1.59148942750166E-16,0.)) ;
#88116=DIRECTION('',(1.,1.59148942750166E-16,0.)) ;
#88117=DIRECTION('center_axis',(0.,0.,1.)) ;
#88118=DIRECTION('ref_axis',(1.,0.,0.)) ;
#88119=DIRECTION('',(0.,0.,1.)) ;
#88120=DIRECTION('center_axis',(0.,0.,-1.)) ;
#88121=DIRECTION('ref_axis',(1.,0.,0.)) ;
#88122=DIRECTION('center_axis',(0.,0.,1.)) ;
#88123=DIRECTION('ref_axis',(1.,0.,0.)) ;
#88124=DIRECTION('center_axis',(-1.,0.,0.)) ;
#88125=DIRECTION('ref_axis',(0.,0.,1.)) ;
#88126=DIRECTION('',(0.,0.,1.)) ;
#88127=DIRECTION('',(0.,-1.,0.)) ;
#88128=DIRECTION('',(0.,1.,0.)) ;
#88129=DIRECTION('center_axis',(0.,0.,1.)) ;
#88130=DIRECTION('ref_axis',(1.,0.,0.)) ;
#88131=DIRECTION('',(0.,0.,1.)) ;
#88132=DIRECTION('center_axis',(0.,0.,1.)) ;
#88133=DIRECTION('ref_axis',(1.,0.,0.)) ;
#88134=DIRECTION('center_axis',(0.,0.,-1.)) ;
#88135=DIRECTION('ref_axis',(1.,0.,0.)) ;
#88136=DIRECTION('center_axis',(0.,1.,0.)) ;
#88137=DIRECTION('ref_axis',(0.,0.,1.)) ;
#88138=DIRECTION('',(0.,0.,1.)) ;
#88139=DIRECTION('',(-1.,0.,0.)) ;
#88140=DIRECTION('',(1.,0.,0.)) ;
#88141=DIRECTION('center_axis',(0.,0.,1.)) ;
#88142=DIRECTION('ref_axis',(1.,0.,0.)) ;
#88143=DIRECTION('',(0.,0.,1.)) ;
#88144=DIRECTION('center_axis',(0.,0.,1.)) ;
#88145=DIRECTION('ref_axis',(1.,0.,0.)) ;
#88146=DIRECTION('center_axis',(0.,0.,-1.)) ;
#88147=DIRECTION('ref_axis',(1.,0.,0.)) ;
#88148=DIRECTION('center_axis',(1.,-4.33680868994203E-15,0.)) ;
#88149=DIRECTION('ref_axis',(4.33680868994203E-15,1.,0.)) ;
#88150=DIRECTION('',(0.,0.,1.)) ;
#88151=DIRECTION('',(4.33680868994203E-15,1.,0.)) ;
#88152=DIRECTION('',(-4.33680868994203E-15,-1.,0.)) ;
#88153=DIRECTION('center_axis',(0.,0.,1.)) ;
#88154=DIRECTION('ref_axis',(1.,0.,0.)) ;
#88155=DIRECTION('',(0.,0.,1.)) ;
#88156=DIRECTION('center_axis',(0.,0.,-1.)) ;
#88157=DIRECTION('ref_axis',(1.,0.,0.)) ;
#88158=DIRECTION('center_axis',(0.,0.,1.)) ;
#88159=DIRECTION('ref_axis',(1.,0.,0.)) ;
#88160=DIRECTION('center_axis',(5.88041856263325E-16,1.,0.)) ;
#88161=DIRECTION('ref_axis',(-1.,5.88041856263325E-16,0.)) ;
#88162=DIRECTION('',(0.,0.,1.)) ;
#88163=DIRECTION('',(-1.,5.88041856263325E-16,0.)) ;
#88164=DIRECTION('',(1.,-5.88041856263325E-16,0.)) ;
#88165=DIRECTION('center_axis',(0.,0.,1.)) ;
#88166=DIRECTION('ref_axis',(1.,0.,0.)) ;
#88167=DIRECTION('',(0.,0.,1.)) ;
#88168=DIRECTION('center_axis',(0.,0.,1.)) ;
#88169=DIRECTION('ref_axis',(1.,0.,0.)) ;
#88170=DIRECTION('center_axis',(0.,0.,-1.)) ;
#88171=DIRECTION('ref_axis',(1.,0.,0.)) ;
#88172=DIRECTION('center_axis',(1.,0.,0.)) ;
#88173=DIRECTION('ref_axis',(0.,0.,-1.)) ;
#88174=DIRECTION('',(0.,1.,0.)) ;
#88175=DIRECTION('',(0.,-1.,0.)) ;
#88176=DIRECTION('center_axis',(-1.,0.,0.)) ;
#88177=DIRECTION('ref_axis',(0.,0.,-1.)) ;
#88178=DIRECTION('',(0.,0.,-1.)) ;
#88179=DIRECTION('',(0.,1.,0.)) ;
#88180=DIRECTION('',(0.,3.99416362155027E-15,1.)) ;
#88181=DIRECTION('center_axis',(-1.,0.,0.)) ;
#88182=DIRECTION('ref_axis',(0.,6.50521303491307E-15,-1.)) ;
#88183=DIRECTION('',(0.,0.707106781186546,0.707106781186549)) ;
#88184=DIRECTION('center_axis',(-1.,0.,0.)) ;
#88185=DIRECTION('ref_axis',(0.,-1.51788304147972E-14,-1.)) ;
#88186=DIRECTION('',(0.,0.,-1.)) ;
#88187=DIRECTION('',(0.,-0.707106781186548,0.707106781186547)) ;
#88188=DIRECTION('center_axis',(-1.,0.,0.)) ;
#88189=DIRECTION('ref_axis',(0.,1.30104260698261E-14,-1.)) ;
#88190=DIRECTION('',(0.,0.,1.)) ;
#88191=DIRECTION('',(0.,-1.,0.)) ;
#88192=DIRECTION('',(0.,0.,-1.)) ;
#88193=DIRECTION('center_axis',(-1.,0.,0.)) ;
#88194=DIRECTION('ref_axis',(0.,1.19262238973406E-14,-1.)) ;
#88195=DIRECTION('',(0.,-1.,-1.07081696047951E-16)) ;
#88196=DIRECTION('center_axis',(-1.,0.,0.)) ;
#88197=DIRECTION('ref_axis',(0.,0.,-1.)) ;
#88198=DIRECTION('',(0.,0.,1.)) ;
#88199=DIRECTION('center_axis',(-1.,0.,0.)) ;
#88200=DIRECTION('ref_axis',(0.,4.33680868994204E-15,-1.)) ;
#88201=DIRECTION('center_axis',(1.,0.,0.)) ;
#88202=DIRECTION('ref_axis',(0.,0.,-1.)) ;
#88203=DIRECTION('center_axis',(-1.,0.,0.)) ;
#88204=DIRECTION('ref_axis',(0.,8.67361737988409E-15,-1.)) ;
#88205=DIRECTION('',(0.,0.,1.)) ;
#88206=DIRECTION('center_axis',(-1.,0.,0.)) ;
#88207=DIRECTION('ref_axis',(0.,0.,-1.)) ;
#88208=DIRECTION('',(0.,1.,1.07081696047951E-16)) ;
#88209=DIRECTION('center_axis',(-1.,0.,0.)) ;
#88210=DIRECTION('ref_axis',(0.,0.,-1.)) ;
#88211=DIRECTION('',(0.,0.,-1.)) ;
#88212=DIRECTION('',(0.,1.,0.)) ;
#88213=DIRECTION('',(0.,3.99416362155027E-15,1.)) ;
#88214=DIRECTION('center_axis',(-1.,0.,0.)) ;
#88215=DIRECTION('ref_axis',(0.,6.50521303491307E-15,-1.)) ;
#88216=DIRECTION('',(0.,0.707106781186546,0.707106781186549)) ;
#88217=DIRECTION('center_axis',(-1.,0.,0.)) ;
#88218=DIRECTION('ref_axis',(0.,0.,-1.)) ;
#88219=DIRECTION('',(0.,0.,-1.)) ;
#88220=DIRECTION('',(0.,-0.707106781186548,0.707106781186547)) ;
#88221=DIRECTION('center_axis',(-1.,0.,0.)) ;
#88222=DIRECTION('ref_axis',(0.,1.30104260698261E-14,-1.)) ;
#88223=DIRECTION('',(0.,0.,1.)) ;
#88224=DIRECTION('',(0.,-1.,0.)) ;
#88225=DIRECTION('',(0.,0.,-1.)) ;
#88226=DIRECTION('center_axis',(-1.,0.,0.)) ;
#88227=DIRECTION('ref_axis',(0.,1.08420217248551E-14,-1.)) ;
#88228=DIRECTION('',(0.,-1.,-1.07081696047951E-16)) ;
#88229=DIRECTION('center_axis',(-1.,0.,0.)) ;
#88230=DIRECTION('ref_axis',(0.,0.,-1.)) ;
#88231=DIRECTION('',(0.,0.,1.)) ;
#88232=DIRECTION('center_axis',(-1.,0.,0.)) ;
#88233=DIRECTION('ref_axis',(0.,4.33680868994204E-15,-1.)) ;
#88234=DIRECTION('center_axis',(1.,0.,0.)) ;
#88235=DIRECTION('ref_axis',(0.,0.,-1.)) ;
#88236=DIRECTION('center_axis',(-1.,0.,0.)) ;
#88237=DIRECTION('ref_axis',(0.,-2.16840434497102E-15,-1.)) ;
#88238=DIRECTION('',(0.,0.,1.)) ;
#88239=DIRECTION('center_axis',(-1.,0.,0.)) ;
#88240=DIRECTION('ref_axis',(0.,0.,-1.)) ;
#88241=DIRECTION('',(0.,1.,1.07081696047951E-16)) ;
#88242=DIRECTION('center_axis',(-1.,0.,0.)) ;
#88243=DIRECTION('ref_axis',(0.,0.,-1.)) ;
#88244=DIRECTION('',(0.,0.,-1.)) ;
#88245=DIRECTION('',(0.,1.,0.)) ;
#88246=DIRECTION('',(0.,3.99416362155027E-15,1.)) ;
#88247=DIRECTION('center_axis',(-1.,0.,0.)) ;
#88248=DIRECTION('ref_axis',(0.,6.50521303491307E-15,-1.)) ;
#88249=DIRECTION('',(0.,0.707106781186546,0.707106781186549)) ;
#88250=DIRECTION('center_axis',(-1.,0.,0.)) ;
#88251=DIRECTION('ref_axis',(0.,0.,-1.)) ;
#88252=DIRECTION('',(0.,0.,-1.)) ;
#88253=DIRECTION('',(0.,-0.707106781186548,0.707106781186547)) ;
#88254=DIRECTION('center_axis',(-1.,0.,0.)) ;
#88255=DIRECTION('ref_axis',(0.,0.,-1.)) ;
#88256=DIRECTION('',(0.,0.,1.)) ;
#88257=DIRECTION('',(0.,-1.,0.)) ;
#88258=DIRECTION('',(0.,0.,-1.)) ;
#88259=DIRECTION('center_axis',(-1.,0.,0.)) ;
#88260=DIRECTION('ref_axis',(0.,1.08420217248551E-14,-1.)) ;
#88261=DIRECTION('',(0.,-1.,-1.07081696047951E-16)) ;
#88262=DIRECTION('center_axis',(-1.,0.,0.)) ;
#88263=DIRECTION('ref_axis',(0.,0.,-1.)) ;
#88264=DIRECTION('',(0.,0.,1.)) ;
#88265=DIRECTION('center_axis',(-1.,0.,0.)) ;
#88266=DIRECTION('ref_axis',(0.,0.,-1.)) ;
#88267=DIRECTION('center_axis',(1.,0.,0.)) ;
#88268=DIRECTION('ref_axis',(0.,0.,-1.)) ;
#88269=DIRECTION('center_axis',(-1.,0.,0.)) ;
#88270=DIRECTION('ref_axis',(0.,-2.16840434497102E-15,-1.)) ;
#88271=DIRECTION('',(0.,0.,1.)) ;
#88272=DIRECTION('center_axis',(-1.,0.,0.)) ;
#88273=DIRECTION('ref_axis',(0.,0.,-1.)) ;
#88274=DIRECTION('',(0.,1.,1.07081696047951E-16)) ;
#88275=DIRECTION('center_axis',(-1.,0.,0.)) ;
#88276=DIRECTION('ref_axis',(0.,0.,-1.)) ;
#88277=DIRECTION('',(0.,0.,-1.)) ;
#88278=DIRECTION('',(0.,1.,0.)) ;
#88279=DIRECTION('',(0.,3.99416362155027E-15,1.)) ;
#88280=DIRECTION('center_axis',(-1.,0.,0.)) ;
#88281=DIRECTION('ref_axis',(0.,6.50521303491307E-15,-1.)) ;
#88282=DIRECTION('',(0.,0.707106781186546,0.707106781186549)) ;
#88283=DIRECTION('center_axis',(-1.,0.,0.)) ;
#88284=DIRECTION('ref_axis',(0.,0.,-1.)) ;
#88285=DIRECTION('',(0.,0.,-1.)) ;
#88286=DIRECTION('',(0.,-0.707106781186548,0.707106781186547)) ;
#88287=DIRECTION('center_axis',(-1.,0.,0.)) ;
#88288=DIRECTION('ref_axis',(0.,0.,-1.)) ;
#88289=DIRECTION('',(0.,0.,1.)) ;
#88290=DIRECTION('',(0.,-1.,0.)) ;
#88291=DIRECTION('',(0.,0.,-1.)) ;
#88292=DIRECTION('center_axis',(-1.,0.,0.)) ;
#88293=DIRECTION('ref_axis',(0.,1.08420217248551E-14,-1.)) ;
#88294=DIRECTION('',(0.,-1.,-1.07081696047951E-16)) ;
#88295=DIRECTION('center_axis',(-1.,0.,0.)) ;
#88296=DIRECTION('ref_axis',(0.,0.,-1.)) ;
#88297=DIRECTION('',(0.,0.,1.)) ;
#88298=DIRECTION('center_axis',(-1.,0.,0.)) ;
#88299=DIRECTION('ref_axis',(0.,0.,-1.)) ;
#88300=DIRECTION('center_axis',(1.,0.,0.)) ;
#88301=DIRECTION('ref_axis',(0.,0.,-1.)) ;
#88302=DIRECTION('center_axis',(-1.,0.,0.)) ;
#88303=DIRECTION('ref_axis',(0.,-2.16840434497102E-15,-1.)) ;
#88304=DIRECTION('',(0.,0.,1.)) ;
#88305=DIRECTION('center_axis',(-1.,0.,0.)) ;
#88306=DIRECTION('ref_axis',(0.,0.,-1.)) ;
#88307=DIRECTION('',(0.,1.,1.07081696047951E-16)) ;
#88308=DIRECTION('center_axis',(-1.,0.,0.)) ;
#88309=DIRECTION('ref_axis',(0.,0.,-1.)) ;
#88310=DIRECTION('',(0.,0.,-1.)) ;
#88311=DIRECTION('',(0.,1.,0.)) ;
#88312=DIRECTION('',(0.,3.99416362155027E-15,1.)) ;
#88313=DIRECTION('center_axis',(-1.,0.,0.)) ;
#88314=DIRECTION('ref_axis',(0.,6.50521303491307E-15,-1.)) ;
#88315=DIRECTION('',(0.,0.707106781186546,0.707106781186549)) ;
#88316=DIRECTION('center_axis',(-1.,0.,0.)) ;
#88317=DIRECTION('ref_axis',(0.,0.,-1.)) ;
#88318=DIRECTION('',(0.,0.,-1.)) ;
#88319=DIRECTION('',(0.,-0.707106781186548,0.707106781186547)) ;
#88320=DIRECTION('center_axis',(-1.,0.,0.)) ;
#88321=DIRECTION('ref_axis',(0.,0.,-1.)) ;
#88322=DIRECTION('',(0.,0.,1.)) ;
#88323=DIRECTION('',(0.,-1.,0.)) ;
#88324=DIRECTION('',(0.,0.,-1.)) ;
#88325=DIRECTION('center_axis',(-1.,0.,0.)) ;
#88326=DIRECTION('ref_axis',(0.,1.08420217248551E-14,-1.)) ;
#88327=DIRECTION('',(0.,-1.,-1.07081696047951E-16)) ;
#88328=DIRECTION('center_axis',(-1.,0.,0.)) ;
#88329=DIRECTION('ref_axis',(0.,0.,-1.)) ;
#88330=DIRECTION('',(0.,0.,1.)) ;
#88331=DIRECTION('center_axis',(-1.,0.,0.)) ;
#88332=DIRECTION('ref_axis',(0.,0.,-1.)) ;
#88333=DIRECTION('center_axis',(1.,0.,0.)) ;
#88334=DIRECTION('ref_axis',(0.,0.,-1.)) ;
#88335=DIRECTION('center_axis',(-1.,0.,0.)) ;
#88336=DIRECTION('ref_axis',(0.,-2.16840434497102E-15,-1.)) ;
#88337=DIRECTION('',(0.,0.,1.)) ;
#88338=DIRECTION('center_axis',(-1.,0.,0.)) ;
#88339=DIRECTION('ref_axis',(0.,0.,-1.)) ;
#88340=DIRECTION('',(0.,1.,1.07081696047951E-16)) ;
#88341=DIRECTION('center_axis',(-1.,0.,0.)) ;
#88342=DIRECTION('ref_axis',(0.,0.,-1.)) ;
#88343=DIRECTION('',(0.,0.,-1.)) ;
#88344=DIRECTION('',(0.,1.,0.)) ;
#88345=DIRECTION('',(0.,3.99416362155027E-15,1.)) ;
#88346=DIRECTION('center_axis',(-1.,0.,0.)) ;
#88347=DIRECTION('ref_axis',(0.,2.16840434497102E-15,-1.)) ;
#88348=DIRECTION('',(0.,0.707106781186546,0.707106781186549)) ;
#88349=DIRECTION('center_axis',(-1.,0.,0.)) ;
#88350=DIRECTION('ref_axis',(0.,0.,-1.)) ;
#88351=DIRECTION('',(0.,0.,-1.)) ;
#88352=DIRECTION('',(0.,-0.707106781186548,0.707106781186547)) ;
#88353=DIRECTION('center_axis',(-1.,0.,0.)) ;
#88354=DIRECTION('ref_axis',(0.,0.,-1.)) ;
#88355=DIRECTION('',(0.,0.,1.)) ;
#88356=DIRECTION('',(0.,-1.,0.)) ;
#88357=DIRECTION('',(0.,0.,-1.)) ;
#88358=DIRECTION('center_axis',(-1.,0.,0.)) ;
#88359=DIRECTION('ref_axis',(0.,1.08420217248551E-14,-1.)) ;
#88360=DIRECTION('',(0.,-1.,-1.07081696047951E-16)) ;
#88361=DIRECTION('center_axis',(-1.,0.,0.)) ;
#88362=DIRECTION('ref_axis',(0.,0.,-1.)) ;
#88363=DIRECTION('',(0.,0.,1.)) ;
#88364=DIRECTION('center_axis',(-1.,0.,0.)) ;
#88365=DIRECTION('ref_axis',(0.,0.,-1.)) ;
#88366=DIRECTION('center_axis',(1.,0.,0.)) ;
#88367=DIRECTION('ref_axis',(0.,0.,-1.)) ;
#88368=DIRECTION('center_axis',(-1.,0.,0.)) ;
#88369=DIRECTION('ref_axis',(0.,-2.168404344971E-15,-1.)) ;
#88370=DIRECTION('',(0.,0.,1.)) ;
#88371=DIRECTION('center_axis',(-1.,0.,0.)) ;
#88372=DIRECTION('ref_axis',(0.,0.,-1.)) ;
#88373=DIRECTION('',(0.,1.,1.07081696047951E-16)) ;
#88374=DIRECTION('center_axis',(-1.,0.,0.)) ;
#88375=DIRECTION('ref_axis',(0.,0.,-1.)) ;
#88376=DIRECTION('',(0.,0.,-1.)) ;
#88377=DIRECTION('',(0.,1.,0.)) ;
#88378=DIRECTION('',(0.,3.99416362155027E-15,1.)) ;
#88379=DIRECTION('center_axis',(-1.,0.,0.)) ;
#88380=DIRECTION('ref_axis',(0.,2.16840434497102E-15,-1.)) ;
#88381=DIRECTION('',(0.,0.707106781186546,0.707106781186549)) ;
#88382=DIRECTION('center_axis',(-1.,0.,0.)) ;
#88383=DIRECTION('ref_axis',(0.,0.,-1.)) ;
#88384=DIRECTION('',(0.,0.,-1.)) ;
#88385=DIRECTION('',(0.,-0.707106781186548,0.707106781186547)) ;
#88386=DIRECTION('center_axis',(-1.,0.,0.)) ;
#88387=DIRECTION('ref_axis',(0.,0.,-1.)) ;
#88388=DIRECTION('',(0.,0.,1.)) ;
#88389=DIRECTION('',(0.,-1.,0.)) ;
#88390=DIRECTION('',(0.,0.,-1.)) ;
#88391=DIRECTION('center_axis',(-1.,0.,0.)) ;
#88392=DIRECTION('ref_axis',(0.,1.0842021724855E-14,-1.)) ;
#88393=DIRECTION('',(0.,-1.,-1.07081696047951E-16)) ;
#88394=DIRECTION('center_axis',(-1.,0.,0.)) ;
#88395=DIRECTION('ref_axis',(0.,0.,-1.)) ;
#88396=DIRECTION('',(0.,0.,1.)) ;
#88397=DIRECTION('center_axis',(-1.,0.,0.)) ;
#88398=DIRECTION('ref_axis',(0.,-2.168404344971E-15,-1.)) ;
#88399=DIRECTION('center_axis',(1.,0.,0.)) ;
#88400=DIRECTION('ref_axis',(0.,0.,-1.)) ;
#88401=DIRECTION('center_axis',(-1.,0.,0.)) ;
#88402=DIRECTION('ref_axis',(0.,-2.168404344971E-15,-1.)) ;
#88403=DIRECTION('',(0.,0.,1.)) ;
#88404=DIRECTION('center_axis',(-1.,0.,0.)) ;
#88405=DIRECTION('ref_axis',(0.,0.,-1.)) ;
#88406=DIRECTION('',(0.,1.,1.07081696047951E-16)) ;
#88407=DIRECTION('center_axis',(-1.,0.,0.)) ;
#88408=DIRECTION('ref_axis',(0.,0.,-1.)) ;
#88409=DIRECTION('',(0.,0.,-1.)) ;
#88410=DIRECTION('',(0.,1.,0.)) ;
#88411=DIRECTION('',(0.,3.99416362155027E-15,1.)) ;
#88412=DIRECTION('center_axis',(-1.,0.,0.)) ;
#88413=DIRECTION('ref_axis',(0.,0.,-1.)) ;
#88414=DIRECTION('',(0.,0.707106781186546,0.707106781186549)) ;
#88415=DIRECTION('center_axis',(-1.,0.,0.)) ;
#88416=DIRECTION('ref_axis',(0.,0.,-1.)) ;
#88417=DIRECTION('',(0.,0.,-1.)) ;
#88418=DIRECTION('',(0.,-0.707106781186548,0.707106781186547)) ;
#88419=DIRECTION('center_axis',(-1.,0.,0.)) ;
#88420=DIRECTION('ref_axis',(0.,0.,-1.)) ;
#88421=DIRECTION('',(0.,0.,1.)) ;
#88422=DIRECTION('',(0.,-1.,0.)) ;
#88423=DIRECTION('',(0.,0.,-1.)) ;
#88424=DIRECTION('center_axis',(-1.,0.,0.)) ;
#88425=DIRECTION('ref_axis',(0.,1.0842021724855E-14,-1.)) ;
#88426=DIRECTION('',(0.,-1.,-1.07081696047951E-16)) ;
#88427=DIRECTION('center_axis',(-1.,0.,0.)) ;
#88428=DIRECTION('ref_axis',(0.,0.,-1.)) ;
#88429=DIRECTION('',(0.,0.,1.)) ;
#88430=DIRECTION('center_axis',(-1.,0.,0.)) ;
#88431=DIRECTION('ref_axis',(0.,-2.168404344971E-15,-1.)) ;
#88432=DIRECTION('center_axis',(1.,0.,0.)) ;
#88433=DIRECTION('ref_axis',(0.,0.,-1.)) ;
#88434=DIRECTION('center_axis',(-1.,0.,0.)) ;
#88435=DIRECTION('ref_axis',(0.,0.,-1.)) ;
#88436=DIRECTION('',(0.,0.,1.)) ;
#88437=DIRECTION('center_axis',(-1.,0.,0.)) ;
#88438=DIRECTION('ref_axis',(0.,0.,-1.)) ;
#88439=DIRECTION('',(0.,1.,1.07081696047951E-16)) ;
#88440=DIRECTION('center_axis',(-1.,0.,0.)) ;
#88441=DIRECTION('ref_axis',(0.,0.,-1.)) ;
#88442=DIRECTION('',(0.,0.,-1.)) ;
#88443=DIRECTION('',(0.,1.,0.)) ;
#88444=DIRECTION('',(0.,3.99416362155027E-15,1.)) ;
#88445=DIRECTION('center_axis',(-1.,0.,0.)) ;
#88446=DIRECTION('ref_axis',(0.,0.,-1.)) ;
#88447=DIRECTION('',(0.,0.707106781186546,0.707106781186549)) ;
#88448=DIRECTION('center_axis',(-1.,0.,0.)) ;
#88449=DIRECTION('ref_axis',(0.,0.,-1.)) ;
#88450=DIRECTION('',(0.,0.,-1.)) ;
#88451=DIRECTION('',(0.,-0.707106781186548,0.707106781186547)) ;
#88452=DIRECTION('center_axis',(-1.,0.,0.)) ;
#88453=DIRECTION('ref_axis',(0.,0.,-1.)) ;
#88454=DIRECTION('',(0.,0.,1.)) ;
#88455=DIRECTION('',(0.,-1.,0.)) ;
#88456=DIRECTION('',(0.,0.,-1.)) ;
#88457=DIRECTION('center_axis',(-1.,0.,0.)) ;
#88458=DIRECTION('ref_axis',(0.,9.75781955236956E-15,-1.)) ;
#88459=DIRECTION('',(0.,-1.,-1.07081696047951E-16)) ;
#88460=DIRECTION('center_axis',(-1.,0.,0.)) ;
#88461=DIRECTION('ref_axis',(0.,0.,-1.)) ;
#88462=DIRECTION('',(0.,0.,1.)) ;
#88463=DIRECTION('center_axis',(-1.,0.,0.)) ;
#88464=DIRECTION('ref_axis',(0.,-2.16840434497101E-15,-1.)) ;
#88465=DIRECTION('center_axis',(1.,0.,0.)) ;
#88466=DIRECTION('ref_axis',(0.,0.,-1.)) ;
#88467=DIRECTION('center_axis',(-1.,0.,0.)) ;
#88468=DIRECTION('ref_axis',(0.,0.,-1.)) ;
#88469=DIRECTION('',(0.,0.,1.)) ;
#88470=DIRECTION('center_axis',(-1.,0.,0.)) ;
#88471=DIRECTION('ref_axis',(0.,0.,-1.)) ;
#88472=DIRECTION('',(0.,1.,1.07081696047951E-16)) ;
#88473=DIRECTION('center_axis',(-1.,0.,0.)) ;
#88474=DIRECTION('ref_axis',(0.,-1.0842021724855E-15,-1.)) ;
#88475=DIRECTION('',(0.,0.,-1.)) ;
#88476=DIRECTION('',(0.,1.,0.)) ;
#88477=DIRECTION('',(0.,3.99416362155027E-15,1.)) ;
#88478=DIRECTION('center_axis',(-1.,0.,0.)) ;
#88479=DIRECTION('ref_axis',(0.,2.16840434497101E-15,-1.)) ;
#88480=DIRECTION('',(0.,0.707106781186546,0.707106781186549)) ;
#88481=DIRECTION('center_axis',(-1.,0.,0.)) ;
#88482=DIRECTION('ref_axis',(0.,0.,-1.)) ;
#88483=DIRECTION('',(0.,0.,-1.)) ;
#88484=DIRECTION('',(0.,-0.707106781186548,0.707106781186547)) ;
#88485=DIRECTION('center_axis',(-1.,0.,0.)) ;
#88486=DIRECTION('ref_axis',(0.,0.,-1.)) ;
#88487=DIRECTION('',(0.,0.,1.)) ;
#88488=DIRECTION('',(0.,-1.,0.)) ;
#88489=DIRECTION('',(0.,0.,-1.)) ;
#88490=DIRECTION('center_axis',(-1.,0.,0.)) ;
#88491=DIRECTION('ref_axis',(0.,8.67361737988403E-15,-1.)) ;
#88492=DIRECTION('',(0.,-1.,-1.07081696047951E-16)) ;
#88493=DIRECTION('center_axis',(-1.,0.,0.)) ;
#88494=DIRECTION('ref_axis',(0.,0.,-1.)) ;
#88495=DIRECTION('',(0.,0.,1.)) ;
#88496=DIRECTION('center_axis',(-1.,0.,0.)) ;
#88497=DIRECTION('ref_axis',(0.,2.16840434497101E-15,-1.)) ;
#88498=DIRECTION('center_axis',(1.,0.,0.)) ;
#88499=DIRECTION('ref_axis',(0.,0.,-1.)) ;
#88500=DIRECTION('center_axis',(-1.,0.,0.)) ;
#88501=DIRECTION('ref_axis',(0.,0.,-1.)) ;
#88502=DIRECTION('',(0.,0.,1.)) ;
#88503=DIRECTION('center_axis',(-1.,0.,0.)) ;
#88504=DIRECTION('ref_axis',(0.,0.,-1.)) ;
#88505=DIRECTION('',(0.,1.,1.07081696047951E-16)) ;
#88506=DIRECTION('center_axis',(0.,0.,1.)) ;
#88507=DIRECTION('ref_axis',(1.,0.,0.)) ;
#88508=DIRECTION('',(0.,-1.,0.)) ;
#88509=DIRECTION('',(-1.,0.,0.)) ;
#88510=DIRECTION('',(-1.2303003375722E-16,1.,0.)) ;
#88511=DIRECTION('',(1.,1.59148942750166E-16,0.)) ;
#88512=DIRECTION('center_axis',(0.,0.,1.)) ;
#88513=DIRECTION('ref_axis',(1.,0.,0.)) ;
#88514=DIRECTION('',(0.,1.,0.)) ;
#88515=DIRECTION('',(1.,0.,0.)) ;
#88516=DIRECTION('',(-4.33680868994203E-15,-1.,0.)) ;
#88517=DIRECTION('center_axis',(0.,0.,1.)) ;
#88518=DIRECTION('ref_axis',(1.,0.,0.)) ;
#88519=DIRECTION('',(1.,-5.88041856263325E-16,0.)) ;
#88520=DIRECTION('center_axis',(0.,0.,1.)) ;
#88521=DIRECTION('ref_axis',(1.,0.,0.)) ;
#88522=DIRECTION('',(1.2303003375722E-16,-1.,0.)) ;
#88523=DIRECTION('',(1.,0.,0.)) ;
#88524=DIRECTION('',(0.,1.,0.)) ;
#88525=DIRECTION('',(-1.,5.88041856263325E-16,0.)) ;
#88526=DIRECTION('center_axis',(0.,0.,-1.)) ;
#88527=DIRECTION('ref_axis',(1.,0.,0.)) ;
#88528=DIRECTION('',(4.33680868994203E-15,1.,0.)) ;
#88529=DIRECTION('',(-1.,0.,0.)) ;
#88530=DIRECTION('',(0.,-1.,0.)) ;
#88531=DIRECTION('center_axis',(0.,0.,-1.)) ;
#88532=DIRECTION('ref_axis',(1.,0.,0.)) ;
#88533=DIRECTION('',(-1.,-1.59148942750166E-16,0.)) ;
#88534=DIRECTION('center_axis',(-1.,-1.53063836115601E-16,0.)) ;
#88535=DIRECTION('ref_axis',(1.53063836115601E-16,-1.,0.)) ;
#88536=DIRECTION('',(0.,0.,1.)) ;
#88537=DIRECTION('',(-1.53063836115601E-16,1.,-1.020425574104E-16)) ;
#88538=DIRECTION('',(0.,0.,-1.)) ;
#88539=DIRECTION('',(1.53063836115601E-16,-1.,5.10212787052002E-17)) ;
#88540=DIRECTION('',(0.,0.,1.)) ;
#88541=DIRECTION('',(-1.53063836115601E-16,1.,-1.30104260698261E-16)) ;
#88542=DIRECTION('center_axis',(-1.,-1.53063836115601E-16,0.)) ;
#88543=DIRECTION('ref_axis',(1.53063836115601E-16,-1.,0.)) ;
#88544=DIRECTION('',(0.,0.,1.)) ;
#88545=DIRECTION('center_axis',(-1.,-1.53063836115601E-16,0.)) ;
#88546=DIRECTION('ref_axis',(1.53063836115601E-16,-1.,0.)) ;
#88547=DIRECTION('',(1.53063836115601E-16,-1.,-1.30104260698261E-16)) ;
#88548=DIRECTION('center_axis',(-1.53063836115601E-16,1.,0.)) ;
#88549=DIRECTION('ref_axis',(-1.,-1.53063836115601E-16,0.)) ;
#88550=DIRECTION('',(-1.,-1.53063836115601E-16,2.73691106313441E-48)) ;
#88551=DIRECTION('',(0.,0.,-1.)) ;
#88552=DIRECTION('',(1.,1.53063836115601E-16,-1.53236300070382E-33)) ;
#88553=DIRECTION('',(0.,0.,1.)) ;
#88554=DIRECTION('center_axis',(1.99142572374599E-32,-1.30104260698261E-16,
-1.)) ;
#88555=DIRECTION('ref_axis',(0.,1.,-1.30104260698261E-16)) ;
#88556=DIRECTION('',(-1.,-1.53063836115601E-16,2.73691106313441E-48)) ;
#88557=DIRECTION('',(1.53063836115601E-16,-1.,1.30104260698261E-16)) ;
#88558=DIRECTION('',(1.,1.53063836115601E-16,-2.73691106313441E-48)) ;
#88559=DIRECTION('center_axis',(-1.53063836115601E-16,1.,0.)) ;
#88560=DIRECTION('ref_axis',(-1.,-1.53063836115601E-16,0.)) ;
#88561=DIRECTION('',(-1.,-1.53063836115601E-16,-2.73691106313441E-48)) ;
#88562=DIRECTION('',(0.,0.,-1.)) ;
#88563=DIRECTION('',(1.,1.53063836115601E-16,-2.73691106313441E-48)) ;
#88564=DIRECTION('',(0.,0.,1.)) ;
#88565=DIRECTION('center_axis',(1.99142572374599E-32,-1.30104260698261E-16,
1.)) ;
#88566=DIRECTION('ref_axis',(0.,-1.,-1.30104260698261E-16)) ;
#88567=DIRECTION('',(-1.,-1.53063836115601E-16,-2.73691106313441E-48)) ;
#88568=DIRECTION('',(-1.53063836115601E-16,1.,1.30104260698261E-16)) ;
#88569=DIRECTION('',(1.,1.53063836115601E-16,2.73691106313441E-48)) ;
#88570=DIRECTION('',(2.16840434497101E-16,-1.,-1.30104260698261E-16)) ;
#88571=DIRECTION('center_axis',(-1.53063836115601E-16,1.,0.)) ;
#88572=DIRECTION('ref_axis',(-1.,-1.53063836115601E-16,0.)) ;
#88573=DIRECTION('',(-1.,-1.53063836115601E-16,3.06472600140763E-33)) ;
#88574=DIRECTION('',(0.,0.,-1.)) ;
#88575=DIRECTION('',(1.,1.53063836115601E-16,2.73691106313441E-48)) ;
#88576=DIRECTION('',(0.,0.,1.)) ;
#88577=DIRECTION('center_axis',(1.,0.,0.)) ;
#88578=DIRECTION('ref_axis',(0.,0.,-1.)) ;
#88579=DIRECTION('',(1.,0.,0.)) ;
#88580=DIRECTION('center_axis',(1.,0.,0.)) ;
#88581=DIRECTION('ref_axis',(0.,0.,1.)) ;
#88582=DIRECTION('',(1.,0.,0.)) ;
#88583=DIRECTION('center_axis',(-1.,0.,0.)) ;
#88584=DIRECTION('ref_axis',(0.,0.,-1.)) ;
#88585=DIRECTION('center_axis',(0.,0.,1.)) ;
#88586=DIRECTION('ref_axis',(1.,0.,0.)) ;
#88587=DIRECTION('',(0.,1.,0.)) ;
#88588=DIRECTION('',(1.,0.,0.)) ;
#88589=DIRECTION('',(0.,-1.,0.)) ;
#88590=DIRECTION('center_axis',(1.,0.,0.)) ;
#88591=DIRECTION('ref_axis',(0.,0.,-1.)) ;
#88592=DIRECTION('center_axis',(1.,0.,0.)) ;
#88593=DIRECTION('ref_axis',(0.,0.,1.)) ;
#88594=DIRECTION('',(1.,0.,0.)) ;
#88595=DIRECTION('center_axis',(-1.,0.,0.)) ;
#88596=DIRECTION('ref_axis',(0.,0.,-1.)) ;
#88597=DIRECTION('center_axis',(0.,-1.,3.99416362155027E-15)) ;
#88598=DIRECTION('ref_axis',(0.,-3.99416362155027E-15,-1.)) ;
#88599=DIRECTION('',(0.,3.99416362155027E-15,1.)) ;
#88600=DIRECTION('',(1.,0.,0.)) ;
#88601=DIRECTION('',(0.,-3.99416362155027E-15,-1.)) ;
#88602=DIRECTION('center_axis',(1.,0.,0.)) ;
#88603=DIRECTION('ref_axis',(0.,0.,-1.)) ;
#88604=DIRECTION('center_axis',(-1.,0.,0.)) ;
#88605=DIRECTION('ref_axis',(0.,0.,-1.)) ;
#88606=DIRECTION('',(1.,0.,0.)) ;
#88607=DIRECTION('center_axis',(1.,0.,0.)) ;
#88608=DIRECTION('ref_axis',(0.,0.,-1.)) ;
#88609=DIRECTION('center_axis',(0.,-0.707106781186549,0.707106781186546)) ;
#88610=DIRECTION('ref_axis',(0.,-0.707106781186546,-0.707106781186549)) ;
#88611=DIRECTION('',(0.,0.707106781186546,0.707106781186549)) ;
#88612=DIRECTION('',(1.,0.,0.)) ;
#88613=DIRECTION('',(0.,-0.707106781186546,-0.707106781186549)) ;
#88614=DIRECTION('center_axis',(1.,0.,0.)) ;
#88615=DIRECTION('ref_axis',(0.,0.382683432365091,0.923879532511286)) ;
#88616=DIRECTION('',(1.,0.,0.)) ;
#88617=DIRECTION('center_axis',(1.,0.,0.)) ;
#88618=DIRECTION('ref_axis',(0.,0.,-1.)) ;
#88619=DIRECTION('center_axis',(0.,1.,0.)) ;
#88620=DIRECTION('ref_axis',(0.,0.,1.)) ;
#88621=DIRECTION('',(0.,0.,-1.)) ;
#88622=DIRECTION('',(0.,0.,1.)) ;
#88623=DIRECTION('center_axis',(0.,-0.707106781186547,-0.707106781186548)) ;
#88624=DIRECTION('ref_axis',(0.,0.707106781186548,-0.707106781186547)) ;
#88625=DIRECTION('',(0.,-0.707106781186548,0.707106781186547)) ;
#88626=DIRECTION('',(1.,0.,0.)) ;
#88627=DIRECTION('',(0.,0.707106781186548,-0.707106781186547)) ;
#88628=DIRECTION('center_axis',(1.,0.,0.)) ;
#88629=DIRECTION('ref_axis',(0.,0.,-1.)) ;
#88630=DIRECTION('center_axis',(-1.,0.,0.)) ;
#88631=DIRECTION('ref_axis',(0.,0.,-1.)) ;
#88632=DIRECTION('',(1.,0.,0.)) ;
#88633=DIRECTION('center_axis',(1.,0.,0.)) ;
#88634=DIRECTION('ref_axis',(0.,0.,-1.)) ;
#88635=DIRECTION('center_axis',(0.,-1.,0.)) ;
#88636=DIRECTION('ref_axis',(0.,0.,-1.)) ;
#88637=DIRECTION('',(0.,0.,1.)) ;
#88638=DIRECTION('',(1.,0.,0.)) ;
#88639=DIRECTION('',(0.,0.,-1.)) ;
#88640=DIRECTION('center_axis',(1.,0.,0.)) ;
#88641=DIRECTION('ref_axis',(0.,0.,-1.)) ;
#88642=DIRECTION('center_axis',(1.,0.,0.)) ;
#88643=DIRECTION('ref_axis',(0.,0.,1.)) ;
#88644=DIRECTION('',(1.,0.,0.)) ;
#88645=DIRECTION('center_axis',(-1.,0.,0.)) ;
#88646=DIRECTION('ref_axis',(0.,0.,-1.)) ;
#88647=DIRECTION('center_axis',(0.,0.,-1.)) ;
#88648=DIRECTION('ref_axis',(-1.,0.,0.)) ;
#88649=DIRECTION('',(0.,-1.,0.)) ;
#88650=DIRECTION('',(1.,0.,0.)) ;
#88651=DIRECTION('',(0.,1.,0.)) ;
#88652=DIRECTION('center_axis',(1.,0.,0.)) ;
#88653=DIRECTION('ref_axis',(0.,0.,-1.)) ;
#88654=DIRECTION('center_axis',(1.,0.,0.)) ;
#88655=DIRECTION('ref_axis',(0.,0.,1.)) ;
#88656=DIRECTION('',(1.,0.,0.)) ;
#88657=DIRECTION('center_axis',(-1.,0.,0.)) ;
#88658=DIRECTION('ref_axis',(0.,0.,-1.)) ;
#88659=DIRECTION('center_axis',(0.,1.,0.)) ;
#88660=DIRECTION('ref_axis',(0.,0.,1.)) ;
#88661=DIRECTION('',(0.,0.,-1.)) ;
#88662=DIRECTION('',(1.,0.,0.)) ;
#88663=DIRECTION('',(0.,0.,1.)) ;
#88664=DIRECTION('center_axis',(1.,0.,0.)) ;
#88665=DIRECTION('ref_axis',(0.,0.,-1.)) ;
#88666=DIRECTION('center_axis',(-1.,0.,0.)) ;
#88667=DIRECTION('ref_axis',(0.,1.51788304147971E-14,-1.)) ;
#88668=DIRECTION('',(1.,0.,0.)) ;
#88669=DIRECTION('center_axis',(1.,0.,0.)) ;
#88670=DIRECTION('ref_axis',(0.,0.,-1.)) ;
#88671=DIRECTION('center_axis',(0.,1.07081696047951E-16,-1.)) ;
#88672=DIRECTION('ref_axis',(0.,1.,1.07081696047951E-16)) ;
#88673=DIRECTION('',(0.,-1.,-1.07081696047951E-16)) ;
#88674=DIRECTION('',(1.,0.,0.)) ;
#88675=DIRECTION('',(0.,1.,1.07081696047951E-16)) ;
#88676=DIRECTION('center_axis',(1.,0.,0.)) ;
#88677=DIRECTION('ref_axis',(0.,0.,-1.)) ;
#88678=DIRECTION('center_axis',(-1.,0.,0.)) ;
#88679=DIRECTION('ref_axis',(0.,0.,-1.)) ;
#88680=DIRECTION('',(1.,0.,0.)) ;
#88681=DIRECTION('center_axis',(1.,0.,0.)) ;
#88682=DIRECTION('ref_axis',(0.,0.,-1.)) ;
#88683=DIRECTION('center_axis',(0.,-1.,0.)) ;
#88684=DIRECTION('ref_axis',(0.,0.,-1.)) ;
#88685=DIRECTION('',(0.,0.,1.)) ;
#88686=DIRECTION('',(1.,0.,0.)) ;
#88687=DIRECTION('',(0.,0.,-1.)) ;
#88688=DIRECTION('center_axis',(1.,0.,0.)) ;
#88689=DIRECTION('ref_axis',(0.,0.,-1.)) ;
#88690=DIRECTION('center_axis',(-1.,0.,0.)) ;
#88691=DIRECTION('ref_axis',(0.,0.,-1.)) ;
#88692=DIRECTION('',(1.,0.,0.)) ;
#88693=DIRECTION('center_axis',(1.,0.,0.)) ;
#88694=DIRECTION('ref_axis',(0.,0.,-1.)) ;
#88695=DIRECTION('center_axis',(1.,0.,0.)) ;
#88696=DIRECTION('ref_axis',(0.,0.,-1.)) ;
#88697=DIRECTION('center_axis',(1.,0.,0.)) ;
#88698=DIRECTION('ref_axis',(0.,0.,1.)) ;
#88699=DIRECTION('',(1.,0.,0.)) ;
#88700=DIRECTION('center_axis',(-1.,0.,0.)) ;
#88701=DIRECTION('ref_axis',(0.,0.,-1.)) ;
#88702=DIRECTION('center_axis',(1.,0.,0.)) ;
#88703=DIRECTION('ref_axis',(0.,0.,-1.)) ;
#88704=DIRECTION('center_axis',(-1.,0.,0.)) ;
#88705=DIRECTION('ref_axis',(0.,0.,-1.)) ;
#88706=DIRECTION('',(1.,0.,0.)) ;
#88707=DIRECTION('center_axis',(1.,0.,0.)) ;
#88708=DIRECTION('ref_axis',(0.,0.,-1.)) ;
#88709=DIRECTION('center_axis',(0.,-1.,0.)) ;
#88710=DIRECTION('ref_axis',(0.,0.,-1.)) ;
#88711=DIRECTION('',(0.,0.,1.)) ;
#88712=DIRECTION('',(1.,0.,0.)) ;
#88713=DIRECTION('',(0.,0.,-1.)) ;
#88714=DIRECTION('center_axis',(1.,0.,0.)) ;
#88715=DIRECTION('ref_axis',(0.,0.,-1.)) ;
#88716=DIRECTION('center_axis',(-1.,0.,0.)) ;
#88717=DIRECTION('ref_axis',(0.,0.,-1.)) ;
#88718=DIRECTION('',(1.,0.,0.)) ;
#88719=DIRECTION('center_axis',(1.,0.,0.)) ;
#88720=DIRECTION('ref_axis',(0.,0.,-1.)) ;
#88721=DIRECTION('center_axis',(0.,-1.07081696047951E-16,1.)) ;
#88722=DIRECTION('ref_axis',(0.,-1.,-1.07081696047951E-16)) ;
#88723=DIRECTION('',(0.,1.,1.07081696047951E-16)) ;
#88724=DIRECTION('',(1.,0.,0.)) ;
#88725=DIRECTION('',(0.,-1.,-1.07081696047951E-16)) ;
#88726=DIRECTION('center_axis',(1.,0.,0.)) ;
#88727=DIRECTION('ref_axis',(0.,0.,-1.)) ;
#88728=DIRECTION('center_axis',(-1.,0.,0.)) ;
#88729=DIRECTION('ref_axis',(0.,0.,-1.)) ;
#88730=DIRECTION('',(1.,0.,0.)) ;
#88731=DIRECTION('center_axis',(1.,0.,0.)) ;
#88732=DIRECTION('ref_axis',(0.,0.,-1.)) ;
#88733=DIRECTION('center_axis',(0.,1.,0.)) ;
#88734=DIRECTION('ref_axis',(0.,0.,1.)) ;
#88735=DIRECTION('',(0.,0.,-1.)) ;
#88736=DIRECTION('',(0.,0.,1.)) ;
#88737=DIRECTION('center_axis',(-1.,0.,0.)) ;
#88738=DIRECTION('ref_axis',(0.,0.,1.)) ;
#88739=DIRECTION('center_axis',(-1.,0.,0.)) ;
#88740=DIRECTION('ref_axis',(0.,0.,1.)) ;
#88741=DIRECTION('',(0.,-1.,0.)) ;
#88742=DIRECTION('center_axis',(-1.,0.,0.)) ;
#88743=DIRECTION('ref_axis',(0.,0.,1.)) ;
#88744=DIRECTION('',(0.,0.,1.)) ;
#88745=DIRECTION('',(0.,-1.,-1.07081696047951E-16)) ;
#88746=DIRECTION('',(0.,0.,-1.)) ;
#88747=DIRECTION('center_axis',(-1.,0.,0.)) ;
#88748=DIRECTION('ref_axis',(0.,0.,1.)) ;
#88749=DIRECTION('',(0.,0.,-1.)) ;
#88750=DIRECTION('',(0.,1.,1.07081696047951E-16)) ;
#88751=DIRECTION('',(0.,0.,1.)) ;
#88752=DIRECTION('center_axis',(-1.,0.,0.)) ;
#88753=DIRECTION('ref_axis',(0.,0.,1.)) ;
#88754=DIRECTION('',(0.,1.,0.)) ;
#88755=DIRECTION('center_axis',(-1.,0.,0.)) ;
#88756=DIRECTION('ref_axis',(0.,0.,1.)) ;
#88757=DIRECTION('',(0.,0.,-1.)) ;
#88758=DIRECTION('',(0.,0.707106781186548,-0.707106781186547)) ;
#88759=DIRECTION('',(0.,0.,1.)) ;
#88760=DIRECTION('',(0.,-0.707106781186546,-0.707106781186549)) ;
#88761=DIRECTION('',(0.,-3.99416362155027E-15,-1.)) ;
#88762=DIRECTION('center_axis',(1.,0.,0.)) ;
#88763=DIRECTION('ref_axis',(0.,0.,-1.)) ;
#88764=DIRECTION('',(0.,-1.,0.)) ;
#88765=DIRECTION('center_axis',(-1.,0.,0.)) ;
#88766=DIRECTION('ref_axis',(0.,0.,-1.)) ;
#88767=DIRECTION('',(0.,0.,-1.)) ;
#88768=DIRECTION('center_axis',(-1.,0.,0.)) ;
#88769=DIRECTION('ref_axis',(0.,-1.0842021724855E-15,-1.)) ;
#88770=DIRECTION('',(0.,-1.,0.)) ;
#88771=DIRECTION('center_axis',(-1.,0.,0.)) ;
#88772=DIRECTION('ref_axis',(0.,0.,-1.)) ;
#88773=DIRECTION('',(0.,0.,1.)) ;
#88774=DIRECTION('center_axis',(-1.,0.,0.)) ;
#88775=DIRECTION('ref_axis',(0.,0.,-1.)) ;
#88776=DIRECTION('center_axis',(1.53063836115601E-16,-1.,-1.30104260698261E-16)) ;
#88777=DIRECTION('ref_axis',(1.,1.53063836115601E-16,1.99142572374599E-32)) ;
#88778=DIRECTION('center_axis',(0.,1.,0.)) ;
#88779=DIRECTION('ref_axis',(0.,0.,1.)) ;
#88780=DIRECTION('center_axis',(0.,-1.,0.)) ;
#88781=DIRECTION('ref_axis',(0.,0.,-1.)) ;
#88782=DIRECTION('center_axis',(1.,1.53063836115601E-16,2.73691106313441E-48)) ;
#88783=DIRECTION('ref_axis',(-1.53063836115601E-16,1.,-4.18922106430579E-64)) ;
#88784=DIRECTION('center_axis',(-1.,0.,0.)) ;
#88785=DIRECTION('ref_axis',(0.,0.,1.)) ;
#88786=DIRECTION('center_axis',(1.,1.53063836115601E-16,0.)) ;
#88787=DIRECTION('ref_axis',(1.53063836115601E-16,-1.,0.)) ;
#88788=DIRECTION('center_axis',(0.,1.,0.)) ;
#88789=DIRECTION('ref_axis',(1.,0.,0.)) ;
#88790=DIRECTION('center_axis',(0.,1.,0.)) ;
#88791=DIRECTION('ref_axis',(0.,0.,-1.)) ;
#88792=DIRECTION('center_axis',(0.,0.,1.)) ;
#88793=DIRECTION('ref_axis',(-1.,0.,0.)) ;
#88794=DIRECTION('center_axis',(0.,1.,0.)) ;
#88795=DIRECTION('ref_axis',(1.,0.,0.)) ;
#88796=DIRECTION('center_axis',(0.,0.,1.)) ;
#88797=DIRECTION('ref_axis',(-1.,0.,0.)) ;
#88798=DIRECTION('center_axis',(1.,1.0842021724855E-15,0.)) ;
#88799=DIRECTION('ref_axis',(1.0842021724855E-15,-1.,0.)) ;
#88800=DIRECTION('center_axis',(-1.,-1.53063836115601E-16,0.)) ;
#88801=DIRECTION('ref_axis',(0.,-1.,0.)) ;
#88802=DIRECTION('center_axis',(0.,0.,-1.)) ;
#88803=DIRECTION('ref_axis',(1.,0.,0.)) ;
#88804=DIRECTION('center_axis',(0.,0.,-1.)) ;
#88805=DIRECTION('ref_axis',(0.804034447892617,0.594582716366709,0.)) ;
#88806=DIRECTION('center_axis',(0.,0.,1.)) ;
#88807=DIRECTION('ref_axis',(1.,0.,0.)) ;
#88808=DIRECTION('',(0.,0.,-1.)) ;
#88809=DIRECTION('center_axis',(-2.16840434497101E-16,1.,1.30104260698261E-16)) ;
#88810=DIRECTION('ref_axis',(1.,2.16840434497101E-16,1.22464679914735E-16)) ;
#88811=DIRECTION('',(-2.16840434497101E-16,1.,1.30104260698261E-16)) ;
#88812=DIRECTION('center_axis',(0.,1.,0.)) ;
#88813=DIRECTION('ref_axis',(0.,0.,1.)) ;
#88814=DIRECTION('center_axis',(-1.,-1.53063836115601E-16,-2.73691106313441E-48)) ;
#88815=DIRECTION('ref_axis',(1.53063836115601E-16,-1.,4.18922106430579E-64)) ;
#88816=DIRECTION('center_axis',(1.,2.16840434497101E-16,0.)) ;
#88817=DIRECTION('ref_axis',(2.16840434497101E-16,-1.,0.)) ;
#88818=DIRECTION('center_axis',(0.,0.,1.)) ;
#88819=DIRECTION('ref_axis',(1.,0.,0.)) ;
#88820=DIRECTION('center_axis',(-1.25542992828747E-32,1.020425574104E-16,
1.)) ;
#88821=DIRECTION('ref_axis',(-1.28107280532009E-48,-1.,1.020425574104E-16)) ;
#88822=DIRECTION('center_axis',(0.,0.,1.)) ;
#88823=DIRECTION('ref_axis',(1.,0.,0.)) ;
#88824=DIRECTION('center_axis',(0.,0.,-1.)) ;
#88825=DIRECTION('ref_axis',(-1.,0.,0.)) ;
#88826=DIRECTION('center_axis',(1.,1.53063836115601E-16,-2.73691106313441E-48)) ;
#88827=DIRECTION('ref_axis',(-1.53063836115601E-16,1.,4.18922106430579E-64)) ;
#88828=DIRECTION('center_axis',(-1.,0.,0.)) ;
#88829=DIRECTION('ref_axis',(0.,0.,1.)) ;
#88830=DIRECTION('center_axis',(1.,1.53063836115601E-16,0.)) ;
#88831=DIRECTION('ref_axis',(1.53063836115601E-16,-1.,0.)) ;
#88832=DIRECTION('center_axis',(0.,1.,0.)) ;
#88833=DIRECTION('ref_axis',(1.,0.,0.)) ;
#88834=DIRECTION('center_axis',(-1.,-2.16840434497101E-16,0.)) ;
#88835=DIRECTION('ref_axis',(0.,-1.,0.)) ;
#88836=DIRECTION('center_axis',(0.,0.,-1.)) ;
#88837=DIRECTION('ref_axis',(1.,0.,0.)) ;
#88838=DIRECTION('center_axis',(-1.25542992828747E-32,1.020425574104E-16,
1.)) ;
#88839=DIRECTION('ref_axis',(0.,-1.,0.)) ;
#88840=DIRECTION('center_axis',(0.,-1.,0.)) ;
#88841=DIRECTION('ref_axis',(-6.50521303491302E-15,0.,1.)) ;
#88842=DIRECTION('center_axis',(-1.,0.,0.)) ;
#88843=DIRECTION('ref_axis',(0.,0.,-1.)) ;
#88844=DIRECTION('center_axis',(-1.,-1.53063836115601E-16,0.)) ;
#88845=DIRECTION('ref_axis',(0.,-1.,0.)) ;
#88846=DIRECTION('center_axis',(0.,-1.,0.)) ;
#88847=DIRECTION('ref_axis',(0.,0.,1.)) ;
#88848=DIRECTION('center_axis',(0.,0.,-1.)) ;
#88849=DIRECTION('ref_axis',(-1.,0.,0.)) ;
#88850=DIRECTION('center_axis',(0.,0.,-1.)) ;
#88851=DIRECTION('ref_axis',(-1.,0.,0.)) ;
#88852=DIRECTION('center_axis',(1.,1.53063836115601E-16,-3.06472600140763E-33)) ;
#88853=DIRECTION('ref_axis',(-1.53063836115601E-16,1.,4.69098718418678E-49)) ;
#88854=DIRECTION('center_axis',(-1.,0.,0.)) ;
#88855=DIRECTION('ref_axis',(0.,0.,1.)) ;
#88856=DIRECTION('center_axis',(-1.53063836115601E-16,1.,-1.020425574104E-16)) ;
#88857=DIRECTION('ref_axis',(-1.,-1.53063836115601E-16,1.3684555315672E-47)) ;
#88858=DIRECTION('',(1.53063836115601E-16,-1.,1.020425574104E-16)) ;
#88859=DIRECTION('center_axis',(0.,-1.,0.)) ;
#88860=DIRECTION('ref_axis',(0.,0.,-1.)) ;
#88861=DIRECTION('center_axis',(-1.53063836115601E-16,1.,-1.30104260698261E-16)) ;
#88862=DIRECTION('ref_axis',(-1.,-1.53063836115601E-16,1.99142572374599E-32)) ;
#88863=DIRECTION('center_axis',(0.,-1.,0.)) ;
#88864=DIRECTION('ref_axis',(0.,0.,-1.)) ;
#88865=DIRECTION('center_axis',(-1.,-1.53063836115601E-16,2.73691106313441E-48)) ;
#88866=DIRECTION('ref_axis',(1.53063836115601E-16,-1.,-4.18922106430579E-64)) ;
#88867=DIRECTION('center_axis',(1.,2.16840434497101E-16,0.)) ;
#88868=DIRECTION('ref_axis',(2.16840434497101E-16,-1.,0.)) ;
#88869=DIRECTION('center_axis',(-1.,0.,2.16840434497101E-15)) ;
#88870=DIRECTION('ref_axis',(2.16840434497101E-15,0.,1.)) ;
#88871=DIRECTION('center_axis',(-1.,-2.16840434497101E-16,0.)) ;
#88872=DIRECTION('ref_axis',(0.,-1.,0.)) ;
#88873=DIRECTION('center_axis',(0.,0.,1.)) ;
#88874=DIRECTION('ref_axis',(-1.,0.,0.)) ;
#88875=DIRECTION('center_axis',(0.,1.,0.)) ;
#88876=DIRECTION('ref_axis',(1.,0.,0.)) ;
#88877=DIRECTION('center_axis',(0.,1.,0.)) ;
#88878=DIRECTION('ref_axis',(0.,0.,-1.)) ;
#88879=DIRECTION('center_axis',(1.,0.,0.)) ;
#88880=DIRECTION('ref_axis',(0.,-1.,0.)) ;
#88881=DIRECTION('center_axis',(1.,6.50521303491304E-15,0.)) ;
#88882=DIRECTION('ref_axis',(-6.50521303491304E-15,1.,0.)) ;
#88883=DIRECTION('center_axis',(8.67361737988403E-15,1.,0.)) ;
#88884=DIRECTION('ref_axis',(-1.,8.67361737988403E-15,0.)) ;
#88885=DIRECTION('center_axis',(1.2303003375722E-16,-1.,1.020425574104E-16)) ;
#88886=DIRECTION('ref_axis',(1.,1.2303003375722E-16,-1.25542992828747E-32)) ;
#88887=DIRECTION('center_axis',(0.,1.,0.)) ;
#88888=DIRECTION('ref_axis',(0.,0.,1.)) ;
#88889=DIRECTION('center_axis',(0.,1.,0.)) ;
#88890=DIRECTION('ref_axis',(1.,0.,0.)) ;
#88891=DIRECTION('center_axis',(1.,1.2303003375722E-16,0.)) ;
#88892=DIRECTION('ref_axis',(1.2303003375722E-16,-1.,0.)) ;
#88893=DIRECTION('center_axis',(-2.16840434497101E-15,0.,1.)) ;
#88894=DIRECTION('ref_axis',(-1.,0.,-2.16840434497101E-15)) ;
#88895=DIRECTION('center_axis',(0.,1.,0.)) ;
#88896=DIRECTION('ref_axis',(1.,0.,0.)) ;
#88897=DIRECTION('center_axis',(0.,0.,-1.)) ;
#88898=DIRECTION('ref_axis',(1.,0.,0.)) ;
#88899=DIRECTION('center_axis',(0.,0.,-1.)) ;
#88900=DIRECTION('ref_axis',(-1.,0.,0.)) ;
#88901=DIRECTION('center_axis',(0.,0.,1.)) ;
#88902=DIRECTION('ref_axis',(1.,0.,0.)) ;
#88903=DIRECTION('center_axis',(-2.16840434497101E-16,1.,-1.020425574104E-16)) ;
#88904=DIRECTION('ref_axis',(-1.,-2.16840434497101E-16,5.47382212626882E-48)) ;
#88905=DIRECTION('center_axis',(0.,1.,0.)) ;
#88906=DIRECTION('ref_axis',(0.,0.,-1.)) ;
#88907=DIRECTION('center_axis',(1.,0.,1.25542992828747E-32)) ;
#88908=DIRECTION('ref_axis',(1.25542992828747E-32,0.,-1.)) ;
#88909=DIRECTION('center_axis',(1.,0.,0.)) ;
#88910=DIRECTION('ref_axis',(0.,0.,-1.)) ;
#88911=DIRECTION('center_axis',(-1.,-1.2303003375722E-16,0.)) ;
#88912=DIRECTION('ref_axis',(0.,-1.,0.)) ;
#88913=DIRECTION('center_axis',(0.,0.,-1.)) ;
#88914=DIRECTION('ref_axis',(1.,0.,0.)) ;
#88915=DIRECTION('center_axis',(0.,0.,-1.)) ;
#88916=DIRECTION('ref_axis',(-1.,0.,0.)) ;
#88917=DIRECTION('',(0.,0.,1.)) ;
#88918=DIRECTION('center_axis',(0.,-2.16840434497101E-15,1.)) ;
#88919=DIRECTION('ref_axis',(0.,-1.,-2.16840434497101E-15)) ;
#88920=DIRECTION('center_axis',(0.,0.,1.)) ;
#88921=DIRECTION('ref_axis',(1.,0.,0.)) ;
#88922=DIRECTION('center_axis',(6.27714964143733E-33,-5.10212787052002E-17,
-1.)) ;
#88923=DIRECTION('ref_axis',(3.20268201330022E-49,1.,-5.10212787052002E-17)) ;
#88924=DIRECTION('center_axis',(1.,1.53063836115601E-16,-1.53236300070382E-33)) ;
#88925=DIRECTION('ref_axis',(-1.53063836115601E-16,1.,2.34549359209339E-49)) ;
#88926=DIRECTION('center_axis',(-1.,0.,0.)) ;
#88927=DIRECTION('ref_axis',(0.,0.,1.)) ;
#88928=DIRECTION('center_axis',(1.,0.,0.)) ;
#88929=DIRECTION('ref_axis',(0.,0.,-1.)) ;
#88930=DIRECTION('center_axis',(0.,1.,0.)) ;
#88931=DIRECTION('ref_axis',(1.,0.,0.)) ;
#88932=DIRECTION('center_axis',(-4.33680868994202E-15,1.,0.)) ;
#88933=DIRECTION('ref_axis',(1.,4.33680868994202E-15,0.)) ;
#88934=DIRECTION('center_axis',(0.,-1.,0.)) ;
#88935=DIRECTION('ref_axis',(0.,0.,-1.)) ;
#88936=DIRECTION('center_axis',(0.,0.,-1.)) ;
#88937=DIRECTION('ref_axis',(1.,0.,0.)) ;
#88938=DIRECTION('center_axis',(0.,0.,1.)) ;
#88939=DIRECTION('ref_axis',(1.,0.,0.)) ;
#88940=DIRECTION('center_axis',(0.,0.,-1.)) ;
#88941=DIRECTION('ref_axis',(-1.,0.,0.)) ;
#88942=DIRECTION('center_axis',(0.,1.,0.)) ;
#88943=DIRECTION('ref_axis',(1.,0.,0.)) ;
#88944=DIRECTION('center_axis',(1.,1.2303003375722E-16,0.)) ;
#88945=DIRECTION('ref_axis',(1.2303003375722E-16,-1.,0.)) ;
#88946=DIRECTION('center_axis',(0.,1.,0.)) ;
#88947=DIRECTION('ref_axis',(-6.50521303491302E-15,0.,-1.)) ;
#88948=DIRECTION('center_axis',(6.27714964143733E-33,-5.10212787052002E-17,
-1.)) ;
#88949=DIRECTION('ref_axis',(0.,1.,0.)) ;
#88950=DIRECTION('center_axis',(0.,-1.,0.)) ;
#88951=DIRECTION('ref_axis',(0.,0.,1.)) ;
#88952=DIRECTION('center_axis',(2.16840434497101E-16,-1.,5.10212787052002E-17)) ;
#88953=DIRECTION('ref_axis',(1.,2.16840434497101E-16,-5.47382212626882E-48)) ;
#88954=DIRECTION('center_axis',(0.,1.,0.)) ;
#88955=DIRECTION('ref_axis',(0.,0.,-1.)) ;
#88956=DIRECTION('center_axis',(0.,0.,1.)) ;
#88957=DIRECTION('ref_axis',(1.,0.,0.)) ;
#88958=DIRECTION('center_axis',(0.,0.,-1.)) ;
#88959=DIRECTION('ref_axis',(-1.,0.,0.)) ;
#88960=DIRECTION('center_axis',(-1.,-1.2303003375722E-16,0.)) ;
#88961=DIRECTION('ref_axis',(0.,-1.,0.)) ;
#88962=DIRECTION('center_axis',(0.,-1.,0.)) ;
#88963=DIRECTION('ref_axis',(0.,0.,1.)) ;
#88964=DIRECTION('center_axis',(1.53063836115601E-16,-1.,5.10212787052002E-17)) ;
#88965=DIRECTION('ref_axis',(1.,1.53063836115601E-16,-6.84227765783602E-48)) ;
#88966=DIRECTION('',(-1.53063836115601E-16,1.,-5.10212787052002E-17)) ;
#88967=DIRECTION('center_axis',(0.,-1.,0.)) ;
#88968=DIRECTION('ref_axis',(0.,0.,-1.)) ;
#88969=DIRECTION('center_axis',(-1.,0.,0.)) ;
#88970=DIRECTION('ref_axis',(0.,0.,-1.)) ;
#88971=DIRECTION('center_axis',(-1.2303003375722E-16,1.,-5.10212787052002E-17)) ;
#88972=DIRECTION('ref_axis',(-1.,-1.2303003375722E-16,6.27714964143733E-33)) ;
#88973=DIRECTION('center_axis',(-8.67361737988403E-15,-1.,0.)) ;
#88974=DIRECTION('ref_axis',(1.,-8.67361737988403E-15,0.)) ;
#88975=DIRECTION('center_axis',(1.,0.,6.27714964143733E-33)) ;
#88976=DIRECTION('ref_axis',(6.27714964143733E-33,0.,-1.)) ;
#88977=DIRECTION('center_axis',(-1.,0.,-6.5052130349128E-15)) ;
#88978=DIRECTION('ref_axis',(-6.5052130349128E-15,0.,1.)) ;
#88979=DIRECTION('center_axis',(1.,0.,0.)) ;
#88980=DIRECTION('ref_axis',(0.,1.,0.)) ;
#88981=DIRECTION('center_axis',(0.,1.,0.)) ;
#88982=DIRECTION('ref_axis',(1.,0.,0.)) ;
#88983=DIRECTION('center_axis',(1.,0.,0.)) ;
#88984=DIRECTION('ref_axis',(0.,0.,-1.)) ;
#88985=DIRECTION('center_axis',(0.,-1.,0.)) ;
#88986=DIRECTION('ref_axis',(0.,0.,-1.)) ;
#88987=DIRECTION('center_axis',(0.,1.,0.)) ;
#88988=DIRECTION('ref_axis',(0.,0.,1.)) ;
#88989=DIRECTION('center_axis',(0.,-1.,0.)) ;
#88990=DIRECTION('ref_axis',(0.,0.,-1.)) ;
#88991=DIRECTION('center_axis',(1.,0.,0.)) ;
#88992=DIRECTION('ref_axis',(0.,0.,-1.)) ;
#88993=DIRECTION('center_axis',(1.,0.,0.)) ;
#88994=DIRECTION('ref_axis',(0.,0.,-1.)) ;
#88995=DIRECTION('center_axis',(0.,0.,1.)) ;
#88996=DIRECTION('ref_axis',(1.,0.,0.)) ;
#88997=DIRECTION('center_axis',(-1.,8.67361737988401E-15,-8.67361737988379E-15)) ;
#88998=DIRECTION('ref_axis',(-8.67361737988401E-15,-1.,1.07724819444908E-44)) ;
#88999=DIRECTION('center_axis',(0.,1.,0.)) ;
#89000=DIRECTION('ref_axis',(1.,0.,0.)) ;
#89001=DIRECTION('center_axis',(0.,-1.,0.)) ;
#89002=DIRECTION('ref_axis',(0.,0.,-1.)) ;
#89003=DIRECTION('center_axis',(1.,1.59148942750166E-16,0.)) ;
#89004=DIRECTION('ref_axis',(-1.59148942750166E-16,1.,0.)) ;
#89005=DIRECTION('center_axis',(-1.,0.,6.50521303491284E-15)) ;
#89006=DIRECTION('ref_axis',(6.50521303491284E-15,0.,1.)) ;
#89007=DIRECTION('center_axis',(-4.33680868994203E-15,-1.,0.)) ;
#89008=DIRECTION('ref_axis',(1.,-4.33680868994203E-15,0.)) ;
#89009=DIRECTION('center_axis',(-8.67361737988401E-15,-1.,0.)) ;
#89010=DIRECTION('ref_axis',(1.,-8.67361737988401E-15,0.)) ;
#89011=DIRECTION('center_axis',(0.,1.,0.)) ;
#89012=DIRECTION('ref_axis',(1.,0.,0.)) ;
#89013=DIRECTION('center_axis',(8.67361737988403E-15,-1.,0.)) ;
#89014=DIRECTION('ref_axis',(1.,8.67361737988403E-15,0.)) ;
#89015=DIRECTION('center_axis',(0.,0.,1.)) ;
#89016=DIRECTION('ref_axis',(1.,0.,0.)) ;
#89017=DIRECTION('center_axis',(1.,8.67361737988401E-15,0.)) ;
#89018=DIRECTION('ref_axis',(-8.67361737988401E-15,1.,0.)) ;
#89019=DIRECTION('center_axis',(-1.2303003375722E-16,1.,0.)) ;
#89020=DIRECTION('ref_axis',(-1.,-1.2303003375722E-16,0.)) ;
#89021=DIRECTION('center_axis',(0.,-1.,8.67361737988379E-15)) ;
#89022=DIRECTION('ref_axis',(0.,-8.67361737988379E-15,-1.)) ;
#89023=DIRECTION('center_axis',(1.,-5.88041856263325E-16,0.)) ;
#89024=DIRECTION('ref_axis',(5.88041856263325E-16,1.,0.)) ;
#89025=DIRECTION('center_axis',(1.,0.,0.)) ;
#89026=DIRECTION('ref_axis',(0.,0.,-1.)) ;
#89027=DIRECTION('center_axis',(0.,1.,0.)) ;
#89028=DIRECTION('ref_axis',(1.,0.,0.)) ;
#89029=DIRECTION('center_axis',(1.,6.50521303491304E-15,0.)) ;
#89030=DIRECTION('ref_axis',(-6.50521303491304E-15,1.,0.)) ;
#89031=DIRECTION('center_axis',(0.,1.,0.)) ;
#89032=DIRECTION('ref_axis',(1.,0.,0.)) ;
#89033=DIRECTION('center_axis',(0.,-1.,0.)) ;
#89034=DIRECTION('ref_axis',(0.,0.,-1.)) ;
#89035=DIRECTION('center_axis',(-1.,0.,0.)) ;
#89036=DIRECTION('ref_axis',(0.,0.,1.)) ;
#89037=DIRECTION('center_axis',(1.,0.,1.73472347597676E-14)) ;
#89038=DIRECTION('ref_axis',(1.73472347597676E-14,0.,-1.)) ;
#89039=DIRECTION('center_axis',(0.,-1.,0.)) ;
#89040=DIRECTION('ref_axis',(0.,0.,-1.)) ;
#89041=DIRECTION('center_axis',(8.67361737988409E-15,-1.,0.)) ;
#89042=DIRECTION('ref_axis',(1.,8.67361737988409E-15,0.)) ;
#89043=DIRECTION('center_axis',(0.,1.,0.)) ;
#89044=DIRECTION('ref_axis',(1.,0.,0.)) ;
#89045=DIRECTION('center_axis',(0.,1.,0.)) ;
#89046=DIRECTION('ref_axis',(1.,0.,0.)) ;
#89047=DIRECTION('center_axis',(1.,0.,0.)) ;
#89048=DIRECTION('ref_axis',(0.,0.,-1.)) ;
#89049=DIRECTION('center_axis',(0.,-1.,0.)) ;
#89050=DIRECTION('ref_axis',(0.,0.,-1.)) ;
#89051=DIRECTION('center_axis',(0.,-1.,0.)) ;
#89052=DIRECTION('ref_axis',(0.,0.,-1.)) ;
#89053=DIRECTION('center_axis',(0.,-1.,0.)) ;
#89054=DIRECTION('ref_axis',(0.,0.,-1.)) ;
#89055=DIRECTION('center_axis',(-1.,0.,0.)) ;
#89056=DIRECTION('ref_axis',(0.,0.,1.)) ;
#89057=DIRECTION('center_axis',(1.,0.,0.)) ;
#89058=DIRECTION('ref_axis',(0.,0.,-1.)) ;
#89059=DIRECTION('center_axis',(0.,0.,1.)) ;
#89060=DIRECTION('ref_axis',(1.,0.,0.)) ;
#89061=DIRECTION('center_axis',(-1.,0.,0.)) ;
#89062=DIRECTION('ref_axis',(0.,0.,1.)) ;
#89063=DIRECTION('center_axis',(0.,1.,0.)) ;
#89064=DIRECTION('ref_axis',(1.,0.,0.)) ;
#89065=DIRECTION('center_axis',(0.,-1.,0.)) ;
#89066=DIRECTION('ref_axis',(0.,0.,-1.)) ;
#89067=DIRECTION('center_axis',(-1.,-1.59148942750166E-16,0.)) ;
#89068=DIRECTION('ref_axis',(1.59148942750166E-16,-1.,0.)) ;
#89069=DIRECTION('center_axis',(-1.,6.50521303491307E-15,0.)) ;
#89070=DIRECTION('ref_axis',(-6.50521303491307E-15,-1.,0.)) ;
#89071=DIRECTION('center_axis',(4.33680868994203E-15,1.,0.)) ;
#89072=DIRECTION('ref_axis',(-1.,4.33680868994203E-15,0.)) ;
#89073=DIRECTION('center_axis',(-8.67361737988401E-15,-1.,0.)) ;
#89074=DIRECTION('ref_axis',(1.,-8.67361737988401E-15,0.)) ;
#89075=DIRECTION('center_axis',(0.,1.,0.)) ;
#89076=DIRECTION('ref_axis',(1.,0.,0.)) ;
#89077=DIRECTION('center_axis',(8.67361737988403E-15,-1.,0.)) ;
#89078=DIRECTION('ref_axis',(1.,8.67361737988403E-15,0.)) ;
#89079=DIRECTION('center_axis',(0.,0.,1.)) ;
#89080=DIRECTION('ref_axis',(1.,0.,0.)) ;
#89081=DIRECTION('center_axis',(1.,8.67361737988401E-15,0.)) ;
#89082=DIRECTION('ref_axis',(-8.67361737988401E-15,1.,0.)) ;
#89083=DIRECTION('center_axis',(1.2303003375722E-16,-1.,0.)) ;
#89084=DIRECTION('ref_axis',(1.,1.2303003375722E-16,0.)) ;
#89085=DIRECTION('center_axis',(-8.67361737988416E-15,-1.,0.)) ;
#89086=DIRECTION('ref_axis',(1.,-8.67361737988416E-15,0.)) ;
#89087=DIRECTION('center_axis',(-1.,5.88041856263325E-16,0.)) ;
#89088=DIRECTION('ref_axis',(-5.88041856263325E-16,-1.,0.)) ;
#89089=DIRECTION('center_axis',(1.,0.,0.)) ;
#89090=DIRECTION('ref_axis',(0.,0.,-1.)) ;
#89091=DIRECTION('center_axis',(0.,1.,0.)) ;
#89092=DIRECTION('ref_axis',(1.,0.,0.)) ;
#89093=DIRECTION('center_axis',(1.,6.50521303491304E-15,0.)) ;
#89094=DIRECTION('ref_axis',(-6.50521303491304E-15,1.,0.)) ;
#89095=DIRECTION('center_axis',(0.,1.,0.)) ;
#89096=DIRECTION('ref_axis',(1.,0.,0.)) ;
#89097=DIRECTION('center_axis',(0.,-1.,0.)) ;
#89098=DIRECTION('ref_axis',(0.,0.,-1.)) ;
#89099=DIRECTION('center_axis',(1.,0.,0.)) ;
#89100=DIRECTION('ref_axis',(0.,0.,-1.)) ;
#89101=DIRECTION('center_axis',(1.,-1.73472347597681E-14,0.)) ;
#89102=DIRECTION('ref_axis',(1.73472347597681E-14,1.,0.)) ;
#89103=DIRECTION('center_axis',(0.,1.,0.)) ;
#89104=DIRECTION('ref_axis',(0.,0.,1.)) ;
#89105=DIRECTION('center_axis',(0.,-1.,-8.67361737988405E-15)) ;
#89106=DIRECTION('ref_axis',(0.,8.67361737988405E-15,-1.)) ;
#89107=DIRECTION('center_axis',(0.,1.,0.)) ;
#89108=DIRECTION('ref_axis',(1.,0.,0.)) ;
#89109=DIRECTION('center_axis',(0.,0.,-1.)) ;
#89110=DIRECTION('ref_axis',(-1.,0.,0.)) ;
#89111=DIRECTION('center_axis',(0.,0.,1.)) ;
#89112=DIRECTION('ref_axis',(1.,0.,0.)) ;
#89113=DIRECTION('center_axis',(0.,0.,-1.)) ;
#89114=DIRECTION('ref_axis',(-1.,0.,0.)) ;
#89115=DIRECTION('center_axis',(-1.,0.,0.)) ;
#89116=DIRECTION('ref_axis',(0.,0.,1.)) ;
#89117=DIRECTION('center_axis',(0.,-1.,0.)) ;
#89118=DIRECTION('ref_axis',(0.,0.,-1.)) ;
#89119=DIRECTION('center_axis',(0.,1.,0.)) ;
#89120=DIRECTION('ref_axis',(0.,0.,1.)) ;
#89121=DIRECTION('center_axis',(0.,1.,-6.50521303491302E-15)) ;
#89122=DIRECTION('ref_axis',(0.,6.50521303491302E-15,1.)) ;
#89123=DIRECTION('center_axis',(0.,-1.,0.)) ;
#89124=DIRECTION('ref_axis',(0.,0.,-1.)) ;
#89125=DIRECTION('center_axis',(0.,-1.,0.)) ;
#89126=DIRECTION('ref_axis',(0.,0.,-1.)) ;
#89127=DIRECTION('center_axis',(0.,-1.,-1.07081696047951E-16)) ;
#89128=DIRECTION('ref_axis',(0.,1.07081696047951E-16,-1.)) ;
#89129=DIRECTION('center_axis',(0.,1.,0.)) ;
#89130=DIRECTION('ref_axis',(0.,0.,1.)) ;
#89131=DIRECTION('center_axis',(-1.,0.,0.)) ;
#89132=DIRECTION('ref_axis',(0.,0.,1.)) ;
#89133=DIRECTION('center_axis',(0.,0.,1.)) ;
#89134=DIRECTION('ref_axis',(1.,0.,0.)) ;
#89135=DIRECTION('center_axis',(0.,1.,0.)) ;
#89136=DIRECTION('ref_axis',(0.,0.,1.)) ;
#89137=DIRECTION('center_axis',(0.,-6.50521303491304E-15,-1.)) ;
#89138=DIRECTION('ref_axis',(0.,1.,-6.50521303491304E-15)) ;
#89139=DIRECTION('center_axis',(0.,0.,1.)) ;
#89140=DIRECTION('ref_axis',(1.,0.,0.)) ;
#89141=DIRECTION('center_axis',(0.,-1.08420217248551E-15,1.)) ;
#89142=DIRECTION('ref_axis',(0.,-1.,-1.08420217248551E-15)) ;
#89143=DIRECTION('center_axis',(0.,0.,1.)) ;
#89144=DIRECTION('ref_axis',(1.,0.,0.)) ;
#89145=DIRECTION('center_axis',(0.,0.,-1.)) ;
#89146=DIRECTION('ref_axis',(-1.,0.,0.)) ;
#89147=DIRECTION('center_axis',(0.,1.,0.)) ;
#89148=DIRECTION('ref_axis',(0.,0.,1.)) ;
#89149=DIRECTION('center_axis',(0.,-0.707106781186548,0.707106781186547)) ;
#89150=DIRECTION('ref_axis',(0.,-0.707106781186547,-0.707106781186548)) ;
#89151=DIRECTION('center_axis',(0.,1.,0.)) ;
#89152=DIRECTION('ref_axis',(0.,0.,1.)) ;
#89153=DIRECTION('center_axis',(0.,-0.5142317969591,-0.857651245551602)) ;
#89154=DIRECTION('ref_axis',(0.,0.857651245551602,-0.5142317969591)) ;
#89155=DIRECTION('center_axis',(0.,-0.707106781186548,0.707106781186547)) ;
#89156=DIRECTION('ref_axis',(0.,-0.707106781186547,-0.707106781186548)) ;
#89157=DIRECTION('center_axis',(0.,-0.70710678118655,0.707106781186545)) ;
#89158=DIRECTION('ref_axis',(0.,-0.707106781186545,-0.70710678118655)) ;
#89159=DIRECTION('center_axis',(-1.,0.,0.)) ;
#89160=DIRECTION('ref_axis',(0.,0.,1.)) ;
#89161=DIRECTION('center_axis',(0.,0.514231796959101,-0.857651245551602)) ;
#89162=DIRECTION('ref_axis',(0.,0.857651245551602,0.514231796959101)) ;
#89163=DIRECTION('center_axis',(0.,1.,0.)) ;
#89164=DIRECTION('ref_axis',(0.,0.,1.)) ;
#89165=DIRECTION('center_axis',(0.,0.,-1.)) ;
#89166=DIRECTION('ref_axis',(-1.,0.,0.)) ;
#89167=DIRECTION('center_axis',(0.,1.,0.)) ;
#89168=DIRECTION('ref_axis',(0.,0.,1.)) ;
#89169=DIRECTION('center_axis',(0.,0.,-1.)) ;
#89170=DIRECTION('ref_axis',(-1.,0.,0.)) ;
#89171=DIRECTION('center_axis',(0.,0.,-1.)) ;
#89172=DIRECTION('ref_axis',(-1.,0.,0.)) ;
#89173=DIRECTION('center_axis',(0.,0.,1.)) ;
#89174=DIRECTION('ref_axis',(1.,0.,0.)) ;
#89175=DIRECTION('center_axis',(0.,0.,-1.)) ;
#89176=DIRECTION('ref_axis',(-1.,0.,0.)) ;
#89177=DIRECTION('center_axis',(0.,1.,0.)) ;
#89178=DIRECTION('ref_axis',(0.,0.,1.)) ;
#89179=DIRECTION('center_axis',(0.,-1.,8.67361737988403E-15)) ;
#89180=DIRECTION('ref_axis',(0.,-8.67361737988403E-15,-1.)) ;
#89181=DIRECTION('center_axis',(0.,0.707106781186546,0.707106781186549)) ;
#89182=DIRECTION('ref_axis',(0.,-0.707106781186549,0.707106781186546)) ;
#89183=DIRECTION('center_axis',(0.,0.707106781186547,0.707106781186548)) ;
#89184=DIRECTION('ref_axis',(0.,-0.707106781186548,0.707106781186547)) ;
#89185=DIRECTION('center_axis',(0.,1.,1.07081696047951E-16)) ;
#89186=DIRECTION('ref_axis',(0.,-1.07081696047951E-16,1.)) ;
#89187=DIRECTION('center_axis',(0.,-1.,0.)) ;
#89188=DIRECTION('ref_axis',(0.,0.,-1.)) ;
#89189=DIRECTION('center_axis',(0.,1.,0.)) ;
#89190=DIRECTION('ref_axis',(0.,0.,1.)) ;
#89191=DIRECTION('center_axis',(0.,-1.08420217248551E-15,1.)) ;
#89192=DIRECTION('ref_axis',(0.,-1.,-1.08420217248551E-15)) ;
#89193=DIRECTION('center_axis',(0.,1.,0.)) ;
#89194=DIRECTION('ref_axis',(0.,0.,1.)) ;
#89195=DIRECTION('center_axis',(0.,6.50521303491302E-15,1.)) ;
#89196=DIRECTION('ref_axis',(0.,-1.,6.50521303491302E-15)) ;
#89197=DIRECTION('center_axis',(0.,3.99416362155027E-15,1.)) ;
#89198=DIRECTION('ref_axis',(0.,-1.,3.99416362155027E-15)) ;
#89199=DIRECTION('center_axis',(0.,0.,1.)) ;
#89200=DIRECTION('ref_axis',(1.,0.,0.)) ;
#89201=DIRECTION('center_axis',(0.,0.,-1.)) ;
#89202=DIRECTION('ref_axis',(-1.,0.,0.)) ;
#89203=DIRECTION('center_axis',(0.,0.,1.)) ;
#89204=DIRECTION('ref_axis',(1.,0.,0.)) ;
#89205=DIRECTION('center_axis',(-1.,0.,0.)) ;
#89206=DIRECTION('ref_axis',(0.,0.,1.)) ;
#89207=DIRECTION('center_axis',(0.,1.,0.)) ;
#89208=DIRECTION('ref_axis',(0.,0.,1.)) ;
#89209=DIRECTION('center_axis',(-1.,0.,0.)) ;
#89210=DIRECTION('ref_axis',(0.,0.,1.)) ;
#89211=DIRECTION('center_axis',(0.,-1.,0.)) ;
#89212=DIRECTION('ref_axis',(0.,0.,-1.)) ;
#89213=DIRECTION('center_axis',(0.,1.,0.)) ;
#89214=DIRECTION('ref_axis',(0.,0.,1.)) ;
#89215=DIRECTION('center_axis',(0.,-1.,0.)) ;
#89216=DIRECTION('ref_axis',(0.,0.,-1.)) ;
#89217=DIRECTION('center_axis',(0.,1.,0.)) ;
#89218=DIRECTION('ref_axis',(0.,0.,1.)) ;
#89219=DIRECTION('center_axis',(0.,-1.,0.)) ;
#89220=DIRECTION('ref_axis',(0.,0.,-1.)) ;
#89221=DIRECTION('center_axis',(0.,1.,0.)) ;
#89222=DIRECTION('ref_axis',(0.,0.,-1.)) ;
#89223=DIRECTION('center_axis',(-4.70197740328919E-30,-1.08420217248551E-15,
-1.)) ;
#89224=DIRECTION('ref_axis',(6.22301527786114E-61,1.,-1.08420217248551E-15)) ;
#89225=DIRECTION('center_axis',(0.,1.,0.)) ;
#89226=DIRECTION('ref_axis',(0.,0.,-1.)) ;
#89227=DIRECTION('center_axis',(0.,0.,-1.)) ;
#89228=DIRECTION('ref_axis',(-1.,0.,0.)) ;
#89229=DIRECTION('center_axis',(0.,0.,1.)) ;
#89230=DIRECTION('ref_axis',(1.,0.,0.)) ;
#89231=DIRECTION('center_axis',(0.,0.,-1.)) ;
#89232=DIRECTION('ref_axis',(-1.,0.,0.)) ;
#89233=DIRECTION('center_axis',(0.,0.,-1.)) ;
#89234=DIRECTION('ref_axis',(-1.,0.,0.)) ;
#89235=DIRECTION('center_axis',(0.,6.50521303491304E-15,-1.)) ;
#89236=DIRECTION('ref_axis',(0.,1.,6.50521303491304E-15)) ;
#89237=DIRECTION('center_axis',(1.,0.,0.)) ;
#89238=DIRECTION('ref_axis',(0.,0.,-1.)) ;
#89239=DIRECTION('center_axis',(0.,0.707106781186548,-0.707106781186548)) ;
#89240=DIRECTION('ref_axis',(0.,0.707106781186548,0.707106781186548)) ;
#89241=DIRECTION('center_axis',(1.,0.,0.)) ;
#89242=DIRECTION('ref_axis',(0.,0.,-1.)) ;
#89243=DIRECTION('center_axis',(0.,-1.,0.)) ;
#89244=DIRECTION('ref_axis',(0.,0.,-1.)) ;
#89245=DIRECTION('center_axis',(0.,-0.707106781186548,0.707106781186547)) ;
#89246=DIRECTION('ref_axis',(0.,-0.707106781186547,-0.707106781186548)) ;
#89247=DIRECTION('center_axis',(0.,-1.,-1.07081696047951E-16)) ;
#89248=DIRECTION('ref_axis',(0.,1.07081696047951E-16,-1.)) ;
#89249=DIRECTION('center_axis',(0.,-1.,-8.67361737988403E-15)) ;
#89250=DIRECTION('ref_axis',(0.,8.67361737988403E-15,-1.)) ;
#89251=DIRECTION('center_axis',(1.,0.,0.)) ;
#89252=DIRECTION('ref_axis',(0.,0.,-1.)) ;
#89253=DIRECTION('center_axis',(0.,0.,1.)) ;
#89254=DIRECTION('ref_axis',(1.,0.,0.)) ;
#89255=DIRECTION('center_axis',(0.,0.,-1.)) ;
#89256=DIRECTION('ref_axis',(-1.,0.,0.)) ;
#89257=DIRECTION('center_axis',(0.,0.,1.)) ;
#89258=DIRECTION('ref_axis',(1.,0.,0.)) ;
#89259=DIRECTION('center_axis',(0.,0.,1.)) ;
#89260=DIRECTION('ref_axis',(1.,0.,0.)) ;
#89261=DIRECTION('center_axis',(0.,0.,1.)) ;
#89262=DIRECTION('ref_axis',(1.,0.,0.)) ;
#89263=DIRECTION('center_axis',(1.,0.,0.)) ;
#89264=DIRECTION('ref_axis',(0.,0.382683432365091,0.923879532511286)) ;
#89265=DIRECTION('center_axis',(0.,-0.707106781186551,-0.707106781186544)) ;
#89266=DIRECTION('ref_axis',(0.,0.707106781186544,-0.707106781186551)) ;
#89267=DIRECTION('center_axis',(1.,0.,0.)) ;
#89268=DIRECTION('ref_axis',(0.,0.,-1.)) ;
#89269=DIRECTION('center_axis',(0.,0.5142317969591,0.857651245551602)) ;
#89270=DIRECTION('ref_axis',(0.,-0.857651245551602,0.5142317969591)) ;
#89271=DIRECTION('center_axis',(0.,0.707106781186546,0.707106781186549)) ;
#89272=DIRECTION('ref_axis',(0.,-0.707106781186549,0.707106781186546)) ;
#89273=DIRECTION('center_axis',(0.,-0.707106781186546,-0.707106781186549)) ;
#89274=DIRECTION('ref_axis',(0.,0.707106781186549,-0.707106781186546)) ;
#89275=DIRECTION('center_axis',(1.,0.,0.)) ;
#89276=DIRECTION('ref_axis',(0.,0.,-1.)) ;
#89277=DIRECTION('center_axis',(0.,-0.514231796959099,0.857651245551603)) ;
#89278=DIRECTION('ref_axis',(0.,-0.857651245551603,-0.514231796959099)) ;
#89279=DIRECTION('center_axis',(1.,0.,0.)) ;
#89280=DIRECTION('ref_axis',(0.,0.,-1.)) ;
#89281=DIRECTION('center_axis',(0.,1.08420217248551E-15,-1.)) ;
#89282=DIRECTION('ref_axis',(0.,1.,1.08420217248551E-15)) ;
#89283=DIRECTION('center_axis',(1.,0.,0.)) ;
#89284=DIRECTION('ref_axis',(0.,0.,-1.)) ;
#89285=DIRECTION('center_axis',(0.,0.,1.)) ;
#89286=DIRECTION('ref_axis',(1.,0.,0.)) ;
#89287=DIRECTION('center_axis',(0.,3.99416362155027E-15,1.)) ;
#89288=DIRECTION('ref_axis',(0.,-1.,3.99416362155027E-15)) ;
#89289=DIRECTION('center_axis',(0.,-4.33680868994202E-15,-1.)) ;
#89290=DIRECTION('ref_axis',(0.,1.,-4.33680868994202E-15)) ;
#89291=DIRECTION('center_axis',(0.,0.,1.)) ;
#89292=DIRECTION('ref_axis',(1.,0.,0.)) ;
#89293=DIRECTION('center_axis',(0.,-6.50521303491304E-15,1.)) ;
#89294=DIRECTION('ref_axis',(0.,-1.,-6.50521303491304E-15)) ;
#89295=DIRECTION('center_axis',(0.,1.,0.)) ;
#89296=DIRECTION('ref_axis',(0.,0.,-1.)) ;
#89297=DIRECTION('center_axis',(0.,-1.,0.)) ;
#89298=DIRECTION('ref_axis',(0.,0.,-1.)) ;
#89299=DIRECTION('center_axis',(1.,0.,0.)) ;
#89300=DIRECTION('ref_axis',(0.,0.,-1.)) ;
#89301=DIRECTION('center_axis',(0.,1.,0.)) ;
#89302=DIRECTION('ref_axis',(0.,0.,1.)) ;
#89303=DIRECTION('center_axis',(0.,1.,0.)) ;
#89304=DIRECTION('ref_axis',(0.,0.,1.)) ;
#89305=DIRECTION('center_axis',(0.,-1.,0.)) ;
#89306=DIRECTION('ref_axis',(0.,0.,-1.)) ;
#89307=DIRECTION('center_axis',(0.,1.,1.07081696047951E-16)) ;
#89308=DIRECTION('ref_axis',(0.,-1.07081696047951E-16,1.)) ;
#89309=DIRECTION('center_axis',(0.,1.,6.50521303491302E-15)) ;
#89310=DIRECTION('ref_axis',(0.,-6.50521303491302E-15,1.)) ;
#89311=DIRECTION('center_axis',(0.,1.,0.)) ;
#89312=DIRECTION('ref_axis',(0.,0.,-1.)) ;
#89313=DIRECTION('center_axis',(0.,0.,1.)) ;
#89314=DIRECTION('ref_axis',(1.,0.,0.)) ;
#89315=DIRECTION('center_axis',(1.,0.,0.)) ;
#89316=DIRECTION('ref_axis',(0.,0.,-1.)) ;
#89317=DIRECTION('center_axis',(0.,0.,-1.)) ;
#89318=DIRECTION('ref_axis',(-1.,0.,0.)) ;
#89319=DIRECTION('center_axis',(0.,0.,-1.)) ;
#89320=DIRECTION('ref_axis',(-1.,0.,0.)) ;
#89321=DIRECTION('center_axis',(1.,-9.85638338623186E-18,0.)) ;
#89322=DIRECTION('ref_axis',(9.85638338623186E-18,1.,0.)) ;
#89323=DIRECTION('',(0.,0.,-1.)) ;
#89324=DIRECTION('',(-9.85638338623186E-18,-1.,0.)) ;
#89325=DIRECTION('',(0.,0.,1.)) ;
#89326=DIRECTION('',(9.85638338623186E-18,1.,0.)) ;
#89327=DIRECTION('center_axis',(0.707106781186548,0.707106781186548,0.)) ;
#89328=DIRECTION('ref_axis',(-0.707106781186548,0.707106781186548,0.)) ;
#89329=DIRECTION('',(0.,0.,1.)) ;
#89330=DIRECTION('',(-0.577350269189625,0.577350269189625,0.577350269189627)) ;
#89331=DIRECTION('',(0.,0.,-1.)) ;
#89332=DIRECTION('',(0.577350269189625,-0.577350269189625,0.577350269189627)) ;
#89333=DIRECTION('center_axis',(0.,1.,0.)) ;
#89334=DIRECTION('ref_axis',(0.,0.,1.)) ;
#89335=DIRECTION('',(0.,0.,1.)) ;
#89336=DIRECTION('',(-1.,0.,-9.8563833862319E-18)) ;
#89337=DIRECTION('',(0.,0.,-1.)) ;
#89338=DIRECTION('',(1.,0.,-9.8563833862319E-18)) ;
#89339=DIRECTION('center_axis',(-0.707106781186548,0.707106781186548,0.)) ;
#89340=DIRECTION('ref_axis',(-0.707106781186548,-0.707106781186548,0.)) ;
#89341=DIRECTION('',(0.,0.,1.)) ;
#89342=DIRECTION('',(-0.577350269189625,-0.577350269189625,-0.577350269189627)) ;
#89343=DIRECTION('',(0.,0.,-1.)) ;
#89344=DIRECTION('',(0.577350269189625,0.577350269189625,-0.577350269189627)) ;
#89345=DIRECTION('center_axis',(-1.,9.85638338623186E-18,0.)) ;
#89346=DIRECTION('ref_axis',(-9.85638338623186E-18,-1.,0.)) ;
#89347=DIRECTION('',(0.,0.,-1.)) ;
#89348=DIRECTION('',(9.85638338623186E-18,1.,0.)) ;
#89349=DIRECTION('',(0.,0.,-1.)) ;
#89350=DIRECTION('',(-9.85638338623186E-18,-1.,0.)) ;
#89351=DIRECTION('center_axis',(0.,0.,1.)) ;
#89352=DIRECTION('ref_axis',(1.,0.,0.)) ;
#89353=DIRECTION('',(9.85638338623186E-18,1.,0.)) ;
#89354=DIRECTION('center_axis',(0.,0.,-1.)) ;
#89355=DIRECTION('ref_axis',(1.,0.,0.)) ;
#89356=DIRECTION('center_axis',(0.,0.,1.)) ;
#89357=DIRECTION('ref_axis',(1.,0.,0.)) ;
#89358=DIRECTION('',(-9.85638338623186E-18,-1.,0.)) ;
#89359=DIRECTION('',(1.,-9.85638338623186E-18,0.)) ;
#89360=DIRECTION('center_axis',(0.,0.,1.)) ;
#89361=DIRECTION('ref_axis',(1.,0.,0.)) ;
#89362=DIRECTION('',(9.85638338623186E-18,1.,0.)) ;
#89363=DIRECTION('center_axis',(0.,0.,-1.)) ;
#89364=DIRECTION('ref_axis',(1.,0.,0.)) ;
#89365=DIRECTION('center_axis',(0.,0.,1.)) ;
#89366=DIRECTION('ref_axis',(1.,0.,0.)) ;
#89367=DIRECTION('',(-9.85638338623186E-18,-1.,0.)) ;
#89368=DIRECTION('',(-1.,9.85638338623186E-18,0.)) ;
#89369=DIRECTION('center_axis',(0.,0.,-1.)) ;
#89370=DIRECTION('ref_axis',(-1.,0.,0.)) ;
#89371=DIRECTION('center_axis',(0.,0.,1.)) ;
#89372=DIRECTION('ref_axis',(1.,0.,0.)) ;
#89373=DIRECTION('center_axis',(0.,0.,-1.)) ;
#89374=DIRECTION('ref_axis',(1.,0.,0.)) ;
#89375=DIRECTION('center_axis',(0.,0.,-1.)) ;
#89376=DIRECTION('ref_axis',(-1.,0.,0.)) ;
#89377=DIRECTION('center_axis',(0.,0.,-1.)) ;
#89378=DIRECTION('ref_axis',(1.,0.,0.)) ;
#89379=DIRECTION('center_axis',(0.,0.,1.)) ;
#89380=DIRECTION('ref_axis',(1.,0.,0.)) ;
#89381=DIRECTION('center_axis',(-0.707106781186548,-0.707106781186547,0.)) ;
#89382=DIRECTION('ref_axis',(0.707106781186547,-0.707106781186548,0.)) ;
#89383=DIRECTION('',(0.,0.,1.)) ;
#89384=DIRECTION('',(0.577350269189625,-0.577350269189626,-0.577350269189626)) ;
#89385=DIRECTION('',(0.,0.,-1.)) ;
#89386=DIRECTION('',(-0.577350269189625,0.577350269189626,-0.577350269189626)) ;
#89387=DIRECTION('center_axis',(1.95511867169517E-16,-1.,0.)) ;
#89388=DIRECTION('ref_axis',(1.,1.95511867169517E-16,0.)) ;
#89389=DIRECTION('',(0.,0.,-1.)) ;
#89390=DIRECTION('',(-1.,-1.95511867169517E-16,0.)) ;
#89391=DIRECTION('',(1.,1.95511867169517E-16,0.)) ;
#89392=DIRECTION('center_axis',(1.06642836637918E-16,1.,0.)) ;
#89393=DIRECTION('ref_axis',(-1.,1.06642836637918E-16,0.)) ;
#89394=DIRECTION('',(1.,-1.06642836637919E-16,0.)) ;
#89395=DIRECTION('',(0.,0.,1.)) ;
#89396=DIRECTION('',(-1.,1.06642836637919E-16,0.)) ;
#89397=DIRECTION('center_axis',(-0.707106781186548,0.707106781186547,0.)) ;
#89398=DIRECTION('ref_axis',(-0.707106781186547,-0.707106781186548,0.)) ;
#89399=DIRECTION('',(0.,0.,1.)) ;
#89400=DIRECTION('',(-0.577350269189625,-0.577350269189626,0.577350269189627)) ;
#89401=DIRECTION('',(0.,0.,-1.)) ;
#89402=DIRECTION('',(0.577350269189625,0.577350269189626,0.577350269189627)) ;
#89403=DIRECTION('center_axis',(-1.,0.,0.)) ;
#89404=DIRECTION('ref_axis',(0.,0.,1.)) ;
#89405=DIRECTION('',(0.,0.,-1.)) ;
#89406=DIRECTION('',(0.,1.,1.95511867169518E-16)) ;
#89407=DIRECTION('',(0.,0.,1.)) ;
#89408=DIRECTION('',(0.,-1.,1.95511867169518E-16)) ;
#89409=DIRECTION('center_axis',(0.,0.,1.)) ;
#89410=DIRECTION('ref_axis',(1.,0.,0.)) ;
#89411=DIRECTION('',(-1.95511867169517E-16,1.,0.)) ;
#89412=DIRECTION('',(-1.,-1.95511867169517E-16,0.)) ;
#89413=DIRECTION('',(1.,-1.06642836637919E-16,0.)) ;
#89414=DIRECTION('center_axis',(0.,0.,1.)) ;
#89415=DIRECTION('ref_axis',(1.,0.,0.)) ;
#89416=DIRECTION('',(1.,1.95511867169517E-16,0.)) ;
#89417=DIRECTION('',(1.95511867169517E-16,-1.,0.)) ;
#89418=DIRECTION('',(-1.,1.06642836637919E-16,0.)) ;
#89419=DIRECTION('center_axis',(6.96951553037899E-18,0.707106781186549,
0.707106781186546)) ;
#89420=DIRECTION('ref_axis',(-8.6424177776148E-34,-0.707106781186546,0.707106781186549)) ;
#89421=DIRECTION('',(-0.577350269189625,0.577350269189625,-0.577350269189627)) ;
#89422=DIRECTION('',(1.,-9.85638338623186E-18,0.)) ;
#89423=DIRECTION('',(-0.577350269189625,-0.577350269189625,0.577350269189627)) ;
#89424=DIRECTION('',(-1.,7.70371977754894E-34,9.8563833862319E-18)) ;
#89425=DIRECTION('center_axis',(6.96951553037899E-18,0.707106781186549,
-0.707106781186546)) ;
#89426=DIRECTION('ref_axis',(8.6424177776148E-34,0.707106781186546,0.707106781186549)) ;
#89427=DIRECTION('',(0.577350269189625,0.577350269189625,0.577350269189627)) ;
#89428=DIRECTION('',(-1.,9.85638338623186E-18,0.)) ;
#89429=DIRECTION('',(0.577350269189625,-0.577350269189625,-0.577350269189627)) ;
#89430=DIRECTION('',(1.,-7.70371977754894E-34,9.8563833862319E-18)) ;
#89431=DIRECTION('center_axis',(-0.707106781186548,-1.38247767078009E-16,
0.707106781186547)) ;
#89432=DIRECTION('ref_axis',(0.707106781186547,8.815972061965E-34,0.707106781186548)) ;
#89433=DIRECTION('',(-0.577350269189625,-0.577350269189626,-0.577350269189626)) ;
#89434=DIRECTION('',(-1.95511867169517E-16,1.,0.)) ;
#89435=DIRECTION('',(0.577350269189625,-0.577350269189626,0.577350269189626)) ;
#89436=DIRECTION('',(0.,-1.,-1.95511867169518E-16)) ;
#89437=DIRECTION('center_axis',(-0.707106781186548,-1.38247767078009E-16,
-0.707106781186547)) ;
#89438=DIRECTION('ref_axis',(-0.707106781186547,-8.815972061965E-34,0.707106781186548)) ;
#89439=DIRECTION('',(-0.577350269189625,0.577350269189626,0.577350269189626)) ;
#89440=DIRECTION('',(1.95511867169517E-16,-1.,0.)) ;
#89441=DIRECTION('',(0.577350269189625,0.577350269189626,-0.577350269189626)) ;
#89442=DIRECTION('',(0.,1.,-1.95511867169518E-16)) ;
#89443=DIRECTION('center_axis',(0.577350269189625,0.577350269189625,-0.577350269189628)) ;
#89444=DIRECTION('ref_axis',(-0.707106781186549,-3.37019869349033E-16,-0.707106781186546)) ;
#89445=DIRECTION('center_axis',(-0.577350269189625,-0.577350269189625,0.577350269189628)) ;
#89446=DIRECTION('ref_axis',(-0.707106781186549,-5.7623968423712E-16,-0.707106781186546)) ;
#89447=DIRECTION('center_axis',(-0.577350269189625,-0.577350269189625,0.577350269189627)) ;
#89448=DIRECTION('ref_axis',(0.707106781186549,-3.64954285315842E-16,0.707106781186546)) ;
#89449=DIRECTION('center_axis',(0.,0.,-1.)) ;
#89450=DIRECTION('ref_axis',(-1.,0.,0.)) ;
#89451=DIRECTION('center_axis',(0.,0.,1.)) ;
#89452=DIRECTION('ref_axis',(-1.,0.,0.)) ;
#89453=DIRECTION('center_axis',(0.,0.,-1.)) ;
#89454=DIRECTION('ref_axis',(-1.,0.,0.)) ;
#89455=DIRECTION('center_axis',(2.08166817117218E-16,1.,0.)) ;
#89456=DIRECTION('ref_axis',(1.,0.,0.)) ;
#89457=DIRECTION('center_axis',(-1.,0.,-3.25824851045218E-15)) ;
#89458=DIRECTION('ref_axis',(3.25824851045218E-15,0.,-1.)) ;
#89459=DIRECTION('center_axis',(2.71050543121376E-15,2.71050543121375E-15,
1.)) ;
#89460=DIRECTION('ref_axis',(-1.,-1.07215069759461E-44,2.71050543121376E-15)) ;
#89461=DIRECTION('center_axis',(-0.577350269189625,-0.577350269189625,-0.577350269189628)) ;
#89462=DIRECTION('ref_axis',(-0.707106781186549,-3.37019869349033E-16,0.707106781186546)) ;
#89463=DIRECTION('center_axis',(-0.577350269189625,-0.577350269189625,-0.577350269189628)) ;
#89464=DIRECTION('ref_axis',(-0.707106781186549,-3.64775444964662E-16,0.707106781186546)) ;
#89465=DIRECTION('center_axis',(-0.577350269189625,-0.577350269189625,-0.577350269189628)) ;
#89466=DIRECTION('ref_axis',(-0.707106781186549,-3.37019869349033E-16,0.707106781186546)) ;
#89467=DIRECTION('center_axis',(0.,0.,-1.)) ;
#89468=DIRECTION('ref_axis',(-1.,0.,0.)) ;
#89469=DIRECTION('center_axis',(6.99565121361789E-15,0.,1.)) ;
#89470=DIRECTION('ref_axis',(1.,0.,-6.99565121361789E-15)) ;
#89471=DIRECTION('center_axis',(-1.,0.,9.8563833862319E-18)) ;
#89472=DIRECTION('ref_axis',(9.8563833862319E-18,0.,1.)) ;
#89473=DIRECTION('center_axis',(-1.,-1.62630325872825E-15,1.62630325872826E-15)) ;
#89474=DIRECTION('ref_axis',(1.62630325872826E-15,2.45227231256843E-45,
1.)) ;
#89475=DIRECTION('center_axis',(2.08166817117218E-16,1.,0.)) ;
#89476=DIRECTION('ref_axis',(1.,0.,0.)) ;
#89477=DIRECTION('center_axis',(-1.,-5.82758667710957E-15,-5.82758667710959E-15)) ;
#89478=DIRECTION('ref_axis',(5.82758667710959E-15,3.92363570010949E-44,
-1.)) ;
#89479=DIRECTION('center_axis',(2.08166817117218E-16,1.,0.)) ;
#89480=DIRECTION('ref_axis',(1.,0.,0.)) ;
#89481=DIRECTION('center_axis',(-0.577350269189626,0.577350269189625,-0.577350269189627)) ;
#89482=DIRECTION('ref_axis',(0.707106781186548,-3.45739798078984E-16,-0.707106781186547)) ;
#89483=DIRECTION('center_axis',(-1.91661677085422E-15,0.,1.)) ;
#89484=DIRECTION('ref_axis',(-1.,0.,-1.91661677085422E-15)) ;
#89485=DIRECTION('center_axis',(-1.,0.,-9.8563833862319E-18)) ;
#89486=DIRECTION('ref_axis',(-9.8563833862319E-18,0.,1.)) ;
#89487=DIRECTION('center_axis',(-1.,0.,-2.77909431773862E-15)) ;
#89488=DIRECTION('ref_axis',(-2.77909431773862E-15,0.,1.)) ;
#89489=DIRECTION('center_axis',(0.,0.,-1.)) ;
#89490=DIRECTION('ref_axis',(-1.,0.,0.)) ;
#89491=DIRECTION('center_axis',(1.49077798716757E-15,-1.49077798716756E-15,
1.)) ;
#89492=DIRECTION('ref_axis',(1.,-2.47036158412635E-45,-1.49077798716757E-15)) ;
#89493=DIRECTION('center_axis',(0.577350269189625,-0.577350269189625,0.577350269189628)) ;
#89494=DIRECTION('ref_axis',(0.707106781186549,-3.37019869349033E-16,-0.707106781186546)) ;
#89495=DIRECTION('center_axis',(0.577350269189625,-0.577350269189625,0.577350269189628)) ;
#89496=DIRECTION('ref_axis',(0.707106781186549,-3.64775444964662E-16,-0.707106781186546)) ;
#89497=DIRECTION('center_axis',(2.08166817117218E-16,1.,0.)) ;
#89498=DIRECTION('ref_axis',(1.,0.,0.)) ;
#89499=DIRECTION('center_axis',(-0.577350269189626,0.577350269189625,0.577350269189627)) ;
#89500=DIRECTION('ref_axis',(-0.707106781186549,-1.20060139371205E-15,-0.707106781186546)) ;
#89501=DIRECTION('center_axis',(0.,0.,-1.)) ;
#89502=DIRECTION('ref_axis',(-1.,0.,0.)) ;
#89503=DIRECTION('center_axis',(0.,0.,1.)) ;
#89504=DIRECTION('ref_axis',(-1.,0.,0.)) ;
#89505=DIRECTION('center_axis',(0.,0.,-1.)) ;
#89506=DIRECTION('ref_axis',(-1.,0.,0.)) ;
#89507=DIRECTION('center_axis',(-0.577350269189625,0.577350269189625,0.577350269189628)) ;
#89508=DIRECTION('ref_axis',(0.707106781186549,-3.64775444964662E-16,0.707106781186546)) ;
#89509=DIRECTION('center_axis',(0.577350269189625,-0.577350269189625,-0.577350269189628)) ;
#89510=DIRECTION('ref_axis',(0.707106781186549,-4.84385352408706E-16,0.707106781186546)) ;
#89511=DIRECTION('center_axis',(-0.577350269189625,0.577350269189626,-0.577350269189626)) ;
#89512=DIRECTION('ref_axis',(5.0289788758123E-16,0.707106781186548,0.707106781186547)) ;
#89513=DIRECTION('center_axis',(0.577350269189625,-0.577350269189626,0.577350269189626)) ;
#89514=DIRECTION('ref_axis',(5.0289788758123E-16,0.707106781186548,0.707106781186547)) ;
#89515=DIRECTION('center_axis',(0.577350269189625,-0.577350269189627,0.577350269189626)) ;
#89516=DIRECTION('ref_axis',(-1.3856936129729E-16,-0.707106781186547,-0.707106781186548)) ;
#89517=DIRECTION('center_axis',(0.,0.,-1.)) ;
#89518=DIRECTION('ref_axis',(-1.,0.,0.)) ;
#89519=DIRECTION('center_axis',(0.,0.,1.)) ;
#89520=DIRECTION('ref_axis',(-1.,-5.42101086242751E-15,0.)) ;
#89521=DIRECTION('center_axis',(0.,0.,-1.)) ;
#89522=DIRECTION('ref_axis',(-1.,0.,0.)) ;
#89523=DIRECTION('center_axis',(0.,1.,0.)) ;
#89524=DIRECTION('ref_axis',(1.,0.,0.)) ;
#89525=DIRECTION('center_axis',(0.,-1.,-4.79154192713555E-15)) ;
#89526=DIRECTION('ref_axis',(0.,-4.79154192713555E-15,1.)) ;
#89527=DIRECTION('center_axis',(-3.18484388167616E-15,3.18484388167617E-15,
1.)) ;
#89528=DIRECTION('ref_axis',(-4.20389539297445E-45,1.,-3.18484388167617E-15)) ;
#89529=DIRECTION('center_axis',(0.577350269189625,-0.577350269189626,-0.577350269189626)) ;
#89530=DIRECTION('ref_axis',(5.0289788758123E-16,0.707106781186548,-0.707106781186547)) ;
#89531=DIRECTION('center_axis',(0.577350269189625,-0.577350269189626,-0.577350269189626)) ;
#89532=DIRECTION('ref_axis',(5.0289788758123E-16,0.707106781186548,-0.707106781186547)) ;
#89533=DIRECTION('center_axis',(0.577350269189625,-0.577350269189626,-0.577350269189626)) ;
#89534=DIRECTION('ref_axis',(5.0289788758123E-16,0.707106781186548,-0.707106781186547)) ;
#89535=DIRECTION('center_axis',(0.,0.,-1.)) ;
#89536=DIRECTION('ref_axis',(-1.,0.,0.)) ;
#89537=DIRECTION('center_axis',(0.,-2.87492515628133E-15,1.)) ;
#89538=DIRECTION('ref_axis',(0.,-1.,-2.87492515628133E-15)) ;
#89539=DIRECTION('center_axis',(0.,1.,1.95511867169518E-16)) ;
#89540=DIRECTION('ref_axis',(0.,-1.95511867169518E-16,1.)) ;
#89541=DIRECTION('center_axis',(2.71050543121375E-15,-1.,2.51884375412834E-15)) ;
#89542=DIRECTION('ref_axis',(1.,2.71050543121375E-15,2.80259692864963E-45)) ;
#89543=DIRECTION('center_axis',(0.,1.,0.)) ;
#89544=DIRECTION('ref_axis',(1.,0.,0.)) ;
#89545=DIRECTION('center_axis',(-2.30392961653169E-15,-1.,2.49559129361712E-15)) ;
#89546=DIRECTION('ref_axis',(-2.67860162145163E-32,2.49559129361712E-15,
1.)) ;
#89547=DIRECTION('center_axis',(0.,1.,0.)) ;
#89548=DIRECTION('ref_axis',(1.,0.,0.)) ;
#89549=DIRECTION('center_axis',(-0.577350269189625,-0.577350269189626,-0.577350269189627)) ;
#89550=DIRECTION('ref_axis',(-8.18676000863892E-15,-0.707106781186544,0.707106781186551)) ;
#89551=DIRECTION('center_axis',(0.,-4.50404941150742E-15,1.)) ;
#89552=DIRECTION('ref_axis',(0.,1.,4.50404941150742E-15)) ;
#89553=DIRECTION('center_axis',(0.,1.,-1.95511867169518E-16)) ;
#89554=DIRECTION('ref_axis',(0.,1.95511867169518E-16,1.)) ;
#89555=DIRECTION('center_axis',(0.,-1.,-2.10827844793964E-15)) ;
#89556=DIRECTION('ref_axis',(0.,2.10827844793964E-15,-1.)) ;
#89557=DIRECTION('center_axis',(0.,0.,-1.)) ;
#89558=DIRECTION('ref_axis',(-1.,0.,0.)) ;
#89559=DIRECTION('center_axis',(-6.77626357803439E-17,-6.7762635780344E-17,
1.)) ;
#89560=DIRECTION('ref_axis',(-1.3684555315672E-48,-1.,-6.7762635780344E-17)) ;
#89561=DIRECTION('center_axis',(0.577350269189625,0.577350269189626,0.577350269189627)) ;
#89562=DIRECTION('ref_axis',(-9.19305248608458E-17,-0.707106781186548,0.707106781186547)) ;
#89563=DIRECTION('center_axis',(0.577350269189625,0.577350269189626,0.577350269189627)) ;
#89564=DIRECTION('ref_axis',(-9.19305248608458E-17,-0.707106781186548,0.707106781186547)) ;
#89565=DIRECTION('center_axis',(0.,1.,0.)) ;
#89566=DIRECTION('ref_axis',(1.,0.,0.)) ;
#89567=DIRECTION('center_axis',(-0.577350269189624,-0.577350269189627,0.577350269189626)) ;
#89568=DIRECTION('ref_axis',(-1.46369207068818E-16,0.707106781186547,0.707106781186548)) ;
#89569=DIRECTION('center_axis',(0.,0.,-1.)) ;
#89570=DIRECTION('ref_axis',(-1.,0.,0.)) ;
#89571=DIRECTION('center_axis',(0.,0.,1.)) ;
#89572=DIRECTION('ref_axis',(-1.,1.0842021724855E-15,0.)) ;
#89573=DIRECTION('center_axis',(0.,0.,-1.)) ;
#89574=DIRECTION('ref_axis',(-1.,0.,0.)) ;
#89575=DIRECTION('center_axis',(-0.577350269189625,-0.577350269189626,0.577350269189627)) ;
#89576=DIRECTION('ref_axis',(-1.51735478582867E-16,-0.707106781186548,-0.707106781186547)) ;
#89577=DIRECTION('center_axis',(0.577350269189625,0.577350269189626,-0.577350269189627)) ;
#89578=DIRECTION('ref_axis',(-8.00734514747286E-15,-0.707106781186544,-0.707106781186551)) ;
#89579=DIRECTION('center_axis',(0.,0.,1.)) ;
#89580=DIRECTION('ref_axis',(1.,0.,0.)) ;
#89581=DIRECTION('center_axis',(0.,-1.,0.)) ;
#89582=DIRECTION('ref_axis',(0.,0.,-1.)) ;
#89583=DIRECTION('center_axis',(9.85638338623186E-18,1.,0.)) ;
#89584=DIRECTION('ref_axis',(-1.,9.85638338623186E-18,0.)) ;
#89585=DIRECTION('center_axis',(0.,-1.,0.)) ;
#89586=DIRECTION('ref_axis',(0.,0.,-1.)) ;
#89587=DIRECTION('center_axis',(0.,1.,0.)) ;
#89588=DIRECTION('ref_axis',(1.,0.,0.)) ;
#89589=DIRECTION('center_axis',(-1.,0.,0.)) ;
#89590=DIRECTION('ref_axis',(0.,0.,1.)) ;
#89591=DIRECTION('center_axis',(1.,-9.85638338623186E-18,0.)) ;
#89592=DIRECTION('ref_axis',(9.85638338623186E-18,1.,0.)) ;
#89593=DIRECTION('center_axis',(-1.,0.,0.)) ;
#89594=DIRECTION('ref_axis',(0.,0.,1.)) ;
#89595=DIRECTION('center_axis',(0.,1.,0.)) ;
#89596=DIRECTION('ref_axis',(1.,0.,0.)) ;
#89597=DIRECTION('center_axis',(0.,1.,0.)) ;
#89598=DIRECTION('ref_axis',(0.,0.,1.)) ;
#89599=DIRECTION('center_axis',(-9.85638338623186E-18,-1.,0.)) ;
#89600=DIRECTION('ref_axis',(1.,-9.85638338623186E-18,0.)) ;
#89601=DIRECTION('center_axis',(0.,1.,0.)) ;
#89602=DIRECTION('ref_axis',(0.,0.,1.)) ;
#89603=DIRECTION('center_axis',(0.,0.,1.)) ;
#89604=DIRECTION('ref_axis',(1.,0.,0.)) ;
#89605=DIRECTION('center_axis',(0.,0.,1.)) ;
#89606=DIRECTION('ref_axis',(1.,0.,0.)) ;
#89607=DIRECTION('center_axis',(0.,-1.,0.)) ;
#89608=DIRECTION('ref_axis',(0.,0.,-1.)) ;
#89609=DIRECTION('center_axis',(-9.85638338623186E-18,-1.,0.)) ;
#89610=DIRECTION('ref_axis',(1.,-9.85638338623186E-18,0.)) ;
#89611=DIRECTION('center_axis',(0.,-1.,0.)) ;
#89612=DIRECTION('ref_axis',(0.,0.,-1.)) ;
#89613=DIRECTION('center_axis',(0.,1.,0.)) ;
#89614=DIRECTION('ref_axis',(1.,0.,0.)) ;
#89615=DIRECTION('center_axis',(1.,-7.66646708341686E-16,0.)) ;
#89616=DIRECTION('ref_axis',(7.66646708341686E-16,1.,0.)) ;
#89617=DIRECTION('center_axis',(1.,-9.85638338623186E-18,0.)) ;
#89618=DIRECTION('ref_axis',(9.85638338623186E-18,1.,0.)) ;
#89619=DIRECTION('center_axis',(1.,0.,0.)) ;
#89620=DIRECTION('ref_axis',(0.,0.,-1.)) ;
#89621=DIRECTION('center_axis',(0.,1.,0.)) ;
#89622=DIRECTION('ref_axis',(1.,0.,0.)) ;
#89623=DIRECTION('center_axis',(0.,1.,0.)) ;
#89624=DIRECTION('ref_axis',(0.,0.,1.)) ;
#89625=DIRECTION('center_axis',(-9.85638338623186E-18,-1.,0.)) ;
#89626=DIRECTION('ref_axis',(1.,-9.85638338623186E-18,0.)) ;
#89627=DIRECTION('center_axis',(0.,1.,0.)) ;
#89628=DIRECTION('ref_axis',(0.,0.,1.)) ;
#89629=DIRECTION('center_axis',(0.,0.,1.)) ;
#89630=DIRECTION('ref_axis',(1.,0.,0.)) ;
#89631=DIRECTION('center_axis',(-1.,-1.95511867169517E-16,0.)) ;
#89632=DIRECTION('ref_axis',(1.95511867169517E-16,-1.,0.)) ;
#89633=DIRECTION('center_axis',(1.,0.,0.)) ;
#89634=DIRECTION('ref_axis',(0.,0.,-1.)) ;
#89635=DIRECTION('center_axis',(0.,1.,0.)) ;
#89636=DIRECTION('ref_axis',(1.,0.,0.)) ;
#89637=DIRECTION('center_axis',(-2.29994012502506E-15,-1.,0.)) ;
#89638=DIRECTION('ref_axis',(1.,-2.29994012502506E-15,0.)) ;
#89639=DIRECTION('center_axis',(-1.95511867169517E-16,1.,0.)) ;
#89640=DIRECTION('ref_axis',(-1.,-1.95511867169517E-16,0.)) ;
#89641=DIRECTION('center_axis',(0.,-1.,0.)) ;
#89642=DIRECTION('ref_axis',(0.,0.,-1.)) ;
#89643=DIRECTION('center_axis',(0.,1.,0.)) ;
#89644=DIRECTION('ref_axis',(1.,0.,0.)) ;
#89645=DIRECTION('center_axis',(-1.,0.,0.)) ;
#89646=DIRECTION('ref_axis',(0.,0.,1.)) ;
#89647=DIRECTION('center_axis',(1.,-1.06642836637918E-16,0.)) ;
#89648=DIRECTION('ref_axis',(1.06642836637918E-16,1.,0.)) ;
#89649=DIRECTION('center_axis',(1.,1.95511867169517E-16,0.)) ;
#89650=DIRECTION('ref_axis',(-1.95511867169517E-16,1.,0.)) ;
#89651=DIRECTION('center_axis',(1.,0.,0.)) ;
#89652=DIRECTION('ref_axis',(0.,0.,-1.)) ;
#89653=DIRECTION('center_axis',(0.,1.,0.)) ;
#89654=DIRECTION('ref_axis',(1.,0.,0.)) ;
#89655=DIRECTION('center_axis',(2.29994012502506E-15,-1.,0.)) ;
#89656=DIRECTION('ref_axis',(1.,2.29994012502506E-15,0.)) ;
#89657=DIRECTION('center_axis',(-1.95511867169517E-16,1.,0.)) ;
#89658=DIRECTION('ref_axis',(-1.,-1.95511867169517E-16,0.)) ;
#89659=DIRECTION('center_axis',(0.,-1.,0.)) ;
#89660=DIRECTION('ref_axis',(0.,0.,-1.)) ;
#89661=DIRECTION('center_axis',(-1.,1.06642836637918E-16,0.)) ;
#89662=DIRECTION('ref_axis',(-1.06642836637918E-16,-1.,0.)) ;
#89663=DIRECTION('center_axis',(1.,0.,0.)) ;
#89664=DIRECTION('ref_axis',(0.,0.,-1.)) ;
#89665=DIRECTION('center_axis',(0.,1.,0.)) ;
#89666=DIRECTION('ref_axis',(1.,0.,0.)) ;
#89667=DIRECTION('center_axis',(-1.,-1.53063836115601E-16,0.)) ;
#89668=DIRECTION('ref_axis',(1.53063836115601E-16,-1.,0.)) ;
#89669=DIRECTION('',(0.,0.,1.)) ;
#89670=DIRECTION('',(-1.53063836115601E-16,1.,-1.020425574104E-16)) ;
#89671=DIRECTION('',(0.,0.,-1.)) ;
#89672=DIRECTION('',(1.53063836115601E-16,-1.,5.10212787052002E-17)) ;
#89673=DIRECTION('',(0.,0.,1.)) ;
#89674=DIRECTION('',(-1.53063836115601E-16,1.,-1.30104260698261E-16)) ;
#89675=DIRECTION('center_axis',(-1.,-1.53063836115601E-16,0.)) ;
#89676=DIRECTION('ref_axis',(1.53063836115601E-16,-1.,0.)) ;
#89677=DIRECTION('',(0.,0.,1.)) ;
#89678=DIRECTION('center_axis',(-1.,-1.53063836115601E-16,0.)) ;
#89679=DIRECTION('ref_axis',(1.53063836115601E-16,-1.,0.)) ;
#89680=DIRECTION('',(1.53063836115601E-16,-1.,-1.30104260698261E-16)) ;
#89681=DIRECTION('center_axis',(-1.,-1.53063836115601E-16,0.)) ;
#89682=DIRECTION('ref_axis',(1.53063836115601E-16,-1.,0.)) ;
#89683=DIRECTION('',(0.,0.,1.)) ;
#89684=DIRECTION('',(-1.53063836115601E-16,1.,-1.020425574104E-16)) ;
#89685=DIRECTION('',(0.,0.,-1.)) ;
#89686=DIRECTION('',(1.53063836115601E-16,-1.,5.10212787052002E-17)) ;
#89687=DIRECTION('',(0.,0.,1.)) ;
#89688=DIRECTION('',(-1.53063836115601E-16,1.,-1.30104260698261E-16)) ;
#89689=DIRECTION('center_axis',(-1.,-1.53063836115601E-16,0.)) ;
#89690=DIRECTION('ref_axis',(1.53063836115601E-16,-1.,0.)) ;
#89691=DIRECTION('',(0.,0.,1.)) ;
#89692=DIRECTION('center_axis',(-1.,-1.53063836115601E-16,0.)) ;
#89693=DIRECTION('ref_axis',(1.53063836115601E-16,-1.,0.)) ;
#89694=DIRECTION('',(1.53063836115601E-16,-1.,-1.30104260698261E-16)) ;
#89695=DIRECTION('center_axis',(-1.,-1.53063836115601E-16,0.)) ;
#89696=DIRECTION('ref_axis',(1.53063836115601E-16,-1.,0.)) ;
#89697=DIRECTION('',(0.,0.,1.)) ;
#89698=DIRECTION('',(-1.53063836115601E-16,1.,-1.020425574104E-16)) ;
#89699=DIRECTION('',(0.,0.,-1.)) ;
#89700=DIRECTION('',(1.53063836115601E-16,-1.,5.10212787052002E-17)) ;
#89701=DIRECTION('',(0.,0.,1.)) ;
#89702=DIRECTION('',(-1.53063836115601E-16,1.,-1.30104260698261E-16)) ;
#89703=DIRECTION('center_axis',(-1.,-1.53063836115601E-16,0.)) ;
#89704=DIRECTION('ref_axis',(1.53063836115601E-16,-1.,0.)) ;
#89705=DIRECTION('',(0.,0.,1.)) ;
#89706=DIRECTION('center_axis',(-1.,-1.53063836115601E-16,0.)) ;
#89707=DIRECTION('ref_axis',(1.53063836115601E-16,-1.,0.)) ;
#89708=DIRECTION('',(1.53063836115601E-16,-1.,-1.30104260698261E-16)) ;
#89709=DIRECTION('center_axis',(-1.,-1.53063836115601E-16,0.)) ;
#89710=DIRECTION('ref_axis',(1.53063836115601E-16,-1.,0.)) ;
#89711=DIRECTION('',(0.,0.,1.)) ;
#89712=DIRECTION('',(-1.53063836115601E-16,1.,-1.020425574104E-16)) ;
#89713=DIRECTION('',(0.,0.,-1.)) ;
#89714=DIRECTION('',(1.53063836115601E-16,-1.,5.10212787052002E-17)) ;
#89715=DIRECTION('',(0.,0.,1.)) ;
#89716=DIRECTION('',(-1.53063836115601E-16,1.,-1.30104260698261E-16)) ;
#89717=DIRECTION('center_axis',(-1.,-1.53063836115601E-16,0.)) ;
#89718=DIRECTION('ref_axis',(1.53063836115601E-16,-1.,0.)) ;
#89719=DIRECTION('',(0.,0.,1.)) ;
#89720=DIRECTION('center_axis',(-1.,-1.53063836115601E-16,0.)) ;
#89721=DIRECTION('ref_axis',(1.53063836115601E-16,-1.,0.)) ;
#89722=DIRECTION('',(1.53063836115601E-16,-1.,-1.30104260698261E-16)) ;
#89723=DIRECTION('center_axis',(-1.,-1.53063836115601E-16,0.)) ;
#89724=DIRECTION('ref_axis',(1.53063836115601E-16,-1.,0.)) ;
#89725=DIRECTION('',(0.,0.,1.)) ;
#89726=DIRECTION('',(-1.53063836115601E-16,1.,-1.020425574104E-16)) ;
#89727=DIRECTION('',(0.,0.,-1.)) ;
#89728=DIRECTION('',(1.53063836115601E-16,-1.,5.10212787052002E-17)) ;
#89729=DIRECTION('',(0.,0.,1.)) ;
#89730=DIRECTION('',(-1.53063836115601E-16,1.,-1.30104260698261E-16)) ;
#89731=DIRECTION('center_axis',(-1.,-1.53063836115601E-16,0.)) ;
#89732=DIRECTION('ref_axis',(1.53063836115601E-16,-1.,0.)) ;
#89733=DIRECTION('',(0.,0.,1.)) ;
#89734=DIRECTION('center_axis',(-1.,-1.53063836115601E-16,0.)) ;
#89735=DIRECTION('ref_axis',(1.53063836115601E-16,-1.,0.)) ;
#89736=DIRECTION('',(1.53063836115601E-16,-1.,-1.30104260698261E-16)) ;
#89737=DIRECTION('center_axis',(-1.,-1.53063836115601E-16,0.)) ;
#89738=DIRECTION('ref_axis',(1.53063836115601E-16,-1.,0.)) ;
#89739=DIRECTION('',(0.,0.,1.)) ;
#89740=DIRECTION('',(-1.53063836115601E-16,1.,-1.020425574104E-16)) ;
#89741=DIRECTION('',(0.,0.,-1.)) ;
#89742=DIRECTION('',(1.53063836115601E-16,-1.,5.10212787052002E-17)) ;
#89743=DIRECTION('',(0.,0.,1.)) ;
#89744=DIRECTION('',(-1.53063836115601E-16,1.,-1.30104260698261E-16)) ;
#89745=DIRECTION('center_axis',(-1.,-1.53063836115601E-16,0.)) ;
#89746=DIRECTION('ref_axis',(1.53063836115601E-16,-1.,0.)) ;
#89747=DIRECTION('',(0.,0.,1.)) ;
#89748=DIRECTION('center_axis',(-1.,-1.53063836115601E-16,0.)) ;
#89749=DIRECTION('ref_axis',(1.53063836115601E-16,-1.,0.)) ;
#89750=DIRECTION('',(1.53063836115601E-16,-1.,-1.30104260698261E-16)) ;
#89751=DIRECTION('center_axis',(-1.,-1.53063836115601E-16,0.)) ;
#89752=DIRECTION('ref_axis',(1.53063836115601E-16,-1.,0.)) ;
#89753=DIRECTION('',(0.,0.,1.)) ;
#89754=DIRECTION('',(-1.53063836115601E-16,1.,-1.020425574104E-16)) ;
#89755=DIRECTION('',(0.,0.,-1.)) ;
#89756=DIRECTION('',(1.53063836115601E-16,-1.,5.10212787052002E-17)) ;
#89757=DIRECTION('',(0.,0.,1.)) ;
#89758=DIRECTION('',(-1.53063836115601E-16,1.,-1.30104260698261E-16)) ;
#89759=DIRECTION('center_axis',(-1.,-1.53063836115601E-16,0.)) ;
#89760=DIRECTION('ref_axis',(1.53063836115601E-16,-1.,0.)) ;
#89761=DIRECTION('',(0.,0.,1.)) ;
#89762=DIRECTION('center_axis',(-1.,-1.53063836115601E-16,0.)) ;
#89763=DIRECTION('ref_axis',(1.53063836115601E-16,-1.,0.)) ;
#89764=DIRECTION('',(1.53063836115601E-16,-1.,-1.30104260698261E-16)) ;
#89765=DIRECTION('center_axis',(-1.,-1.53063836115601E-16,0.)) ;
#89766=DIRECTION('ref_axis',(1.53063836115601E-16,-1.,0.)) ;
#89767=DIRECTION('',(0.,0.,1.)) ;
#89768=DIRECTION('',(-1.53063836115601E-16,1.,-1.020425574104E-16)) ;
#89769=DIRECTION('',(0.,0.,-1.)) ;
#89770=DIRECTION('',(1.53063836115601E-16,-1.,5.10212787052002E-17)) ;
#89771=DIRECTION('',(0.,0.,1.)) ;
#89772=DIRECTION('',(-1.53063836115601E-16,1.,-1.30104260698261E-16)) ;
#89773=DIRECTION('center_axis',(-1.,-1.53063836115601E-16,0.)) ;
#89774=DIRECTION('ref_axis',(1.53063836115601E-16,-1.,0.)) ;
#89775=DIRECTION('',(0.,0.,1.)) ;
#89776=DIRECTION('center_axis',(-1.,-1.53063836115601E-16,0.)) ;
#89777=DIRECTION('ref_axis',(1.53063836115601E-16,-1.,0.)) ;
#89778=DIRECTION('',(1.53063836115601E-16,-1.,-1.30104260698261E-16)) ;
#89779=DIRECTION('center_axis',(-1.,-1.53063836115601E-16,0.)) ;
#89780=DIRECTION('ref_axis',(1.53063836115601E-16,-1.,0.)) ;
#89781=DIRECTION('',(0.,0.,1.)) ;
#89782=DIRECTION('',(-1.53063836115601E-16,1.,-1.020425574104E-16)) ;
#89783=DIRECTION('',(0.,0.,-1.)) ;
#89784=DIRECTION('',(1.53063836115601E-16,-1.,5.10212787052002E-17)) ;
#89785=DIRECTION('',(0.,0.,1.)) ;
#89786=DIRECTION('',(-1.53063836115601E-16,1.,-1.30104260698261E-16)) ;
#89787=DIRECTION('center_axis',(-1.,-1.53063836115601E-16,0.)) ;
#89788=DIRECTION('ref_axis',(1.53063836115601E-16,-1.,0.)) ;
#89789=DIRECTION('',(0.,0.,1.)) ;
#89790=DIRECTION('center_axis',(-1.,-1.53063836115601E-16,0.)) ;
#89791=DIRECTION('ref_axis',(1.53063836115601E-16,-1.,0.)) ;
#89792=DIRECTION('',(1.53063836115601E-16,-1.,-1.30104260698261E-16)) ;
#89793=DIRECTION('center_axis',(-1.53063836115601E-16,1.,0.)) ;
#89794=DIRECTION('ref_axis',(-1.,-1.53063836115601E-16,0.)) ;
#89795=DIRECTION('',(-1.,-1.53063836115601E-16,2.73691106313441E-48)) ;
#89796=DIRECTION('',(0.,0.,-1.)) ;
#89797=DIRECTION('',(1.,1.53063836115601E-16,-1.53236300070382E-33)) ;
#89798=DIRECTION('',(0.,0.,1.)) ;
#89799=DIRECTION('center_axis',(1.99142572374599E-32,-1.30104260698261E-16,
-1.)) ;
#89800=DIRECTION('ref_axis',(0.,1.,-1.30104260698261E-16)) ;
#89801=DIRECTION('',(-1.,-1.53063836115601E-16,2.73691106313441E-48)) ;
#89802=DIRECTION('',(1.53063836115601E-16,-1.,1.30104260698261E-16)) ;
#89803=DIRECTION('',(1.,1.53063836115601E-16,-2.73691106313441E-48)) ;
#89804=DIRECTION('center_axis',(-1.53063836115601E-16,1.,0.)) ;
#89805=DIRECTION('ref_axis',(-1.,-1.53063836115601E-16,0.)) ;
#89806=DIRECTION('',(-1.,-1.53063836115601E-16,-2.73691106313441E-48)) ;
#89807=DIRECTION('',(0.,0.,-1.)) ;
#89808=DIRECTION('',(1.,1.53063836115601E-16,-2.73691106313441E-48)) ;
#89809=DIRECTION('',(0.,0.,1.)) ;
#89810=DIRECTION('center_axis',(1.99142572374599E-32,-1.30104260698261E-16,
1.)) ;
#89811=DIRECTION('ref_axis',(0.,-1.,-1.30104260698261E-16)) ;
#89812=DIRECTION('',(-1.,-1.53063836115601E-16,-2.73691106313441E-48)) ;
#89813=DIRECTION('',(-1.53063836115601E-16,1.,1.30104260698261E-16)) ;
#89814=DIRECTION('',(1.,1.53063836115601E-16,2.73691106313441E-48)) ;
#89815=DIRECTION('',(2.16840434497101E-16,-1.,-1.30104260698261E-16)) ;
#89816=DIRECTION('center_axis',(-1.53063836115601E-16,1.,0.)) ;
#89817=DIRECTION('ref_axis',(-1.,-1.53063836115601E-16,0.)) ;
#89818=DIRECTION('',(-1.,-1.53063836115601E-16,3.06472600140763E-33)) ;
#89819=DIRECTION('',(0.,0.,-1.)) ;
#89820=DIRECTION('',(1.,1.53063836115601E-16,2.73691106313441E-48)) ;
#89821=DIRECTION('',(0.,0.,1.)) ;
#89822=DIRECTION('center_axis',(-1.53063836115601E-16,1.,0.)) ;
#89823=DIRECTION('ref_axis',(-1.,-1.53063836115601E-16,0.)) ;
#89824=DIRECTION('',(-1.,-1.53063836115601E-16,2.73691106313441E-48)) ;
#89825=DIRECTION('',(0.,0.,-1.)) ;
#89826=DIRECTION('',(1.,1.53063836115601E-16,-1.53236300070382E-33)) ;
#89827=DIRECTION('',(0.,0.,1.)) ;
#89828=DIRECTION('center_axis',(1.99142572374599E-32,-1.30104260698261E-16,
-1.)) ;
#89829=DIRECTION('ref_axis',(0.,1.,-1.30104260698261E-16)) ;
#89830=DIRECTION('',(-1.,-1.53063836115601E-16,2.73691106313441E-48)) ;
#89831=DIRECTION('',(1.53063836115601E-16,-1.,1.30104260698261E-16)) ;
#89832=DIRECTION('',(1.,1.53063836115601E-16,-2.73691106313441E-48)) ;
#89833=DIRECTION('center_axis',(-1.53063836115601E-16,1.,0.)) ;
#89834=DIRECTION('ref_axis',(-1.,-1.53063836115601E-16,0.)) ;
#89835=DIRECTION('',(-1.,-1.53063836115601E-16,-2.73691106313441E-48)) ;
#89836=DIRECTION('',(0.,0.,-1.)) ;
#89837=DIRECTION('',(1.,1.53063836115601E-16,-2.73691106313441E-48)) ;
#89838=DIRECTION('',(0.,0.,1.)) ;
#89839=DIRECTION('center_axis',(1.99142572374599E-32,-1.30104260698261E-16,
1.)) ;
#89840=DIRECTION('ref_axis',(0.,-1.,-1.30104260698261E-16)) ;
#89841=DIRECTION('',(-1.,-1.53063836115601E-16,-2.73691106313441E-48)) ;
#89842=DIRECTION('',(-1.53063836115601E-16,1.,1.30104260698261E-16)) ;
#89843=DIRECTION('',(1.,1.53063836115601E-16,2.73691106313441E-48)) ;
#89844=DIRECTION('',(2.16840434497101E-16,-1.,-1.30104260698261E-16)) ;
#89845=DIRECTION('center_axis',(-1.53063836115601E-16,1.,0.)) ;
#89846=DIRECTION('ref_axis',(-1.,-1.53063836115601E-16,0.)) ;
#89847=DIRECTION('',(-1.,-1.53063836115601E-16,3.06472600140763E-33)) ;
#89848=DIRECTION('',(0.,0.,-1.)) ;
#89849=DIRECTION('',(1.,1.53063836115601E-16,2.73691106313441E-48)) ;
#89850=DIRECTION('',(0.,0.,1.)) ;
#89851=DIRECTION('center_axis',(-1.53063836115601E-16,1.,0.)) ;
#89852=DIRECTION('ref_axis',(-1.,-1.53063836115601E-16,0.)) ;
#89853=DIRECTION('',(-1.,-1.53063836115601E-16,2.73691106313441E-48)) ;
#89854=DIRECTION('',(0.,0.,-1.)) ;
#89855=DIRECTION('',(1.,1.53063836115601E-16,-1.53236300070382E-33)) ;
#89856=DIRECTION('',(0.,0.,1.)) ;
#89857=DIRECTION('center_axis',(1.99142572374599E-32,-1.30104260698261E-16,
-1.)) ;
#89858=DIRECTION('ref_axis',(0.,1.,-1.30104260698261E-16)) ;
#89859=DIRECTION('',(-1.,-1.53063836115601E-16,2.73691106313441E-48)) ;
#89860=DIRECTION('',(1.53063836115601E-16,-1.,1.30104260698261E-16)) ;
#89861=DIRECTION('',(1.,1.53063836115601E-16,-2.73691106313441E-48)) ;
#89862=DIRECTION('center_axis',(-1.53063836115601E-16,1.,0.)) ;
#89863=DIRECTION('ref_axis',(-1.,-1.53063836115601E-16,0.)) ;
#89864=DIRECTION('',(-1.,-1.53063836115601E-16,-2.73691106313441E-48)) ;
#89865=DIRECTION('',(0.,0.,-1.)) ;
#89866=DIRECTION('',(1.,1.53063836115601E-16,-2.73691106313441E-48)) ;
#89867=DIRECTION('',(0.,0.,1.)) ;
#89868=DIRECTION('center_axis',(1.99142572374599E-32,-1.30104260698261E-16,
1.)) ;
#89869=DIRECTION('ref_axis',(0.,-1.,-1.30104260698261E-16)) ;
#89870=DIRECTION('',(-1.,-1.53063836115601E-16,-2.73691106313441E-48)) ;
#89871=DIRECTION('',(-1.53063836115601E-16,1.,1.30104260698261E-16)) ;
#89872=DIRECTION('',(1.,1.53063836115601E-16,2.73691106313441E-48)) ;
#89873=DIRECTION('',(2.16840434497101E-16,-1.,-1.30104260698261E-16)) ;
#89874=DIRECTION('center_axis',(-1.53063836115601E-16,1.,0.)) ;
#89875=DIRECTION('ref_axis',(-1.,-1.53063836115601E-16,0.)) ;
#89876=DIRECTION('',(-1.,-1.53063836115601E-16,3.06472600140763E-33)) ;
#89877=DIRECTION('',(0.,0.,-1.)) ;
#89878=DIRECTION('',(1.,1.53063836115601E-16,2.73691106313441E-48)) ;
#89879=DIRECTION('',(0.,0.,1.)) ;
#89880=DIRECTION('center_axis',(-1.53063836115601E-16,1.,0.)) ;
#89881=DIRECTION('ref_axis',(-1.,-1.53063836115601E-16,0.)) ;
#89882=DIRECTION('',(-1.,-1.53063836115601E-16,2.73691106313441E-48)) ;
#89883=DIRECTION('',(0.,0.,-1.)) ;
#89884=DIRECTION('',(1.,1.53063836115601E-16,-1.53236300070382E-33)) ;
#89885=DIRECTION('',(0.,0.,1.)) ;
#89886=DIRECTION('center_axis',(1.99142572374599E-32,-1.30104260698261E-16,
-1.)) ;
#89887=DIRECTION('ref_axis',(0.,1.,-1.30104260698261E-16)) ;
#89888=DIRECTION('',(-1.,-1.53063836115601E-16,2.73691106313441E-48)) ;
#89889=DIRECTION('',(1.53063836115601E-16,-1.,1.30104260698261E-16)) ;
#89890=DIRECTION('',(1.,1.53063836115601E-16,-2.73691106313441E-48)) ;
#89891=DIRECTION('center_axis',(-1.53063836115601E-16,1.,0.)) ;
#89892=DIRECTION('ref_axis',(-1.,-1.53063836115601E-16,0.)) ;
#89893=DIRECTION('',(-1.,-1.53063836115601E-16,-2.73691106313441E-48)) ;
#89894=DIRECTION('',(0.,0.,-1.)) ;
#89895=DIRECTION('',(1.,1.53063836115601E-16,-2.73691106313441E-48)) ;
#89896=DIRECTION('',(0.,0.,1.)) ;
#89897=DIRECTION('center_axis',(1.99142572374599E-32,-1.30104260698261E-16,
1.)) ;
#89898=DIRECTION('ref_axis',(0.,-1.,-1.30104260698261E-16)) ;
#89899=DIRECTION('',(-1.,-1.53063836115601E-16,-2.73691106313441E-48)) ;
#89900=DIRECTION('',(-1.53063836115601E-16,1.,1.30104260698261E-16)) ;
#89901=DIRECTION('',(1.,1.53063836115601E-16,2.73691106313441E-48)) ;
#89902=DIRECTION('',(2.16840434497101E-16,-1.,-1.30104260698261E-16)) ;
#89903=DIRECTION('center_axis',(-1.53063836115601E-16,1.,0.)) ;
#89904=DIRECTION('ref_axis',(-1.,-1.53063836115601E-16,0.)) ;
#89905=DIRECTION('',(-1.,-1.53063836115601E-16,3.06472600140763E-33)) ;
#89906=DIRECTION('',(0.,0.,-1.)) ;
#89907=DIRECTION('',(1.,1.53063836115601E-16,2.73691106313441E-48)) ;
#89908=DIRECTION('',(0.,0.,1.)) ;
#89909=DIRECTION('center_axis',(-1.53063836115601E-16,1.,0.)) ;
#89910=DIRECTION('ref_axis',(-1.,-1.53063836115601E-16,0.)) ;
#89911=DIRECTION('',(-1.,-1.53063836115601E-16,2.73691106313441E-48)) ;
#89912=DIRECTION('',(0.,0.,-1.)) ;
#89913=DIRECTION('',(1.,1.53063836115601E-16,-1.53236300070382E-33)) ;
#89914=DIRECTION('',(0.,0.,1.)) ;
#89915=DIRECTION('center_axis',(1.99142572374599E-32,-1.30104260698261E-16,
-1.)) ;
#89916=DIRECTION('ref_axis',(0.,1.,-1.30104260698261E-16)) ;
#89917=DIRECTION('',(-1.,-1.53063836115601E-16,2.73691106313441E-48)) ;
#89918=DIRECTION('',(1.53063836115601E-16,-1.,1.30104260698261E-16)) ;
#89919=DIRECTION('',(1.,1.53063836115601E-16,-2.73691106313441E-48)) ;
#89920=DIRECTION('center_axis',(-1.53063836115601E-16,1.,0.)) ;
#89921=DIRECTION('ref_axis',(-1.,-1.53063836115601E-16,0.)) ;
#89922=DIRECTION('',(-1.,-1.53063836115601E-16,-2.73691106313441E-48)) ;
#89923=DIRECTION('',(0.,0.,-1.)) ;
#89924=DIRECTION('',(1.,1.53063836115601E-16,-2.73691106313441E-48)) ;
#89925=DIRECTION('',(0.,0.,1.)) ;
#89926=DIRECTION('center_axis',(1.99142572374599E-32,-1.30104260698261E-16,
1.)) ;
#89927=DIRECTION('ref_axis',(0.,-1.,-1.30104260698261E-16)) ;
#89928=DIRECTION('',(-1.,-1.53063836115601E-16,-2.73691106313441E-48)) ;
#89929=DIRECTION('',(-1.53063836115601E-16,1.,1.30104260698261E-16)) ;
#89930=DIRECTION('',(1.,1.53063836115601E-16,2.73691106313441E-48)) ;
#89931=DIRECTION('',(2.16840434497101E-16,-1.,-1.30104260698261E-16)) ;
#89932=DIRECTION('center_axis',(-1.53063836115601E-16,1.,0.)) ;
#89933=DIRECTION('ref_axis',(-1.,-1.53063836115601E-16,0.)) ;
#89934=DIRECTION('',(-1.,-1.53063836115601E-16,3.06472600140763E-33)) ;
#89935=DIRECTION('',(0.,0.,-1.)) ;
#89936=DIRECTION('',(1.,1.53063836115601E-16,2.73691106313441E-48)) ;
#89937=DIRECTION('',(0.,0.,1.)) ;
#89938=DIRECTION('center_axis',(-1.53063836115601E-16,1.,0.)) ;
#89939=DIRECTION('ref_axis',(-1.,-1.53063836115601E-16,0.)) ;
#89940=DIRECTION('',(-1.,-1.53063836115601E-16,2.73691106313441E-48)) ;
#89941=DIRECTION('',(0.,0.,-1.)) ;
#89942=DIRECTION('',(1.,1.53063836115601E-16,-1.53236300070382E-33)) ;
#89943=DIRECTION('',(0.,0.,1.)) ;
#89944=DIRECTION('center_axis',(1.99142572374599E-32,-1.30104260698261E-16,
-1.)) ;
#89945=DIRECTION('ref_axis',(0.,1.,-1.30104260698261E-16)) ;
#89946=DIRECTION('',(-1.,-1.53063836115601E-16,2.73691106313441E-48)) ;
#89947=DIRECTION('',(1.53063836115601E-16,-1.,1.30104260698261E-16)) ;
#89948=DIRECTION('',(1.,1.53063836115601E-16,-2.73691106313441E-48)) ;
#89949=DIRECTION('center_axis',(-1.53063836115601E-16,1.,0.)) ;
#89950=DIRECTION('ref_axis',(-1.,-1.53063836115601E-16,0.)) ;
#89951=DIRECTION('',(-1.,-1.53063836115601E-16,-2.73691106313441E-48)) ;
#89952=DIRECTION('',(0.,0.,-1.)) ;
#89953=DIRECTION('',(1.,1.53063836115601E-16,-2.73691106313441E-48)) ;
#89954=DIRECTION('',(0.,0.,1.)) ;
#89955=DIRECTION('center_axis',(1.99142572374599E-32,-1.30104260698261E-16,
1.)) ;
#89956=DIRECTION('ref_axis',(0.,-1.,-1.30104260698261E-16)) ;
#89957=DIRECTION('',(-1.,-1.53063836115601E-16,-2.73691106313441E-48)) ;
#89958=DIRECTION('',(-1.53063836115601E-16,1.,1.30104260698261E-16)) ;
#89959=DIRECTION('',(1.,1.53063836115601E-16,2.73691106313441E-48)) ;
#89960=DIRECTION('',(2.16840434497101E-16,-1.,-1.30104260698261E-16)) ;
#89961=DIRECTION('center_axis',(-1.53063836115601E-16,1.,0.)) ;
#89962=DIRECTION('ref_axis',(-1.,-1.53063836115601E-16,0.)) ;
#89963=DIRECTION('',(-1.,-1.53063836115601E-16,3.06472600140763E-33)) ;
#89964=DIRECTION('',(0.,0.,-1.)) ;
#89965=DIRECTION('',(1.,1.53063836115601E-16,2.73691106313441E-48)) ;
#89966=DIRECTION('',(0.,0.,1.)) ;
#89967=DIRECTION('center_axis',(-1.53063836115601E-16,1.,0.)) ;
#89968=DIRECTION('ref_axis',(-1.,-1.53063836115601E-16,0.)) ;
#89969=DIRECTION('',(-1.,-1.53063836115601E-16,2.73691106313441E-48)) ;
#89970=DIRECTION('',(0.,0.,-1.)) ;
#89971=DIRECTION('',(1.,1.53063836115601E-16,-1.53236300070382E-33)) ;
#89972=DIRECTION('',(0.,0.,1.)) ;
#89973=DIRECTION('center_axis',(1.99142572374599E-32,-1.30104260698261E-16,
-1.)) ;
#89974=DIRECTION('ref_axis',(0.,1.,-1.30104260698261E-16)) ;
#89975=DIRECTION('',(-1.,-1.53063836115601E-16,2.73691106313441E-48)) ;
#89976=DIRECTION('',(1.53063836115601E-16,-1.,1.30104260698261E-16)) ;
#89977=DIRECTION('',(1.,1.53063836115601E-16,-2.73691106313441E-48)) ;
#89978=DIRECTION('center_axis',(-1.53063836115601E-16,1.,0.)) ;
#89979=DIRECTION('ref_axis',(-1.,-1.53063836115601E-16,0.)) ;
#89980=DIRECTION('',(-1.,-1.53063836115601E-16,-2.73691106313441E-48)) ;
#89981=DIRECTION('',(0.,0.,-1.)) ;
#89982=DIRECTION('',(1.,1.53063836115601E-16,-2.73691106313441E-48)) ;
#89983=DIRECTION('',(0.,0.,1.)) ;
#89984=DIRECTION('center_axis',(1.99142572374599E-32,-1.30104260698261E-16,
1.)) ;
#89985=DIRECTION('ref_axis',(0.,-1.,-1.30104260698261E-16)) ;
#89986=DIRECTION('',(-1.,-1.53063836115601E-16,-2.73691106313441E-48)) ;
#89987=DIRECTION('',(-1.53063836115601E-16,1.,1.30104260698261E-16)) ;
#89988=DIRECTION('',(1.,1.53063836115601E-16,2.73691106313441E-48)) ;
#89989=DIRECTION('',(2.16840434497101E-16,-1.,-1.30104260698261E-16)) ;
#89990=DIRECTION('center_axis',(-1.53063836115601E-16,1.,0.)) ;
#89991=DIRECTION('ref_axis',(-1.,-1.53063836115601E-16,0.)) ;
#89992=DIRECTION('',(-1.,-1.53063836115601E-16,3.06472600140763E-33)) ;
#89993=DIRECTION('',(0.,0.,-1.)) ;
#89994=DIRECTION('',(1.,1.53063836115601E-16,2.73691106313441E-48)) ;
#89995=DIRECTION('',(0.,0.,1.)) ;
#89996=DIRECTION('center_axis',(-1.53063836115601E-16,1.,0.)) ;
#89997=DIRECTION('ref_axis',(-1.,-1.53063836115601E-16,0.)) ;
#89998=DIRECTION('',(-1.,-1.53063836115601E-16,2.73691106313441E-48)) ;
#89999=DIRECTION('',(0.,0.,-1.)) ;
#90000=DIRECTION('',(1.,1.53063836115601E-16,-1.53236300070382E-33)) ;
#90001=DIRECTION('',(0.,0.,1.)) ;
#90002=DIRECTION('center_axis',(1.99142572374599E-32,-1.30104260698261E-16,
-1.)) ;
#90003=DIRECTION('ref_axis',(0.,1.,-1.30104260698261E-16)) ;
#90004=DIRECTION('',(-1.,-1.53063836115601E-16,2.73691106313441E-48)) ;
#90005=DIRECTION('',(1.53063836115601E-16,-1.,1.30104260698261E-16)) ;
#90006=DIRECTION('',(1.,1.53063836115601E-16,-2.73691106313441E-48)) ;
#90007=DIRECTION('center_axis',(-1.53063836115601E-16,1.,0.)) ;
#90008=DIRECTION('ref_axis',(-1.,-1.53063836115601E-16,0.)) ;
#90009=DIRECTION('',(-1.,-1.53063836115601E-16,-2.73691106313441E-48)) ;
#90010=DIRECTION('',(0.,0.,-1.)) ;
#90011=DIRECTION('',(1.,1.53063836115601E-16,-2.73691106313441E-48)) ;
#90012=DIRECTION('',(0.,0.,1.)) ;
#90013=DIRECTION('center_axis',(1.99142572374599E-32,-1.30104260698261E-16,
1.)) ;
#90014=DIRECTION('ref_axis',(0.,-1.,-1.30104260698261E-16)) ;
#90015=DIRECTION('',(-1.,-1.53063836115601E-16,-2.73691106313441E-48)) ;
#90016=DIRECTION('',(-1.53063836115601E-16,1.,1.30104260698261E-16)) ;
#90017=DIRECTION('',(1.,1.53063836115601E-16,2.73691106313441E-48)) ;
#90018=DIRECTION('',(2.16840434497101E-16,-1.,-1.30104260698261E-16)) ;
#90019=DIRECTION('center_axis',(-1.53063836115601E-16,1.,0.)) ;
#90020=DIRECTION('ref_axis',(-1.,-1.53063836115601E-16,0.)) ;
#90021=DIRECTION('',(-1.,-1.53063836115601E-16,3.06472600140763E-33)) ;
#90022=DIRECTION('',(0.,0.,-1.)) ;
#90023=DIRECTION('',(1.,1.53063836115601E-16,2.73691106313441E-48)) ;
#90024=DIRECTION('',(0.,0.,1.)) ;
#90025=DIRECTION('center_axis',(-1.53063836115601E-16,1.,0.)) ;
#90026=DIRECTION('ref_axis',(-1.,-1.53063836115601E-16,0.)) ;
#90027=DIRECTION('',(-1.,-1.53063836115601E-16,2.73691106313441E-48)) ;
#90028=DIRECTION('',(0.,0.,-1.)) ;
#90029=DIRECTION('',(1.,1.53063836115601E-16,-1.53236300070382E-33)) ;
#90030=DIRECTION('',(0.,0.,1.)) ;
#90031=DIRECTION('center_axis',(1.99142572374599E-32,-1.30104260698261E-16,
-1.)) ;
#90032=DIRECTION('ref_axis',(0.,1.,-1.30104260698261E-16)) ;
#90033=DIRECTION('',(-1.,-1.53063836115601E-16,2.73691106313441E-48)) ;
#90034=DIRECTION('',(1.53063836115601E-16,-1.,1.30104260698261E-16)) ;
#90035=DIRECTION('',(1.,1.53063836115601E-16,-2.73691106313441E-48)) ;
#90036=DIRECTION('center_axis',(-1.53063836115601E-16,1.,0.)) ;
#90037=DIRECTION('ref_axis',(-1.,-1.53063836115601E-16,0.)) ;
#90038=DIRECTION('',(-1.,-1.53063836115601E-16,-2.73691106313441E-48)) ;
#90039=DIRECTION('',(0.,0.,-1.)) ;
#90040=DIRECTION('',(1.,1.53063836115601E-16,-2.73691106313441E-48)) ;
#90041=DIRECTION('',(0.,0.,1.)) ;
#90042=DIRECTION('center_axis',(1.99142572374599E-32,-1.30104260698261E-16,
1.)) ;
#90043=DIRECTION('ref_axis',(0.,-1.,-1.30104260698261E-16)) ;
#90044=DIRECTION('',(-1.,-1.53063836115601E-16,-2.73691106313441E-48)) ;
#90045=DIRECTION('',(-1.53063836115601E-16,1.,1.30104260698261E-16)) ;
#90046=DIRECTION('',(1.,1.53063836115601E-16,2.73691106313441E-48)) ;
#90047=DIRECTION('',(2.16840434497101E-16,-1.,-1.30104260698261E-16)) ;
#90048=DIRECTION('center_axis',(-1.53063836115601E-16,1.,0.)) ;
#90049=DIRECTION('ref_axis',(-1.,-1.53063836115601E-16,0.)) ;
#90050=DIRECTION('',(-1.,-1.53063836115601E-16,3.06472600140763E-33)) ;
#90051=DIRECTION('',(0.,0.,-1.)) ;
#90052=DIRECTION('',(1.,1.53063836115601E-16,2.73691106313441E-48)) ;
#90053=DIRECTION('',(0.,0.,1.)) ;
#90054=DIRECTION('center_axis',(1.,0.,0.)) ;
#90055=DIRECTION('ref_axis',(0.,0.,-1.)) ;
#90056=DIRECTION('',(1.,0.,0.)) ;
#90057=DIRECTION('center_axis',(1.,0.,0.)) ;
#90058=DIRECTION('ref_axis',(0.,0.,1.)) ;
#90059=DIRECTION('',(1.,0.,0.)) ;
#90060=DIRECTION('center_axis',(-1.,0.,0.)) ;
#90061=DIRECTION('ref_axis',(0.,0.,-1.)) ;
#90062=DIRECTION('center_axis',(0.,0.,1.)) ;
#90063=DIRECTION('ref_axis',(1.,0.,0.)) ;
#90064=DIRECTION('',(0.,1.,0.)) ;
#90065=DIRECTION('',(1.,0.,0.)) ;
#90066=DIRECTION('',(0.,-1.,0.)) ;
#90067=DIRECTION('center_axis',(1.,0.,0.)) ;
#90068=DIRECTION('ref_axis',(0.,0.,-1.)) ;
#90069=DIRECTION('center_axis',(1.,0.,0.)) ;
#90070=DIRECTION('ref_axis',(0.,0.,1.)) ;
#90071=DIRECTION('',(1.,0.,0.)) ;
#90072=DIRECTION('center_axis',(-1.,0.,0.)) ;
#90073=DIRECTION('ref_axis',(0.,0.,-1.)) ;
#90074=DIRECTION('center_axis',(0.,-1.,3.99416362155027E-15)) ;
#90075=DIRECTION('ref_axis',(0.,-3.99416362155027E-15,-1.)) ;
#90076=DIRECTION('',(0.,3.99416362155027E-15,1.)) ;
#90077=DIRECTION('',(1.,0.,0.)) ;
#90078=DIRECTION('',(0.,-3.99416362155027E-15,-1.)) ;
#90079=DIRECTION('center_axis',(1.,0.,0.)) ;
#90080=DIRECTION('ref_axis',(0.,0.,-1.)) ;
#90081=DIRECTION('center_axis',(-1.,0.,0.)) ;
#90082=DIRECTION('ref_axis',(0.,1.30104260698266E-14,-1.)) ;
#90083=DIRECTION('',(1.,0.,0.)) ;
#90084=DIRECTION('center_axis',(1.,0.,0.)) ;
#90085=DIRECTION('ref_axis',(0.,0.,-1.)) ;
#90086=DIRECTION('center_axis',(0.,-0.707106781186549,0.707106781186546)) ;
#90087=DIRECTION('ref_axis',(0.,-0.707106781186546,-0.707106781186549)) ;
#90088=DIRECTION('',(0.,0.707106781186546,0.707106781186549)) ;
#90089=DIRECTION('',(1.,0.,0.)) ;
#90090=DIRECTION('',(0.,-0.707106781186546,-0.707106781186549)) ;
#90091=DIRECTION('center_axis',(1.,0.,0.)) ;
#90092=DIRECTION('ref_axis',(0.,0.382683432365084,0.923879532511289)) ;
#90093=DIRECTION('',(1.,0.,0.)) ;
#90094=DIRECTION('center_axis',(1.,0.,0.)) ;
#90095=DIRECTION('ref_axis',(0.,0.,-1.)) ;
#90096=DIRECTION('center_axis',(0.,1.,0.)) ;
#90097=DIRECTION('ref_axis',(0.,0.,1.)) ;
#90098=DIRECTION('',(0.,0.,-1.)) ;
#90099=DIRECTION('',(0.,0.,1.)) ;
#90100=DIRECTION('center_axis',(0.,-0.707106781186547,-0.707106781186548)) ;
#90101=DIRECTION('ref_axis',(0.,0.707106781186548,-0.707106781186547)) ;
#90102=DIRECTION('',(0.,-0.707106781186548,0.707106781186547)) ;
#90103=DIRECTION('',(1.,0.,0.)) ;
#90104=DIRECTION('',(0.,0.707106781186548,-0.707106781186547)) ;
#90105=DIRECTION('center_axis',(1.,0.,0.)) ;
#90106=DIRECTION('ref_axis',(0.,0.,-1.)) ;
#90107=DIRECTION('center_axis',(-1.,0.,0.)) ;
#90108=DIRECTION('ref_axis',(0.,1.73472347597676E-14,-1.)) ;
#90109=DIRECTION('',(1.,0.,0.)) ;
#90110=DIRECTION('center_axis',(1.,0.,0.)) ;
#90111=DIRECTION('ref_axis',(0.,0.,-1.)) ;
#90112=DIRECTION('center_axis',(0.,-1.,0.)) ;
#90113=DIRECTION('ref_axis',(0.,0.,-1.)) ;
#90114=DIRECTION('',(0.,0.,1.)) ;
#90115=DIRECTION('',(1.,0.,0.)) ;
#90116=DIRECTION('',(0.,0.,-1.)) ;
#90117=DIRECTION('center_axis',(1.,0.,0.)) ;
#90118=DIRECTION('ref_axis',(0.,0.,-1.)) ;
#90119=DIRECTION('center_axis',(1.,0.,0.)) ;
#90120=DIRECTION('ref_axis',(0.,0.,1.)) ;
#90121=DIRECTION('',(1.,0.,0.)) ;
#90122=DIRECTION('center_axis',(-1.,0.,0.)) ;
#90123=DIRECTION('ref_axis',(0.,0.,-1.)) ;
#90124=DIRECTION('center_axis',(0.,0.,-1.)) ;
#90125=DIRECTION('ref_axis',(-1.,0.,0.)) ;
#90126=DIRECTION('',(0.,-1.,0.)) ;
#90127=DIRECTION('',(1.,0.,0.)) ;
#90128=DIRECTION('',(0.,1.,0.)) ;
#90129=DIRECTION('center_axis',(1.,0.,0.)) ;
#90130=DIRECTION('ref_axis',(0.,0.,-1.)) ;
#90131=DIRECTION('center_axis',(1.,0.,0.)) ;
#90132=DIRECTION('ref_axis',(0.,0.,1.)) ;
#90133=DIRECTION('',(1.,0.,0.)) ;
#90134=DIRECTION('center_axis',(-1.,0.,0.)) ;
#90135=DIRECTION('ref_axis',(0.,0.,-1.)) ;
#90136=DIRECTION('center_axis',(0.,1.,0.)) ;
#90137=DIRECTION('ref_axis',(0.,0.,1.)) ;
#90138=DIRECTION('',(0.,0.,-1.)) ;
#90139=DIRECTION('',(1.,0.,0.)) ;
#90140=DIRECTION('',(0.,0.,1.)) ;
#90141=DIRECTION('center_axis',(1.,0.,0.)) ;
#90142=DIRECTION('ref_axis',(0.,0.,-1.)) ;
#90143=DIRECTION('center_axis',(-1.,0.,0.)) ;
#90144=DIRECTION('ref_axis',(0.,1.95156391047385E-14,-1.)) ;
#90145=DIRECTION('',(1.,0.,0.)) ;
#90146=DIRECTION('center_axis',(1.,0.,0.)) ;
#90147=DIRECTION('ref_axis',(0.,0.,-1.)) ;
#90148=DIRECTION('center_axis',(0.,1.07081696047951E-16,-1.)) ;
#90149=DIRECTION('ref_axis',(0.,1.,1.07081696047951E-16)) ;
#90150=DIRECTION('',(0.,-1.,-1.07081696047951E-16)) ;
#90151=DIRECTION('',(1.,0.,0.)) ;
#90152=DIRECTION('',(0.,1.,1.07081696047951E-16)) ;
#90153=DIRECTION('center_axis',(1.,0.,0.)) ;
#90154=DIRECTION('ref_axis',(0.,0.,-1.)) ;
#90155=DIRECTION('center_axis',(-1.,0.,0.)) ;
#90156=DIRECTION('ref_axis',(0.,0.,-1.)) ;
#90157=DIRECTION('',(1.,0.,0.)) ;
#90158=DIRECTION('center_axis',(1.,0.,0.)) ;
#90159=DIRECTION('ref_axis',(0.,0.,-1.)) ;
#90160=DIRECTION('center_axis',(0.,-1.,0.)) ;
#90161=DIRECTION('ref_axis',(0.,0.,-1.)) ;
#90162=DIRECTION('',(0.,0.,1.)) ;
#90163=DIRECTION('',(1.,0.,0.)) ;
#90164=DIRECTION('',(0.,0.,-1.)) ;
#90165=DIRECTION('center_axis',(1.,0.,0.)) ;
#90166=DIRECTION('ref_axis',(0.,0.,-1.)) ;
#90167=DIRECTION('center_axis',(-1.,0.,0.)) ;
#90168=DIRECTION('ref_axis',(0.,3.03576608295933E-14,-1.)) ;
#90169=DIRECTION('',(1.,0.,0.)) ;
#90170=DIRECTION('center_axis',(1.,0.,0.)) ;
#90171=DIRECTION('ref_axis',(0.,0.,-1.)) ;
#90172=DIRECTION('center_axis',(1.,0.,0.)) ;
#90173=DIRECTION('ref_axis',(0.,0.,-1.)) ;
#90174=DIRECTION('center_axis',(1.,0.,0.)) ;
#90175=DIRECTION('ref_axis',(0.,-7.85535158932895E-16,1.)) ;
#90176=DIRECTION('',(1.,0.,0.)) ;
#90177=DIRECTION('center_axis',(-1.,0.,0.)) ;
#90178=DIRECTION('ref_axis',(0.,-7.85535158932895E-16,-1.)) ;
#90179=DIRECTION('center_axis',(1.,0.,0.)) ;
#90180=DIRECTION('ref_axis',(0.,0.,-1.)) ;
#90181=DIRECTION('center_axis',(-1.,0.,0.)) ;
#90182=DIRECTION('ref_axis',(0.,3.46944695195352E-14,-1.)) ;
#90183=DIRECTION('',(1.,0.,0.)) ;
#90184=DIRECTION('center_axis',(1.,0.,0.)) ;
#90185=DIRECTION('ref_axis',(0.,0.,-1.)) ;
#90186=DIRECTION('center_axis',(0.,-1.,0.)) ;
#90187=DIRECTION('ref_axis',(0.,0.,-1.)) ;
#90188=DIRECTION('',(0.,0.,1.)) ;
#90189=DIRECTION('',(1.,0.,0.)) ;
#90190=DIRECTION('',(0.,0.,-1.)) ;
#90191=DIRECTION('center_axis',(1.,0.,0.)) ;
#90192=DIRECTION('ref_axis',(0.,0.,-1.)) ;
#90193=DIRECTION('center_axis',(-1.,0.,0.)) ;
#90194=DIRECTION('ref_axis',(0.,0.,-1.)) ;
#90195=DIRECTION('',(1.,0.,0.)) ;
#90196=DIRECTION('center_axis',(1.,0.,0.)) ;
#90197=DIRECTION('ref_axis',(0.,0.,-1.)) ;
#90198=DIRECTION('center_axis',(0.,-1.07081696047951E-16,1.)) ;
#90199=DIRECTION('ref_axis',(0.,-1.,-1.07081696047951E-16)) ;
#90200=DIRECTION('',(0.,1.,1.07081696047951E-16)) ;
#90201=DIRECTION('',(1.,0.,0.)) ;
#90202=DIRECTION('',(0.,-1.,-1.07081696047951E-16)) ;
#90203=DIRECTION('center_axis',(1.,0.,0.)) ;
#90204=DIRECTION('ref_axis',(0.,0.,-1.)) ;
#90205=DIRECTION('center_axis',(-1.,0.,0.)) ;
#90206=DIRECTION('ref_axis',(0.,0.,-1.)) ;
#90207=DIRECTION('',(1.,0.,0.)) ;
#90208=DIRECTION('center_axis',(1.,0.,0.)) ;
#90209=DIRECTION('ref_axis',(0.,0.,-1.)) ;
#90210=DIRECTION('center_axis',(0.,1.,0.)) ;
#90211=DIRECTION('ref_axis',(0.,0.,1.)) ;
#90212=DIRECTION('',(0.,0.,-1.)) ;
#90213=DIRECTION('',(0.,0.,1.)) ;
#90214=DIRECTION('center_axis',(-1.,0.,0.)) ;
#90215=DIRECTION('ref_axis',(0.,0.,1.)) ;
#90216=DIRECTION('center_axis',(-1.,0.,0.)) ;
#90217=DIRECTION('ref_axis',(0.,0.,1.)) ;
#90218=DIRECTION('',(0.,-1.,0.)) ;
#90219=DIRECTION('center_axis',(-1.,0.,0.)) ;
#90220=DIRECTION('ref_axis',(0.,0.,1.)) ;
#90221=DIRECTION('',(0.,0.,1.)) ;
#90222=DIRECTION('',(0.,-1.,-1.07081696047951E-16)) ;
#90223=DIRECTION('',(0.,0.,-1.)) ;
#90224=DIRECTION('center_axis',(-1.,0.,0.)) ;
#90225=DIRECTION('ref_axis',(0.,0.,1.)) ;
#90226=DIRECTION('',(0.,0.,-1.)) ;
#90227=DIRECTION('',(0.,1.,1.07081696047951E-16)) ;
#90228=DIRECTION('',(0.,0.,1.)) ;
#90229=DIRECTION('center_axis',(-1.,0.,0.)) ;
#90230=DIRECTION('ref_axis',(0.,0.,1.)) ;
#90231=DIRECTION('',(0.,1.,0.)) ;
#90232=DIRECTION('center_axis',(-1.,0.,0.)) ;
#90233=DIRECTION('ref_axis',(0.,0.,1.)) ;
#90234=DIRECTION('',(0.,0.,-1.)) ;
#90235=DIRECTION('',(0.,0.707106781186548,-0.707106781186547)) ;
#90236=DIRECTION('',(0.,0.,1.)) ;
#90237=DIRECTION('',(0.,-0.707106781186546,-0.707106781186549)) ;
#90238=DIRECTION('',(0.,-3.99416362155027E-15,-1.)) ;
#90239=DIRECTION('center_axis',(1.,0.,0.)) ;
#90240=DIRECTION('ref_axis',(0.,0.,-1.)) ;
#90241=DIRECTION('',(1.,0.,0.)) ;
#90242=DIRECTION('center_axis',(1.,0.,0.)) ;
#90243=DIRECTION('ref_axis',(0.,0.,1.)) ;
#90244=DIRECTION('',(1.,0.,0.)) ;
#90245=DIRECTION('center_axis',(-1.,0.,0.)) ;
#90246=DIRECTION('ref_axis',(0.,0.,-1.)) ;
#90247=DIRECTION('center_axis',(0.,0.,1.)) ;
#90248=DIRECTION('ref_axis',(1.,0.,0.)) ;
#90249=DIRECTION('',(0.,1.,0.)) ;
#90250=DIRECTION('',(1.,0.,0.)) ;
#90251=DIRECTION('',(0.,-1.,0.)) ;
#90252=DIRECTION('center_axis',(1.,0.,0.)) ;
#90253=DIRECTION('ref_axis',(0.,0.,-1.)) ;
#90254=DIRECTION('center_axis',(1.,0.,0.)) ;
#90255=DIRECTION('ref_axis',(0.,0.,1.)) ;
#90256=DIRECTION('',(1.,0.,0.)) ;
#90257=DIRECTION('center_axis',(-1.,0.,0.)) ;
#90258=DIRECTION('ref_axis',(0.,0.,-1.)) ;
#90259=DIRECTION('center_axis',(0.,-1.,3.99416362155027E-15)) ;
#90260=DIRECTION('ref_axis',(0.,-3.99416362155027E-15,-1.)) ;
#90261=DIRECTION('',(0.,3.99416362155027E-15,1.)) ;
#90262=DIRECTION('',(1.,0.,0.)) ;
#90263=DIRECTION('',(0.,-3.99416362155027E-15,-1.)) ;
#90264=DIRECTION('center_axis',(1.,0.,0.)) ;
#90265=DIRECTION('ref_axis',(0.,0.,-1.)) ;
#90266=DIRECTION('center_axis',(-1.,0.,0.)) ;
#90267=DIRECTION('ref_axis',(0.,1.30104260698261E-14,-1.)) ;
#90268=DIRECTION('',(1.,0.,0.)) ;
#90269=DIRECTION('center_axis',(1.,0.,0.)) ;
#90270=DIRECTION('ref_axis',(0.,0.,-1.)) ;
#90271=DIRECTION('center_axis',(0.,-0.707106781186549,0.707106781186546)) ;
#90272=DIRECTION('ref_axis',(0.,-0.707106781186546,-0.707106781186549)) ;
#90273=DIRECTION('',(0.,0.707106781186546,0.707106781186549)) ;
#90274=DIRECTION('',(1.,0.,0.)) ;
#90275=DIRECTION('',(0.,-0.707106781186546,-0.707106781186549)) ;
#90276=DIRECTION('center_axis',(1.,0.,0.)) ;
#90277=DIRECTION('ref_axis',(0.,0.382683432365098,0.923879532511283)) ;
#90278=DIRECTION('',(1.,0.,0.)) ;
#90279=DIRECTION('center_axis',(1.,0.,0.)) ;
#90280=DIRECTION('ref_axis',(0.,0.,-1.)) ;
#90281=DIRECTION('center_axis',(0.,1.,0.)) ;
#90282=DIRECTION('ref_axis',(0.,0.,1.)) ;
#90283=DIRECTION('',(0.,0.,-1.)) ;
#90284=DIRECTION('',(0.,0.,1.)) ;
#90285=DIRECTION('center_axis',(0.,-0.707106781186547,-0.707106781186548)) ;
#90286=DIRECTION('ref_axis',(0.,0.707106781186548,-0.707106781186547)) ;
#90287=DIRECTION('',(0.,-0.707106781186548,0.707106781186547)) ;
#90288=DIRECTION('',(1.,0.,0.)) ;
#90289=DIRECTION('',(0.,0.707106781186548,-0.707106781186547)) ;
#90290=DIRECTION('center_axis',(1.,0.,0.)) ;
#90291=DIRECTION('ref_axis',(0.,0.,-1.)) ;
#90292=DIRECTION('center_axis',(-1.,0.,0.)) ;
#90293=DIRECTION('ref_axis',(0.,1.73472347597676E-14,-1.)) ;
#90294=DIRECTION('',(1.,0.,0.)) ;
#90295=DIRECTION('center_axis',(1.,0.,0.)) ;
#90296=DIRECTION('ref_axis',(0.,0.,-1.)) ;
#90297=DIRECTION('center_axis',(0.,-1.,0.)) ;
#90298=DIRECTION('ref_axis',(0.,0.,-1.)) ;
#90299=DIRECTION('',(0.,0.,1.)) ;
#90300=DIRECTION('',(1.,0.,0.)) ;
#90301=DIRECTION('',(0.,0.,-1.)) ;
#90302=DIRECTION('center_axis',(1.,0.,0.)) ;
#90303=DIRECTION('ref_axis',(0.,0.,-1.)) ;
#90304=DIRECTION('center_axis',(1.,0.,0.)) ;
#90305=DIRECTION('ref_axis',(0.,0.,1.)) ;
#90306=DIRECTION('',(1.,0.,0.)) ;
#90307=DIRECTION('center_axis',(-1.,0.,0.)) ;
#90308=DIRECTION('ref_axis',(0.,0.,-1.)) ;
#90309=DIRECTION('center_axis',(0.,0.,-1.)) ;
#90310=DIRECTION('ref_axis',(-1.,0.,0.)) ;
#90311=DIRECTION('',(0.,-1.,0.)) ;
#90312=DIRECTION('',(1.,0.,0.)) ;
#90313=DIRECTION('',(0.,1.,0.)) ;
#90314=DIRECTION('center_axis',(1.,0.,0.)) ;
#90315=DIRECTION('ref_axis',(0.,0.,-1.)) ;
#90316=DIRECTION('center_axis',(1.,0.,0.)) ;
#90317=DIRECTION('ref_axis',(0.,0.,1.)) ;
#90318=DIRECTION('',(1.,0.,0.)) ;
#90319=DIRECTION('center_axis',(-1.,0.,0.)) ;
#90320=DIRECTION('ref_axis',(0.,0.,-1.)) ;
#90321=DIRECTION('center_axis',(0.,1.,0.)) ;
#90322=DIRECTION('ref_axis',(0.,0.,1.)) ;
#90323=DIRECTION('',(0.,0.,-1.)) ;
#90324=DIRECTION('',(1.,0.,0.)) ;
#90325=DIRECTION('',(0.,0.,1.)) ;
#90326=DIRECTION('center_axis',(1.,0.,0.)) ;
#90327=DIRECTION('ref_axis',(0.,0.,-1.)) ;
#90328=DIRECTION('center_axis',(-1.,0.,0.)) ;
#90329=DIRECTION('ref_axis',(0.,1.95156391047385E-14,-1.)) ;
#90330=DIRECTION('',(1.,0.,0.)) ;
#90331=DIRECTION('center_axis',(1.,0.,0.)) ;
#90332=DIRECTION('ref_axis',(0.,0.,-1.)) ;
#90333=DIRECTION('center_axis',(0.,1.07081696047951E-16,-1.)) ;
#90334=DIRECTION('ref_axis',(0.,1.,1.07081696047951E-16)) ;
#90335=DIRECTION('',(0.,-1.,-1.07081696047951E-16)) ;
#90336=DIRECTION('',(1.,0.,0.)) ;
#90337=DIRECTION('',(0.,1.,1.07081696047951E-16)) ;
#90338=DIRECTION('center_axis',(1.,0.,0.)) ;
#90339=DIRECTION('ref_axis',(0.,0.,-1.)) ;
#90340=DIRECTION('center_axis',(-1.,0.,0.)) ;
#90341=DIRECTION('ref_axis',(0.,0.,-1.)) ;
#90342=DIRECTION('',(1.,0.,0.)) ;
#90343=DIRECTION('center_axis',(1.,0.,0.)) ;
#90344=DIRECTION('ref_axis',(0.,0.,-1.)) ;
#90345=DIRECTION('center_axis',(0.,-1.,0.)) ;
#90346=DIRECTION('ref_axis',(0.,0.,-1.)) ;
#90347=DIRECTION('',(0.,0.,1.)) ;
#90348=DIRECTION('',(1.,0.,0.)) ;
#90349=DIRECTION('',(0.,0.,-1.)) ;
#90350=DIRECTION('center_axis',(1.,0.,0.)) ;
#90351=DIRECTION('ref_axis',(0.,0.,-1.)) ;
#90352=DIRECTION('center_axis',(-1.,0.,0.)) ;
#90353=DIRECTION('ref_axis',(0.,3.03576608295933E-14,-1.)) ;
#90354=DIRECTION('',(1.,0.,0.)) ;
#90355=DIRECTION('center_axis',(1.,0.,0.)) ;
#90356=DIRECTION('ref_axis',(0.,0.,-1.)) ;
#90357=DIRECTION('center_axis',(1.,0.,0.)) ;
#90358=DIRECTION('ref_axis',(0.,0.,-1.)) ;
#90359=DIRECTION('center_axis',(1.,0.,0.)) ;
#90360=DIRECTION('ref_axis',(0.,-7.85535158932895E-16,1.)) ;
#90361=DIRECTION('',(1.,0.,0.)) ;
#90362=DIRECTION('center_axis',(-1.,0.,0.)) ;
#90363=DIRECTION('ref_axis',(0.,-7.85535158932895E-16,-1.)) ;
#90364=DIRECTION('center_axis',(1.,0.,0.)) ;
#90365=DIRECTION('ref_axis',(0.,0.,-1.)) ;
#90366=DIRECTION('center_axis',(-1.,0.,0.)) ;
#90367=DIRECTION('ref_axis',(0.,4.33680868994204E-15,-1.)) ;
#90368=DIRECTION('',(1.,0.,0.)) ;
#90369=DIRECTION('center_axis',(1.,0.,0.)) ;
#90370=DIRECTION('ref_axis',(0.,0.,-1.)) ;
#90371=DIRECTION('center_axis',(0.,-1.,0.)) ;
#90372=DIRECTION('ref_axis',(0.,0.,-1.)) ;
#90373=DIRECTION('',(0.,0.,1.)) ;
#90374=DIRECTION('',(1.,0.,0.)) ;
#90375=DIRECTION('',(0.,0.,-1.)) ;
#90376=DIRECTION('center_axis',(1.,0.,0.)) ;
#90377=DIRECTION('ref_axis',(0.,0.,-1.)) ;
#90378=DIRECTION('center_axis',(-1.,0.,0.)) ;
#90379=DIRECTION('ref_axis',(0.,0.,-1.)) ;
#90380=DIRECTION('',(1.,0.,0.)) ;
#90381=DIRECTION('center_axis',(1.,0.,0.)) ;
#90382=DIRECTION('ref_axis',(0.,0.,-1.)) ;
#90383=DIRECTION('center_axis',(0.,-1.07081696047951E-16,1.)) ;
#90384=DIRECTION('ref_axis',(0.,-1.,-1.07081696047951E-16)) ;
#90385=DIRECTION('',(0.,1.,1.07081696047951E-16)) ;
#90386=DIRECTION('',(1.,0.,0.)) ;
#90387=DIRECTION('',(0.,-1.,-1.07081696047951E-16)) ;
#90388=DIRECTION('center_axis',(1.,0.,0.)) ;
#90389=DIRECTION('ref_axis',(0.,0.,-1.)) ;
#90390=DIRECTION('center_axis',(-1.,0.,0.)) ;
#90391=DIRECTION('ref_axis',(0.,0.,-1.)) ;
#90392=DIRECTION('',(1.,0.,0.)) ;
#90393=DIRECTION('center_axis',(1.,0.,0.)) ;
#90394=DIRECTION('ref_axis',(0.,0.,-1.)) ;
#90395=DIRECTION('center_axis',(0.,1.,0.)) ;
#90396=DIRECTION('ref_axis',(0.,0.,1.)) ;
#90397=DIRECTION('',(0.,0.,-1.)) ;
#90398=DIRECTION('',(0.,0.,1.)) ;
#90399=DIRECTION('center_axis',(-1.,0.,0.)) ;
#90400=DIRECTION('ref_axis',(0.,0.,1.)) ;
#90401=DIRECTION('center_axis',(-1.,0.,0.)) ;
#90402=DIRECTION('ref_axis',(0.,0.,1.)) ;
#90403=DIRECTION('',(0.,-1.,0.)) ;
#90404=DIRECTION('center_axis',(-1.,0.,0.)) ;
#90405=DIRECTION('ref_axis',(0.,0.,1.)) ;
#90406=DIRECTION('',(0.,0.,1.)) ;
#90407=DIRECTION('',(0.,-1.,-1.07081696047951E-16)) ;
#90408=DIRECTION('',(0.,0.,-1.)) ;
#90409=DIRECTION('center_axis',(-1.,0.,0.)) ;
#90410=DIRECTION('ref_axis',(0.,0.,1.)) ;
#90411=DIRECTION('',(0.,0.,-1.)) ;
#90412=DIRECTION('',(0.,1.,1.07081696047951E-16)) ;
#90413=DIRECTION('',(0.,0.,1.)) ;
#90414=DIRECTION('center_axis',(-1.,0.,0.)) ;
#90415=DIRECTION('ref_axis',(0.,0.,1.)) ;
#90416=DIRECTION('',(0.,1.,0.)) ;
#90417=DIRECTION('center_axis',(-1.,0.,0.)) ;
#90418=DIRECTION('ref_axis',(0.,0.,1.)) ;
#90419=DIRECTION('',(0.,0.,-1.)) ;
#90420=DIRECTION('',(0.,0.707106781186548,-0.707106781186547)) ;
#90421=DIRECTION('',(0.,0.,1.)) ;
#90422=DIRECTION('',(0.,-0.707106781186546,-0.707106781186549)) ;
#90423=DIRECTION('',(0.,-3.99416362155027E-15,-1.)) ;
#90424=DIRECTION('center_axis',(1.,0.,0.)) ;
#90425=DIRECTION('ref_axis',(0.,0.,-1.)) ;
#90426=DIRECTION('',(1.,0.,0.)) ;
#90427=DIRECTION('center_axis',(1.,0.,0.)) ;
#90428=DIRECTION('ref_axis',(0.,0.,1.)) ;
#90429=DIRECTION('',(1.,0.,0.)) ;
#90430=DIRECTION('center_axis',(-1.,0.,0.)) ;
#90431=DIRECTION('ref_axis',(0.,0.,-1.)) ;
#90432=DIRECTION('center_axis',(0.,0.,1.)) ;
#90433=DIRECTION('ref_axis',(1.,0.,0.)) ;
#90434=DIRECTION('',(0.,1.,0.)) ;
#90435=DIRECTION('',(1.,0.,0.)) ;
#90436=DIRECTION('',(0.,-1.,0.)) ;
#90437=DIRECTION('center_axis',(1.,0.,0.)) ;
#90438=DIRECTION('ref_axis',(0.,0.,-1.)) ;
#90439=DIRECTION('center_axis',(1.,0.,0.)) ;
#90440=DIRECTION('ref_axis',(0.,0.,1.)) ;
#90441=DIRECTION('',(1.,0.,0.)) ;
#90442=DIRECTION('center_axis',(-1.,0.,0.)) ;
#90443=DIRECTION('ref_axis',(0.,0.,-1.)) ;
#90444=DIRECTION('center_axis',(0.,-1.,3.99416362155027E-15)) ;
#90445=DIRECTION('ref_axis',(0.,-3.99416362155027E-15,-1.)) ;
#90446=DIRECTION('',(0.,3.99416362155027E-15,1.)) ;
#90447=DIRECTION('',(1.,0.,0.)) ;
#90448=DIRECTION('',(0.,-3.99416362155027E-15,-1.)) ;
#90449=DIRECTION('center_axis',(1.,0.,0.)) ;
#90450=DIRECTION('ref_axis',(0.,0.,-1.)) ;
#90451=DIRECTION('center_axis',(-1.,0.,0.)) ;
#90452=DIRECTION('ref_axis',(0.,1.30104260698261E-14,-1.)) ;
#90453=DIRECTION('',(1.,0.,0.)) ;
#90454=DIRECTION('center_axis',(1.,0.,0.)) ;
#90455=DIRECTION('ref_axis',(0.,0.,-1.)) ;
#90456=DIRECTION('center_axis',(0.,-0.707106781186549,0.707106781186546)) ;
#90457=DIRECTION('ref_axis',(0.,-0.707106781186546,-0.707106781186549)) ;
#90458=DIRECTION('',(0.,0.707106781186546,0.707106781186549)) ;
#90459=DIRECTION('',(1.,0.,0.)) ;
#90460=DIRECTION('',(0.,-0.707106781186546,-0.707106781186549)) ;
#90461=DIRECTION('center_axis',(1.,0.,0.)) ;
#90462=DIRECTION('ref_axis',(0.,0.382683432365098,0.923879532511283)) ;
#90463=DIRECTION('',(1.,0.,0.)) ;
#90464=DIRECTION('center_axis',(1.,0.,0.)) ;
#90465=DIRECTION('ref_axis',(0.,0.,-1.)) ;
#90466=DIRECTION('center_axis',(0.,1.,0.)) ;
#90467=DIRECTION('ref_axis',(0.,0.,1.)) ;
#90468=DIRECTION('',(0.,0.,-1.)) ;
#90469=DIRECTION('',(0.,0.,1.)) ;
#90470=DIRECTION('center_axis',(0.,-0.707106781186547,-0.707106781186548)) ;
#90471=DIRECTION('ref_axis',(0.,0.707106781186548,-0.707106781186547)) ;
#90472=DIRECTION('',(0.,-0.707106781186548,0.707106781186547)) ;
#90473=DIRECTION('',(1.,0.,0.)) ;
#90474=DIRECTION('',(0.,0.707106781186548,-0.707106781186547)) ;
#90475=DIRECTION('center_axis',(1.,0.,0.)) ;
#90476=DIRECTION('ref_axis',(0.,0.,-1.)) ;
#90477=DIRECTION('center_axis',(-1.,0.,0.)) ;
#90478=DIRECTION('ref_axis',(0.,-1.73472347597682E-14,-1.)) ;
#90479=DIRECTION('',(1.,0.,0.)) ;
#90480=DIRECTION('center_axis',(1.,0.,0.)) ;
#90481=DIRECTION('ref_axis',(0.,0.,-1.)) ;
#90482=DIRECTION('center_axis',(0.,-1.,0.)) ;
#90483=DIRECTION('ref_axis',(0.,0.,-1.)) ;
#90484=DIRECTION('',(0.,0.,1.)) ;
#90485=DIRECTION('',(1.,0.,0.)) ;
#90486=DIRECTION('',(0.,0.,-1.)) ;
#90487=DIRECTION('center_axis',(1.,0.,0.)) ;
#90488=DIRECTION('ref_axis',(0.,0.,-1.)) ;
#90489=DIRECTION('center_axis',(1.,0.,0.)) ;
#90490=DIRECTION('ref_axis',(0.,0.,1.)) ;
#90491=DIRECTION('',(1.,0.,0.)) ;
#90492=DIRECTION('center_axis',(-1.,0.,0.)) ;
#90493=DIRECTION('ref_axis',(0.,0.,-1.)) ;
#90494=DIRECTION('center_axis',(0.,0.,-1.)) ;
#90495=DIRECTION('ref_axis',(-1.,0.,0.)) ;
#90496=DIRECTION('',(0.,-1.,0.)) ;
#90497=DIRECTION('',(1.,0.,0.)) ;
#90498=DIRECTION('',(0.,1.,0.)) ;
#90499=DIRECTION('center_axis',(1.,0.,0.)) ;
#90500=DIRECTION('ref_axis',(0.,0.,-1.)) ;
#90501=DIRECTION('center_axis',(1.,0.,0.)) ;
#90502=DIRECTION('ref_axis',(0.,0.,1.)) ;
#90503=DIRECTION('',(1.,0.,0.)) ;
#90504=DIRECTION('center_axis',(-1.,0.,0.)) ;
#90505=DIRECTION('ref_axis',(0.,0.,-1.)) ;
#90506=DIRECTION('center_axis',(0.,1.,0.)) ;
#90507=DIRECTION('ref_axis',(0.,0.,1.)) ;
#90508=DIRECTION('',(0.,0.,-1.)) ;
#90509=DIRECTION('',(1.,0.,0.)) ;
#90510=DIRECTION('',(0.,0.,1.)) ;
#90511=DIRECTION('center_axis',(1.,0.,0.)) ;
#90512=DIRECTION('ref_axis',(0.,0.,-1.)) ;
#90513=DIRECTION('center_axis',(-1.,0.,0.)) ;
#90514=DIRECTION('ref_axis',(0.,1.95156391047392E-14,-1.)) ;
#90515=DIRECTION('',(1.,0.,0.)) ;
#90516=DIRECTION('center_axis',(1.,0.,0.)) ;
#90517=DIRECTION('ref_axis',(0.,0.,-1.)) ;
#90518=DIRECTION('center_axis',(0.,1.07081696047951E-16,-1.)) ;
#90519=DIRECTION('ref_axis',(0.,1.,1.07081696047951E-16)) ;
#90520=DIRECTION('',(0.,-1.,-1.07081696047951E-16)) ;
#90521=DIRECTION('',(1.,0.,0.)) ;
#90522=DIRECTION('',(0.,1.,1.07081696047951E-16)) ;
#90523=DIRECTION('center_axis',(1.,0.,0.)) ;
#90524=DIRECTION('ref_axis',(0.,0.,-1.)) ;
#90525=DIRECTION('center_axis',(-1.,0.,0.)) ;
#90526=DIRECTION('ref_axis',(0.,0.,-1.)) ;
#90527=DIRECTION('',(1.,0.,0.)) ;
#90528=DIRECTION('center_axis',(1.,0.,0.)) ;
#90529=DIRECTION('ref_axis',(0.,0.,-1.)) ;
#90530=DIRECTION('center_axis',(0.,-1.,0.)) ;
#90531=DIRECTION('ref_axis',(0.,0.,-1.)) ;
#90532=DIRECTION('',(0.,0.,1.)) ;
#90533=DIRECTION('',(1.,0.,0.)) ;
#90534=DIRECTION('',(0.,0.,-1.)) ;
#90535=DIRECTION('center_axis',(1.,0.,0.)) ;
#90536=DIRECTION('ref_axis',(0.,0.,-1.)) ;
#90537=DIRECTION('center_axis',(-1.,0.,0.)) ;
#90538=DIRECTION('ref_axis',(0.,4.33680868994204E-15,-1.)) ;
#90539=DIRECTION('',(1.,0.,0.)) ;
#90540=DIRECTION('center_axis',(1.,0.,0.)) ;
#90541=DIRECTION('ref_axis',(0.,0.,-1.)) ;
#90542=DIRECTION('center_axis',(1.,0.,0.)) ;
#90543=DIRECTION('ref_axis',(0.,0.,-1.)) ;
#90544=DIRECTION('center_axis',(1.,0.,0.)) ;
#90545=DIRECTION('ref_axis',(0.,-7.85535158932895E-16,1.)) ;
#90546=DIRECTION('',(1.,0.,0.)) ;
#90547=DIRECTION('center_axis',(-1.,0.,0.)) ;
#90548=DIRECTION('ref_axis',(0.,-7.85535158932895E-16,-1.)) ;
#90549=DIRECTION('center_axis',(1.,0.,0.)) ;
#90550=DIRECTION('ref_axis',(0.,0.,-1.)) ;
#90551=DIRECTION('center_axis',(-1.,0.,0.)) ;
#90552=DIRECTION('ref_axis',(0.,4.33680868994204E-15,-1.)) ;
#90553=DIRECTION('',(1.,0.,0.)) ;
#90554=DIRECTION('center_axis',(1.,0.,0.)) ;
#90555=DIRECTION('ref_axis',(0.,0.,-1.)) ;
#90556=DIRECTION('center_axis',(0.,-1.,0.)) ;
#90557=DIRECTION('ref_axis',(0.,0.,-1.)) ;
#90558=DIRECTION('',(0.,0.,1.)) ;
#90559=DIRECTION('',(1.,0.,0.)) ;
#90560=DIRECTION('',(0.,0.,-1.)) ;
#90561=DIRECTION('center_axis',(1.,0.,0.)) ;
#90562=DIRECTION('ref_axis',(0.,0.,-1.)) ;
#90563=DIRECTION('center_axis',(-1.,0.,0.)) ;
#90564=DIRECTION('ref_axis',(0.,0.,-1.)) ;
#90565=DIRECTION('',(1.,0.,0.)) ;
#90566=DIRECTION('center_axis',(1.,0.,0.)) ;
#90567=DIRECTION('ref_axis',(0.,0.,-1.)) ;
#90568=DIRECTION('center_axis',(0.,-1.07081696047951E-16,1.)) ;
#90569=DIRECTION('ref_axis',(0.,-1.,-1.07081696047951E-16)) ;
#90570=DIRECTION('',(0.,1.,1.07081696047951E-16)) ;
#90571=DIRECTION('',(1.,0.,0.)) ;
#90572=DIRECTION('',(0.,-1.,-1.07081696047951E-16)) ;
#90573=DIRECTION('center_axis',(1.,0.,0.)) ;
#90574=DIRECTION('ref_axis',(0.,0.,-1.)) ;
#90575=DIRECTION('center_axis',(-1.,0.,0.)) ;
#90576=DIRECTION('ref_axis',(0.,0.,-1.)) ;
#90577=DIRECTION('',(1.,0.,0.)) ;
#90578=DIRECTION('center_axis',(1.,0.,0.)) ;
#90579=DIRECTION('ref_axis',(0.,0.,-1.)) ;
#90580=DIRECTION('center_axis',(0.,1.,0.)) ;
#90581=DIRECTION('ref_axis',(0.,0.,1.)) ;
#90582=DIRECTION('',(0.,0.,-1.)) ;
#90583=DIRECTION('',(0.,0.,1.)) ;
#90584=DIRECTION('center_axis',(-1.,0.,0.)) ;
#90585=DIRECTION('ref_axis',(0.,0.,1.)) ;
#90586=DIRECTION('center_axis',(-1.,0.,0.)) ;
#90587=DIRECTION('ref_axis',(0.,0.,1.)) ;
#90588=DIRECTION('',(0.,-1.,0.)) ;
#90589=DIRECTION('center_axis',(-1.,0.,0.)) ;
#90590=DIRECTION('ref_axis',(0.,0.,1.)) ;
#90591=DIRECTION('',(0.,0.,1.)) ;
#90592=DIRECTION('',(0.,-1.,-1.07081696047951E-16)) ;
#90593=DIRECTION('',(0.,0.,-1.)) ;
#90594=DIRECTION('center_axis',(-1.,0.,0.)) ;
#90595=DIRECTION('ref_axis',(0.,0.,1.)) ;
#90596=DIRECTION('',(0.,0.,-1.)) ;
#90597=DIRECTION('',(0.,1.,1.07081696047951E-16)) ;
#90598=DIRECTION('',(0.,0.,1.)) ;
#90599=DIRECTION('center_axis',(-1.,0.,0.)) ;
#90600=DIRECTION('ref_axis',(0.,0.,1.)) ;
#90601=DIRECTION('',(0.,1.,0.)) ;
#90602=DIRECTION('center_axis',(-1.,0.,0.)) ;
#90603=DIRECTION('ref_axis',(0.,0.,1.)) ;
#90604=DIRECTION('',(0.,0.,-1.)) ;
#90605=DIRECTION('',(0.,0.707106781186548,-0.707106781186547)) ;
#90606=DIRECTION('',(0.,0.,1.)) ;
#90607=DIRECTION('',(0.,-0.707106781186546,-0.707106781186549)) ;
#90608=DIRECTION('',(0.,-3.99416362155027E-15,-1.)) ;
#90609=DIRECTION('center_axis',(1.,0.,0.)) ;
#90610=DIRECTION('ref_axis',(0.,0.,-1.)) ;
#90611=DIRECTION('',(1.,0.,0.)) ;
#90612=DIRECTION('center_axis',(1.,0.,0.)) ;
#90613=DIRECTION('ref_axis',(0.,0.,1.)) ;
#90614=DIRECTION('',(1.,0.,0.)) ;
#90615=DIRECTION('center_axis',(-1.,0.,0.)) ;
#90616=DIRECTION('ref_axis',(0.,0.,-1.)) ;
#90617=DIRECTION('center_axis',(0.,0.,1.)) ;
#90618=DIRECTION('ref_axis',(1.,0.,0.)) ;
#90619=DIRECTION('',(0.,1.,0.)) ;
#90620=DIRECTION('',(1.,0.,0.)) ;
#90621=DIRECTION('',(0.,-1.,0.)) ;
#90622=DIRECTION('center_axis',(1.,0.,0.)) ;
#90623=DIRECTION('ref_axis',(0.,0.,-1.)) ;
#90624=DIRECTION('center_axis',(1.,0.,0.)) ;
#90625=DIRECTION('ref_axis',(0.,0.,1.)) ;
#90626=DIRECTION('',(1.,0.,0.)) ;
#90627=DIRECTION('center_axis',(-1.,0.,0.)) ;
#90628=DIRECTION('ref_axis',(0.,0.,-1.)) ;
#90629=DIRECTION('center_axis',(0.,-1.,3.99416362155027E-15)) ;
#90630=DIRECTION('ref_axis',(0.,-3.99416362155027E-15,-1.)) ;
#90631=DIRECTION('',(0.,3.99416362155027E-15,1.)) ;
#90632=DIRECTION('',(1.,0.,0.)) ;
#90633=DIRECTION('',(0.,-3.99416362155027E-15,-1.)) ;
#90634=DIRECTION('center_axis',(1.,0.,0.)) ;
#90635=DIRECTION('ref_axis',(0.,0.,-1.)) ;
#90636=DIRECTION('center_axis',(-1.,0.,0.)) ;
#90637=DIRECTION('ref_axis',(0.,1.30104260698261E-14,-1.)) ;
#90638=DIRECTION('',(1.,0.,0.)) ;
#90639=DIRECTION('center_axis',(1.,0.,0.)) ;
#90640=DIRECTION('ref_axis',(0.,0.,-1.)) ;
#90641=DIRECTION('center_axis',(0.,-0.707106781186549,0.707106781186546)) ;
#90642=DIRECTION('ref_axis',(0.,-0.707106781186546,-0.707106781186549)) ;
#90643=DIRECTION('',(0.,0.707106781186546,0.707106781186549)) ;
#90644=DIRECTION('',(1.,0.,0.)) ;
#90645=DIRECTION('',(0.,-0.707106781186546,-0.707106781186549)) ;
#90646=DIRECTION('center_axis',(1.,0.,0.)) ;
#90647=DIRECTION('ref_axis',(0.,0.382683432365098,0.923879532511283)) ;
#90648=DIRECTION('',(1.,0.,0.)) ;
#90649=DIRECTION('center_axis',(1.,0.,0.)) ;
#90650=DIRECTION('ref_axis',(0.,0.,-1.)) ;
#90651=DIRECTION('center_axis',(0.,1.,0.)) ;
#90652=DIRECTION('ref_axis',(0.,0.,1.)) ;
#90653=DIRECTION('',(0.,0.,-1.)) ;
#90654=DIRECTION('',(0.,0.,1.)) ;
#90655=DIRECTION('center_axis',(0.,-0.707106781186547,-0.707106781186548)) ;
#90656=DIRECTION('ref_axis',(0.,0.707106781186548,-0.707106781186547)) ;
#90657=DIRECTION('',(0.,-0.707106781186548,0.707106781186547)) ;
#90658=DIRECTION('',(1.,0.,0.)) ;
#90659=DIRECTION('',(0.,0.707106781186548,-0.707106781186547)) ;
#90660=DIRECTION('center_axis',(1.,0.,0.)) ;
#90661=DIRECTION('ref_axis',(0.,0.,-1.)) ;
#90662=DIRECTION('center_axis',(-1.,0.,0.)) ;
#90663=DIRECTION('ref_axis',(0.,-1.73472347597682E-14,-1.)) ;
#90664=DIRECTION('',(1.,0.,0.)) ;
#90665=DIRECTION('center_axis',(1.,0.,0.)) ;
#90666=DIRECTION('ref_axis',(0.,0.,-1.)) ;
#90667=DIRECTION('center_axis',(0.,-1.,0.)) ;
#90668=DIRECTION('ref_axis',(0.,0.,-1.)) ;
#90669=DIRECTION('',(0.,0.,1.)) ;
#90670=DIRECTION('',(1.,0.,0.)) ;
#90671=DIRECTION('',(0.,0.,-1.)) ;
#90672=DIRECTION('center_axis',(1.,0.,0.)) ;
#90673=DIRECTION('ref_axis',(0.,0.,-1.)) ;
#90674=DIRECTION('center_axis',(1.,0.,0.)) ;
#90675=DIRECTION('ref_axis',(0.,0.,1.)) ;
#90676=DIRECTION('',(1.,0.,0.)) ;
#90677=DIRECTION('center_axis',(-1.,0.,0.)) ;
#90678=DIRECTION('ref_axis',(0.,0.,-1.)) ;
#90679=DIRECTION('center_axis',(0.,0.,-1.)) ;
#90680=DIRECTION('ref_axis',(-1.,0.,0.)) ;
#90681=DIRECTION('',(0.,-1.,0.)) ;
#90682=DIRECTION('',(1.,0.,0.)) ;
#90683=DIRECTION('',(0.,1.,0.)) ;
#90684=DIRECTION('center_axis',(1.,0.,0.)) ;
#90685=DIRECTION('ref_axis',(0.,0.,-1.)) ;
#90686=DIRECTION('center_axis',(1.,0.,0.)) ;
#90687=DIRECTION('ref_axis',(0.,0.,1.)) ;
#90688=DIRECTION('',(1.,0.,0.)) ;
#90689=DIRECTION('center_axis',(-1.,0.,0.)) ;
#90690=DIRECTION('ref_axis',(0.,0.,-1.)) ;
#90691=DIRECTION('center_axis',(0.,1.,0.)) ;
#90692=DIRECTION('ref_axis',(0.,0.,1.)) ;
#90693=DIRECTION('',(0.,0.,-1.)) ;
#90694=DIRECTION('',(1.,0.,0.)) ;
#90695=DIRECTION('',(0.,0.,1.)) ;
#90696=DIRECTION('center_axis',(1.,0.,0.)) ;
#90697=DIRECTION('ref_axis',(0.,0.,-1.)) ;
#90698=DIRECTION('center_axis',(-1.,0.,0.)) ;
#90699=DIRECTION('ref_axis',(0.,1.95156391047392E-14,-1.)) ;
#90700=DIRECTION('',(1.,0.,0.)) ;
#90701=DIRECTION('center_axis',(1.,0.,0.)) ;
#90702=DIRECTION('ref_axis',(0.,0.,-1.)) ;
#90703=DIRECTION('center_axis',(0.,1.07081696047951E-16,-1.)) ;
#90704=DIRECTION('ref_axis',(0.,1.,1.07081696047951E-16)) ;
#90705=DIRECTION('',(0.,-1.,-1.07081696047951E-16)) ;
#90706=DIRECTION('',(1.,0.,0.)) ;
#90707=DIRECTION('',(0.,1.,1.07081696047951E-16)) ;
#90708=DIRECTION('center_axis',(1.,0.,0.)) ;
#90709=DIRECTION('ref_axis',(0.,0.,-1.)) ;
#90710=DIRECTION('center_axis',(-1.,0.,0.)) ;
#90711=DIRECTION('ref_axis',(0.,0.,-1.)) ;
#90712=DIRECTION('',(1.,0.,0.)) ;
#90713=DIRECTION('center_axis',(1.,0.,0.)) ;
#90714=DIRECTION('ref_axis',(0.,0.,-1.)) ;
#90715=DIRECTION('center_axis',(0.,-1.,0.)) ;
#90716=DIRECTION('ref_axis',(0.,0.,-1.)) ;
#90717=DIRECTION('',(0.,0.,1.)) ;
#90718=DIRECTION('',(1.,0.,0.)) ;
#90719=DIRECTION('',(0.,0.,-1.)) ;
#90720=DIRECTION('center_axis',(1.,0.,0.)) ;
#90721=DIRECTION('ref_axis',(0.,0.,-1.)) ;
#90722=DIRECTION('center_axis',(-1.,0.,0.)) ;
#90723=DIRECTION('ref_axis',(0.,4.33680868994204E-15,-1.)) ;
#90724=DIRECTION('',(1.,0.,0.)) ;
#90725=DIRECTION('center_axis',(1.,0.,0.)) ;
#90726=DIRECTION('ref_axis',(0.,0.,-1.)) ;
#90727=DIRECTION('center_axis',(1.,0.,0.)) ;
#90728=DIRECTION('ref_axis',(0.,0.,-1.)) ;
#90729=DIRECTION('center_axis',(1.,0.,0.)) ;
#90730=DIRECTION('ref_axis',(0.,-7.85535158932895E-16,1.)) ;
#90731=DIRECTION('',(1.,0.,0.)) ;
#90732=DIRECTION('center_axis',(-1.,0.,0.)) ;
#90733=DIRECTION('ref_axis',(0.,-7.85535158932895E-16,-1.)) ;
#90734=DIRECTION('center_axis',(1.,0.,0.)) ;
#90735=DIRECTION('ref_axis',(0.,0.,-1.)) ;
#90736=DIRECTION('center_axis',(-1.,0.,0.)) ;
#90737=DIRECTION('ref_axis',(0.,4.33680868994204E-15,-1.)) ;
#90738=DIRECTION('',(1.,0.,0.)) ;
#90739=DIRECTION('center_axis',(1.,0.,0.)) ;
#90740=DIRECTION('ref_axis',(0.,0.,-1.)) ;
#90741=DIRECTION('center_axis',(0.,-1.,0.)) ;
#90742=DIRECTION('ref_axis',(0.,0.,-1.)) ;
#90743=DIRECTION('',(0.,0.,1.)) ;
#90744=DIRECTION('',(1.,0.,0.)) ;
#90745=DIRECTION('',(0.,0.,-1.)) ;
#90746=DIRECTION('center_axis',(1.,0.,0.)) ;
#90747=DIRECTION('ref_axis',(0.,0.,-1.)) ;
#90748=DIRECTION('center_axis',(-1.,0.,0.)) ;
#90749=DIRECTION('ref_axis',(0.,0.,-1.)) ;
#90750=DIRECTION('',(1.,0.,0.)) ;
#90751=DIRECTION('center_axis',(1.,0.,0.)) ;
#90752=DIRECTION('ref_axis',(0.,0.,-1.)) ;
#90753=DIRECTION('center_axis',(0.,-1.07081696047951E-16,1.)) ;
#90754=DIRECTION('ref_axis',(0.,-1.,-1.07081696047951E-16)) ;
#90755=DIRECTION('',(0.,1.,1.07081696047951E-16)) ;
#90756=DIRECTION('',(1.,0.,0.)) ;
#90757=DIRECTION('',(0.,-1.,-1.07081696047951E-16)) ;
#90758=DIRECTION('center_axis',(1.,0.,0.)) ;
#90759=DIRECTION('ref_axis',(0.,0.,-1.)) ;
#90760=DIRECTION('center_axis',(-1.,0.,0.)) ;
#90761=DIRECTION('ref_axis',(0.,0.,-1.)) ;
#90762=DIRECTION('',(1.,0.,0.)) ;
#90763=DIRECTION('center_axis',(1.,0.,0.)) ;
#90764=DIRECTION('ref_axis',(0.,0.,-1.)) ;
#90765=DIRECTION('center_axis',(0.,1.,0.)) ;
#90766=DIRECTION('ref_axis',(0.,0.,1.)) ;
#90767=DIRECTION('',(0.,0.,-1.)) ;
#90768=DIRECTION('',(0.,0.,1.)) ;
#90769=DIRECTION('center_axis',(-1.,0.,0.)) ;
#90770=DIRECTION('ref_axis',(0.,0.,1.)) ;
#90771=DIRECTION('center_axis',(-1.,0.,0.)) ;
#90772=DIRECTION('ref_axis',(0.,0.,1.)) ;
#90773=DIRECTION('',(0.,-1.,0.)) ;
#90774=DIRECTION('center_axis',(-1.,0.,0.)) ;
#90775=DIRECTION('ref_axis',(0.,0.,1.)) ;
#90776=DIRECTION('',(0.,0.,1.)) ;
#90777=DIRECTION('',(0.,-1.,-1.07081696047951E-16)) ;
#90778=DIRECTION('',(0.,0.,-1.)) ;
#90779=DIRECTION('center_axis',(-1.,0.,0.)) ;
#90780=DIRECTION('ref_axis',(0.,0.,1.)) ;
#90781=DIRECTION('',(0.,0.,-1.)) ;
#90782=DIRECTION('',(0.,1.,1.07081696047951E-16)) ;
#90783=DIRECTION('',(0.,0.,1.)) ;
#90784=DIRECTION('center_axis',(-1.,0.,0.)) ;
#90785=DIRECTION('ref_axis',(0.,0.,1.)) ;
#90786=DIRECTION('',(0.,1.,0.)) ;
#90787=DIRECTION('center_axis',(-1.,0.,0.)) ;
#90788=DIRECTION('ref_axis',(0.,0.,1.)) ;
#90789=DIRECTION('',(0.,0.,-1.)) ;
#90790=DIRECTION('',(0.,0.707106781186548,-0.707106781186547)) ;
#90791=DIRECTION('',(0.,0.,1.)) ;
#90792=DIRECTION('',(0.,-0.707106781186546,-0.707106781186549)) ;
#90793=DIRECTION('',(0.,-3.99416362155027E-15,-1.)) ;
#90794=DIRECTION('center_axis',(1.,0.,0.)) ;
#90795=DIRECTION('ref_axis',(0.,0.,-1.)) ;
#90796=DIRECTION('',(1.,0.,0.)) ;
#90797=DIRECTION('center_axis',(1.,0.,0.)) ;
#90798=DIRECTION('ref_axis',(0.,0.,1.)) ;
#90799=DIRECTION('',(1.,0.,0.)) ;
#90800=DIRECTION('center_axis',(-1.,0.,0.)) ;
#90801=DIRECTION('ref_axis',(0.,0.,-1.)) ;
#90802=DIRECTION('center_axis',(0.,0.,1.)) ;
#90803=DIRECTION('ref_axis',(1.,0.,0.)) ;
#90804=DIRECTION('',(0.,1.,0.)) ;
#90805=DIRECTION('',(1.,0.,0.)) ;
#90806=DIRECTION('',(0.,-1.,0.)) ;
#90807=DIRECTION('center_axis',(1.,0.,0.)) ;
#90808=DIRECTION('ref_axis',(0.,0.,-1.)) ;
#90809=DIRECTION('center_axis',(1.,0.,0.)) ;
#90810=DIRECTION('ref_axis',(0.,0.,1.)) ;
#90811=DIRECTION('',(1.,0.,0.)) ;
#90812=DIRECTION('center_axis',(-1.,0.,0.)) ;
#90813=DIRECTION('ref_axis',(0.,0.,-1.)) ;
#90814=DIRECTION('center_axis',(0.,-1.,3.99416362155027E-15)) ;
#90815=DIRECTION('ref_axis',(0.,-3.99416362155027E-15,-1.)) ;
#90816=DIRECTION('',(0.,3.99416362155027E-15,1.)) ;
#90817=DIRECTION('',(1.,0.,0.)) ;
#90818=DIRECTION('',(0.,-3.99416362155027E-15,-1.)) ;
#90819=DIRECTION('center_axis',(1.,0.,0.)) ;
#90820=DIRECTION('ref_axis',(0.,0.,-1.)) ;
#90821=DIRECTION('center_axis',(-1.,0.,0.)) ;
#90822=DIRECTION('ref_axis',(0.,1.30104260698261E-14,-1.)) ;
#90823=DIRECTION('',(1.,0.,0.)) ;
#90824=DIRECTION('center_axis',(1.,0.,0.)) ;
#90825=DIRECTION('ref_axis',(0.,0.,-1.)) ;
#90826=DIRECTION('center_axis',(0.,-0.707106781186549,0.707106781186546)) ;
#90827=DIRECTION('ref_axis',(0.,-0.707106781186546,-0.707106781186549)) ;
#90828=DIRECTION('',(0.,0.707106781186546,0.707106781186549)) ;
#90829=DIRECTION('',(1.,0.,0.)) ;
#90830=DIRECTION('',(0.,-0.707106781186546,-0.707106781186549)) ;
#90831=DIRECTION('center_axis',(1.,0.,0.)) ;
#90832=DIRECTION('ref_axis',(0.,0.38268343236508,0.923879532511291)) ;
#90833=DIRECTION('',(1.,0.,0.)) ;
#90834=DIRECTION('center_axis',(1.,0.,0.)) ;
#90835=DIRECTION('ref_axis',(0.,0.,-1.)) ;
#90836=DIRECTION('center_axis',(0.,1.,0.)) ;
#90837=DIRECTION('ref_axis',(0.,0.,1.)) ;
#90838=DIRECTION('',(0.,0.,-1.)) ;
#90839=DIRECTION('',(0.,0.,1.)) ;
#90840=DIRECTION('center_axis',(0.,-0.707106781186547,-0.707106781186548)) ;
#90841=DIRECTION('ref_axis',(0.,0.707106781186548,-0.707106781186547)) ;
#90842=DIRECTION('',(0.,-0.707106781186548,0.707106781186547)) ;
#90843=DIRECTION('',(1.,0.,0.)) ;
#90844=DIRECTION('',(0.,0.707106781186548,-0.707106781186547)) ;
#90845=DIRECTION('center_axis',(1.,0.,0.)) ;
#90846=DIRECTION('ref_axis',(0.,0.,-1.)) ;
#90847=DIRECTION('center_axis',(-1.,0.,0.)) ;
#90848=DIRECTION('ref_axis',(0.,-1.73472347597682E-14,-1.)) ;
#90849=DIRECTION('',(1.,0.,0.)) ;
#90850=DIRECTION('center_axis',(1.,0.,0.)) ;
#90851=DIRECTION('ref_axis',(0.,0.,-1.)) ;
#90852=DIRECTION('center_axis',(0.,-1.,0.)) ;
#90853=DIRECTION('ref_axis',(0.,0.,-1.)) ;
#90854=DIRECTION('',(0.,0.,1.)) ;
#90855=DIRECTION('',(1.,0.,0.)) ;
#90856=DIRECTION('',(0.,0.,-1.)) ;
#90857=DIRECTION('center_axis',(1.,0.,0.)) ;
#90858=DIRECTION('ref_axis',(0.,0.,-1.)) ;
#90859=DIRECTION('center_axis',(1.,0.,0.)) ;
#90860=DIRECTION('ref_axis',(0.,0.,1.)) ;
#90861=DIRECTION('',(1.,0.,0.)) ;
#90862=DIRECTION('center_axis',(-1.,0.,0.)) ;
#90863=DIRECTION('ref_axis',(0.,0.,-1.)) ;
#90864=DIRECTION('center_axis',(0.,0.,-1.)) ;
#90865=DIRECTION('ref_axis',(-1.,0.,0.)) ;
#90866=DIRECTION('',(0.,-1.,0.)) ;
#90867=DIRECTION('',(1.,0.,0.)) ;
#90868=DIRECTION('',(0.,1.,0.)) ;
#90869=DIRECTION('center_axis',(1.,0.,0.)) ;
#90870=DIRECTION('ref_axis',(0.,0.,-1.)) ;
#90871=DIRECTION('center_axis',(1.,0.,0.)) ;
#90872=DIRECTION('ref_axis',(0.,0.,1.)) ;
#90873=DIRECTION('',(1.,0.,0.)) ;
#90874=DIRECTION('center_axis',(-1.,0.,0.)) ;
#90875=DIRECTION('ref_axis',(0.,0.,-1.)) ;
#90876=DIRECTION('center_axis',(0.,1.,0.)) ;
#90877=DIRECTION('ref_axis',(0.,0.,1.)) ;
#90878=DIRECTION('',(0.,0.,-1.)) ;
#90879=DIRECTION('',(1.,0.,0.)) ;
#90880=DIRECTION('',(0.,0.,1.)) ;
#90881=DIRECTION('center_axis',(1.,0.,0.)) ;
#90882=DIRECTION('ref_axis',(0.,0.,-1.)) ;
#90883=DIRECTION('center_axis',(-1.,0.,0.)) ;
#90884=DIRECTION('ref_axis',(0.,1.95156391047392E-14,-1.)) ;
#90885=DIRECTION('',(1.,0.,0.)) ;
#90886=DIRECTION('center_axis',(1.,0.,0.)) ;
#90887=DIRECTION('ref_axis',(0.,0.,-1.)) ;
#90888=DIRECTION('center_axis',(0.,1.07081696047951E-16,-1.)) ;
#90889=DIRECTION('ref_axis',(0.,1.,1.07081696047951E-16)) ;
#90890=DIRECTION('',(0.,-1.,-1.07081696047951E-16)) ;
#90891=DIRECTION('',(1.,0.,0.)) ;
#90892=DIRECTION('',(0.,1.,1.07081696047951E-16)) ;
#90893=DIRECTION('center_axis',(1.,0.,0.)) ;
#90894=DIRECTION('ref_axis',(0.,0.,-1.)) ;
#90895=DIRECTION('center_axis',(-1.,0.,0.)) ;
#90896=DIRECTION('ref_axis',(0.,0.,-1.)) ;
#90897=DIRECTION('',(1.,0.,0.)) ;
#90898=DIRECTION('center_axis',(1.,0.,0.)) ;
#90899=DIRECTION('ref_axis',(0.,0.,-1.)) ;
#90900=DIRECTION('center_axis',(0.,-1.,0.)) ;
#90901=DIRECTION('ref_axis',(0.,0.,-1.)) ;
#90902=DIRECTION('',(0.,0.,1.)) ;
#90903=DIRECTION('',(1.,0.,0.)) ;
#90904=DIRECTION('',(0.,0.,-1.)) ;
#90905=DIRECTION('center_axis',(1.,0.,0.)) ;
#90906=DIRECTION('ref_axis',(0.,0.,-1.)) ;
#90907=DIRECTION('center_axis',(-1.,0.,0.)) ;
#90908=DIRECTION('ref_axis',(0.,4.33680868994204E-15,-1.)) ;
#90909=DIRECTION('',(1.,0.,0.)) ;
#90910=DIRECTION('center_axis',(1.,0.,0.)) ;
#90911=DIRECTION('ref_axis',(0.,0.,-1.)) ;
#90912=DIRECTION('center_axis',(1.,0.,0.)) ;
#90913=DIRECTION('ref_axis',(0.,0.,-1.)) ;
#90914=DIRECTION('center_axis',(1.,0.,0.)) ;
#90915=DIRECTION('ref_axis',(0.,-7.85535158932895E-16,1.)) ;
#90916=DIRECTION('',(1.,0.,0.)) ;
#90917=DIRECTION('center_axis',(-1.,0.,0.)) ;
#90918=DIRECTION('ref_axis',(0.,-7.85535158932895E-16,-1.)) ;
#90919=DIRECTION('center_axis',(1.,0.,0.)) ;
#90920=DIRECTION('ref_axis',(0.,0.,-1.)) ;
#90921=DIRECTION('center_axis',(-1.,0.,0.)) ;
#90922=DIRECTION('ref_axis',(0.,4.33680868994204E-15,-1.)) ;
#90923=DIRECTION('',(1.,0.,0.)) ;
#90924=DIRECTION('center_axis',(1.,0.,0.)) ;
#90925=DIRECTION('ref_axis',(0.,0.,-1.)) ;
#90926=DIRECTION('center_axis',(0.,-1.,0.)) ;
#90927=DIRECTION('ref_axis',(0.,0.,-1.)) ;
#90928=DIRECTION('',(0.,0.,1.)) ;
#90929=DIRECTION('',(1.,0.,0.)) ;
#90930=DIRECTION('',(0.,0.,-1.)) ;
#90931=DIRECTION('center_axis',(1.,0.,0.)) ;
#90932=DIRECTION('ref_axis',(0.,0.,-1.)) ;
#90933=DIRECTION('center_axis',(-1.,0.,0.)) ;
#90934=DIRECTION('ref_axis',(0.,0.,-1.)) ;
#90935=DIRECTION('',(1.,0.,0.)) ;
#90936=DIRECTION('center_axis',(1.,0.,0.)) ;
#90937=DIRECTION('ref_axis',(0.,0.,-1.)) ;
#90938=DIRECTION('center_axis',(0.,-1.07081696047951E-16,1.)) ;
#90939=DIRECTION('ref_axis',(0.,-1.,-1.07081696047951E-16)) ;
#90940=DIRECTION('',(0.,1.,1.07081696047951E-16)) ;
#90941=DIRECTION('',(1.,0.,0.)) ;
#90942=DIRECTION('',(0.,-1.,-1.07081696047951E-16)) ;
#90943=DIRECTION('center_axis',(1.,0.,0.)) ;
#90944=DIRECTION('ref_axis',(0.,0.,-1.)) ;
#90945=DIRECTION('center_axis',(-1.,0.,0.)) ;
#90946=DIRECTION('ref_axis',(0.,0.,-1.)) ;
#90947=DIRECTION('',(1.,0.,0.)) ;
#90948=DIRECTION('center_axis',(1.,0.,0.)) ;
#90949=DIRECTION('ref_axis',(0.,0.,-1.)) ;
#90950=DIRECTION('center_axis',(0.,1.,0.)) ;
#90951=DIRECTION('ref_axis',(0.,0.,1.)) ;
#90952=DIRECTION('',(0.,0.,-1.)) ;
#90953=DIRECTION('',(0.,0.,1.)) ;
#90954=DIRECTION('center_axis',(-1.,0.,0.)) ;
#90955=DIRECTION('ref_axis',(0.,0.,1.)) ;
#90956=DIRECTION('center_axis',(-1.,0.,0.)) ;
#90957=DIRECTION('ref_axis',(0.,0.,1.)) ;
#90958=DIRECTION('',(0.,-1.,0.)) ;
#90959=DIRECTION('center_axis',(-1.,0.,0.)) ;
#90960=DIRECTION('ref_axis',(0.,0.,1.)) ;
#90961=DIRECTION('',(0.,0.,1.)) ;
#90962=DIRECTION('',(0.,-1.,-1.07081696047951E-16)) ;
#90963=DIRECTION('',(0.,0.,-1.)) ;
#90964=DIRECTION('center_axis',(-1.,0.,0.)) ;
#90965=DIRECTION('ref_axis',(0.,0.,1.)) ;
#90966=DIRECTION('',(0.,0.,-1.)) ;
#90967=DIRECTION('',(0.,1.,1.07081696047951E-16)) ;
#90968=DIRECTION('',(0.,0.,1.)) ;
#90969=DIRECTION('center_axis',(-1.,0.,0.)) ;
#90970=DIRECTION('ref_axis',(0.,0.,1.)) ;
#90971=DIRECTION('',(0.,1.,0.)) ;
#90972=DIRECTION('center_axis',(-1.,0.,0.)) ;
#90973=DIRECTION('ref_axis',(0.,0.,1.)) ;
#90974=DIRECTION('',(0.,0.,-1.)) ;
#90975=DIRECTION('',(0.,0.707106781186548,-0.707106781186547)) ;
#90976=DIRECTION('',(0.,0.,1.)) ;
#90977=DIRECTION('',(0.,-0.707106781186546,-0.707106781186549)) ;
#90978=DIRECTION('',(0.,-3.99416362155027E-15,-1.)) ;
#90979=DIRECTION('center_axis',(1.,0.,0.)) ;
#90980=DIRECTION('ref_axis',(0.,0.,-1.)) ;
#90981=DIRECTION('',(1.,0.,0.)) ;
#90982=DIRECTION('center_axis',(1.,0.,0.)) ;
#90983=DIRECTION('ref_axis',(0.,0.,1.)) ;
#90984=DIRECTION('',(1.,0.,0.)) ;
#90985=DIRECTION('center_axis',(-1.,0.,0.)) ;
#90986=DIRECTION('ref_axis',(0.,0.,-1.)) ;
#90987=DIRECTION('center_axis',(0.,0.,1.)) ;
#90988=DIRECTION('ref_axis',(1.,0.,0.)) ;
#90989=DIRECTION('',(0.,1.,0.)) ;
#90990=DIRECTION('',(1.,0.,0.)) ;
#90991=DIRECTION('',(0.,-1.,0.)) ;
#90992=DIRECTION('center_axis',(1.,0.,0.)) ;
#90993=DIRECTION('ref_axis',(0.,0.,-1.)) ;
#90994=DIRECTION('center_axis',(1.,0.,0.)) ;
#90995=DIRECTION('ref_axis',(0.,0.,1.)) ;
#90996=DIRECTION('',(1.,0.,0.)) ;
#90997=DIRECTION('center_axis',(-1.,0.,0.)) ;
#90998=DIRECTION('ref_axis',(0.,0.,-1.)) ;
#90999=DIRECTION('center_axis',(0.,-1.,3.99416362155027E-15)) ;
#91000=DIRECTION('ref_axis',(0.,-3.99416362155027E-15,-1.)) ;
#91001=DIRECTION('',(0.,3.99416362155027E-15,1.)) ;
#91002=DIRECTION('',(1.,0.,0.)) ;
#91003=DIRECTION('',(0.,-3.99416362155027E-15,-1.)) ;
#91004=DIRECTION('center_axis',(1.,0.,0.)) ;
#91005=DIRECTION('ref_axis',(0.,0.,-1.)) ;
#91006=DIRECTION('center_axis',(-1.,0.,0.)) ;
#91007=DIRECTION('ref_axis',(0.,1.30104260698261E-14,-1.)) ;
#91008=DIRECTION('',(1.,0.,0.)) ;
#91009=DIRECTION('center_axis',(1.,0.,0.)) ;
#91010=DIRECTION('ref_axis',(0.,0.,-1.)) ;
#91011=DIRECTION('center_axis',(0.,-0.707106781186549,0.707106781186546)) ;
#91012=DIRECTION('ref_axis',(0.,-0.707106781186546,-0.707106781186549)) ;
#91013=DIRECTION('',(0.,0.707106781186546,0.707106781186549)) ;
#91014=DIRECTION('',(1.,0.,0.)) ;
#91015=DIRECTION('',(0.,-0.707106781186546,-0.707106781186549)) ;
#91016=DIRECTION('center_axis',(1.,0.,0.)) ;
#91017=DIRECTION('ref_axis',(0.,0.382683432365084,0.923879532511289)) ;
#91018=DIRECTION('',(1.,0.,0.)) ;
#91019=DIRECTION('center_axis',(1.,0.,0.)) ;
#91020=DIRECTION('ref_axis',(0.,0.,-1.)) ;
#91021=DIRECTION('center_axis',(0.,1.,0.)) ;
#91022=DIRECTION('ref_axis',(0.,0.,1.)) ;
#91023=DIRECTION('',(0.,0.,-1.)) ;
#91024=DIRECTION('',(0.,0.,1.)) ;
#91025=DIRECTION('center_axis',(0.,-0.707106781186547,-0.707106781186548)) ;
#91026=DIRECTION('ref_axis',(0.,0.707106781186548,-0.707106781186547)) ;
#91027=DIRECTION('',(0.,-0.707106781186548,0.707106781186547)) ;
#91028=DIRECTION('',(1.,0.,0.)) ;
#91029=DIRECTION('',(0.,0.707106781186548,-0.707106781186547)) ;
#91030=DIRECTION('center_axis',(1.,0.,0.)) ;
#91031=DIRECTION('ref_axis',(0.,0.,-1.)) ;
#91032=DIRECTION('center_axis',(-1.,0.,0.)) ;
#91033=DIRECTION('ref_axis',(0.,-1.73472347597682E-14,-1.)) ;
#91034=DIRECTION('',(1.,0.,0.)) ;
#91035=DIRECTION('center_axis',(1.,0.,0.)) ;
#91036=DIRECTION('ref_axis',(0.,0.,-1.)) ;
#91037=DIRECTION('center_axis',(0.,-1.,0.)) ;
#91038=DIRECTION('ref_axis',(0.,0.,-1.)) ;
#91039=DIRECTION('',(0.,0.,1.)) ;
#91040=DIRECTION('',(1.,0.,0.)) ;
#91041=DIRECTION('',(0.,0.,-1.)) ;
#91042=DIRECTION('center_axis',(1.,0.,0.)) ;
#91043=DIRECTION('ref_axis',(0.,0.,-1.)) ;
#91044=DIRECTION('center_axis',(1.,0.,0.)) ;
#91045=DIRECTION('ref_axis',(0.,0.,1.)) ;
#91046=DIRECTION('',(1.,0.,0.)) ;
#91047=DIRECTION('center_axis',(-1.,0.,0.)) ;
#91048=DIRECTION('ref_axis',(0.,0.,-1.)) ;
#91049=DIRECTION('center_axis',(0.,0.,-1.)) ;
#91050=DIRECTION('ref_axis',(-1.,0.,0.)) ;
#91051=DIRECTION('',(0.,-1.,0.)) ;
#91052=DIRECTION('',(1.,0.,0.)) ;
#91053=DIRECTION('',(0.,1.,0.)) ;
#91054=DIRECTION('center_axis',(1.,0.,0.)) ;
#91055=DIRECTION('ref_axis',(0.,0.,-1.)) ;
#91056=DIRECTION('center_axis',(1.,0.,0.)) ;
#91057=DIRECTION('ref_axis',(0.,0.,1.)) ;
#91058=DIRECTION('',(1.,0.,0.)) ;
#91059=DIRECTION('center_axis',(-1.,0.,0.)) ;
#91060=DIRECTION('ref_axis',(0.,0.,-1.)) ;
#91061=DIRECTION('center_axis',(0.,1.,0.)) ;
#91062=DIRECTION('ref_axis',(0.,0.,1.)) ;
#91063=DIRECTION('',(0.,0.,-1.)) ;
#91064=DIRECTION('',(1.,0.,0.)) ;
#91065=DIRECTION('',(0.,0.,1.)) ;
#91066=DIRECTION('center_axis',(1.,0.,0.)) ;
#91067=DIRECTION('ref_axis',(0.,0.,-1.)) ;
#91068=DIRECTION('center_axis',(-1.,0.,0.)) ;
#91069=DIRECTION('ref_axis',(0.,1.95156391047392E-14,-1.)) ;
#91070=DIRECTION('',(1.,0.,0.)) ;
#91071=DIRECTION('center_axis',(1.,0.,0.)) ;
#91072=DIRECTION('ref_axis',(0.,0.,-1.)) ;
#91073=DIRECTION('center_axis',(0.,1.07081696047951E-16,-1.)) ;
#91074=DIRECTION('ref_axis',(0.,1.,1.07081696047951E-16)) ;
#91075=DIRECTION('',(0.,-1.,-1.07081696047951E-16)) ;
#91076=DIRECTION('',(1.,0.,0.)) ;
#91077=DIRECTION('',(0.,1.,1.07081696047951E-16)) ;
#91078=DIRECTION('center_axis',(1.,0.,0.)) ;
#91079=DIRECTION('ref_axis',(0.,0.,-1.)) ;
#91080=DIRECTION('center_axis',(-1.,0.,0.)) ;
#91081=DIRECTION('ref_axis',(0.,0.,-1.)) ;
#91082=DIRECTION('',(1.,0.,0.)) ;
#91083=DIRECTION('center_axis',(1.,0.,0.)) ;
#91084=DIRECTION('ref_axis',(0.,0.,-1.)) ;
#91085=DIRECTION('center_axis',(0.,-1.,0.)) ;
#91086=DIRECTION('ref_axis',(0.,0.,-1.)) ;
#91087=DIRECTION('',(0.,0.,1.)) ;
#91088=DIRECTION('',(1.,0.,0.)) ;
#91089=DIRECTION('',(0.,0.,-1.)) ;
#91090=DIRECTION('center_axis',(1.,0.,0.)) ;
#91091=DIRECTION('ref_axis',(0.,0.,-1.)) ;
#91092=DIRECTION('center_axis',(-1.,0.,0.)) ;
#91093=DIRECTION('ref_axis',(0.,4.33680868994204E-15,-1.)) ;
#91094=DIRECTION('',(1.,0.,0.)) ;
#91095=DIRECTION('center_axis',(1.,0.,0.)) ;
#91096=DIRECTION('ref_axis',(0.,0.,-1.)) ;
#91097=DIRECTION('center_axis',(1.,0.,0.)) ;
#91098=DIRECTION('ref_axis',(0.,0.,-1.)) ;
#91099=DIRECTION('center_axis',(1.,0.,0.)) ;
#91100=DIRECTION('ref_axis',(0.,-7.85535158932894E-16,1.)) ;
#91101=DIRECTION('',(1.,0.,0.)) ;
#91102=DIRECTION('center_axis',(-1.,0.,0.)) ;
#91103=DIRECTION('ref_axis',(0.,-7.85535158932895E-16,-1.)) ;
#91104=DIRECTION('center_axis',(1.,0.,0.)) ;
#91105=DIRECTION('ref_axis',(0.,0.,-1.)) ;
#91106=DIRECTION('center_axis',(-1.,0.,0.)) ;
#91107=DIRECTION('ref_axis',(0.,-8.67361737988409E-15,-1.)) ;
#91108=DIRECTION('',(1.,0.,0.)) ;
#91109=DIRECTION('center_axis',(1.,0.,0.)) ;
#91110=DIRECTION('ref_axis',(0.,0.,-1.)) ;
#91111=DIRECTION('center_axis',(0.,-1.,0.)) ;
#91112=DIRECTION('ref_axis',(0.,0.,-1.)) ;
#91113=DIRECTION('',(0.,0.,1.)) ;
#91114=DIRECTION('',(1.,0.,0.)) ;
#91115=DIRECTION('',(0.,0.,-1.)) ;
#91116=DIRECTION('center_axis',(1.,0.,0.)) ;
#91117=DIRECTION('ref_axis',(0.,0.,-1.)) ;
#91118=DIRECTION('center_axis',(-1.,0.,0.)) ;
#91119=DIRECTION('ref_axis',(0.,0.,-1.)) ;
#91120=DIRECTION('',(1.,0.,0.)) ;
#91121=DIRECTION('center_axis',(1.,0.,0.)) ;
#91122=DIRECTION('ref_axis',(0.,0.,-1.)) ;
#91123=DIRECTION('center_axis',(0.,-1.07081696047951E-16,1.)) ;
#91124=DIRECTION('ref_axis',(0.,-1.,-1.07081696047951E-16)) ;
#91125=DIRECTION('',(0.,1.,1.07081696047951E-16)) ;
#91126=DIRECTION('',(1.,0.,0.)) ;
#91127=DIRECTION('',(0.,-1.,-1.07081696047951E-16)) ;
#91128=DIRECTION('center_axis',(1.,0.,0.)) ;
#91129=DIRECTION('ref_axis',(0.,0.,-1.)) ;
#91130=DIRECTION('center_axis',(-1.,0.,0.)) ;
#91131=DIRECTION('ref_axis',(0.,0.,-1.)) ;
#91132=DIRECTION('',(1.,0.,0.)) ;
#91133=DIRECTION('center_axis',(1.,0.,0.)) ;
#91134=DIRECTION('ref_axis',(0.,0.,-1.)) ;
#91135=DIRECTION('center_axis',(0.,1.,0.)) ;
#91136=DIRECTION('ref_axis',(0.,0.,1.)) ;
#91137=DIRECTION('',(0.,0.,-1.)) ;
#91138=DIRECTION('',(0.,0.,1.)) ;
#91139=DIRECTION('center_axis',(-1.,0.,0.)) ;
#91140=DIRECTION('ref_axis',(0.,0.,1.)) ;
#91141=DIRECTION('center_axis',(-1.,0.,0.)) ;
#91142=DIRECTION('ref_axis',(0.,0.,1.)) ;
#91143=DIRECTION('',(0.,-1.,0.)) ;
#91144=DIRECTION('center_axis',(-1.,0.,0.)) ;
#91145=DIRECTION('ref_axis',(0.,0.,1.)) ;
#91146=DIRECTION('',(0.,0.,1.)) ;
#91147=DIRECTION('',(0.,-1.,-1.07081696047951E-16)) ;
#91148=DIRECTION('',(0.,0.,-1.)) ;
#91149=DIRECTION('center_axis',(-1.,0.,0.)) ;
#91150=DIRECTION('ref_axis',(0.,0.,1.)) ;
#91151=DIRECTION('',(0.,0.,-1.)) ;
#91152=DIRECTION('',(0.,1.,1.07081696047951E-16)) ;
#91153=DIRECTION('',(0.,0.,1.)) ;
#91154=DIRECTION('center_axis',(-1.,0.,0.)) ;
#91155=DIRECTION('ref_axis',(0.,0.,1.)) ;
#91156=DIRECTION('',(0.,1.,0.)) ;
#91157=DIRECTION('center_axis',(-1.,0.,0.)) ;
#91158=DIRECTION('ref_axis',(0.,0.,1.)) ;
#91159=DIRECTION('',(0.,0.,-1.)) ;
#91160=DIRECTION('',(0.,0.707106781186548,-0.707106781186547)) ;
#91161=DIRECTION('',(0.,0.,1.)) ;
#91162=DIRECTION('',(0.,-0.707106781186546,-0.707106781186549)) ;
#91163=DIRECTION('',(0.,-3.99416362155027E-15,-1.)) ;
#91164=DIRECTION('center_axis',(1.,0.,0.)) ;
#91165=DIRECTION('ref_axis',(0.,0.,-1.)) ;
#91166=DIRECTION('',(1.,0.,0.)) ;
#91167=DIRECTION('center_axis',(1.,0.,0.)) ;
#91168=DIRECTION('ref_axis',(0.,0.,1.)) ;
#91169=DIRECTION('',(1.,0.,0.)) ;
#91170=DIRECTION('center_axis',(-1.,0.,0.)) ;
#91171=DIRECTION('ref_axis',(0.,0.,-1.)) ;
#91172=DIRECTION('center_axis',(0.,0.,1.)) ;
#91173=DIRECTION('ref_axis',(1.,0.,0.)) ;
#91174=DIRECTION('',(0.,1.,0.)) ;
#91175=DIRECTION('',(1.,0.,0.)) ;
#91176=DIRECTION('',(0.,-1.,0.)) ;
#91177=DIRECTION('center_axis',(1.,0.,0.)) ;
#91178=DIRECTION('ref_axis',(0.,0.,-1.)) ;
#91179=DIRECTION('center_axis',(1.,0.,0.)) ;
#91180=DIRECTION('ref_axis',(0.,0.,1.)) ;
#91181=DIRECTION('',(1.,0.,0.)) ;
#91182=DIRECTION('center_axis',(-1.,0.,0.)) ;
#91183=DIRECTION('ref_axis',(0.,0.,-1.)) ;
#91184=DIRECTION('center_axis',(0.,-1.,3.99416362155027E-15)) ;
#91185=DIRECTION('ref_axis',(0.,-3.99416362155027E-15,-1.)) ;
#91186=DIRECTION('',(0.,3.99416362155027E-15,1.)) ;
#91187=DIRECTION('',(1.,0.,0.)) ;
#91188=DIRECTION('',(0.,-3.99416362155027E-15,-1.)) ;
#91189=DIRECTION('center_axis',(1.,0.,0.)) ;
#91190=DIRECTION('ref_axis',(0.,0.,-1.)) ;
#91191=DIRECTION('center_axis',(-1.,0.,0.)) ;
#91192=DIRECTION('ref_axis',(0.,1.30104260698261E-14,-1.)) ;
#91193=DIRECTION('',(1.,0.,0.)) ;
#91194=DIRECTION('center_axis',(1.,0.,0.)) ;
#91195=DIRECTION('ref_axis',(0.,0.,-1.)) ;
#91196=DIRECTION('center_axis',(0.,-0.707106781186549,0.707106781186546)) ;
#91197=DIRECTION('ref_axis',(0.,-0.707106781186546,-0.707106781186549)) ;
#91198=DIRECTION('',(0.,0.707106781186546,0.707106781186549)) ;
#91199=DIRECTION('',(1.,0.,0.)) ;
#91200=DIRECTION('',(0.,-0.707106781186546,-0.707106781186549)) ;
#91201=DIRECTION('center_axis',(1.,0.,0.)) ;
#91202=DIRECTION('ref_axis',(0.,0.382683432365088,0.923879532511288)) ;
#91203=DIRECTION('',(1.,0.,0.)) ;
#91204=DIRECTION('center_axis',(1.,0.,0.)) ;
#91205=DIRECTION('ref_axis',(0.,0.,-1.)) ;
#91206=DIRECTION('center_axis',(0.,1.,0.)) ;
#91207=DIRECTION('ref_axis',(0.,0.,1.)) ;
#91208=DIRECTION('',(0.,0.,-1.)) ;
#91209=DIRECTION('',(0.,0.,1.)) ;
#91210=DIRECTION('center_axis',(0.,-0.707106781186547,-0.707106781186548)) ;
#91211=DIRECTION('ref_axis',(0.,0.707106781186548,-0.707106781186547)) ;
#91212=DIRECTION('',(0.,-0.707106781186548,0.707106781186547)) ;
#91213=DIRECTION('',(1.,0.,0.)) ;
#91214=DIRECTION('',(0.,0.707106781186548,-0.707106781186547)) ;
#91215=DIRECTION('center_axis',(1.,0.,0.)) ;
#91216=DIRECTION('ref_axis',(0.,0.,-1.)) ;
#91217=DIRECTION('center_axis',(-1.,0.,0.)) ;
#91218=DIRECTION('ref_axis',(0.,0.,-1.)) ;
#91219=DIRECTION('',(1.,0.,0.)) ;
#91220=DIRECTION('center_axis',(1.,0.,0.)) ;
#91221=DIRECTION('ref_axis',(0.,0.,-1.)) ;
#91222=DIRECTION('center_axis',(0.,-1.,0.)) ;
#91223=DIRECTION('ref_axis',(0.,0.,-1.)) ;
#91224=DIRECTION('',(0.,0.,1.)) ;
#91225=DIRECTION('',(1.,0.,0.)) ;
#91226=DIRECTION('',(0.,0.,-1.)) ;
#91227=DIRECTION('center_axis',(1.,0.,0.)) ;
#91228=DIRECTION('ref_axis',(0.,0.,-1.)) ;
#91229=DIRECTION('center_axis',(1.,0.,0.)) ;
#91230=DIRECTION('ref_axis',(0.,0.,1.)) ;
#91231=DIRECTION('',(1.,0.,0.)) ;
#91232=DIRECTION('center_axis',(-1.,0.,0.)) ;
#91233=DIRECTION('ref_axis',(0.,0.,-1.)) ;
#91234=DIRECTION('center_axis',(0.,0.,-1.)) ;
#91235=DIRECTION('ref_axis',(-1.,0.,0.)) ;
#91236=DIRECTION('',(0.,-1.,0.)) ;
#91237=DIRECTION('',(1.,0.,0.)) ;
#91238=DIRECTION('',(0.,1.,0.)) ;
#91239=DIRECTION('center_axis',(1.,0.,0.)) ;
#91240=DIRECTION('ref_axis',(0.,0.,-1.)) ;
#91241=DIRECTION('center_axis',(1.,0.,0.)) ;
#91242=DIRECTION('ref_axis',(0.,0.,1.)) ;
#91243=DIRECTION('',(1.,0.,0.)) ;
#91244=DIRECTION('center_axis',(-1.,0.,0.)) ;
#91245=DIRECTION('ref_axis',(0.,0.,-1.)) ;
#91246=DIRECTION('center_axis',(0.,1.,0.)) ;
#91247=DIRECTION('ref_axis',(0.,0.,1.)) ;
#91248=DIRECTION('',(0.,0.,-1.)) ;
#91249=DIRECTION('',(1.,0.,0.)) ;
#91250=DIRECTION('',(0.,0.,1.)) ;
#91251=DIRECTION('center_axis',(1.,0.,0.)) ;
#91252=DIRECTION('ref_axis',(0.,0.,-1.)) ;
#91253=DIRECTION('center_axis',(-1.,0.,0.)) ;
#91254=DIRECTION('ref_axis',(0.,1.95156391047392E-14,-1.)) ;
#91255=DIRECTION('',(1.,0.,0.)) ;
#91256=DIRECTION('center_axis',(1.,0.,0.)) ;
#91257=DIRECTION('ref_axis',(0.,0.,-1.)) ;
#91258=DIRECTION('center_axis',(0.,1.07081696047951E-16,-1.)) ;
#91259=DIRECTION('ref_axis',(0.,1.,1.07081696047951E-16)) ;
#91260=DIRECTION('',(0.,-1.,-1.07081696047951E-16)) ;
#91261=DIRECTION('',(1.,0.,0.)) ;
#91262=DIRECTION('',(0.,1.,1.07081696047951E-16)) ;
#91263=DIRECTION('center_axis',(1.,0.,0.)) ;
#91264=DIRECTION('ref_axis',(0.,0.,-1.)) ;
#91265=DIRECTION('center_axis',(-1.,0.,0.)) ;
#91266=DIRECTION('ref_axis',(0.,0.,-1.)) ;
#91267=DIRECTION('',(1.,0.,0.)) ;
#91268=DIRECTION('center_axis',(1.,0.,0.)) ;
#91269=DIRECTION('ref_axis',(0.,0.,-1.)) ;
#91270=DIRECTION('center_axis',(0.,-1.,0.)) ;
#91271=DIRECTION('ref_axis',(0.,0.,-1.)) ;
#91272=DIRECTION('',(0.,0.,1.)) ;
#91273=DIRECTION('',(1.,0.,0.)) ;
#91274=DIRECTION('',(0.,0.,-1.)) ;
#91275=DIRECTION('center_axis',(1.,0.,0.)) ;
#91276=DIRECTION('ref_axis',(0.,0.,-1.)) ;
#91277=DIRECTION('center_axis',(-1.,0.,0.)) ;
#91278=DIRECTION('ref_axis',(0.,-4.33680868994204E-15,-1.)) ;
#91279=DIRECTION('',(1.,0.,0.)) ;
#91280=DIRECTION('center_axis',(1.,0.,0.)) ;
#91281=DIRECTION('ref_axis',(0.,0.,-1.)) ;
#91282=DIRECTION('center_axis',(1.,0.,0.)) ;
#91283=DIRECTION('ref_axis',(0.,0.,-1.)) ;
#91284=DIRECTION('center_axis',(1.,0.,0.)) ;
#91285=DIRECTION('ref_axis',(0.,-7.85535158932894E-16,1.)) ;
#91286=DIRECTION('',(1.,0.,0.)) ;
#91287=DIRECTION('center_axis',(-1.,0.,0.)) ;
#91288=DIRECTION('ref_axis',(0.,-7.85535158932894E-16,-1.)) ;
#91289=DIRECTION('center_axis',(1.,0.,0.)) ;
#91290=DIRECTION('ref_axis',(0.,0.,-1.)) ;
#91291=DIRECTION('center_axis',(-1.,0.,0.)) ;
#91292=DIRECTION('ref_axis',(0.,-8.67361737988409E-15,-1.)) ;
#91293=DIRECTION('',(1.,0.,0.)) ;
#91294=DIRECTION('center_axis',(1.,0.,0.)) ;
#91295=DIRECTION('ref_axis',(0.,0.,-1.)) ;
#91296=DIRECTION('center_axis',(0.,-1.,0.)) ;
#91297=DIRECTION('ref_axis',(0.,0.,-1.)) ;
#91298=DIRECTION('',(0.,0.,1.)) ;
#91299=DIRECTION('',(1.,0.,0.)) ;
#91300=DIRECTION('',(0.,0.,-1.)) ;
#91301=DIRECTION('center_axis',(1.,0.,0.)) ;
#91302=DIRECTION('ref_axis',(0.,0.,-1.)) ;
#91303=DIRECTION('center_axis',(-1.,0.,0.)) ;
#91304=DIRECTION('ref_axis',(0.,0.,-1.)) ;
#91305=DIRECTION('',(1.,0.,0.)) ;
#91306=DIRECTION('center_axis',(1.,0.,0.)) ;
#91307=DIRECTION('ref_axis',(0.,0.,-1.)) ;
#91308=DIRECTION('center_axis',(0.,-1.07081696047951E-16,1.)) ;
#91309=DIRECTION('ref_axis',(0.,-1.,-1.07081696047951E-16)) ;
#91310=DIRECTION('',(0.,1.,1.07081696047951E-16)) ;
#91311=DIRECTION('',(1.,0.,0.)) ;
#91312=DIRECTION('',(0.,-1.,-1.07081696047951E-16)) ;
#91313=DIRECTION('center_axis',(1.,0.,0.)) ;
#91314=DIRECTION('ref_axis',(0.,0.,-1.)) ;
#91315=DIRECTION('center_axis',(-1.,0.,0.)) ;
#91316=DIRECTION('ref_axis',(0.,0.,-1.)) ;
#91317=DIRECTION('',(1.,0.,0.)) ;
#91318=DIRECTION('center_axis',(1.,0.,0.)) ;
#91319=DIRECTION('ref_axis',(0.,0.,-1.)) ;
#91320=DIRECTION('center_axis',(0.,1.,0.)) ;
#91321=DIRECTION('ref_axis',(0.,0.,1.)) ;
#91322=DIRECTION('',(0.,0.,-1.)) ;
#91323=DIRECTION('',(0.,0.,1.)) ;
#91324=DIRECTION('center_axis',(-1.,0.,0.)) ;
#91325=DIRECTION('ref_axis',(0.,0.,1.)) ;
#91326=DIRECTION('center_axis',(-1.,0.,0.)) ;
#91327=DIRECTION('ref_axis',(0.,0.,1.)) ;
#91328=DIRECTION('',(0.,-1.,0.)) ;
#91329=DIRECTION('center_axis',(-1.,0.,0.)) ;
#91330=DIRECTION('ref_axis',(0.,0.,1.)) ;
#91331=DIRECTION('',(0.,0.,1.)) ;
#91332=DIRECTION('',(0.,-1.,-1.07081696047951E-16)) ;
#91333=DIRECTION('',(0.,0.,-1.)) ;
#91334=DIRECTION('center_axis',(-1.,0.,0.)) ;
#91335=DIRECTION('ref_axis',(0.,0.,1.)) ;
#91336=DIRECTION('',(0.,0.,-1.)) ;
#91337=DIRECTION('',(0.,1.,1.07081696047951E-16)) ;
#91338=DIRECTION('',(0.,0.,1.)) ;
#91339=DIRECTION('center_axis',(-1.,0.,0.)) ;
#91340=DIRECTION('ref_axis',(0.,0.,1.)) ;
#91341=DIRECTION('',(0.,1.,0.)) ;
#91342=DIRECTION('center_axis',(-1.,0.,0.)) ;
#91343=DIRECTION('ref_axis',(0.,0.,1.)) ;
#91344=DIRECTION('',(0.,0.,-1.)) ;
#91345=DIRECTION('',(0.,0.707106781186548,-0.707106781186547)) ;
#91346=DIRECTION('',(0.,0.,1.)) ;
#91347=DIRECTION('',(0.,-0.707106781186546,-0.707106781186549)) ;
#91348=DIRECTION('',(0.,-3.99416362155027E-15,-1.)) ;
#91349=DIRECTION('center_axis',(1.,0.,0.)) ;
#91350=DIRECTION('ref_axis',(0.,0.,-1.)) ;
#91351=DIRECTION('',(1.,0.,0.)) ;
#91352=DIRECTION('center_axis',(1.,0.,0.)) ;
#91353=DIRECTION('ref_axis',(0.,0.,1.)) ;
#91354=DIRECTION('',(1.,0.,0.)) ;
#91355=DIRECTION('center_axis',(-1.,0.,0.)) ;
#91356=DIRECTION('ref_axis',(0.,0.,-1.)) ;
#91357=DIRECTION('center_axis',(0.,0.,1.)) ;
#91358=DIRECTION('ref_axis',(1.,0.,0.)) ;
#91359=DIRECTION('',(0.,1.,0.)) ;
#91360=DIRECTION('',(1.,0.,0.)) ;
#91361=DIRECTION('',(0.,-1.,0.)) ;
#91362=DIRECTION('center_axis',(1.,0.,0.)) ;
#91363=DIRECTION('ref_axis',(0.,0.,-1.)) ;
#91364=DIRECTION('center_axis',(1.,0.,0.)) ;
#91365=DIRECTION('ref_axis',(0.,0.,1.)) ;
#91366=DIRECTION('',(1.,0.,0.)) ;
#91367=DIRECTION('center_axis',(-1.,0.,0.)) ;
#91368=DIRECTION('ref_axis',(0.,0.,-1.)) ;
#91369=DIRECTION('center_axis',(0.,-1.,3.99416362155027E-15)) ;
#91370=DIRECTION('ref_axis',(0.,-3.99416362155027E-15,-1.)) ;
#91371=DIRECTION('',(0.,3.99416362155027E-15,1.)) ;
#91372=DIRECTION('',(1.,0.,0.)) ;
#91373=DIRECTION('',(0.,-3.99416362155027E-15,-1.)) ;
#91374=DIRECTION('center_axis',(1.,0.,0.)) ;
#91375=DIRECTION('ref_axis',(0.,0.,-1.)) ;
#91376=DIRECTION('center_axis',(-1.,0.,0.)) ;
#91377=DIRECTION('ref_axis',(0.,0.,-1.)) ;
#91378=DIRECTION('',(1.,0.,0.)) ;
#91379=DIRECTION('center_axis',(1.,0.,0.)) ;
#91380=DIRECTION('ref_axis',(0.,0.,-1.)) ;
#91381=DIRECTION('center_axis',(0.,-0.707106781186549,0.707106781186546)) ;
#91382=DIRECTION('ref_axis',(0.,-0.707106781186546,-0.707106781186549)) ;
#91383=DIRECTION('',(0.,0.707106781186546,0.707106781186549)) ;
#91384=DIRECTION('',(1.,0.,0.)) ;
#91385=DIRECTION('',(0.,-0.707106781186546,-0.707106781186549)) ;
#91386=DIRECTION('center_axis',(1.,0.,0.)) ;
#91387=DIRECTION('ref_axis',(0.,0.382683432365092,0.923879532511286)) ;
#91388=DIRECTION('',(1.,0.,0.)) ;
#91389=DIRECTION('center_axis',(1.,0.,0.)) ;
#91390=DIRECTION('ref_axis',(0.,0.,-1.)) ;
#91391=DIRECTION('center_axis',(0.,1.,0.)) ;
#91392=DIRECTION('ref_axis',(0.,0.,1.)) ;
#91393=DIRECTION('',(0.,0.,-1.)) ;
#91394=DIRECTION('',(0.,0.,1.)) ;
#91395=DIRECTION('center_axis',(0.,-0.707106781186547,-0.707106781186548)) ;
#91396=DIRECTION('ref_axis',(0.,0.707106781186548,-0.707106781186547)) ;
#91397=DIRECTION('',(0.,-0.707106781186548,0.707106781186547)) ;
#91398=DIRECTION('',(1.,0.,0.)) ;
#91399=DIRECTION('',(0.,0.707106781186548,-0.707106781186547)) ;
#91400=DIRECTION('center_axis',(1.,0.,0.)) ;
#91401=DIRECTION('ref_axis',(0.,0.,-1.)) ;
#91402=DIRECTION('center_axis',(-1.,0.,0.)) ;
#91403=DIRECTION('ref_axis',(0.,0.,-1.)) ;
#91404=DIRECTION('',(1.,0.,0.)) ;
#91405=DIRECTION('center_axis',(1.,0.,0.)) ;
#91406=DIRECTION('ref_axis',(0.,0.,-1.)) ;
#91407=DIRECTION('center_axis',(0.,-1.,0.)) ;
#91408=DIRECTION('ref_axis',(0.,0.,-1.)) ;
#91409=DIRECTION('',(0.,0.,1.)) ;
#91410=DIRECTION('',(1.,0.,0.)) ;
#91411=DIRECTION('',(0.,0.,-1.)) ;
#91412=DIRECTION('center_axis',(1.,0.,0.)) ;
#91413=DIRECTION('ref_axis',(0.,0.,-1.)) ;
#91414=DIRECTION('center_axis',(1.,0.,0.)) ;
#91415=DIRECTION('ref_axis',(0.,0.,1.)) ;
#91416=DIRECTION('',(1.,0.,0.)) ;
#91417=DIRECTION('center_axis',(-1.,0.,0.)) ;
#91418=DIRECTION('ref_axis',(0.,0.,-1.)) ;
#91419=DIRECTION('center_axis',(0.,0.,-1.)) ;
#91420=DIRECTION('ref_axis',(-1.,0.,0.)) ;
#91421=DIRECTION('',(0.,-1.,0.)) ;
#91422=DIRECTION('',(1.,0.,0.)) ;
#91423=DIRECTION('',(0.,1.,0.)) ;
#91424=DIRECTION('center_axis',(1.,0.,0.)) ;
#91425=DIRECTION('ref_axis',(0.,0.,-1.)) ;
#91426=DIRECTION('center_axis',(1.,0.,0.)) ;
#91427=DIRECTION('ref_axis',(0.,0.,1.)) ;
#91428=DIRECTION('',(1.,0.,0.)) ;
#91429=DIRECTION('center_axis',(-1.,0.,0.)) ;
#91430=DIRECTION('ref_axis',(0.,0.,-1.)) ;
#91431=DIRECTION('center_axis',(0.,1.,0.)) ;
#91432=DIRECTION('ref_axis',(0.,0.,1.)) ;
#91433=DIRECTION('',(0.,0.,-1.)) ;
#91434=DIRECTION('',(1.,0.,0.)) ;
#91435=DIRECTION('',(0.,0.,1.)) ;
#91436=DIRECTION('center_axis',(1.,0.,0.)) ;
#91437=DIRECTION('ref_axis',(0.,0.,-1.)) ;
#91438=DIRECTION('center_axis',(-1.,0.,0.)) ;
#91439=DIRECTION('ref_axis',(0.,1.95156391047392E-14,-1.)) ;
#91440=DIRECTION('',(1.,0.,0.)) ;
#91441=DIRECTION('center_axis',(1.,0.,0.)) ;
#91442=DIRECTION('ref_axis',(0.,0.,-1.)) ;
#91443=DIRECTION('center_axis',(0.,1.07081696047951E-16,-1.)) ;
#91444=DIRECTION('ref_axis',(0.,1.,1.07081696047951E-16)) ;
#91445=DIRECTION('',(0.,-1.,-1.07081696047951E-16)) ;
#91446=DIRECTION('',(1.,0.,0.)) ;
#91447=DIRECTION('',(0.,1.,1.07081696047951E-16)) ;
#91448=DIRECTION('center_axis',(1.,0.,0.)) ;
#91449=DIRECTION('ref_axis',(0.,0.,-1.)) ;
#91450=DIRECTION('center_axis',(-1.,0.,0.)) ;
#91451=DIRECTION('ref_axis',(0.,0.,-1.)) ;
#91452=DIRECTION('',(1.,0.,0.)) ;
#91453=DIRECTION('center_axis',(1.,0.,0.)) ;
#91454=DIRECTION('ref_axis',(0.,0.,-1.)) ;
#91455=DIRECTION('center_axis',(0.,-1.,0.)) ;
#91456=DIRECTION('ref_axis',(0.,0.,-1.)) ;
#91457=DIRECTION('',(0.,0.,1.)) ;
#91458=DIRECTION('',(1.,0.,0.)) ;
#91459=DIRECTION('',(0.,0.,-1.)) ;
#91460=DIRECTION('center_axis',(1.,0.,0.)) ;
#91461=DIRECTION('ref_axis',(0.,0.,-1.)) ;
#91462=DIRECTION('center_axis',(-1.,0.,0.)) ;
#91463=DIRECTION('ref_axis',(0.,-4.33680868994204E-15,-1.)) ;
#91464=DIRECTION('',(1.,0.,0.)) ;
#91465=DIRECTION('center_axis',(1.,0.,0.)) ;
#91466=DIRECTION('ref_axis',(0.,0.,-1.)) ;
#91467=DIRECTION('center_axis',(1.,0.,0.)) ;
#91468=DIRECTION('ref_axis',(0.,0.,-1.)) ;
#91469=DIRECTION('center_axis',(1.,0.,0.)) ;
#91470=DIRECTION('ref_axis',(0.,-7.85535158932894E-16,1.)) ;
#91471=DIRECTION('',(1.,0.,0.)) ;
#91472=DIRECTION('center_axis',(-1.,0.,0.)) ;
#91473=DIRECTION('ref_axis',(0.,-7.85535158932894E-16,-1.)) ;
#91474=DIRECTION('center_axis',(1.,0.,0.)) ;
#91475=DIRECTION('ref_axis',(0.,0.,-1.)) ;
#91476=DIRECTION('center_axis',(-1.,0.,0.)) ;
#91477=DIRECTION('ref_axis',(0.,0.,-1.)) ;
#91478=DIRECTION('',(1.,0.,0.)) ;
#91479=DIRECTION('center_axis',(1.,0.,0.)) ;
#91480=DIRECTION('ref_axis',(0.,0.,-1.)) ;
#91481=DIRECTION('center_axis',(0.,-1.,0.)) ;
#91482=DIRECTION('ref_axis',(0.,0.,-1.)) ;
#91483=DIRECTION('',(0.,0.,1.)) ;
#91484=DIRECTION('',(1.,0.,0.)) ;
#91485=DIRECTION('',(0.,0.,-1.)) ;
#91486=DIRECTION('center_axis',(1.,0.,0.)) ;
#91487=DIRECTION('ref_axis',(0.,0.,-1.)) ;
#91488=DIRECTION('center_axis',(-1.,0.,0.)) ;
#91489=DIRECTION('ref_axis',(0.,0.,-1.)) ;
#91490=DIRECTION('',(1.,0.,0.)) ;
#91491=DIRECTION('center_axis',(1.,0.,0.)) ;
#91492=DIRECTION('ref_axis',(0.,0.,-1.)) ;
#91493=DIRECTION('center_axis',(0.,-1.07081696047951E-16,1.)) ;
#91494=DIRECTION('ref_axis',(0.,-1.,-1.07081696047951E-16)) ;
#91495=DIRECTION('',(0.,1.,1.07081696047951E-16)) ;
#91496=DIRECTION('',(1.,0.,0.)) ;
#91497=DIRECTION('',(0.,-1.,-1.07081696047951E-16)) ;
#91498=DIRECTION('center_axis',(1.,0.,0.)) ;
#91499=DIRECTION('ref_axis',(0.,0.,-1.)) ;
#91500=DIRECTION('center_axis',(-1.,0.,0.)) ;
#91501=DIRECTION('ref_axis',(0.,0.,-1.)) ;
#91502=DIRECTION('',(1.,0.,0.)) ;
#91503=DIRECTION('center_axis',(1.,0.,0.)) ;
#91504=DIRECTION('ref_axis',(0.,0.,-1.)) ;
#91505=DIRECTION('center_axis',(0.,1.,0.)) ;
#91506=DIRECTION('ref_axis',(0.,0.,1.)) ;
#91507=DIRECTION('',(0.,0.,-1.)) ;
#91508=DIRECTION('',(0.,0.,1.)) ;
#91509=DIRECTION('center_axis',(-1.,0.,0.)) ;
#91510=DIRECTION('ref_axis',(0.,0.,1.)) ;
#91511=DIRECTION('center_axis',(-1.,0.,0.)) ;
#91512=DIRECTION('ref_axis',(0.,0.,1.)) ;
#91513=DIRECTION('',(0.,-1.,0.)) ;
#91514=DIRECTION('center_axis',(-1.,0.,0.)) ;
#91515=DIRECTION('ref_axis',(0.,0.,1.)) ;
#91516=DIRECTION('',(0.,0.,1.)) ;
#91517=DIRECTION('',(0.,-1.,-1.07081696047951E-16)) ;
#91518=DIRECTION('',(0.,0.,-1.)) ;
#91519=DIRECTION('center_axis',(-1.,0.,0.)) ;
#91520=DIRECTION('ref_axis',(0.,0.,1.)) ;
#91521=DIRECTION('',(0.,0.,-1.)) ;
#91522=DIRECTION('',(0.,1.,1.07081696047951E-16)) ;
#91523=DIRECTION('',(0.,0.,1.)) ;
#91524=DIRECTION('center_axis',(-1.,0.,0.)) ;
#91525=DIRECTION('ref_axis',(0.,0.,1.)) ;
#91526=DIRECTION('',(0.,1.,0.)) ;
#91527=DIRECTION('center_axis',(-1.,0.,0.)) ;
#91528=DIRECTION('ref_axis',(0.,0.,1.)) ;
#91529=DIRECTION('',(0.,0.,-1.)) ;
#91530=DIRECTION('',(0.,0.707106781186548,-0.707106781186547)) ;
#91531=DIRECTION('',(0.,0.,1.)) ;
#91532=DIRECTION('',(0.,-0.707106781186546,-0.707106781186549)) ;
#91533=DIRECTION('',(0.,-3.99416362155027E-15,-1.)) ;
#91534=DIRECTION('center_axis',(1.,0.,0.)) ;
#91535=DIRECTION('ref_axis',(0.,0.,-1.)) ;
#91536=DIRECTION('',(1.,0.,0.)) ;
#91537=DIRECTION('center_axis',(1.,0.,0.)) ;
#91538=DIRECTION('ref_axis',(0.,0.,1.)) ;
#91539=DIRECTION('',(1.,0.,0.)) ;
#91540=DIRECTION('center_axis',(-1.,0.,0.)) ;
#91541=DIRECTION('ref_axis',(0.,0.,-1.)) ;
#91542=DIRECTION('center_axis',(0.,0.,1.)) ;
#91543=DIRECTION('ref_axis',(1.,0.,0.)) ;
#91544=DIRECTION('',(0.,1.,0.)) ;
#91545=DIRECTION('',(1.,0.,0.)) ;
#91546=DIRECTION('',(0.,-1.,0.)) ;
#91547=DIRECTION('center_axis',(1.,0.,0.)) ;
#91548=DIRECTION('ref_axis',(0.,0.,-1.)) ;
#91549=DIRECTION('center_axis',(1.,0.,0.)) ;
#91550=DIRECTION('ref_axis',(0.,0.,1.)) ;
#91551=DIRECTION('',(1.,0.,0.)) ;
#91552=DIRECTION('center_axis',(-1.,0.,0.)) ;
#91553=DIRECTION('ref_axis',(0.,0.,-1.)) ;
#91554=DIRECTION('center_axis',(0.,-1.,3.99416362155027E-15)) ;
#91555=DIRECTION('ref_axis',(0.,-3.99416362155027E-15,-1.)) ;
#91556=DIRECTION('',(0.,3.99416362155027E-15,1.)) ;
#91557=DIRECTION('',(1.,0.,0.)) ;
#91558=DIRECTION('',(0.,-3.99416362155027E-15,-1.)) ;
#91559=DIRECTION('center_axis',(1.,0.,0.)) ;
#91560=DIRECTION('ref_axis',(0.,0.,-1.)) ;
#91561=DIRECTION('center_axis',(-1.,0.,0.)) ;
#91562=DIRECTION('ref_axis',(0.,0.,-1.)) ;
#91563=DIRECTION('',(1.,0.,0.)) ;
#91564=DIRECTION('center_axis',(1.,0.,0.)) ;
#91565=DIRECTION('ref_axis',(0.,0.,-1.)) ;
#91566=DIRECTION('center_axis',(0.,-0.707106781186549,0.707106781186546)) ;
#91567=DIRECTION('ref_axis',(0.,-0.707106781186546,-0.707106781186549)) ;
#91568=DIRECTION('',(0.,0.707106781186546,0.707106781186549)) ;
#91569=DIRECTION('',(1.,0.,0.)) ;
#91570=DIRECTION('',(0.,-0.707106781186546,-0.707106781186549)) ;
#91571=DIRECTION('center_axis',(1.,0.,0.)) ;
#91572=DIRECTION('ref_axis',(0.,0.382683432365092,0.923879532511286)) ;
#91573=DIRECTION('',(1.,0.,0.)) ;
#91574=DIRECTION('center_axis',(1.,0.,0.)) ;
#91575=DIRECTION('ref_axis',(0.,0.,-1.)) ;
#91576=DIRECTION('center_axis',(0.,1.,0.)) ;
#91577=DIRECTION('ref_axis',(0.,0.,1.)) ;
#91578=DIRECTION('',(0.,0.,-1.)) ;
#91579=DIRECTION('',(0.,0.,1.)) ;
#91580=DIRECTION('center_axis',(0.,-0.707106781186547,-0.707106781186548)) ;
#91581=DIRECTION('ref_axis',(0.,0.707106781186548,-0.707106781186547)) ;
#91582=DIRECTION('',(0.,-0.707106781186548,0.707106781186547)) ;
#91583=DIRECTION('',(1.,0.,0.)) ;
#91584=DIRECTION('',(0.,0.707106781186548,-0.707106781186547)) ;
#91585=DIRECTION('center_axis',(1.,0.,0.)) ;
#91586=DIRECTION('ref_axis',(0.,0.,-1.)) ;
#91587=DIRECTION('center_axis',(-1.,0.,0.)) ;
#91588=DIRECTION('ref_axis',(0.,0.,-1.)) ;
#91589=DIRECTION('',(1.,0.,0.)) ;
#91590=DIRECTION('center_axis',(1.,0.,0.)) ;
#91591=DIRECTION('ref_axis',(0.,0.,-1.)) ;
#91592=DIRECTION('center_axis',(0.,-1.,0.)) ;
#91593=DIRECTION('ref_axis',(0.,0.,-1.)) ;
#91594=DIRECTION('',(0.,0.,1.)) ;
#91595=DIRECTION('',(1.,0.,0.)) ;
#91596=DIRECTION('',(0.,0.,-1.)) ;
#91597=DIRECTION('center_axis',(1.,0.,0.)) ;
#91598=DIRECTION('ref_axis',(0.,0.,-1.)) ;
#91599=DIRECTION('center_axis',(1.,0.,0.)) ;
#91600=DIRECTION('ref_axis',(0.,0.,1.)) ;
#91601=DIRECTION('',(1.,0.,0.)) ;
#91602=DIRECTION('center_axis',(-1.,0.,0.)) ;
#91603=DIRECTION('ref_axis',(0.,0.,-1.)) ;
#91604=DIRECTION('center_axis',(0.,0.,-1.)) ;
#91605=DIRECTION('ref_axis',(-1.,0.,0.)) ;
#91606=DIRECTION('',(0.,-1.,0.)) ;
#91607=DIRECTION('',(1.,0.,0.)) ;
#91608=DIRECTION('',(0.,1.,0.)) ;
#91609=DIRECTION('center_axis',(1.,0.,0.)) ;
#91610=DIRECTION('ref_axis',(0.,0.,-1.)) ;
#91611=DIRECTION('center_axis',(1.,0.,0.)) ;
#91612=DIRECTION('ref_axis',(0.,0.,1.)) ;
#91613=DIRECTION('',(1.,0.,0.)) ;
#91614=DIRECTION('center_axis',(-1.,0.,0.)) ;
#91615=DIRECTION('ref_axis',(0.,0.,-1.)) ;
#91616=DIRECTION('center_axis',(0.,1.,0.)) ;
#91617=DIRECTION('ref_axis',(0.,0.,1.)) ;
#91618=DIRECTION('',(0.,0.,-1.)) ;
#91619=DIRECTION('',(1.,0.,0.)) ;
#91620=DIRECTION('',(0.,0.,1.)) ;
#91621=DIRECTION('center_axis',(1.,0.,0.)) ;
#91622=DIRECTION('ref_axis',(0.,0.,-1.)) ;
#91623=DIRECTION('center_axis',(-1.,0.,0.)) ;
#91624=DIRECTION('ref_axis',(0.,1.7347234759768E-14,-1.)) ;
#91625=DIRECTION('',(1.,0.,0.)) ;
#91626=DIRECTION('center_axis',(1.,0.,0.)) ;
#91627=DIRECTION('ref_axis',(0.,0.,-1.)) ;
#91628=DIRECTION('center_axis',(0.,1.07081696047951E-16,-1.)) ;
#91629=DIRECTION('ref_axis',(0.,1.,1.07081696047951E-16)) ;
#91630=DIRECTION('',(0.,-1.,-1.07081696047951E-16)) ;
#91631=DIRECTION('',(1.,0.,0.)) ;
#91632=DIRECTION('',(0.,1.,1.07081696047951E-16)) ;
#91633=DIRECTION('center_axis',(1.,0.,0.)) ;
#91634=DIRECTION('ref_axis',(0.,0.,-1.)) ;
#91635=DIRECTION('center_axis',(-1.,0.,0.)) ;
#91636=DIRECTION('ref_axis',(0.,0.,-1.)) ;
#91637=DIRECTION('',(1.,0.,0.)) ;
#91638=DIRECTION('center_axis',(1.,0.,0.)) ;
#91639=DIRECTION('ref_axis',(0.,0.,-1.)) ;
#91640=DIRECTION('center_axis',(0.,-1.,0.)) ;
#91641=DIRECTION('ref_axis',(0.,0.,-1.)) ;
#91642=DIRECTION('',(0.,0.,1.)) ;
#91643=DIRECTION('',(1.,0.,0.)) ;
#91644=DIRECTION('',(0.,0.,-1.)) ;
#91645=DIRECTION('center_axis',(1.,0.,0.)) ;
#91646=DIRECTION('ref_axis',(0.,0.,-1.)) ;
#91647=DIRECTION('center_axis',(-1.,0.,0.)) ;
#91648=DIRECTION('ref_axis',(0.,0.,-1.)) ;
#91649=DIRECTION('',(1.,0.,0.)) ;
#91650=DIRECTION('center_axis',(1.,0.,0.)) ;
#91651=DIRECTION('ref_axis',(0.,0.,-1.)) ;
#91652=DIRECTION('center_axis',(1.,0.,0.)) ;
#91653=DIRECTION('ref_axis',(0.,0.,-1.)) ;
#91654=DIRECTION('center_axis',(1.,0.,0.)) ;
#91655=DIRECTION('ref_axis',(0.,-7.85535158932894E-16,1.)) ;
#91656=DIRECTION('',(1.,0.,0.)) ;
#91657=DIRECTION('center_axis',(-1.,0.,0.)) ;
#91658=DIRECTION('ref_axis',(0.,-7.85535158932894E-16,-1.)) ;
#91659=DIRECTION('center_axis',(1.,0.,0.)) ;
#91660=DIRECTION('ref_axis',(0.,0.,-1.)) ;
#91661=DIRECTION('center_axis',(-1.,0.,0.)) ;
#91662=DIRECTION('ref_axis',(0.,0.,-1.)) ;
#91663=DIRECTION('',(1.,0.,0.)) ;
#91664=DIRECTION('center_axis',(1.,0.,0.)) ;
#91665=DIRECTION('ref_axis',(0.,0.,-1.)) ;
#91666=DIRECTION('center_axis',(0.,-1.,0.)) ;
#91667=DIRECTION('ref_axis',(0.,0.,-1.)) ;
#91668=DIRECTION('',(0.,0.,1.)) ;
#91669=DIRECTION('',(1.,0.,0.)) ;
#91670=DIRECTION('',(0.,0.,-1.)) ;
#91671=DIRECTION('center_axis',(1.,0.,0.)) ;
#91672=DIRECTION('ref_axis',(0.,0.,-1.)) ;
#91673=DIRECTION('center_axis',(-1.,0.,0.)) ;
#91674=DIRECTION('ref_axis',(0.,0.,-1.)) ;
#91675=DIRECTION('',(1.,0.,0.)) ;
#91676=DIRECTION('center_axis',(1.,0.,0.)) ;
#91677=DIRECTION('ref_axis',(0.,0.,-1.)) ;
#91678=DIRECTION('center_axis',(0.,-1.07081696047951E-16,1.)) ;
#91679=DIRECTION('ref_axis',(0.,-1.,-1.07081696047951E-16)) ;
#91680=DIRECTION('',(0.,1.,1.07081696047951E-16)) ;
#91681=DIRECTION('',(1.,0.,0.)) ;
#91682=DIRECTION('',(0.,-1.,-1.07081696047951E-16)) ;
#91683=DIRECTION('center_axis',(1.,0.,0.)) ;
#91684=DIRECTION('ref_axis',(0.,0.,-1.)) ;
#91685=DIRECTION('center_axis',(-1.,0.,0.)) ;
#91686=DIRECTION('ref_axis',(0.,0.,-1.)) ;
#91687=DIRECTION('',(1.,0.,0.)) ;
#91688=DIRECTION('center_axis',(1.,0.,0.)) ;
#91689=DIRECTION('ref_axis',(0.,0.,-1.)) ;
#91690=DIRECTION('center_axis',(0.,1.,0.)) ;
#91691=DIRECTION('ref_axis',(0.,0.,1.)) ;
#91692=DIRECTION('',(0.,0.,-1.)) ;
#91693=DIRECTION('',(0.,0.,1.)) ;
#91694=DIRECTION('center_axis',(-1.,0.,0.)) ;
#91695=DIRECTION('ref_axis',(0.,0.,1.)) ;
#91696=DIRECTION('center_axis',(-1.,0.,0.)) ;
#91697=DIRECTION('ref_axis',(0.,0.,1.)) ;
#91698=DIRECTION('',(0.,-1.,0.)) ;
#91699=DIRECTION('center_axis',(-1.,0.,0.)) ;
#91700=DIRECTION('ref_axis',(0.,0.,1.)) ;
#91701=DIRECTION('',(0.,0.,1.)) ;
#91702=DIRECTION('',(0.,-1.,-1.07081696047951E-16)) ;
#91703=DIRECTION('',(0.,0.,-1.)) ;
#91704=DIRECTION('center_axis',(-1.,0.,0.)) ;
#91705=DIRECTION('ref_axis',(0.,0.,1.)) ;
#91706=DIRECTION('',(0.,0.,-1.)) ;
#91707=DIRECTION('',(0.,1.,1.07081696047951E-16)) ;
#91708=DIRECTION('',(0.,0.,1.)) ;
#91709=DIRECTION('center_axis',(-1.,0.,0.)) ;
#91710=DIRECTION('ref_axis',(0.,0.,1.)) ;
#91711=DIRECTION('',(0.,1.,0.)) ;
#91712=DIRECTION('center_axis',(-1.,0.,0.)) ;
#91713=DIRECTION('ref_axis',(0.,0.,1.)) ;
#91714=DIRECTION('',(0.,0.,-1.)) ;
#91715=DIRECTION('',(0.,0.707106781186548,-0.707106781186547)) ;
#91716=DIRECTION('',(0.,0.,1.)) ;
#91717=DIRECTION('',(0.,-0.707106781186546,-0.707106781186549)) ;
#91718=DIRECTION('',(0.,-3.99416362155027E-15,-1.)) ;
#91719=DIRECTION('center_axis',(1.,0.,0.)) ;
#91720=DIRECTION('ref_axis',(0.,0.,-1.)) ;
#91721=DIRECTION('',(0.,-1.,0.)) ;
#91722=DIRECTION('center_axis',(-1.,0.,0.)) ;
#91723=DIRECTION('ref_axis',(0.,0.,-1.)) ;
#91724=DIRECTION('',(0.,0.,-1.)) ;
#91725=DIRECTION('center_axis',(-1.,0.,0.)) ;
#91726=DIRECTION('ref_axis',(0.,1.0842021724855E-15,-1.)) ;
#91727=DIRECTION('',(0.,-1.,0.)) ;
#91728=DIRECTION('center_axis',(-1.,0.,0.)) ;
#91729=DIRECTION('ref_axis',(0.,0.,-1.)) ;
#91730=DIRECTION('',(0.,0.,1.)) ;
#91731=DIRECTION('center_axis',(-1.,0.,0.)) ;
#91732=DIRECTION('ref_axis',(0.,0.,-1.)) ;
#91733=DIRECTION('center_axis',(1.,0.,0.)) ;
#91734=DIRECTION('ref_axis',(0.,0.,-1.)) ;
#91735=DIRECTION('',(0.,-1.,0.)) ;
#91736=DIRECTION('center_axis',(-1.,0.,0.)) ;
#91737=DIRECTION('ref_axis',(0.,0.,-1.)) ;
#91738=DIRECTION('',(0.,0.,-1.)) ;
#91739=DIRECTION('center_axis',(-1.,0.,0.)) ;
#91740=DIRECTION('ref_axis',(0.,-1.62630325872827E-15,-1.)) ;
#91741=DIRECTION('',(0.,-1.,0.)) ;
#91742=DIRECTION('center_axis',(-1.,0.,0.)) ;
#91743=DIRECTION('ref_axis',(0.,0.,-1.)) ;
#91744=DIRECTION('',(0.,0.,1.)) ;
#91745=DIRECTION('center_axis',(-1.,0.,0.)) ;
#91746=DIRECTION('ref_axis',(0.,0.,-1.)) ;
#91747=DIRECTION('center_axis',(1.,0.,0.)) ;
#91748=DIRECTION('ref_axis',(0.,0.,-1.)) ;
#91749=DIRECTION('',(0.,-1.,0.)) ;
#91750=DIRECTION('center_axis',(-1.,0.,0.)) ;
#91751=DIRECTION('ref_axis',(0.,0.,-1.)) ;
#91752=DIRECTION('',(0.,0.,-1.)) ;
#91753=DIRECTION('center_axis',(-1.,0.,0.)) ;
#91754=DIRECTION('ref_axis',(0.,0.,-1.)) ;
#91755=DIRECTION('',(0.,-1.,0.)) ;
#91756=DIRECTION('center_axis',(-1.,0.,0.)) ;
#91757=DIRECTION('ref_axis',(0.,0.,-1.)) ;
#91758=DIRECTION('',(0.,0.,1.)) ;
#91759=DIRECTION('center_axis',(-1.,0.,0.)) ;
#91760=DIRECTION('ref_axis',(0.,0.,-1.)) ;
#91761=DIRECTION('center_axis',(1.,0.,0.)) ;
#91762=DIRECTION('ref_axis',(0.,0.,-1.)) ;
#91763=DIRECTION('',(0.,-1.,0.)) ;
#91764=DIRECTION('center_axis',(-1.,0.,0.)) ;
#91765=DIRECTION('ref_axis',(0.,0.,-1.)) ;
#91766=DIRECTION('',(0.,0.,-1.)) ;
#91767=DIRECTION('center_axis',(-1.,0.,0.)) ;
#91768=DIRECTION('ref_axis',(0.,-1.62630325872827E-15,-1.)) ;
#91769=DIRECTION('',(0.,-1.,0.)) ;
#91770=DIRECTION('center_axis',(-1.,0.,0.)) ;
#91771=DIRECTION('ref_axis',(0.,0.,-1.)) ;
#91772=DIRECTION('',(0.,0.,1.)) ;
#91773=DIRECTION('center_axis',(-1.,0.,0.)) ;
#91774=DIRECTION('ref_axis',(0.,0.,-1.)) ;
#91775=DIRECTION('center_axis',(1.,0.,0.)) ;
#91776=DIRECTION('ref_axis',(0.,0.,-1.)) ;
#91777=DIRECTION('',(0.,-1.,0.)) ;
#91778=DIRECTION('center_axis',(-1.,0.,0.)) ;
#91779=DIRECTION('ref_axis',(0.,0.,-1.)) ;
#91780=DIRECTION('',(0.,0.,-1.)) ;
#91781=DIRECTION('center_axis',(-1.,0.,0.)) ;
#91782=DIRECTION('ref_axis',(0.,0.,-1.)) ;
#91783=DIRECTION('',(0.,-1.,0.)) ;
#91784=DIRECTION('center_axis',(-1.,0.,0.)) ;
#91785=DIRECTION('ref_axis',(0.,0.,-1.)) ;
#91786=DIRECTION('',(0.,0.,1.)) ;
#91787=DIRECTION('center_axis',(-1.,0.,0.)) ;
#91788=DIRECTION('ref_axis',(0.,0.,-1.)) ;
#91789=DIRECTION('center_axis',(1.,0.,0.)) ;
#91790=DIRECTION('ref_axis',(0.,0.,-1.)) ;
#91791=DIRECTION('',(0.,-1.,0.)) ;
#91792=DIRECTION('center_axis',(-1.,0.,0.)) ;
#91793=DIRECTION('ref_axis',(0.,0.,-1.)) ;
#91794=DIRECTION('',(0.,0.,-1.)) ;
#91795=DIRECTION('center_axis',(-1.,0.,0.)) ;
#91796=DIRECTION('ref_axis',(0.,0.,-1.)) ;
#91797=DIRECTION('',(0.,-1.,0.)) ;
#91798=DIRECTION('center_axis',(-1.,0.,0.)) ;
#91799=DIRECTION('ref_axis',(0.,0.,-1.)) ;
#91800=DIRECTION('',(0.,0.,1.)) ;
#91801=DIRECTION('center_axis',(-1.,0.,0.)) ;
#91802=DIRECTION('ref_axis',(0.,0.,-1.)) ;
#91803=DIRECTION('center_axis',(1.,0.,0.)) ;
#91804=DIRECTION('ref_axis',(0.,0.,-1.)) ;
#91805=DIRECTION('',(0.,-1.,0.)) ;
#91806=DIRECTION('center_axis',(-1.,0.,0.)) ;
#91807=DIRECTION('ref_axis',(0.,0.,-1.)) ;
#91808=DIRECTION('',(0.,0.,-1.)) ;
#91809=DIRECTION('center_axis',(-1.,0.,0.)) ;
#91810=DIRECTION('ref_axis',(0.,0.,-1.)) ;
#91811=DIRECTION('',(0.,-1.,0.)) ;
#91812=DIRECTION('center_axis',(-1.,0.,0.)) ;
#91813=DIRECTION('ref_axis',(0.,0.,-1.)) ;
#91814=DIRECTION('',(0.,0.,1.)) ;
#91815=DIRECTION('center_axis',(-1.,0.,0.)) ;
#91816=DIRECTION('ref_axis',(0.,0.,-1.)) ;
#91817=DIRECTION('center_axis',(1.,0.,0.)) ;
#91818=DIRECTION('ref_axis',(0.,0.,-1.)) ;
#91819=DIRECTION('',(0.,-1.,0.)) ;
#91820=DIRECTION('center_axis',(-1.,0.,0.)) ;
#91821=DIRECTION('ref_axis',(0.,0.,-1.)) ;
#91822=DIRECTION('',(0.,0.,-1.)) ;
#91823=DIRECTION('center_axis',(-1.,0.,0.)) ;
#91824=DIRECTION('ref_axis',(0.,0.,-1.)) ;
#91825=DIRECTION('',(0.,-1.,0.)) ;
#91826=DIRECTION('center_axis',(-1.,0.,0.)) ;
#91827=DIRECTION('ref_axis',(0.,0.,-1.)) ;
#91828=DIRECTION('',(0.,0.,1.)) ;
#91829=DIRECTION('center_axis',(-1.,0.,0.)) ;
#91830=DIRECTION('ref_axis',(0.,0.,-1.)) ;
#91831=DIRECTION('center_axis',(1.,0.,0.)) ;
#91832=DIRECTION('ref_axis',(0.,0.,-1.)) ;
#91833=DIRECTION('',(0.,-1.,0.)) ;
#91834=DIRECTION('center_axis',(-1.,0.,0.)) ;
#91835=DIRECTION('ref_axis',(0.,0.,-1.)) ;
#91836=DIRECTION('',(0.,0.,-1.)) ;
#91837=DIRECTION('center_axis',(-1.,0.,0.)) ;
#91838=DIRECTION('ref_axis',(0.,0.,-1.)) ;
#91839=DIRECTION('',(0.,-1.,0.)) ;
#91840=DIRECTION('center_axis',(-1.,0.,0.)) ;
#91841=DIRECTION('ref_axis',(0.,0.,-1.)) ;
#91842=DIRECTION('',(0.,0.,1.)) ;
#91843=DIRECTION('center_axis',(-1.,0.,0.)) ;
#91844=DIRECTION('ref_axis',(0.,0.,-1.)) ;
#91845=DIRECTION('center_axis',(1.53063836115601E-16,-1.,-1.30104260698261E-16)) ;
#91846=DIRECTION('ref_axis',(1.,1.53063836115601E-16,1.99142572374599E-32)) ;
#91847=DIRECTION('center_axis',(0.,1.,0.)) ;
#91848=DIRECTION('ref_axis',(0.,0.,1.)) ;
#91849=DIRECTION('center_axis',(0.,-1.,0.)) ;
#91850=DIRECTION('ref_axis',(0.,0.,-1.)) ;
#91851=DIRECTION('center_axis',(1.,1.53063836115601E-16,2.73691106313441E-48)) ;
#91852=DIRECTION('ref_axis',(-1.53063836115601E-16,1.,-4.18922106430579E-64)) ;
#91853=DIRECTION('center_axis',(-1.,0.,0.)) ;
#91854=DIRECTION('ref_axis',(0.,0.,1.)) ;
#91855=DIRECTION('center_axis',(1.,1.53063836115601E-16,0.)) ;
#91856=DIRECTION('ref_axis',(1.53063836115601E-16,-1.,0.)) ;
#91857=DIRECTION('center_axis',(0.,1.,0.)) ;
#91858=DIRECTION('ref_axis',(1.,0.,0.)) ;
#91859=DIRECTION('center_axis',(0.,1.,0.)) ;
#91860=DIRECTION('ref_axis',(0.,0.,-1.)) ;
#91861=DIRECTION('center_axis',(0.,0.,1.)) ;
#91862=DIRECTION('ref_axis',(-1.,0.,0.)) ;
#91863=DIRECTION('center_axis',(0.,1.,0.)) ;
#91864=DIRECTION('ref_axis',(1.,0.,0.)) ;
#91865=DIRECTION('center_axis',(0.,0.,1.)) ;
#91866=DIRECTION('ref_axis',(-1.,0.,0.)) ;
#91867=DIRECTION('center_axis',(1.,1.0842021724855E-15,0.)) ;
#91868=DIRECTION('ref_axis',(1.0842021724855E-15,-1.,0.)) ;
#91869=DIRECTION('center_axis',(-1.,-1.53063836115601E-16,0.)) ;
#91870=DIRECTION('ref_axis',(0.,-1.,0.)) ;
#91871=DIRECTION('center_axis',(0.,0.,-1.)) ;
#91872=DIRECTION('ref_axis',(1.,0.,0.)) ;
#91873=DIRECTION('center_axis',(0.,0.,-1.)) ;
#91874=DIRECTION('ref_axis',(0.804034447892617,0.594582716366709,0.)) ;
#91875=DIRECTION('center_axis',(0.,0.,1.)) ;
#91876=DIRECTION('ref_axis',(1.,0.,0.)) ;
#91877=DIRECTION('',(0.,0.,-1.)) ;
#91878=DIRECTION('center_axis',(-2.16840434497101E-16,1.,1.30104260698261E-16)) ;
#91879=DIRECTION('ref_axis',(1.,2.16840434497101E-16,1.22464679914735E-16)) ;
#91880=DIRECTION('',(-2.16840434497101E-16,1.,1.30104260698261E-16)) ;
#91881=DIRECTION('center_axis',(0.,1.,0.)) ;
#91882=DIRECTION('ref_axis',(0.,0.,1.)) ;
#91883=DIRECTION('center_axis',(-1.,-1.53063836115601E-16,-2.73691106313441E-48)) ;
#91884=DIRECTION('ref_axis',(1.53063836115601E-16,-1.,4.18922106430579E-64)) ;
#91885=DIRECTION('center_axis',(1.,2.16840434497101E-16,0.)) ;
#91886=DIRECTION('ref_axis',(2.16840434497101E-16,-1.,0.)) ;
#91887=DIRECTION('center_axis',(0.,0.,1.)) ;
#91888=DIRECTION('ref_axis',(1.,0.,0.)) ;
#91889=DIRECTION('center_axis',(-1.25542992828747E-32,1.020425574104E-16,
1.)) ;
#91890=DIRECTION('ref_axis',(-1.28107280532009E-48,-1.,1.020425574104E-16)) ;
#91891=DIRECTION('center_axis',(0.,0.,1.)) ;
#91892=DIRECTION('ref_axis',(1.,0.,0.)) ;
#91893=DIRECTION('center_axis',(0.,0.,-1.)) ;
#91894=DIRECTION('ref_axis',(-1.,0.,0.)) ;
#91895=DIRECTION('center_axis',(1.,1.53063836115601E-16,-2.73691106313441E-48)) ;
#91896=DIRECTION('ref_axis',(-1.53063836115601E-16,1.,4.18922106430579E-64)) ;
#91897=DIRECTION('center_axis',(-1.,0.,0.)) ;
#91898=DIRECTION('ref_axis',(0.,0.,1.)) ;
#91899=DIRECTION('center_axis',(1.,1.53063836115601E-16,0.)) ;
#91900=DIRECTION('ref_axis',(1.53063836115601E-16,-1.,0.)) ;
#91901=DIRECTION('center_axis',(0.,1.,0.)) ;
#91902=DIRECTION('ref_axis',(1.,0.,0.)) ;
#91903=DIRECTION('center_axis',(-1.,-2.16840434497101E-16,0.)) ;
#91904=DIRECTION('ref_axis',(0.,-1.,0.)) ;
#91905=DIRECTION('center_axis',(0.,0.,-1.)) ;
#91906=DIRECTION('ref_axis',(1.,0.,0.)) ;
#91907=DIRECTION('center_axis',(-1.25542992828747E-32,1.020425574104E-16,
1.)) ;
#91908=DIRECTION('ref_axis',(0.,-1.,0.)) ;
#91909=DIRECTION('center_axis',(0.,-1.,0.)) ;
#91910=DIRECTION('ref_axis',(-6.50521303491304E-15,0.,1.)) ;
#91911=DIRECTION('center_axis',(-1.,0.,0.)) ;
#91912=DIRECTION('ref_axis',(0.,0.,-1.)) ;
#91913=DIRECTION('center_axis',(-1.,-1.53063836115601E-16,0.)) ;
#91914=DIRECTION('ref_axis',(0.,-1.,0.)) ;
#91915=DIRECTION('center_axis',(0.,-1.,0.)) ;
#91916=DIRECTION('ref_axis',(0.,0.,1.)) ;
#91917=DIRECTION('center_axis',(0.,0.,-1.)) ;
#91918=DIRECTION('ref_axis',(-1.,0.,0.)) ;
#91919=DIRECTION('center_axis',(-4.33680868994202E-15,0.,-1.)) ;
#91920=DIRECTION('ref_axis',(-1.,0.,4.33680868994202E-15)) ;
#91921=DIRECTION('center_axis',(1.,1.53063836115601E-16,-3.06472600140763E-33)) ;
#91922=DIRECTION('ref_axis',(-1.53063836115601E-16,1.,4.69098718418678E-49)) ;
#91923=DIRECTION('center_axis',(-1.,0.,0.)) ;
#91924=DIRECTION('ref_axis',(0.,0.,1.)) ;
#91925=DIRECTION('center_axis',(-1.53063836115601E-16,1.,-1.020425574104E-16)) ;
#91926=DIRECTION('ref_axis',(-1.,-1.53063836115601E-16,1.3684555315672E-47)) ;
#91927=DIRECTION('',(1.53063836115601E-16,-1.,1.020425574104E-16)) ;
#91928=DIRECTION('center_axis',(0.,-1.,0.)) ;
#91929=DIRECTION('ref_axis',(0.,0.,-1.)) ;
#91930=DIRECTION('center_axis',(-1.53063836115601E-16,1.,-1.30104260698261E-16)) ;
#91931=DIRECTION('ref_axis',(-1.,-1.53063836115601E-16,1.99142572374599E-32)) ;
#91932=DIRECTION('center_axis',(0.,-1.,0.)) ;
#91933=DIRECTION('ref_axis',(0.,0.,-1.)) ;
#91934=DIRECTION('center_axis',(-1.,-1.53063836115601E-16,2.73691106313441E-48)) ;
#91935=DIRECTION('ref_axis',(1.53063836115601E-16,-1.,-4.18922106430579E-64)) ;
#91936=DIRECTION('center_axis',(1.,2.16840434497101E-16,0.)) ;
#91937=DIRECTION('ref_axis',(2.16840434497101E-16,-1.,0.)) ;
#91938=DIRECTION('center_axis',(-1.,0.,2.168404344971E-15)) ;
#91939=DIRECTION('ref_axis',(2.168404344971E-15,0.,1.)) ;
#91940=DIRECTION('center_axis',(-1.,-2.16840434497101E-16,0.)) ;
#91941=DIRECTION('ref_axis',(0.,-1.,0.)) ;
#91942=DIRECTION('center_axis',(0.,0.,1.)) ;
#91943=DIRECTION('ref_axis',(-1.,0.,0.)) ;
#91944=DIRECTION('center_axis',(0.,1.,0.)) ;
#91945=DIRECTION('ref_axis',(1.,0.,0.)) ;
#91946=DIRECTION('center_axis',(0.,1.,0.)) ;
#91947=DIRECTION('ref_axis',(0.,0.,-1.)) ;
#91948=DIRECTION('center_axis',(1.,0.,0.)) ;
#91949=DIRECTION('ref_axis',(0.,-1.,0.)) ;
#91950=DIRECTION('center_axis',(1.,6.50521303491304E-15,0.)) ;
#91951=DIRECTION('ref_axis',(-6.50521303491304E-15,1.,0.)) ;
#91952=DIRECTION('center_axis',(8.67361737988403E-15,1.,0.)) ;
#91953=DIRECTION('ref_axis',(-1.,8.67361737988403E-15,0.)) ;
#91954=DIRECTION('center_axis',(1.2303003375722E-16,-1.,1.020425574104E-16)) ;
#91955=DIRECTION('ref_axis',(1.,1.2303003375722E-16,-1.25542992828747E-32)) ;
#91956=DIRECTION('center_axis',(0.,1.,0.)) ;
#91957=DIRECTION('ref_axis',(0.,0.,1.)) ;
#91958=DIRECTION('center_axis',(0.,1.,0.)) ;
#91959=DIRECTION('ref_axis',(1.,0.,0.)) ;
#91960=DIRECTION('center_axis',(1.,1.2303003375722E-16,0.)) ;
#91961=DIRECTION('ref_axis',(1.2303003375722E-16,-1.,0.)) ;
#91962=DIRECTION('center_axis',(0.,0.,1.)) ;
#91963=DIRECTION('ref_axis',(-1.,0.,0.)) ;
#91964=DIRECTION('center_axis',(0.,1.,0.)) ;
#91965=DIRECTION('ref_axis',(1.,0.,0.)) ;
#91966=DIRECTION('center_axis',(0.,0.,-1.)) ;
#91967=DIRECTION('ref_axis',(1.,0.,0.)) ;
#91968=DIRECTION('center_axis',(0.,0.,-1.)) ;
#91969=DIRECTION('ref_axis',(-1.,0.,0.)) ;
#91970=DIRECTION('center_axis',(0.,0.,1.)) ;
#91971=DIRECTION('ref_axis',(1.,0.,0.)) ;
#91972=DIRECTION('center_axis',(-2.16840434497101E-16,1.,-1.020425574104E-16)) ;
#91973=DIRECTION('ref_axis',(-1.,-2.16840434497101E-16,5.47382212626882E-48)) ;
#91974=DIRECTION('center_axis',(0.,1.,0.)) ;
#91975=DIRECTION('ref_axis',(0.,0.,-1.)) ;
#91976=DIRECTION('center_axis',(1.,0.,1.25542992828747E-32)) ;
#91977=DIRECTION('ref_axis',(1.25542992828747E-32,0.,-1.)) ;
#91978=DIRECTION('center_axis',(1.,0.,0.)) ;
#91979=DIRECTION('ref_axis',(0.,0.,-1.)) ;
#91980=DIRECTION('center_axis',(-1.,-1.2303003375722E-16,0.)) ;
#91981=DIRECTION('ref_axis',(0.,-1.,0.)) ;
#91982=DIRECTION('center_axis',(0.,0.,-1.)) ;
#91983=DIRECTION('ref_axis',(1.,0.,0.)) ;
#91984=DIRECTION('center_axis',(0.,0.,-1.)) ;
#91985=DIRECTION('ref_axis',(-1.,0.,0.)) ;
#91986=DIRECTION('',(0.,0.,1.)) ;
#91987=DIRECTION('center_axis',(0.,0.,1.)) ;
#91988=DIRECTION('ref_axis',(1.,0.,0.)) ;
#91989=DIRECTION('center_axis',(0.,0.,1.)) ;
#91990=DIRECTION('ref_axis',(1.,0.,0.)) ;
#91991=DIRECTION('center_axis',(6.27714964143733E-33,-5.10212787052002E-17,
-1.)) ;
#91992=DIRECTION('ref_axis',(3.20268201330022E-49,1.,-5.10212787052002E-17)) ;
#91993=DIRECTION('center_axis',(1.,1.53063836115601E-16,-1.53236300070382E-33)) ;
#91994=DIRECTION('ref_axis',(-1.53063836115601E-16,1.,2.34549359209339E-49)) ;
#91995=DIRECTION('center_axis',(-1.,0.,0.)) ;
#91996=DIRECTION('ref_axis',(0.,0.,1.)) ;
#91997=DIRECTION('center_axis',(1.,0.,0.)) ;
#91998=DIRECTION('ref_axis',(0.,0.,-1.)) ;
#91999=DIRECTION('center_axis',(0.,1.,0.)) ;
#92000=DIRECTION('ref_axis',(1.,0.,0.)) ;
#92001=DIRECTION('center_axis',(-4.33680868994202E-15,1.,0.)) ;
#92002=DIRECTION('ref_axis',(1.,4.33680868994202E-15,0.)) ;
#92003=DIRECTION('center_axis',(0.,-1.,0.)) ;
#92004=DIRECTION('ref_axis',(0.,0.,-1.)) ;
#92005=DIRECTION('center_axis',(0.,0.,-1.)) ;
#92006=DIRECTION('ref_axis',(1.,0.,0.)) ;
#92007=DIRECTION('center_axis',(0.,0.,1.)) ;
#92008=DIRECTION('ref_axis',(1.,0.,0.)) ;
#92009=DIRECTION('center_axis',(0.,0.,-1.)) ;
#92010=DIRECTION('ref_axis',(-1.,0.,0.)) ;
#92011=DIRECTION('center_axis',(0.,1.,0.)) ;
#92012=DIRECTION('ref_axis',(1.,0.,0.)) ;
#92013=DIRECTION('center_axis',(1.,1.2303003375722E-16,0.)) ;
#92014=DIRECTION('ref_axis',(1.2303003375722E-16,-1.,0.)) ;
#92015=DIRECTION('center_axis',(0.,1.,0.)) ;
#92016=DIRECTION('ref_axis',(-6.50521303491301E-15,0.,-1.)) ;
#92017=DIRECTION('center_axis',(6.27714964143733E-33,-5.10212787052002E-17,
-1.)) ;
#92018=DIRECTION('ref_axis',(0.,1.,0.)) ;
#92019=DIRECTION('center_axis',(0.,-1.,0.)) ;
#92020=DIRECTION('ref_axis',(0.,0.,1.)) ;
#92021=DIRECTION('center_axis',(2.16840434497101E-16,-1.,5.10212787052002E-17)) ;
#92022=DIRECTION('ref_axis',(1.,2.16840434497101E-16,-5.47382212626882E-48)) ;
#92023=DIRECTION('center_axis',(0.,1.,0.)) ;
#92024=DIRECTION('ref_axis',(0.,0.,-1.)) ;
#92025=DIRECTION('center_axis',(0.,0.,1.)) ;
#92026=DIRECTION('ref_axis',(1.,0.,0.)) ;
#92027=DIRECTION('center_axis',(0.,0.,-1.)) ;
#92028=DIRECTION('ref_axis',(-1.,0.,0.)) ;
#92029=DIRECTION('center_axis',(-1.,-1.2303003375722E-16,0.)) ;
#92030=DIRECTION('ref_axis',(0.,-1.,0.)) ;
#92031=DIRECTION('center_axis',(0.,-1.,0.)) ;
#92032=DIRECTION('ref_axis',(0.,0.,1.)) ;
#92033=DIRECTION('center_axis',(1.53063836115601E-16,-1.,5.10212787052002E-17)) ;
#92034=DIRECTION('ref_axis',(1.,1.53063836115601E-16,-6.84227765783602E-48)) ;
#92035=DIRECTION('',(-1.53063836115601E-16,1.,-5.10212787052002E-17)) ;
#92036=DIRECTION('center_axis',(0.,-1.,0.)) ;
#92037=DIRECTION('ref_axis',(0.,0.,-1.)) ;
#92038=DIRECTION('center_axis',(-1.,0.,0.)) ;
#92039=DIRECTION('ref_axis',(0.,0.,-1.)) ;
#92040=DIRECTION('center_axis',(-1.2303003375722E-16,1.,-5.10212787052002E-17)) ;
#92041=DIRECTION('ref_axis',(-1.,-1.2303003375722E-16,6.27714964143733E-33)) ;
#92042=DIRECTION('center_axis',(-8.67361737988403E-15,-1.,0.)) ;
#92043=DIRECTION('ref_axis',(1.,-8.67361737988403E-15,0.)) ;
#92044=DIRECTION('center_axis',(1.,0.,6.27714964143733E-33)) ;
#92045=DIRECTION('ref_axis',(6.27714964143733E-33,0.,-1.)) ;
#92046=DIRECTION('center_axis',(-1.,0.,-6.50521303491318E-15)) ;
#92047=DIRECTION('ref_axis',(-6.50521303491318E-15,0.,1.)) ;
#92048=DIRECTION('center_axis',(1.,0.,0.)) ;
#92049=DIRECTION('ref_axis',(0.,1.,0.)) ;
#92050=DIRECTION('center_axis',(0.,0.,-1.)) ;
#92051=DIRECTION('ref_axis',(-1.,0.,0.)) ;
#92052=DIRECTION('center_axis',(0.,0.,1.)) ;
#92053=DIRECTION('ref_axis',(1.,0.,0.)) ;
#92054=DIRECTION('center_axis',(0.,0.,-1.)) ;
#92055=DIRECTION('ref_axis',(-1.,0.,0.)) ;
#92056=DIRECTION('center_axis',(-1.,0.,0.)) ;
#92057=DIRECTION('ref_axis',(0.,0.,1.)) ;
#92058=DIRECTION('center_axis',(0.,-1.,0.)) ;
#92059=DIRECTION('ref_axis',(0.,0.,-1.)) ;
#92060=DIRECTION('center_axis',(0.,1.,0.)) ;
#92061=DIRECTION('ref_axis',(0.,0.,1.)) ;
#92062=DIRECTION('center_axis',(0.,1.,-6.50521303491301E-15)) ;
#92063=DIRECTION('ref_axis',(0.,6.50521303491301E-15,1.)) ;
#92064=DIRECTION('center_axis',(0.,-1.,0.)) ;
#92065=DIRECTION('ref_axis',(0.,0.,-1.)) ;
#92066=DIRECTION('center_axis',(0.,-1.,0.)) ;
#92067=DIRECTION('ref_axis',(0.,0.,-1.)) ;
#92068=DIRECTION('center_axis',(0.,-1.,-1.07081696047951E-16)) ;
#92069=DIRECTION('ref_axis',(0.,1.07081696047951E-16,-1.)) ;
#92070=DIRECTION('center_axis',(0.,1.,0.)) ;
#92071=DIRECTION('ref_axis',(0.,0.,1.)) ;
#92072=DIRECTION('center_axis',(-1.,0.,0.)) ;
#92073=DIRECTION('ref_axis',(0.,0.,1.)) ;
#92074=DIRECTION('center_axis',(0.,0.,1.)) ;
#92075=DIRECTION('ref_axis',(1.,0.,0.)) ;
#92076=DIRECTION('center_axis',(0.,1.,0.)) ;
#92077=DIRECTION('ref_axis',(0.,0.,1.)) ;
#92078=DIRECTION('center_axis',(0.,0.,-1.)) ;
#92079=DIRECTION('ref_axis',(-1.,0.,0.)) ;
#92080=DIRECTION('center_axis',(0.,0.,1.)) ;
#92081=DIRECTION('ref_axis',(1.,0.,0.)) ;
#92082=DIRECTION('center_axis',(0.,0.,1.)) ;
#92083=DIRECTION('ref_axis',(1.,0.,0.)) ;
#92084=DIRECTION('center_axis',(0.,0.,1.)) ;
#92085=DIRECTION('ref_axis',(1.,0.,0.)) ;
#92086=DIRECTION('center_axis',(0.,0.,-1.)) ;
#92087=DIRECTION('ref_axis',(-1.,0.,0.)) ;
#92088=DIRECTION('center_axis',(0.,1.,0.)) ;
#92089=DIRECTION('ref_axis',(0.,0.,1.)) ;
#92090=DIRECTION('center_axis',(0.,-0.707106781186545,0.70710678118655)) ;
#92091=DIRECTION('ref_axis',(0.,-0.70710678118655,-0.707106781186545)) ;
#92092=DIRECTION('center_axis',(0.,1.,0.)) ;
#92093=DIRECTION('ref_axis',(0.,0.,1.)) ;
#92094=DIRECTION('center_axis',(0.,-0.514231796959101,-0.857651245551602)) ;
#92095=DIRECTION('ref_axis',(0.,0.857651245551602,-0.514231796959101)) ;
#92096=DIRECTION('center_axis',(0.,-0.707106781186548,0.707106781186547)) ;
#92097=DIRECTION('ref_axis',(0.,-0.707106781186547,-0.707106781186548)) ;
#92098=DIRECTION('center_axis',(0.,-0.707106781186552,0.707106781186543)) ;
#92099=DIRECTION('ref_axis',(0.,-0.707106781186543,-0.707106781186552)) ;
#92100=DIRECTION('center_axis',(-1.,0.,0.)) ;
#92101=DIRECTION('ref_axis',(0.,0.,1.)) ;
#92102=DIRECTION('center_axis',(0.,0.514231796959101,-0.857651245551602)) ;
#92103=DIRECTION('ref_axis',(0.,0.857651245551602,0.514231796959101)) ;
#92104=DIRECTION('center_axis',(0.,1.,0.)) ;
#92105=DIRECTION('ref_axis',(0.,0.,1.)) ;
#92106=DIRECTION('center_axis',(0.,0.,-1.)) ;
#92107=DIRECTION('ref_axis',(-1.,0.,0.)) ;
#92108=DIRECTION('center_axis',(0.,1.,0.)) ;
#92109=DIRECTION('ref_axis',(0.,0.,1.)) ;
#92110=DIRECTION('center_axis',(0.,0.,-1.)) ;
#92111=DIRECTION('ref_axis',(-1.,0.,0.)) ;
#92112=DIRECTION('center_axis',(0.,0.,-1.)) ;
#92113=DIRECTION('ref_axis',(-1.,0.,0.)) ;
#92114=DIRECTION('center_axis',(0.,0.,1.)) ;
#92115=DIRECTION('ref_axis',(1.,0.,0.)) ;
#92116=DIRECTION('center_axis',(0.,0.,-1.)) ;
#92117=DIRECTION('ref_axis',(-1.,0.,0.)) ;
#92118=DIRECTION('center_axis',(0.,1.,0.)) ;
#92119=DIRECTION('ref_axis',(0.,0.,1.)) ;
#92120=DIRECTION('center_axis',(0.,-1.,8.67361737988405E-15)) ;
#92121=DIRECTION('ref_axis',(0.,-8.67361737988405E-15,-1.)) ;
#92122=DIRECTION('center_axis',(0.,0.707106781186546,0.707106781186549)) ;
#92123=DIRECTION('ref_axis',(0.,-0.707106781186549,0.707106781186546)) ;
#92124=DIRECTION('center_axis',(0.,0.707106781186545,0.70710678118655)) ;
#92125=DIRECTION('ref_axis',(0.,-0.70710678118655,0.707106781186545)) ;
#92126=DIRECTION('center_axis',(0.,1.,1.07081696047951E-16)) ;
#92127=DIRECTION('ref_axis',(0.,-1.07081696047951E-16,1.)) ;
#92128=DIRECTION('center_axis',(0.,-1.,0.)) ;
#92129=DIRECTION('ref_axis',(0.,0.,-1.)) ;
#92130=DIRECTION('center_axis',(0.,1.,0.)) ;
#92131=DIRECTION('ref_axis',(0.,0.,1.)) ;
#92132=DIRECTION('center_axis',(0.,0.,1.)) ;
#92133=DIRECTION('ref_axis',(1.,0.,0.)) ;
#92134=DIRECTION('center_axis',(0.,1.,0.)) ;
#92135=DIRECTION('ref_axis',(0.,0.,1.)) ;
#92136=DIRECTION('center_axis',(0.,8.67361737988403E-15,1.)) ;
#92137=DIRECTION('ref_axis',(0.,-1.,8.67361737988403E-15)) ;
#92138=DIRECTION('center_axis',(0.,3.99416362155027E-15,1.)) ;
#92139=DIRECTION('ref_axis',(0.,-1.,3.99416362155027E-15)) ;
#92140=DIRECTION('center_axis',(0.,0.,1.)) ;
#92141=DIRECTION('ref_axis',(1.,0.,0.)) ;
#92142=DIRECTION('center_axis',(0.,0.,-1.)) ;
#92143=DIRECTION('ref_axis',(-1.,0.,0.)) ;
#92144=DIRECTION('center_axis',(0.,0.,1.)) ;
#92145=DIRECTION('ref_axis',(1.,0.,0.)) ;
#92146=DIRECTION('center_axis',(-1.,0.,0.)) ;
#92147=DIRECTION('ref_axis',(0.,0.,1.)) ;
#92148=DIRECTION('center_axis',(0.,1.,0.)) ;
#92149=DIRECTION('ref_axis',(0.,0.,1.)) ;
#92150=DIRECTION('center_axis',(-1.,0.,0.)) ;
#92151=DIRECTION('ref_axis',(0.,0.,1.)) ;
#92152=DIRECTION('center_axis',(0.,-1.,0.)) ;
#92153=DIRECTION('ref_axis',(0.,0.,-1.)) ;
#92154=DIRECTION('center_axis',(0.,1.,0.)) ;
#92155=DIRECTION('ref_axis',(0.,0.,1.)) ;
#92156=DIRECTION('center_axis',(0.,-1.,0.)) ;
#92157=DIRECTION('ref_axis',(0.,0.,-1.)) ;
#92158=DIRECTION('center_axis',(0.,1.,0.)) ;
#92159=DIRECTION('ref_axis',(0.,0.,1.)) ;
#92160=DIRECTION('center_axis',(0.,-1.,0.)) ;
#92161=DIRECTION('ref_axis',(0.,0.,-1.)) ;
#92162=DIRECTION('center_axis',(0.,1.,0.)) ;
#92163=DIRECTION('ref_axis',(0.,0.,-1.)) ;
#92164=DIRECTION('center_axis',(0.,0.,-1.)) ;
#92165=DIRECTION('ref_axis',(-1.,0.,0.)) ;
#92166=DIRECTION('center_axis',(0.,1.,0.)) ;
#92167=DIRECTION('ref_axis',(0.,0.,-1.)) ;
#92168=DIRECTION('center_axis',(0.,0.,-1.)) ;
#92169=DIRECTION('ref_axis',(-1.,0.,0.)) ;
#92170=DIRECTION('center_axis',(0.,0.,1.)) ;
#92171=DIRECTION('ref_axis',(1.,0.,0.)) ;
#92172=DIRECTION('center_axis',(0.,0.,-1.)) ;
#92173=DIRECTION('ref_axis',(-1.,0.,0.)) ;
#92174=DIRECTION('center_axis',(0.,0.,-1.)) ;
#92175=DIRECTION('ref_axis',(-1.,0.,0.)) ;
#92176=DIRECTION('center_axis',(0.,6.93889390390724E-14,-1.)) ;
#92177=DIRECTION('ref_axis',(0.,1.,6.93889390390724E-14)) ;
#92178=DIRECTION('center_axis',(1.,0.,0.)) ;
#92179=DIRECTION('ref_axis',(0.,0.,-1.)) ;
#92180=DIRECTION('center_axis',(3.0665868333667E-15,0.707106781186532,-0.707106781186563)) ;
#92181=DIRECTION('ref_axis',(-5.39294103027656E-31,0.707106781186563,0.707106781186532)) ;
#92182=DIRECTION('center_axis',(1.,0.,0.)) ;
#92183=DIRECTION('ref_axis',(0.,0.,-1.)) ;
#92184=DIRECTION('center_axis',(0.,-1.,0.)) ;
#92185=DIRECTION('ref_axis',(0.,0.,-1.)) ;
#92186=DIRECTION('center_axis',(0.,-0.707106781186548,0.707106781186547)) ;
#92187=DIRECTION('ref_axis',(0.,-0.707106781186547,-0.707106781186548)) ;
#92188=DIRECTION('center_axis',(0.,-1.,-1.07081696047951E-16)) ;
#92189=DIRECTION('ref_axis',(0.,1.07081696047951E-16,-1.)) ;
#92190=DIRECTION('center_axis',(0.,-1.,-8.67361737988379E-15)) ;
#92191=DIRECTION('ref_axis',(0.,8.67361737988379E-15,-1.)) ;
#92192=DIRECTION('center_axis',(1.,0.,0.)) ;
#92193=DIRECTION('ref_axis',(0.,0.,-1.)) ;
#92194=DIRECTION('center_axis',(0.,0.,1.)) ;
#92195=DIRECTION('ref_axis',(1.,0.,0.)) ;
#92196=DIRECTION('center_axis',(0.,0.,-1.)) ;
#92197=DIRECTION('ref_axis',(-1.,0.,0.)) ;
#92198=DIRECTION('center_axis',(0.,0.,1.)) ;
#92199=DIRECTION('ref_axis',(1.,0.,0.)) ;
#92200=DIRECTION('center_axis',(0.,0.,1.)) ;
#92201=DIRECTION('ref_axis',(1.,0.,0.)) ;
#92202=DIRECTION('center_axis',(0.,0.,1.)) ;
#92203=DIRECTION('ref_axis',(1.,0.,0.)) ;
#92204=DIRECTION('center_axis',(1.,0.,0.)) ;
#92205=DIRECTION('ref_axis',(0.,0.382683432365085,0.923879532511289)) ;
#92206=DIRECTION('center_axis',(-3.0665868333667E-15,-0.707106781186532,
-0.707106781186563)) ;
#92207=DIRECTION('ref_axis',(-5.39294103027656E-31,0.707106781186563,-0.707106781186532)) ;
#92208=DIRECTION('center_axis',(1.,0.,0.)) ;
#92209=DIRECTION('ref_axis',(0.,0.,-1.)) ;
#92210=DIRECTION('center_axis',(0.,0.514231796959126,0.857651245551587)) ;
#92211=DIRECTION('ref_axis',(0.,-0.857651245551587,0.514231796959126)) ;
#92212=DIRECTION('center_axis',(0.,0.707106781186546,0.707106781186549)) ;
#92213=DIRECTION('ref_axis',(0.,-0.707106781186549,0.707106781186546)) ;
#92214=DIRECTION('center_axis',(3.06658683336673E-15,-0.707106781186539,
-0.707106781186556)) ;
#92215=DIRECTION('ref_axis',(1.90456316695698E-29,0.707106781186556,-0.707106781186539)) ;
#92216=DIRECTION('center_axis',(1.,0.,0.)) ;
#92217=DIRECTION('ref_axis',(0.,0.,-1.)) ;
#92218=DIRECTION('center_axis',(0.,-0.514231796959058,0.857651245551628)) ;
#92219=DIRECTION('ref_axis',(0.,-0.857651245551628,-0.514231796959058)) ;
#92220=DIRECTION('center_axis',(1.,0.,0.)) ;
#92221=DIRECTION('ref_axis',(0.,0.,-1.)) ;
#92222=DIRECTION('center_axis',(0.,0.,-1.)) ;
#92223=DIRECTION('ref_axis',(-1.,0.,0.)) ;
#92224=DIRECTION('center_axis',(1.,0.,0.)) ;
#92225=DIRECTION('ref_axis',(0.,0.,-1.)) ;
#92226=DIRECTION('center_axis',(0.,0.,1.)) ;
#92227=DIRECTION('ref_axis',(1.,0.,0.)) ;
#92228=DIRECTION('center_axis',(0.,3.99416362155027E-15,1.)) ;
#92229=DIRECTION('ref_axis',(0.,-1.,3.99416362155027E-15)) ;
#92230=DIRECTION('center_axis',(0.,0.,-1.)) ;
#92231=DIRECTION('ref_axis',(-1.,0.,0.)) ;
#92232=DIRECTION('center_axis',(0.,0.,1.)) ;
#92233=DIRECTION('ref_axis',(1.,0.,0.)) ;
#92234=DIRECTION('center_axis',(0.,-6.93889390390724E-14,1.)) ;
#92235=DIRECTION('ref_axis',(0.,-1.,-6.93889390390724E-14)) ;
#92236=DIRECTION('center_axis',(0.,1.,0.)) ;
#92237=DIRECTION('ref_axis',(0.,0.,-1.)) ;
#92238=DIRECTION('center_axis',(0.,-1.,0.)) ;
#92239=DIRECTION('ref_axis',(0.,0.,-1.)) ;
#92240=DIRECTION('center_axis',(1.,0.,0.)) ;
#92241=DIRECTION('ref_axis',(0.,0.,-1.)) ;
#92242=DIRECTION('center_axis',(0.,1.,0.)) ;
#92243=DIRECTION('ref_axis',(0.,0.,1.)) ;
#92244=DIRECTION('center_axis',(0.,1.,0.)) ;
#92245=DIRECTION('ref_axis',(0.,0.,1.)) ;
#92246=DIRECTION('center_axis',(0.,-1.,0.)) ;
#92247=DIRECTION('ref_axis',(0.,0.,-1.)) ;
#92248=DIRECTION('center_axis',(0.,1.,1.07081696047951E-16)) ;
#92249=DIRECTION('ref_axis',(0.,-1.07081696047951E-16,1.)) ;
#92250=DIRECTION('center_axis',(0.,1.,6.50521303491284E-15)) ;
#92251=DIRECTION('ref_axis',(0.,-6.50521303491284E-15,1.)) ;
#92252=DIRECTION('center_axis',(0.,1.,0.)) ;
#92253=DIRECTION('ref_axis',(0.,0.,-1.)) ;
#92254=DIRECTION('center_axis',(0.,0.,1.)) ;
#92255=DIRECTION('ref_axis',(1.,0.,0.)) ;
#92256=DIRECTION('center_axis',(1.,0.,0.)) ;
#92257=DIRECTION('ref_axis',(0.,0.,-1.)) ;
#92258=DIRECTION('center_axis',(0.,0.,-1.)) ;
#92259=DIRECTION('ref_axis',(-1.,0.,0.)) ;
#92260=DIRECTION('center_axis',(0.,0.,-1.)) ;
#92261=DIRECTION('ref_axis',(-1.,0.,0.)) ;
#92262=DIRECTION('center_axis',(0.,-1.,0.)) ;
#92263=DIRECTION('ref_axis',(0.,0.,-1.)) ;
#92264=DIRECTION('center_axis',(0.,1.,0.)) ;
#92265=DIRECTION('ref_axis',(0.,0.,1.)) ;
#92266=DIRECTION('center_axis',(0.,-1.,0.)) ;
#92267=DIRECTION('ref_axis',(0.,0.,-1.)) ;
#92268=DIRECTION('center_axis',(0.,1.,0.)) ;
#92269=DIRECTION('ref_axis',(0.,0.,-1.)) ;
#92270=DIRECTION('center_axis',(0.,0.,-1.)) ;
#92271=DIRECTION('ref_axis',(-1.,0.,0.)) ;
#92272=DIRECTION('center_axis',(0.,1.,0.)) ;
#92273=DIRECTION('ref_axis',(0.,0.,-1.)) ;
#92274=DIRECTION('center_axis',(0.,0.,-1.)) ;
#92275=DIRECTION('ref_axis',(-1.,0.,0.)) ;
#92276=DIRECTION('center_axis',(0.,0.,1.)) ;
#92277=DIRECTION('ref_axis',(1.,0.,0.)) ;
#92278=DIRECTION('center_axis',(0.,0.,-1.)) ;
#92279=DIRECTION('ref_axis',(-1.,0.,0.)) ;
#92280=DIRECTION('center_axis',(0.,0.,-1.)) ;
#92281=DIRECTION('ref_axis',(-1.,0.,0.)) ;
#92282=DIRECTION('center_axis',(0.,0.,-1.)) ;
#92283=DIRECTION('ref_axis',(-1.,0.,0.)) ;
#92284=DIRECTION('center_axis',(1.,0.,0.)) ;
#92285=DIRECTION('ref_axis',(0.,0.,-1.)) ;
#92286=DIRECTION('center_axis',(3.0665868333667E-15,0.707106781186532,-0.707106781186563)) ;
#92287=DIRECTION('ref_axis',(-5.39294103027656E-31,0.707106781186563,0.707106781186532)) ;
#92288=DIRECTION('center_axis',(1.,0.,0.)) ;
#92289=DIRECTION('ref_axis',(0.,0.,-1.)) ;
#92290=DIRECTION('center_axis',(0.,-1.,0.)) ;
#92291=DIRECTION('ref_axis',(0.,0.,-1.)) ;
#92292=DIRECTION('center_axis',(0.,-0.707106781186548,0.707106781186547)) ;
#92293=DIRECTION('ref_axis',(0.,-0.707106781186547,-0.707106781186548)) ;
#92294=DIRECTION('center_axis',(0.,-1.,-1.07081696047951E-16)) ;
#92295=DIRECTION('ref_axis',(0.,1.07081696047951E-16,-1.)) ;
#92296=DIRECTION('center_axis',(0.,-1.,-8.67361737988379E-15)) ;
#92297=DIRECTION('ref_axis',(0.,8.67361737988379E-15,-1.)) ;
#92298=DIRECTION('center_axis',(1.,0.,0.)) ;
#92299=DIRECTION('ref_axis',(0.,0.,-1.)) ;
#92300=DIRECTION('center_axis',(0.,0.,1.)) ;
#92301=DIRECTION('ref_axis',(1.,0.,0.)) ;
#92302=DIRECTION('center_axis',(0.,0.,-1.)) ;
#92303=DIRECTION('ref_axis',(-1.,0.,0.)) ;
#92304=DIRECTION('center_axis',(0.,0.,1.)) ;
#92305=DIRECTION('ref_axis',(1.,0.,0.)) ;
#92306=DIRECTION('center_axis',(0.,0.,1.)) ;
#92307=DIRECTION('ref_axis',(1.,0.,0.)) ;
#92308=DIRECTION('center_axis',(0.,0.,1.)) ;
#92309=DIRECTION('ref_axis',(1.,0.,0.)) ;
#92310=DIRECTION('center_axis',(1.,0.,0.)) ;
#92311=DIRECTION('ref_axis',(0.,0.382683432365093,0.923879532511286)) ;
#92312=DIRECTION('center_axis',(6.13317366673366E-15,-0.707106781186563,
-0.707106781186532)) ;
#92313=DIRECTION('ref_axis',(-1.7381816909424E-29,0.707106781186532,-0.707106781186563)) ;
#92314=DIRECTION('center_axis',(1.,0.,0.)) ;
#92315=DIRECTION('ref_axis',(0.,0.,-1.)) ;
#92316=DIRECTION('center_axis',(0.,0.514231796959126,0.857651245551587)) ;
#92317=DIRECTION('ref_axis',(0.,-0.857651245551587,0.514231796959126)) ;
#92318=DIRECTION('center_axis',(0.,0.707106781186546,0.707106781186549)) ;
#92319=DIRECTION('ref_axis',(0.,-0.707106781186549,0.707106781186546)) ;
#92320=DIRECTION('center_axis',(3.06658683336673E-15,-0.707106781186539,
-0.707106781186556)) ;
#92321=DIRECTION('ref_axis',(1.90456316695698E-29,0.707106781186556,-0.707106781186539)) ;
#92322=DIRECTION('center_axis',(1.,0.,0.)) ;
#92323=DIRECTION('ref_axis',(0.,0.,-1.)) ;
#92324=DIRECTION('center_axis',(0.,-0.514231796959091,0.857651245551608)) ;
#92325=DIRECTION('ref_axis',(0.,-0.857651245551608,-0.514231796959091)) ;
#92326=DIRECTION('center_axis',(1.,0.,0.)) ;
#92327=DIRECTION('ref_axis',(0.,0.,-1.)) ;
#92328=DIRECTION('center_axis',(0.,0.,-1.)) ;
#92329=DIRECTION('ref_axis',(-1.,0.,0.)) ;
#92330=DIRECTION('center_axis',(1.,0.,0.)) ;
#92331=DIRECTION('ref_axis',(0.,0.,-1.)) ;
#92332=DIRECTION('center_axis',(0.,0.,1.)) ;
#92333=DIRECTION('ref_axis',(1.,0.,0.)) ;
#92334=DIRECTION('center_axis',(0.,3.99416362155027E-15,1.)) ;
#92335=DIRECTION('ref_axis',(0.,-1.,3.99416362155027E-15)) ;
#92336=DIRECTION('center_axis',(0.,0.,-1.)) ;
#92337=DIRECTION('ref_axis',(-1.,0.,0.)) ;
#92338=DIRECTION('center_axis',(0.,0.,1.)) ;
#92339=DIRECTION('ref_axis',(1.,0.,0.)) ;
#92340=DIRECTION('center_axis',(0.,0.,1.)) ;
#92341=DIRECTION('ref_axis',(1.,0.,0.)) ;
#92342=DIRECTION('center_axis',(0.,1.,0.)) ;
#92343=DIRECTION('ref_axis',(0.,0.,-1.)) ;
#92344=DIRECTION('center_axis',(0.,-1.,0.)) ;
#92345=DIRECTION('ref_axis',(0.,0.,-1.)) ;
#92346=DIRECTION('center_axis',(1.,0.,0.)) ;
#92347=DIRECTION('ref_axis',(0.,0.,-1.)) ;
#92348=DIRECTION('center_axis',(0.,1.,0.)) ;
#92349=DIRECTION('ref_axis',(0.,0.,1.)) ;
#92350=DIRECTION('center_axis',(0.,1.,0.)) ;
#92351=DIRECTION('ref_axis',(0.,0.,1.)) ;
#92352=DIRECTION('center_axis',(0.,-1.,0.)) ;
#92353=DIRECTION('ref_axis',(0.,0.,-1.)) ;
#92354=DIRECTION('center_axis',(0.,1.,1.07081696047951E-16)) ;
#92355=DIRECTION('ref_axis',(0.,-1.07081696047951E-16,1.)) ;
#92356=DIRECTION('center_axis',(0.,1.,6.50521303491307E-15)) ;
#92357=DIRECTION('ref_axis',(0.,-6.50521303491307E-15,1.)) ;
#92358=DIRECTION('center_axis',(0.,1.,0.)) ;
#92359=DIRECTION('ref_axis',(0.,0.,-1.)) ;
#92360=DIRECTION('center_axis',(0.,0.,1.)) ;
#92361=DIRECTION('ref_axis',(1.,0.,0.)) ;
#92362=DIRECTION('center_axis',(1.,0.,0.)) ;
#92363=DIRECTION('ref_axis',(0.,0.,-1.)) ;
#92364=DIRECTION('center_axis',(0.,0.,-1.)) ;
#92365=DIRECTION('ref_axis',(-1.,0.,0.)) ;
#92366=DIRECTION('center_axis',(0.,0.,-1.)) ;
#92367=DIRECTION('ref_axis',(-1.,0.,0.)) ;
#92368=DIRECTION('center_axis',(0.,-1.,0.)) ;
#92369=DIRECTION('ref_axis',(0.,0.,-1.)) ;
#92370=DIRECTION('center_axis',(0.,1.,0.)) ;
#92371=DIRECTION('ref_axis',(0.,0.,1.)) ;
#92372=DIRECTION('center_axis',(0.,-1.,0.)) ;
#92373=DIRECTION('ref_axis',(0.,0.,-1.)) ;
#92374=DIRECTION('center_axis',(0.,1.,0.)) ;
#92375=DIRECTION('ref_axis',(0.,0.,-1.)) ;
#92376=DIRECTION('center_axis',(0.,0.,-1.)) ;
#92377=DIRECTION('ref_axis',(-1.,0.,0.)) ;
#92378=DIRECTION('center_axis',(0.,1.,0.)) ;
#92379=DIRECTION('ref_axis',(0.,0.,-1.)) ;
#92380=DIRECTION('center_axis',(0.,0.,-1.)) ;
#92381=DIRECTION('ref_axis',(-1.,0.,0.)) ;
#92382=DIRECTION('center_axis',(0.,0.,1.)) ;
#92383=DIRECTION('ref_axis',(1.,0.,0.)) ;
#92384=DIRECTION('center_axis',(0.,0.,-1.)) ;
#92385=DIRECTION('ref_axis',(-1.,0.,0.)) ;
#92386=DIRECTION('center_axis',(0.,0.,-1.)) ;
#92387=DIRECTION('ref_axis',(-1.,0.,0.)) ;
#92388=DIRECTION('center_axis',(0.,0.,-1.)) ;
#92389=DIRECTION('ref_axis',(-1.,0.,0.)) ;
#92390=DIRECTION('center_axis',(1.,0.,0.)) ;
#92391=DIRECTION('ref_axis',(0.,0.,-1.)) ;
#92392=DIRECTION('center_axis',(-6.13317366673366E-15,0.707106781186563,
-0.707106781186532)) ;
#92393=DIRECTION('ref_axis',(-1.7381816909424E-29,0.707106781186532,0.707106781186563)) ;
#92394=DIRECTION('center_axis',(1.,0.,0.)) ;
#92395=DIRECTION('ref_axis',(0.,0.,-1.)) ;
#92396=DIRECTION('center_axis',(0.,-1.,0.)) ;
#92397=DIRECTION('ref_axis',(0.,0.,-1.)) ;
#92398=DIRECTION('center_axis',(0.,-0.707106781186548,0.707106781186547)) ;
#92399=DIRECTION('ref_axis',(0.,-0.707106781186547,-0.707106781186548)) ;
#92400=DIRECTION('center_axis',(0.,-1.,-1.07081696047951E-16)) ;
#92401=DIRECTION('ref_axis',(0.,1.07081696047951E-16,-1.)) ;
#92402=DIRECTION('center_axis',(0.,-1.,-8.67361737988409E-15)) ;
#92403=DIRECTION('ref_axis',(0.,8.67361737988409E-15,-1.)) ;
#92404=DIRECTION('center_axis',(1.,0.,0.)) ;
#92405=DIRECTION('ref_axis',(0.,0.,-1.)) ;
#92406=DIRECTION('center_axis',(0.,0.,1.)) ;
#92407=DIRECTION('ref_axis',(1.,0.,0.)) ;
#92408=DIRECTION('center_axis',(0.,0.,-1.)) ;
#92409=DIRECTION('ref_axis',(-1.,0.,0.)) ;
#92410=DIRECTION('center_axis',(0.,0.,1.)) ;
#92411=DIRECTION('ref_axis',(1.,0.,0.)) ;
#92412=DIRECTION('center_axis',(0.,0.,1.)) ;
#92413=DIRECTION('ref_axis',(1.,0.,0.)) ;
#92414=DIRECTION('center_axis',(0.,0.,1.)) ;
#92415=DIRECTION('ref_axis',(1.,0.,0.)) ;
#92416=DIRECTION('center_axis',(1.,0.,0.)) ;
#92417=DIRECTION('ref_axis',(0.,0.382683432365093,0.923879532511286)) ;
#92418=DIRECTION('center_axis',(6.13317366673366E-15,-0.707106781186563,
-0.707106781186532)) ;
#92419=DIRECTION('ref_axis',(-1.7381816909424E-29,0.707106781186532,-0.707106781186563)) ;
#92420=DIRECTION('center_axis',(1.,0.,0.)) ;
#92421=DIRECTION('ref_axis',(0.,0.,-1.)) ;
#92422=DIRECTION('center_axis',(0.,0.514231796959093,0.857651245551607)) ;
#92423=DIRECTION('ref_axis',(0.,-0.857651245551607,0.514231796959093)) ;
#92424=DIRECTION('center_axis',(0.,0.707106781186546,0.707106781186549)) ;
#92425=DIRECTION('ref_axis',(0.,-0.707106781186549,0.707106781186546)) ;
#92426=DIRECTION('center_axis',(3.06658683336673E-15,-0.707106781186539,
-0.707106781186556)) ;
#92427=DIRECTION('ref_axis',(1.90456316695698E-29,0.707106781186556,-0.707106781186539)) ;
#92428=DIRECTION('center_axis',(1.,0.,0.)) ;
#92429=DIRECTION('ref_axis',(0.,0.,-1.)) ;
#92430=DIRECTION('center_axis',(0.,-0.514231796959091,0.857651245551608)) ;
#92431=DIRECTION('ref_axis',(0.,-0.857651245551608,-0.514231796959091)) ;
#92432=DIRECTION('center_axis',(1.,0.,0.)) ;
#92433=DIRECTION('ref_axis',(0.,0.,-1.)) ;
#92434=DIRECTION('center_axis',(0.,0.,-1.)) ;
#92435=DIRECTION('ref_axis',(-1.,0.,0.)) ;
#92436=DIRECTION('center_axis',(1.,0.,0.)) ;
#92437=DIRECTION('ref_axis',(0.,0.,-1.)) ;
#92438=DIRECTION('center_axis',(0.,0.,1.)) ;
#92439=DIRECTION('ref_axis',(1.,0.,0.)) ;
#92440=DIRECTION('center_axis',(0.,3.99416362155027E-15,1.)) ;
#92441=DIRECTION('ref_axis',(0.,-1.,3.99416362155027E-15)) ;
#92442=DIRECTION('center_axis',(0.,0.,-1.)) ;
#92443=DIRECTION('ref_axis',(-1.,0.,0.)) ;
#92444=DIRECTION('center_axis',(0.,0.,1.)) ;
#92445=DIRECTION('ref_axis',(1.,0.,0.)) ;
#92446=DIRECTION('center_axis',(0.,0.,1.)) ;
#92447=DIRECTION('ref_axis',(1.,0.,0.)) ;
#92448=DIRECTION('center_axis',(0.,1.,0.)) ;
#92449=DIRECTION('ref_axis',(0.,0.,-1.)) ;
#92450=DIRECTION('center_axis',(0.,-1.,0.)) ;
#92451=DIRECTION('ref_axis',(0.,0.,-1.)) ;
#92452=DIRECTION('center_axis',(1.,0.,0.)) ;
#92453=DIRECTION('ref_axis',(0.,0.,-1.)) ;
#92454=DIRECTION('center_axis',(0.,1.,0.)) ;
#92455=DIRECTION('ref_axis',(0.,0.,1.)) ;
#92456=DIRECTION('center_axis',(0.,1.,0.)) ;
#92457=DIRECTION('ref_axis',(0.,0.,1.)) ;
#92458=DIRECTION('center_axis',(0.,-1.,0.)) ;
#92459=DIRECTION('ref_axis',(0.,0.,-1.)) ;
#92460=DIRECTION('center_axis',(0.,1.,1.07081696047951E-16)) ;
#92461=DIRECTION('ref_axis',(0.,-1.07081696047951E-16,1.)) ;
#92462=DIRECTION('center_axis',(0.,1.,6.50521303491307E-15)) ;
#92463=DIRECTION('ref_axis',(0.,-6.50521303491307E-15,1.)) ;
#92464=DIRECTION('center_axis',(0.,1.,0.)) ;
#92465=DIRECTION('ref_axis',(0.,0.,-1.)) ;
#92466=DIRECTION('center_axis',(0.,0.,1.)) ;
#92467=DIRECTION('ref_axis',(1.,0.,0.)) ;
#92468=DIRECTION('center_axis',(1.,0.,0.)) ;
#92469=DIRECTION('ref_axis',(0.,0.,-1.)) ;
#92470=DIRECTION('center_axis',(0.,0.,-1.)) ;
#92471=DIRECTION('ref_axis',(-1.,0.,0.)) ;
#92472=DIRECTION('center_axis',(0.,0.,-1.)) ;
#92473=DIRECTION('ref_axis',(-1.,0.,0.)) ;
#92474=DIRECTION('center_axis',(0.,-1.,0.)) ;
#92475=DIRECTION('ref_axis',(0.,0.,-1.)) ;
#92476=DIRECTION('center_axis',(0.,1.,0.)) ;
#92477=DIRECTION('ref_axis',(0.,0.,1.)) ;
#92478=DIRECTION('center_axis',(0.,-1.,0.)) ;
#92479=DIRECTION('ref_axis',(0.,0.,-1.)) ;
#92480=DIRECTION('center_axis',(0.,1.,0.)) ;
#92481=DIRECTION('ref_axis',(0.,0.,-1.)) ;
#92482=DIRECTION('center_axis',(0.,0.,-1.)) ;
#92483=DIRECTION('ref_axis',(-1.,0.,0.)) ;
#92484=DIRECTION('center_axis',(0.,1.,0.)) ;
#92485=DIRECTION('ref_axis',(0.,0.,-1.)) ;
#92486=DIRECTION('center_axis',(0.,0.,-1.)) ;
#92487=DIRECTION('ref_axis',(-1.,0.,0.)) ;
#92488=DIRECTION('center_axis',(0.,0.,1.)) ;
#92489=DIRECTION('ref_axis',(1.,0.,0.)) ;
#92490=DIRECTION('center_axis',(0.,0.,-1.)) ;
#92491=DIRECTION('ref_axis',(-1.,0.,0.)) ;
#92492=DIRECTION('center_axis',(0.,0.,-1.)) ;
#92493=DIRECTION('ref_axis',(-1.,0.,0.)) ;
#92494=DIRECTION('center_axis',(0.,0.,-1.)) ;
#92495=DIRECTION('ref_axis',(-1.,0.,0.)) ;
#92496=DIRECTION('center_axis',(1.,0.,0.)) ;
#92497=DIRECTION('ref_axis',(0.,0.,-1.)) ;
#92498=DIRECTION('center_axis',(-6.13317366673366E-15,0.707106781186563,
-0.707106781186532)) ;
#92499=DIRECTION('ref_axis',(-1.7381816909424E-29,0.707106781186532,0.707106781186563)) ;
#92500=DIRECTION('center_axis',(1.,0.,0.)) ;
#92501=DIRECTION('ref_axis',(0.,0.,-1.)) ;
#92502=DIRECTION('center_axis',(0.,-1.,0.)) ;
#92503=DIRECTION('ref_axis',(0.,0.,-1.)) ;
#92504=DIRECTION('center_axis',(0.,-0.707106781186548,0.707106781186547)) ;
#92505=DIRECTION('ref_axis',(0.,-0.707106781186547,-0.707106781186548)) ;
#92506=DIRECTION('center_axis',(0.,-1.,-1.07081696047951E-16)) ;
#92507=DIRECTION('ref_axis',(0.,1.07081696047951E-16,-1.)) ;
#92508=DIRECTION('center_axis',(0.,-1.,-8.67361737988409E-15)) ;
#92509=DIRECTION('ref_axis',(0.,8.67361737988409E-15,-1.)) ;
#92510=DIRECTION('center_axis',(1.,0.,0.)) ;
#92511=DIRECTION('ref_axis',(0.,0.,-1.)) ;
#92512=DIRECTION('center_axis',(0.,0.,1.)) ;
#92513=DIRECTION('ref_axis',(1.,0.,0.)) ;
#92514=DIRECTION('center_axis',(0.,0.,-1.)) ;
#92515=DIRECTION('ref_axis',(-1.,0.,0.)) ;
#92516=DIRECTION('center_axis',(0.,0.,1.)) ;
#92517=DIRECTION('ref_axis',(1.,0.,0.)) ;
#92518=DIRECTION('center_axis',(0.,0.,1.)) ;
#92519=DIRECTION('ref_axis',(1.,0.,0.)) ;
#92520=DIRECTION('center_axis',(0.,0.,1.)) ;
#92521=DIRECTION('ref_axis',(1.,0.,0.)) ;
#92522=DIRECTION('center_axis',(1.,0.,0.)) ;
#92523=DIRECTION('ref_axis',(0.,0.382683432365092,0.923879532511286)) ;
#92524=DIRECTION('center_axis',(6.13317366673366E-15,-0.707106781186563,
-0.707106781186532)) ;
#92525=DIRECTION('ref_axis',(-1.7381816909424E-29,0.707106781186532,-0.707106781186563)) ;
#92526=DIRECTION('center_axis',(1.,0.,0.)) ;
#92527=DIRECTION('ref_axis',(0.,0.,-1.)) ;
#92528=DIRECTION('center_axis',(0.,0.514231796959093,0.857651245551607)) ;
#92529=DIRECTION('ref_axis',(0.,-0.857651245551607,0.514231796959093)) ;
#92530=DIRECTION('center_axis',(0.,0.707106781186546,0.707106781186549)) ;
#92531=DIRECTION('ref_axis',(0.,-0.707106781186549,0.707106781186546)) ;
#92532=DIRECTION('center_axis',(3.06658683336673E-15,-0.707106781186539,
-0.707106781186556)) ;
#92533=DIRECTION('ref_axis',(1.90456316695698E-29,0.707106781186556,-0.707106781186539)) ;
#92534=DIRECTION('center_axis',(1.,0.,0.)) ;
#92535=DIRECTION('ref_axis',(0.,0.,-1.)) ;
#92536=DIRECTION('center_axis',(0.,-0.514231796959091,0.857651245551608)) ;
#92537=DIRECTION('ref_axis',(0.,-0.857651245551608,-0.514231796959091)) ;
#92538=DIRECTION('center_axis',(1.,0.,0.)) ;
#92539=DIRECTION('ref_axis',(0.,0.,-1.)) ;
#92540=DIRECTION('center_axis',(0.,0.,-1.)) ;
#92541=DIRECTION('ref_axis',(-1.,0.,0.)) ;
#92542=DIRECTION('center_axis',(1.,0.,0.)) ;
#92543=DIRECTION('ref_axis',(0.,0.,-1.)) ;
#92544=DIRECTION('center_axis',(0.,0.,1.)) ;
#92545=DIRECTION('ref_axis',(1.,0.,0.)) ;
#92546=DIRECTION('center_axis',(0.,3.99416362155027E-15,1.)) ;
#92547=DIRECTION('ref_axis',(0.,-1.,3.99416362155027E-15)) ;
#92548=DIRECTION('center_axis',(0.,0.,-1.)) ;
#92549=DIRECTION('ref_axis',(-1.,0.,0.)) ;
#92550=DIRECTION('center_axis',(0.,0.,1.)) ;
#92551=DIRECTION('ref_axis',(1.,0.,0.)) ;
#92552=DIRECTION('center_axis',(0.,0.,1.)) ;
#92553=DIRECTION('ref_axis',(1.,0.,0.)) ;
#92554=DIRECTION('center_axis',(0.,1.,0.)) ;
#92555=DIRECTION('ref_axis',(0.,0.,-1.)) ;
#92556=DIRECTION('center_axis',(0.,-1.,0.)) ;
#92557=DIRECTION('ref_axis',(0.,0.,-1.)) ;
#92558=DIRECTION('center_axis',(1.,0.,0.)) ;
#92559=DIRECTION('ref_axis',(0.,0.,-1.)) ;
#92560=DIRECTION('center_axis',(0.,1.,0.)) ;
#92561=DIRECTION('ref_axis',(0.,0.,1.)) ;
#92562=DIRECTION('center_axis',(0.,1.,0.)) ;
#92563=DIRECTION('ref_axis',(0.,0.,1.)) ;
#92564=DIRECTION('center_axis',(0.,-1.,0.)) ;
#92565=DIRECTION('ref_axis',(0.,0.,-1.)) ;
#92566=DIRECTION('center_axis',(0.,1.,1.07081696047951E-16)) ;
#92567=DIRECTION('ref_axis',(0.,-1.07081696047951E-16,1.)) ;
#92568=DIRECTION('center_axis',(0.,1.,6.50521303491307E-15)) ;
#92569=DIRECTION('ref_axis',(0.,-6.50521303491307E-15,1.)) ;
#92570=DIRECTION('center_axis',(0.,1.,0.)) ;
#92571=DIRECTION('ref_axis',(0.,0.,-1.)) ;
#92572=DIRECTION('center_axis',(0.,0.,1.)) ;
#92573=DIRECTION('ref_axis',(1.,0.,0.)) ;
#92574=DIRECTION('center_axis',(1.,0.,0.)) ;
#92575=DIRECTION('ref_axis',(0.,0.,-1.)) ;
#92576=DIRECTION('center_axis',(0.,0.,-1.)) ;
#92577=DIRECTION('ref_axis',(-1.,0.,0.)) ;
#92578=DIRECTION('center_axis',(0.,0.,-1.)) ;
#92579=DIRECTION('ref_axis',(-1.,0.,0.)) ;
#92580=DIRECTION('center_axis',(0.,-1.,0.)) ;
#92581=DIRECTION('ref_axis',(0.,0.,-1.)) ;
#92582=DIRECTION('center_axis',(0.,1.,0.)) ;
#92583=DIRECTION('ref_axis',(0.,0.,1.)) ;
#92584=DIRECTION('center_axis',(0.,-1.,0.)) ;
#92585=DIRECTION('ref_axis',(0.,0.,-1.)) ;
#92586=DIRECTION('center_axis',(0.,1.,0.)) ;
#92587=DIRECTION('ref_axis',(0.,0.,-1.)) ;
#92588=DIRECTION('center_axis',(0.,0.,-1.)) ;
#92589=DIRECTION('ref_axis',(-1.,0.,0.)) ;
#92590=DIRECTION('center_axis',(0.,1.,0.)) ;
#92591=DIRECTION('ref_axis',(0.,0.,-1.)) ;
#92592=DIRECTION('center_axis',(0.,0.,-1.)) ;
#92593=DIRECTION('ref_axis',(-1.,0.,0.)) ;
#92594=DIRECTION('center_axis',(0.,0.,1.)) ;
#92595=DIRECTION('ref_axis',(1.,0.,0.)) ;
#92596=DIRECTION('center_axis',(0.,0.,-1.)) ;
#92597=DIRECTION('ref_axis',(-1.,0.,0.)) ;
#92598=DIRECTION('center_axis',(0.,0.,-1.)) ;
#92599=DIRECTION('ref_axis',(-1.,0.,0.)) ;
#92600=DIRECTION('center_axis',(0.,0.,-1.)) ;
#92601=DIRECTION('ref_axis',(-1.,0.,0.)) ;
#92602=DIRECTION('center_axis',(1.,0.,0.)) ;
#92603=DIRECTION('ref_axis',(0.,0.,-1.)) ;
#92604=DIRECTION('center_axis',(-6.13317366673366E-15,0.707106781186563,
-0.707106781186532)) ;
#92605=DIRECTION('ref_axis',(-1.7381816909424E-29,0.707106781186532,0.707106781186563)) ;
#92606=DIRECTION('center_axis',(1.,0.,0.)) ;
#92607=DIRECTION('ref_axis',(0.,0.,-1.)) ;
#92608=DIRECTION('center_axis',(0.,-1.,0.)) ;
#92609=DIRECTION('ref_axis',(0.,0.,-1.)) ;
#92610=DIRECTION('center_axis',(0.,-0.707106781186548,0.707106781186547)) ;
#92611=DIRECTION('ref_axis',(0.,-0.707106781186547,-0.707106781186548)) ;
#92612=DIRECTION('center_axis',(0.,-1.,-1.07081696047951E-16)) ;
#92613=DIRECTION('ref_axis',(0.,1.07081696047951E-16,-1.)) ;
#92614=DIRECTION('center_axis',(0.,-1.,-8.67361737988409E-15)) ;
#92615=DIRECTION('ref_axis',(0.,8.67361737988409E-15,-1.)) ;
#92616=DIRECTION('center_axis',(1.,0.,0.)) ;
#92617=DIRECTION('ref_axis',(0.,0.,-1.)) ;
#92618=DIRECTION('center_axis',(0.,0.,1.)) ;
#92619=DIRECTION('ref_axis',(1.,0.,0.)) ;
#92620=DIRECTION('center_axis',(0.,0.,-1.)) ;
#92621=DIRECTION('ref_axis',(-1.,0.,0.)) ;
#92622=DIRECTION('center_axis',(0.,0.,1.)) ;
#92623=DIRECTION('ref_axis',(1.,0.,0.)) ;
#92624=DIRECTION('center_axis',(0.,0.,1.)) ;
#92625=DIRECTION('ref_axis',(1.,0.,0.)) ;
#92626=DIRECTION('center_axis',(0.,0.,1.)) ;
#92627=DIRECTION('ref_axis',(1.,0.,0.)) ;
#92628=DIRECTION('center_axis',(1.,0.,0.)) ;
#92629=DIRECTION('ref_axis',(0.,0.382683432365085,0.923879532511289)) ;
#92630=DIRECTION('center_axis',(6.13317366673366E-15,-0.707106781186563,
-0.707106781186532)) ;
#92631=DIRECTION('ref_axis',(-1.7381816909424E-29,0.707106781186532,-0.707106781186563)) ;
#92632=DIRECTION('center_axis',(1.,0.,0.)) ;
#92633=DIRECTION('ref_axis',(0.,0.,-1.)) ;
#92634=DIRECTION('center_axis',(0.,0.514231796959093,0.857651245551607)) ;
#92635=DIRECTION('ref_axis',(0.,-0.857651245551607,0.514231796959093)) ;
#92636=DIRECTION('center_axis',(0.,0.707106781186546,0.707106781186549)) ;
#92637=DIRECTION('ref_axis',(0.,-0.707106781186549,0.707106781186546)) ;
#92638=DIRECTION('center_axis',(3.06658683336673E-15,-0.707106781186539,
-0.707106781186556)) ;
#92639=DIRECTION('ref_axis',(1.90456316695698E-29,0.707106781186556,-0.707106781186539)) ;
#92640=DIRECTION('center_axis',(1.,0.,0.)) ;
#92641=DIRECTION('ref_axis',(0.,0.,-1.)) ;
#92642=DIRECTION('center_axis',(0.,-0.514231796959091,0.857651245551608)) ;
#92643=DIRECTION('ref_axis',(0.,-0.857651245551608,-0.514231796959091)) ;
#92644=DIRECTION('center_axis',(1.,0.,0.)) ;
#92645=DIRECTION('ref_axis',(0.,0.,-1.)) ;
#92646=DIRECTION('center_axis',(0.,0.,-1.)) ;
#92647=DIRECTION('ref_axis',(-1.,0.,0.)) ;
#92648=DIRECTION('center_axis',(1.,0.,0.)) ;
#92649=DIRECTION('ref_axis',(0.,0.,-1.)) ;
#92650=DIRECTION('center_axis',(0.,0.,1.)) ;
#92651=DIRECTION('ref_axis',(1.,0.,0.)) ;
#92652=DIRECTION('center_axis',(0.,3.99416362155027E-15,1.)) ;
#92653=DIRECTION('ref_axis',(0.,-1.,3.99416362155027E-15)) ;
#92654=DIRECTION('center_axis',(0.,0.,-1.)) ;
#92655=DIRECTION('ref_axis',(-1.,0.,0.)) ;
#92656=DIRECTION('center_axis',(0.,0.,1.)) ;
#92657=DIRECTION('ref_axis',(1.,0.,0.)) ;
#92658=DIRECTION('center_axis',(0.,0.,1.)) ;
#92659=DIRECTION('ref_axis',(1.,0.,0.)) ;
#92660=DIRECTION('center_axis',(0.,1.,0.)) ;
#92661=DIRECTION('ref_axis',(0.,0.,-1.)) ;
#92662=DIRECTION('center_axis',(0.,-1.,0.)) ;
#92663=DIRECTION('ref_axis',(0.,0.,-1.)) ;
#92664=DIRECTION('center_axis',(1.,0.,0.)) ;
#92665=DIRECTION('ref_axis',(0.,0.,-1.)) ;
#92666=DIRECTION('center_axis',(0.,1.,0.)) ;
#92667=DIRECTION('ref_axis',(0.,0.,1.)) ;
#92668=DIRECTION('center_axis',(0.,1.,0.)) ;
#92669=DIRECTION('ref_axis',(0.,0.,1.)) ;
#92670=DIRECTION('center_axis',(0.,-1.,0.)) ;
#92671=DIRECTION('ref_axis',(0.,0.,-1.)) ;
#92672=DIRECTION('center_axis',(0.,1.,1.07081696047951E-16)) ;
#92673=DIRECTION('ref_axis',(0.,-1.07081696047951E-16,1.)) ;
#92674=DIRECTION('center_axis',(0.,1.,6.50521303491307E-15)) ;
#92675=DIRECTION('ref_axis',(0.,-6.50521303491307E-15,1.)) ;
#92676=DIRECTION('center_axis',(0.,1.,0.)) ;
#92677=DIRECTION('ref_axis',(0.,0.,-1.)) ;
#92678=DIRECTION('center_axis',(0.,0.,1.)) ;
#92679=DIRECTION('ref_axis',(1.,0.,0.)) ;
#92680=DIRECTION('center_axis',(1.,0.,0.)) ;
#92681=DIRECTION('ref_axis',(0.,0.,-1.)) ;
#92682=DIRECTION('center_axis',(0.,0.,-1.)) ;
#92683=DIRECTION('ref_axis',(-1.,0.,0.)) ;
#92684=DIRECTION('center_axis',(0.,0.,-1.)) ;
#92685=DIRECTION('ref_axis',(-1.,0.,0.)) ;
#92686=DIRECTION('center_axis',(0.,-1.,0.)) ;
#92687=DIRECTION('ref_axis',(0.,0.,-1.)) ;
#92688=DIRECTION('center_axis',(0.,1.,0.)) ;
#92689=DIRECTION('ref_axis',(0.,0.,1.)) ;
#92690=DIRECTION('center_axis',(0.,-1.,0.)) ;
#92691=DIRECTION('ref_axis',(0.,0.,-1.)) ;
#92692=DIRECTION('center_axis',(0.,1.,0.)) ;
#92693=DIRECTION('ref_axis',(0.,0.,-1.)) ;
#92694=DIRECTION('center_axis',(0.,0.,-1.)) ;
#92695=DIRECTION('ref_axis',(-1.,0.,0.)) ;
#92696=DIRECTION('center_axis',(0.,1.,0.)) ;
#92697=DIRECTION('ref_axis',(0.,0.,-1.)) ;
#92698=DIRECTION('center_axis',(0.,0.,-1.)) ;
#92699=DIRECTION('ref_axis',(-1.,0.,0.)) ;
#92700=DIRECTION('center_axis',(0.,0.,1.)) ;
#92701=DIRECTION('ref_axis',(1.,0.,0.)) ;
#92702=DIRECTION('center_axis',(0.,0.,-1.)) ;
#92703=DIRECTION('ref_axis',(-1.,0.,0.)) ;
#92704=DIRECTION('center_axis',(0.,0.,-1.)) ;
#92705=DIRECTION('ref_axis',(-1.,0.,0.)) ;
#92706=DIRECTION('center_axis',(0.,0.,-1.)) ;
#92707=DIRECTION('ref_axis',(-1.,0.,0.)) ;
#92708=DIRECTION('center_axis',(1.,0.,0.)) ;
#92709=DIRECTION('ref_axis',(0.,0.,-1.)) ;
#92710=DIRECTION('center_axis',(-6.13317366673366E-15,0.707106781186563,
-0.707106781186532)) ;
#92711=DIRECTION('ref_axis',(-1.7381816909424E-29,0.707106781186532,0.707106781186563)) ;
#92712=DIRECTION('center_axis',(1.,0.,0.)) ;
#92713=DIRECTION('ref_axis',(0.,0.,-1.)) ;
#92714=DIRECTION('center_axis',(0.,-1.,0.)) ;
#92715=DIRECTION('ref_axis',(0.,0.,-1.)) ;
#92716=DIRECTION('center_axis',(0.,-0.707106781186548,0.707106781186547)) ;
#92717=DIRECTION('ref_axis',(0.,-0.707106781186547,-0.707106781186548)) ;
#92718=DIRECTION('center_axis',(0.,-1.,-1.07081696047951E-16)) ;
#92719=DIRECTION('ref_axis',(0.,1.07081696047951E-16,-1.)) ;
#92720=DIRECTION('center_axis',(0.,-1.,-8.67361737988409E-15)) ;
#92721=DIRECTION('ref_axis',(0.,8.67361737988409E-15,-1.)) ;
#92722=DIRECTION('center_axis',(1.,0.,0.)) ;
#92723=DIRECTION('ref_axis',(0.,0.,-1.)) ;
#92724=DIRECTION('center_axis',(0.,0.,1.)) ;
#92725=DIRECTION('ref_axis',(1.,0.,0.)) ;
#92726=DIRECTION('center_axis',(0.,0.,-1.)) ;
#92727=DIRECTION('ref_axis',(-1.,0.,0.)) ;
#92728=DIRECTION('center_axis',(0.,0.,1.)) ;
#92729=DIRECTION('ref_axis',(1.,0.,0.)) ;
#92730=DIRECTION('center_axis',(0.,0.,1.)) ;
#92731=DIRECTION('ref_axis',(1.,0.,0.)) ;
#92732=DIRECTION('center_axis',(0.,0.,1.)) ;
#92733=DIRECTION('ref_axis',(1.,0.,0.)) ;
#92734=DIRECTION('center_axis',(1.,0.,0.)) ;
#92735=DIRECTION('ref_axis',(0.,0.382683432365081,0.92387953251129)) ;
#92736=DIRECTION('center_axis',(0.,-0.707106781186548,-0.707106781186548)) ;
#92737=DIRECTION('ref_axis',(0.,0.707106781186548,-0.707106781186548)) ;
#92738=DIRECTION('center_axis',(1.,0.,0.)) ;
#92739=DIRECTION('ref_axis',(0.,0.,-1.)) ;
#92740=DIRECTION('center_axis',(0.,0.514231796959093,0.857651245551607)) ;
#92741=DIRECTION('ref_axis',(0.,-0.857651245551607,0.514231796959093)) ;
#92742=DIRECTION('center_axis',(0.,0.707106781186546,0.707106781186549)) ;
#92743=DIRECTION('ref_axis',(0.,-0.707106781186549,0.707106781186546)) ;
#92744=DIRECTION('center_axis',(0.,-0.707106781186548,-0.707106781186548)) ;
#92745=DIRECTION('ref_axis',(0.,0.707106781186548,-0.707106781186548)) ;
#92746=DIRECTION('center_axis',(1.,0.,0.)) ;
#92747=DIRECTION('ref_axis',(0.,0.,-1.)) ;
#92748=DIRECTION('center_axis',(0.,-0.514231796959109,0.857651245551597)) ;
#92749=DIRECTION('ref_axis',(0.,-0.857651245551597,-0.514231796959109)) ;
#92750=DIRECTION('center_axis',(1.,0.,0.)) ;
#92751=DIRECTION('ref_axis',(0.,0.,-1.)) ;
#92752=DIRECTION('center_axis',(0.,0.,-1.)) ;
#92753=DIRECTION('ref_axis',(-1.,0.,0.)) ;
#92754=DIRECTION('center_axis',(1.,0.,0.)) ;
#92755=DIRECTION('ref_axis',(0.,0.,-1.)) ;
#92756=DIRECTION('center_axis',(0.,0.,1.)) ;
#92757=DIRECTION('ref_axis',(1.,0.,0.)) ;
#92758=DIRECTION('center_axis',(0.,3.99416362155027E-15,1.)) ;
#92759=DIRECTION('ref_axis',(0.,-1.,3.99416362155027E-15)) ;
#92760=DIRECTION('center_axis',(0.,0.,-1.)) ;
#92761=DIRECTION('ref_axis',(-1.,0.,0.)) ;
#92762=DIRECTION('center_axis',(0.,0.,1.)) ;
#92763=DIRECTION('ref_axis',(1.,0.,0.)) ;
#92764=DIRECTION('center_axis',(0.,0.,1.)) ;
#92765=DIRECTION('ref_axis',(1.,0.,0.)) ;
#92766=DIRECTION('center_axis',(0.,1.,0.)) ;
#92767=DIRECTION('ref_axis',(0.,0.,-1.)) ;
#92768=DIRECTION('center_axis',(0.,-1.,0.)) ;
#92769=DIRECTION('ref_axis',(0.,0.,-1.)) ;
#92770=DIRECTION('center_axis',(1.,0.,0.)) ;
#92771=DIRECTION('ref_axis',(0.,0.,-1.)) ;
#92772=DIRECTION('center_axis',(0.,1.,0.)) ;
#92773=DIRECTION('ref_axis',(0.,0.,1.)) ;
#92774=DIRECTION('center_axis',(0.,1.,0.)) ;
#92775=DIRECTION('ref_axis',(0.,0.,1.)) ;
#92776=DIRECTION('center_axis',(0.,-1.,0.)) ;
#92777=DIRECTION('ref_axis',(0.,0.,-1.)) ;
#92778=DIRECTION('center_axis',(0.,1.,1.07081696047951E-16)) ;
#92779=DIRECTION('ref_axis',(0.,-1.07081696047951E-16,1.)) ;
#92780=DIRECTION('center_axis',(0.,1.,6.50521303491307E-15)) ;
#92781=DIRECTION('ref_axis',(0.,-6.50521303491307E-15,1.)) ;
#92782=DIRECTION('center_axis',(0.,1.,0.)) ;
#92783=DIRECTION('ref_axis',(0.,0.,-1.)) ;
#92784=DIRECTION('center_axis',(0.,0.,1.)) ;
#92785=DIRECTION('ref_axis',(1.,0.,0.)) ;
#92786=DIRECTION('center_axis',(1.,0.,0.)) ;
#92787=DIRECTION('ref_axis',(0.,0.,-1.)) ;
#92788=DIRECTION('center_axis',(0.,0.,-1.)) ;
#92789=DIRECTION('ref_axis',(-1.,0.,0.)) ;
#92790=DIRECTION('center_axis',(0.,0.,-1.)) ;
#92791=DIRECTION('ref_axis',(-1.,0.,0.)) ;
#92792=DIRECTION('center_axis',(0.,-1.,0.)) ;
#92793=DIRECTION('ref_axis',(0.,0.,-1.)) ;
#92794=DIRECTION('center_axis',(0.,1.,0.)) ;
#92795=DIRECTION('ref_axis',(0.,0.,1.)) ;
#92796=DIRECTION('center_axis',(0.,-1.,0.)) ;
#92797=DIRECTION('ref_axis',(0.,0.,-1.)) ;
#92798=DIRECTION('center_axis',(0.,1.,0.)) ;
#92799=DIRECTION('ref_axis',(0.,0.,-1.)) ;
#92800=DIRECTION('center_axis',(0.,0.,-1.)) ;
#92801=DIRECTION('ref_axis',(-1.,0.,0.)) ;
#92802=DIRECTION('center_axis',(0.,1.,0.)) ;
#92803=DIRECTION('ref_axis',(0.,0.,-1.)) ;
#92804=DIRECTION('center_axis',(0.,0.,-1.)) ;
#92805=DIRECTION('ref_axis',(-1.,0.,0.)) ;
#92806=DIRECTION('center_axis',(0.,0.,1.)) ;
#92807=DIRECTION('ref_axis',(1.,0.,0.)) ;
#92808=DIRECTION('center_axis',(0.,0.,-1.)) ;
#92809=DIRECTION('ref_axis',(-1.,0.,0.)) ;
#92810=DIRECTION('center_axis',(0.,0.,-1.)) ;
#92811=DIRECTION('ref_axis',(-1.,0.,0.)) ;
#92812=DIRECTION('center_axis',(0.,0.,-1.)) ;
#92813=DIRECTION('ref_axis',(-1.,0.,0.)) ;
#92814=DIRECTION('center_axis',(1.,0.,0.)) ;
#92815=DIRECTION('ref_axis',(0.,0.,-1.)) ;
#92816=DIRECTION('center_axis',(0.,0.707106781186548,-0.707106781186548)) ;
#92817=DIRECTION('ref_axis',(0.,0.707106781186548,0.707106781186548)) ;
#92818=DIRECTION('center_axis',(1.,0.,0.)) ;
#92819=DIRECTION('ref_axis',(0.,0.,-1.)) ;
#92820=DIRECTION('center_axis',(0.,-1.,0.)) ;
#92821=DIRECTION('ref_axis',(0.,0.,-1.)) ;
#92822=DIRECTION('center_axis',(0.,-0.707106781186548,0.707106781186547)) ;
#92823=DIRECTION('ref_axis',(0.,-0.707106781186547,-0.707106781186548)) ;
#92824=DIRECTION('center_axis',(0.,-1.,-1.07081696047951E-16)) ;
#92825=DIRECTION('ref_axis',(0.,1.07081696047951E-16,-1.)) ;
#92826=DIRECTION('center_axis',(0.,-1.,-8.67361737988409E-15)) ;
#92827=DIRECTION('ref_axis',(0.,8.67361737988409E-15,-1.)) ;
#92828=DIRECTION('center_axis',(1.,0.,0.)) ;
#92829=DIRECTION('ref_axis',(0.,0.,-1.)) ;
#92830=DIRECTION('center_axis',(0.,0.,1.)) ;
#92831=DIRECTION('ref_axis',(1.,0.,0.)) ;
#92832=DIRECTION('center_axis',(0.,0.,-1.)) ;
#92833=DIRECTION('ref_axis',(-1.,0.,0.)) ;
#92834=DIRECTION('center_axis',(0.,0.,1.)) ;
#92835=DIRECTION('ref_axis',(1.,0.,0.)) ;
#92836=DIRECTION('center_axis',(0.,0.,1.)) ;
#92837=DIRECTION('ref_axis',(1.,0.,0.)) ;
#92838=DIRECTION('center_axis',(0.,0.,1.)) ;
#92839=DIRECTION('ref_axis',(1.,0.,0.)) ;
#92840=DIRECTION('center_axis',(1.,0.,0.)) ;
#92841=DIRECTION('ref_axis',(0.,0.382683432365087,0.923879532511288)) ;
#92842=DIRECTION('center_axis',(0.,-0.707106781186548,-0.707106781186548)) ;
#92843=DIRECTION('ref_axis',(0.,0.707106781186548,-0.707106781186548)) ;
#92844=DIRECTION('center_axis',(1.,0.,0.)) ;
#92845=DIRECTION('ref_axis',(0.,0.,-1.)) ;
#92846=DIRECTION('center_axis',(0.,0.514231796959109,0.857651245551597)) ;
#92847=DIRECTION('ref_axis',(0.,-0.857651245551597,0.514231796959109)) ;
#92848=DIRECTION('center_axis',(0.,0.707106781186546,0.707106781186549)) ;
#92849=DIRECTION('ref_axis',(0.,-0.707106781186549,0.707106781186546)) ;
#92850=DIRECTION('center_axis',(0.,-0.707106781186548,-0.707106781186548)) ;
#92851=DIRECTION('ref_axis',(0.,0.707106781186548,-0.707106781186548)) ;
#92852=DIRECTION('center_axis',(1.,0.,0.)) ;
#92853=DIRECTION('ref_axis',(0.,0.,-1.)) ;
#92854=DIRECTION('center_axis',(0.,-0.514231796959109,0.857651245551597)) ;
#92855=DIRECTION('ref_axis',(0.,-0.857651245551597,-0.514231796959109)) ;
#92856=DIRECTION('center_axis',(1.,0.,0.)) ;
#92857=DIRECTION('ref_axis',(0.,0.,-1.)) ;
#92858=DIRECTION('center_axis',(0.,0.,-1.)) ;
#92859=DIRECTION('ref_axis',(-1.,0.,0.)) ;
#92860=DIRECTION('center_axis',(1.,0.,0.)) ;
#92861=DIRECTION('ref_axis',(0.,0.,-1.)) ;
#92862=DIRECTION('center_axis',(0.,0.,1.)) ;
#92863=DIRECTION('ref_axis',(1.,0.,0.)) ;
#92864=DIRECTION('center_axis',(0.,3.99416362155027E-15,1.)) ;
#92865=DIRECTION('ref_axis',(0.,-1.,3.99416362155027E-15)) ;
#92866=DIRECTION('center_axis',(0.,0.,-1.)) ;
#92867=DIRECTION('ref_axis',(-1.,0.,0.)) ;
#92868=DIRECTION('center_axis',(0.,0.,1.)) ;
#92869=DIRECTION('ref_axis',(1.,0.,0.)) ;
#92870=DIRECTION('center_axis',(0.,0.,1.)) ;
#92871=DIRECTION('ref_axis',(1.,0.,0.)) ;
#92872=DIRECTION('center_axis',(0.,1.,0.)) ;
#92873=DIRECTION('ref_axis',(0.,0.,-1.)) ;
#92874=DIRECTION('center_axis',(0.,-1.,0.)) ;
#92875=DIRECTION('ref_axis',(0.,0.,-1.)) ;
#92876=DIRECTION('center_axis',(1.,0.,0.)) ;
#92877=DIRECTION('ref_axis',(0.,0.,-1.)) ;
#92878=DIRECTION('center_axis',(0.,1.,0.)) ;
#92879=DIRECTION('ref_axis',(0.,0.,1.)) ;
#92880=DIRECTION('center_axis',(0.,1.,0.)) ;
#92881=DIRECTION('ref_axis',(0.,0.,1.)) ;
#92882=DIRECTION('center_axis',(0.,-1.,0.)) ;
#92883=DIRECTION('ref_axis',(0.,0.,-1.)) ;
#92884=DIRECTION('center_axis',(0.,1.,1.07081696047951E-16)) ;
#92885=DIRECTION('ref_axis',(0.,-1.07081696047951E-16,1.)) ;
#92886=DIRECTION('center_axis',(0.,1.,6.50521303491307E-15)) ;
#92887=DIRECTION('ref_axis',(0.,-6.50521303491307E-15,1.)) ;
#92888=DIRECTION('center_axis',(0.,1.,0.)) ;
#92889=DIRECTION('ref_axis',(0.,0.,-1.)) ;
#92890=DIRECTION('center_axis',(0.,0.,1.)) ;
#92891=DIRECTION('ref_axis',(1.,0.,0.)) ;
#92892=DIRECTION('center_axis',(1.,0.,0.)) ;
#92893=DIRECTION('ref_axis',(0.,0.,-1.)) ;
#92894=DIRECTION('center_axis',(0.,0.,-1.)) ;
#92895=DIRECTION('ref_axis',(-1.,0.,0.)) ;
#92896=DIRECTION('center_axis',(0.,0.,-1.)) ;
#92897=DIRECTION('ref_axis',(-1.,0.,0.)) ;
#92898=DIRECTION('center_axis',(0.,-1.,0.)) ;
#92899=DIRECTION('ref_axis',(0.,0.,-1.)) ;
#92900=DIRECTION('center_axis',(0.,1.,0.)) ;
#92901=DIRECTION('ref_axis',(0.,0.,1.)) ;
#92902=DIRECTION('center_axis',(0.,-1.,0.)) ;
#92903=DIRECTION('ref_axis',(0.,0.,-1.)) ;
#92904=DIRECTION('center_axis',(0.,1.,0.)) ;
#92905=DIRECTION('ref_axis',(0.,0.,-1.)) ;
#92906=DIRECTION('center_axis',(0.,0.,-1.)) ;
#92907=DIRECTION('ref_axis',(-1.,0.,0.)) ;
#92908=DIRECTION('center_axis',(0.,1.,0.)) ;
#92909=DIRECTION('ref_axis',(0.,0.,-1.)) ;
#92910=DIRECTION('center_axis',(0.,0.,-1.)) ;
#92911=DIRECTION('ref_axis',(-1.,0.,0.)) ;
#92912=DIRECTION('center_axis',(0.,0.,1.)) ;
#92913=DIRECTION('ref_axis',(1.,0.,0.)) ;
#92914=DIRECTION('center_axis',(0.,0.,-1.)) ;
#92915=DIRECTION('ref_axis',(-1.,0.,0.)) ;
#92916=DIRECTION('center_axis',(0.,0.,-1.)) ;
#92917=DIRECTION('ref_axis',(-1.,0.,0.)) ;
#92918=DIRECTION('center_axis',(0.,0.,-1.)) ;
#92919=DIRECTION('ref_axis',(-1.,0.,0.)) ;
#92920=DIRECTION('center_axis',(1.,0.,0.)) ;
#92921=DIRECTION('ref_axis',(0.,0.,-1.)) ;
#92922=DIRECTION('center_axis',(0.,0.707106781186548,-0.707106781186548)) ;
#92923=DIRECTION('ref_axis',(0.,0.707106781186548,0.707106781186548)) ;
#92924=DIRECTION('center_axis',(1.,0.,0.)) ;
#92925=DIRECTION('ref_axis',(0.,0.,-1.)) ;
#92926=DIRECTION('center_axis',(0.,-1.,0.)) ;
#92927=DIRECTION('ref_axis',(0.,0.,-1.)) ;
#92928=DIRECTION('center_axis',(0.,-0.707106781186548,0.707106781186547)) ;
#92929=DIRECTION('ref_axis',(0.,-0.707106781186547,-0.707106781186548)) ;
#92930=DIRECTION('center_axis',(0.,-1.,-1.07081696047951E-16)) ;
#92931=DIRECTION('ref_axis',(0.,1.07081696047951E-16,-1.)) ;
#92932=DIRECTION('center_axis',(0.,-1.,-8.67361737988409E-15)) ;
#92933=DIRECTION('ref_axis',(0.,8.67361737988409E-15,-1.)) ;
#92934=DIRECTION('center_axis',(1.,0.,0.)) ;
#92935=DIRECTION('ref_axis',(0.,0.,-1.)) ;
#92936=DIRECTION('center_axis',(0.,0.,1.)) ;
#92937=DIRECTION('ref_axis',(1.,0.,0.)) ;
#92938=DIRECTION('center_axis',(0.,0.,-1.)) ;
#92939=DIRECTION('ref_axis',(-1.,0.,0.)) ;
#92940=DIRECTION('center_axis',(0.,0.,1.)) ;
#92941=DIRECTION('ref_axis',(1.,0.,0.)) ;
#92942=DIRECTION('center_axis',(0.,0.,1.)) ;
#92943=DIRECTION('ref_axis',(1.,0.,0.)) ;
#92944=DIRECTION('center_axis',(0.,0.,1.)) ;
#92945=DIRECTION('ref_axis',(1.,0.,0.)) ;
#92946=DIRECTION('center_axis',(1.,0.,0.)) ;
#92947=DIRECTION('ref_axis',(0.,0.382683432365088,0.923879532511288)) ;
#92948=DIRECTION('center_axis',(0.,-0.707106781186548,-0.707106781186548)) ;
#92949=DIRECTION('ref_axis',(0.,0.707106781186548,-0.707106781186548)) ;
#92950=DIRECTION('center_axis',(1.,0.,0.)) ;
#92951=DIRECTION('ref_axis',(0.,0.,-1.)) ;
#92952=DIRECTION('center_axis',(0.,0.514231796959109,0.857651245551597)) ;
#92953=DIRECTION('ref_axis',(0.,-0.857651245551597,0.514231796959109)) ;
#92954=DIRECTION('center_axis',(0.,0.707106781186546,0.707106781186549)) ;
#92955=DIRECTION('ref_axis',(0.,-0.707106781186549,0.707106781186546)) ;
#92956=DIRECTION('center_axis',(0.,-0.707106781186548,-0.707106781186548)) ;
#92957=DIRECTION('ref_axis',(0.,0.707106781186548,-0.707106781186548)) ;
#92958=DIRECTION('center_axis',(1.,0.,0.)) ;
#92959=DIRECTION('ref_axis',(0.,0.,-1.)) ;
#92960=DIRECTION('center_axis',(0.,-0.514231796959101,0.857651245551602)) ;
#92961=DIRECTION('ref_axis',(0.,-0.857651245551602,-0.514231796959101)) ;
#92962=DIRECTION('center_axis',(1.,0.,0.)) ;
#92963=DIRECTION('ref_axis',(0.,0.,-1.)) ;
#92964=DIRECTION('center_axis',(0.,8.67361737988405E-15,-1.)) ;
#92965=DIRECTION('ref_axis',(0.,1.,8.67361737988405E-15)) ;
#92966=DIRECTION('center_axis',(1.,0.,0.)) ;
#92967=DIRECTION('ref_axis',(0.,0.,-1.)) ;
#92968=DIRECTION('center_axis',(0.,0.,1.)) ;
#92969=DIRECTION('ref_axis',(1.,0.,0.)) ;
#92970=DIRECTION('center_axis',(0.,3.99416362155027E-15,1.)) ;
#92971=DIRECTION('ref_axis',(0.,-1.,3.99416362155027E-15)) ;
#92972=DIRECTION('center_axis',(0.,0.,-1.)) ;
#92973=DIRECTION('ref_axis',(-1.,0.,0.)) ;
#92974=DIRECTION('center_axis',(0.,0.,1.)) ;
#92975=DIRECTION('ref_axis',(1.,0.,0.)) ;
#92976=DIRECTION('center_axis',(0.,0.,1.)) ;
#92977=DIRECTION('ref_axis',(1.,0.,0.)) ;
#92978=DIRECTION('center_axis',(0.,1.,0.)) ;
#92979=DIRECTION('ref_axis',(0.,0.,-1.)) ;
#92980=DIRECTION('center_axis',(0.,-1.,0.)) ;
#92981=DIRECTION('ref_axis',(0.,0.,-1.)) ;
#92982=DIRECTION('center_axis',(1.,0.,0.)) ;
#92983=DIRECTION('ref_axis',(0.,0.,-1.)) ;
#92984=DIRECTION('center_axis',(0.,1.,0.)) ;
#92985=DIRECTION('ref_axis',(0.,0.,1.)) ;
#92986=DIRECTION('center_axis',(0.,1.,0.)) ;
#92987=DIRECTION('ref_axis',(0.,0.,1.)) ;
#92988=DIRECTION('center_axis',(0.,-1.,0.)) ;
#92989=DIRECTION('ref_axis',(0.,0.,-1.)) ;
#92990=DIRECTION('center_axis',(0.,1.,1.07081696047951E-16)) ;
#92991=DIRECTION('ref_axis',(0.,-1.07081696047951E-16,1.)) ;
#92992=DIRECTION('center_axis',(0.,1.,6.50521303491301E-15)) ;
#92993=DIRECTION('ref_axis',(0.,-6.50521303491301E-15,1.)) ;
#92994=DIRECTION('center_axis',(0.,1.,0.)) ;
#92995=DIRECTION('ref_axis',(0.,0.,-1.)) ;
#92996=DIRECTION('center_axis',(0.,0.,1.)) ;
#92997=DIRECTION('ref_axis',(1.,0.,0.)) ;
#92998=DIRECTION('center_axis',(1.,0.,0.)) ;
#92999=DIRECTION('ref_axis',(0.,0.,-1.)) ;
#93000=DIRECTION('center_axis',(0.,0.,-1.)) ;
#93001=DIRECTION('ref_axis',(-1.,0.,0.)) ;
#93002=DIRECTION('center_axis',(0.,0.,-1.)) ;
#93003=DIRECTION('ref_axis',(-1.,0.,0.)) ;
#93004=DIRECTION('center_axis',(0.,-1.,0.)) ;
#93005=DIRECTION('ref_axis',(0.,0.,-1.)) ;
#93006=DIRECTION('center_axis',(0.,1.,0.)) ;
#93007=DIRECTION('ref_axis',(0.,0.,1.)) ;
#93008=DIRECTION('center_axis',(0.,-1.,0.)) ;
#93009=DIRECTION('ref_axis',(0.,0.,-1.)) ;
#93010=DIRECTION('center_axis',(0.,1.,0.)) ;
#93011=DIRECTION('ref_axis',(0.,0.,-1.)) ;
#93012=DIRECTION('center_axis',(0.,0.,-1.)) ;
#93013=DIRECTION('ref_axis',(-1.,0.,0.)) ;
#93014=DIRECTION('center_axis',(0.,1.,0.)) ;
#93015=DIRECTION('ref_axis',(0.,0.,-1.)) ;
#93016=DIRECTION('center_axis',(0.,0.,-1.)) ;
#93017=DIRECTION('ref_axis',(-1.,0.,0.)) ;
#93018=DIRECTION('center_axis',(0.,0.,1.)) ;
#93019=DIRECTION('ref_axis',(1.,0.,0.)) ;
#93020=DIRECTION('center_axis',(0.,0.,-1.)) ;
#93021=DIRECTION('ref_axis',(-1.,0.,0.)) ;
#93022=DIRECTION('center_axis',(0.,0.,-1.)) ;
#93023=DIRECTION('ref_axis',(-1.,0.,0.)) ;
#93024=DIRECTION('center_axis',(0.,8.67361737988405E-15,-1.)) ;
#93025=DIRECTION('ref_axis',(0.,1.,8.67361737988405E-15)) ;
#93026=DIRECTION('center_axis',(1.,0.,0.)) ;
#93027=DIRECTION('ref_axis',(0.,0.,-1.)) ;
#93028=DIRECTION('center_axis',(0.,0.707106781186548,-0.707106781186548)) ;
#93029=DIRECTION('ref_axis',(0.,0.707106781186548,0.707106781186548)) ;
#93030=DIRECTION('center_axis',(1.,0.,0.)) ;
#93031=DIRECTION('ref_axis',(0.,0.,-1.)) ;
#93032=DIRECTION('center_axis',(0.,-1.,0.)) ;
#93033=DIRECTION('ref_axis',(0.,0.,-1.)) ;
#93034=DIRECTION('center_axis',(0.,-0.707106781186548,0.707106781186547)) ;
#93035=DIRECTION('ref_axis',(0.,-0.707106781186547,-0.707106781186548)) ;
#93036=DIRECTION('center_axis',(0.,-1.,-1.07081696047951E-16)) ;
#93037=DIRECTION('ref_axis',(0.,1.07081696047951E-16,-1.)) ;
#93038=DIRECTION('center_axis',(0.,-1.,-8.67361737988401E-15)) ;
#93039=DIRECTION('ref_axis',(0.,8.67361737988401E-15,-1.)) ;
#93040=DIRECTION('center_axis',(1.,0.,0.)) ;
#93041=DIRECTION('ref_axis',(0.,0.,-1.)) ;
#93042=DIRECTION('center_axis',(0.,0.,1.)) ;
#93043=DIRECTION('ref_axis',(1.,0.,0.)) ;
#93044=DIRECTION('center_axis',(0.,0.,-1.)) ;
#93045=DIRECTION('ref_axis',(-1.,0.,0.)) ;
#93046=DIRECTION('center_axis',(0.,0.,1.)) ;
#93047=DIRECTION('ref_axis',(1.,0.,0.)) ;
#93048=DIRECTION('center_axis',(0.,0.,1.)) ;
#93049=DIRECTION('ref_axis',(1.,0.,0.)) ;
#93050=DIRECTION('center_axis',(0.,0.,1.)) ;
#93051=DIRECTION('ref_axis',(1.,0.,0.)) ;
#93052=DIRECTION('center_axis',(1.,0.,0.)) ;
#93053=DIRECTION('ref_axis',(0.,0.38268343236509,0.923879532511287)) ;
#93054=DIRECTION('center_axis',(0.,-0.70710678118655,-0.707106781186545)) ;
#93055=DIRECTION('ref_axis',(0.,0.707106781186545,-0.70710678118655)) ;
#93056=DIRECTION('center_axis',(1.,0.,0.)) ;
#93057=DIRECTION('ref_axis',(0.,0.,-1.)) ;
#93058=DIRECTION('center_axis',(0.,0.514231796959101,0.857651245551602)) ;
#93059=DIRECTION('ref_axis',(0.,-0.857651245551602,0.514231796959101)) ;
#93060=DIRECTION('center_axis',(0.,0.707106781186546,0.707106781186549)) ;
#93061=DIRECTION('ref_axis',(0.,-0.707106781186549,0.707106781186546)) ;
#93062=DIRECTION('center_axis',(1.88079096131567E-29,-0.707106781186545,
-0.70710678118655)) ;
#93063=DIRECTION('ref_axis',(7.62257770433106E-46,0.70710678118655,-0.707106781186545)) ;
#93064=DIRECTION('center_axis',(1.,0.,0.)) ;
#93065=DIRECTION('ref_axis',(0.,0.,-1.)) ;
#93066=DIRECTION('center_axis',(0.,-0.514231796959101,0.857651245551602)) ;
#93067=DIRECTION('ref_axis',(0.,-0.857651245551602,-0.514231796959101)) ;
#93068=DIRECTION('center_axis',(1.,0.,0.)) ;
#93069=DIRECTION('ref_axis',(0.,0.,-1.)) ;
#93070=DIRECTION('center_axis',(0.,0.,-1.)) ;
#93071=DIRECTION('ref_axis',(-1.,0.,0.)) ;
#93072=DIRECTION('center_axis',(1.,0.,0.)) ;
#93073=DIRECTION('ref_axis',(0.,0.,-1.)) ;
#93074=DIRECTION('center_axis',(0.,0.,1.)) ;
#93075=DIRECTION('ref_axis',(1.,0.,0.)) ;
#93076=DIRECTION('center_axis',(0.,3.99416362155027E-15,1.)) ;
#93077=DIRECTION('ref_axis',(0.,-1.,3.99416362155027E-15)) ;
#93078=DIRECTION('center_axis',(0.,-4.33680868994202E-15,-1.)) ;
#93079=DIRECTION('ref_axis',(0.,1.,-4.33680868994202E-15)) ;
#93080=DIRECTION('center_axis',(0.,0.,1.)) ;
#93081=DIRECTION('ref_axis',(1.,0.,0.)) ;
#93082=DIRECTION('center_axis',(0.,-4.33680868994202E-15,1.)) ;
#93083=DIRECTION('ref_axis',(0.,-1.,-4.33680868994202E-15)) ;
#93084=DIRECTION('center_axis',(0.,1.,0.)) ;
#93085=DIRECTION('ref_axis',(0.,0.,-1.)) ;
#93086=DIRECTION('center_axis',(0.,-1.,0.)) ;
#93087=DIRECTION('ref_axis',(0.,0.,-1.)) ;
#93088=DIRECTION('center_axis',(1.,0.,0.)) ;
#93089=DIRECTION('ref_axis',(0.,0.,-1.)) ;
#93090=DIRECTION('center_axis',(0.,1.,0.)) ;
#93091=DIRECTION('ref_axis',(0.,0.,1.)) ;
#93092=DIRECTION('center_axis',(0.,1.,0.)) ;
#93093=DIRECTION('ref_axis',(0.,0.,1.)) ;
#93094=DIRECTION('center_axis',(0.,-1.,0.)) ;
#93095=DIRECTION('ref_axis',(0.,0.,-1.)) ;
#93096=DIRECTION('center_axis',(0.,1.,1.07081696047951E-16)) ;
#93097=DIRECTION('ref_axis',(0.,-1.07081696047951E-16,1.)) ;
#93098=DIRECTION('center_axis',(0.,1.,6.50521303491304E-15)) ;
#93099=DIRECTION('ref_axis',(0.,-6.50521303491304E-15,1.)) ;
#93100=DIRECTION('center_axis',(0.,1.,0.)) ;
#93101=DIRECTION('ref_axis',(0.,0.,-1.)) ;
#93102=DIRECTION('center_axis',(0.,0.,1.)) ;
#93103=DIRECTION('ref_axis',(1.,0.,0.)) ;
#93104=DIRECTION('center_axis',(1.,0.,0.)) ;
#93105=DIRECTION('ref_axis',(0.,0.,-1.)) ;
#93106=DIRECTION('center_axis',(0.,0.,-1.)) ;
#93107=DIRECTION('ref_axis',(-1.,0.,0.)) ;
#93108=DIRECTION('center_axis',(0.,0.,-1.)) ;
#93109=DIRECTION('ref_axis',(-1.,0.,0.)) ;
#93110=DIRECTION('center_axis',(1.53063836115601E-16,-1.,-1.30104260698261E-16)) ;
#93111=DIRECTION('ref_axis',(1.,1.53063836115601E-16,1.99142572374599E-32)) ;
#93112=DIRECTION('center_axis',(0.,1.,0.)) ;
#93113=DIRECTION('ref_axis',(0.,0.,1.)) ;
#93114=DIRECTION('center_axis',(0.,-1.,0.)) ;
#93115=DIRECTION('ref_axis',(0.,0.,-1.)) ;
#93116=DIRECTION('center_axis',(1.,1.53063836115601E-16,2.73691106313441E-48)) ;
#93117=DIRECTION('ref_axis',(-1.53063836115601E-16,1.,-4.18922106430579E-64)) ;
#93118=DIRECTION('center_axis',(-1.,0.,0.)) ;
#93119=DIRECTION('ref_axis',(0.,0.,1.)) ;
#93120=DIRECTION('center_axis',(1.,1.53063836115601E-16,0.)) ;
#93121=DIRECTION('ref_axis',(1.53063836115601E-16,-1.,0.)) ;
#93122=DIRECTION('center_axis',(0.,1.,0.)) ;
#93123=DIRECTION('ref_axis',(1.,0.,0.)) ;
#93124=DIRECTION('center_axis',(0.,1.,0.)) ;
#93125=DIRECTION('ref_axis',(0.,0.,-1.)) ;
#93126=DIRECTION('center_axis',(0.,0.,1.)) ;
#93127=DIRECTION('ref_axis',(-1.,0.,0.)) ;
#93128=DIRECTION('center_axis',(0.,1.,0.)) ;
#93129=DIRECTION('ref_axis',(1.,0.,0.)) ;
#93130=DIRECTION('center_axis',(0.,0.,1.)) ;
#93131=DIRECTION('ref_axis',(-1.,0.,0.)) ;
#93132=DIRECTION('center_axis',(1.,1.0842021724855E-15,0.)) ;
#93133=DIRECTION('ref_axis',(1.0842021724855E-15,-1.,0.)) ;
#93134=DIRECTION('center_axis',(-1.,-1.53063836115601E-16,0.)) ;
#93135=DIRECTION('ref_axis',(0.,-1.,0.)) ;
#93136=DIRECTION('center_axis',(0.,0.,-1.)) ;
#93137=DIRECTION('ref_axis',(1.,0.,0.)) ;
#93138=DIRECTION('center_axis',(0.,0.,-1.)) ;
#93139=DIRECTION('ref_axis',(0.804034447892619,0.594582716366707,0.)) ;
#93140=DIRECTION('center_axis',(0.,0.,1.)) ;
#93141=DIRECTION('ref_axis',(1.,0.,0.)) ;
#93142=DIRECTION('',(0.,0.,-1.)) ;
#93143=DIRECTION('center_axis',(-2.16840434497101E-16,1.,1.30104260698261E-16)) ;
#93144=DIRECTION('ref_axis',(1.,2.16840434497101E-16,1.22464679914735E-16)) ;
#93145=DIRECTION('',(-2.16840434497101E-16,1.,1.30104260698261E-16)) ;
#93146=DIRECTION('center_axis',(0.,1.,0.)) ;
#93147=DIRECTION('ref_axis',(0.,0.,1.)) ;
#93148=DIRECTION('center_axis',(-1.,-1.53063836115601E-16,-2.73691106313441E-48)) ;
#93149=DIRECTION('ref_axis',(1.53063836115601E-16,-1.,4.18922106430579E-64)) ;
#93150=DIRECTION('center_axis',(1.,2.16840434497101E-16,0.)) ;
#93151=DIRECTION('ref_axis',(2.16840434497101E-16,-1.,0.)) ;
#93152=DIRECTION('center_axis',(0.,0.,1.)) ;
#93153=DIRECTION('ref_axis',(1.,0.,0.)) ;
#93154=DIRECTION('center_axis',(-1.25542992828747E-32,1.020425574104E-16,
1.)) ;
#93155=DIRECTION('ref_axis',(-1.28107280532009E-48,-1.,1.020425574104E-16)) ;
#93156=DIRECTION('center_axis',(0.,0.,1.)) ;
#93157=DIRECTION('ref_axis',(1.,0.,0.)) ;
#93158=DIRECTION('center_axis',(0.,0.,-1.)) ;
#93159=DIRECTION('ref_axis',(-1.,0.,0.)) ;
#93160=DIRECTION('center_axis',(1.,1.53063836115601E-16,-2.73691106313441E-48)) ;
#93161=DIRECTION('ref_axis',(-1.53063836115601E-16,1.,4.18922106430579E-64)) ;
#93162=DIRECTION('center_axis',(-1.,0.,0.)) ;
#93163=DIRECTION('ref_axis',(0.,0.,1.)) ;
#93164=DIRECTION('center_axis',(1.,1.53063836115601E-16,0.)) ;
#93165=DIRECTION('ref_axis',(1.53063836115601E-16,-1.,0.)) ;
#93166=DIRECTION('center_axis',(0.,1.,0.)) ;
#93167=DIRECTION('ref_axis',(1.,0.,0.)) ;
#93168=DIRECTION('center_axis',(-1.,-2.16840434497101E-16,0.)) ;
#93169=DIRECTION('ref_axis',(0.,-1.,0.)) ;
#93170=DIRECTION('center_axis',(0.,0.,-1.)) ;
#93171=DIRECTION('ref_axis',(1.,0.,0.)) ;
#93172=DIRECTION('center_axis',(-1.25542992828747E-32,1.020425574104E-16,
1.)) ;
#93173=DIRECTION('ref_axis',(0.,-1.,0.)) ;
#93174=DIRECTION('center_axis',(0.,-1.,0.)) ;
#93175=DIRECTION('ref_axis',(-6.50521303491301E-15,0.,1.)) ;
#93176=DIRECTION('center_axis',(-1.,0.,0.)) ;
#93177=DIRECTION('ref_axis',(0.,0.,-1.)) ;
#93178=DIRECTION('center_axis',(-1.,-1.53063836115601E-16,0.)) ;
#93179=DIRECTION('ref_axis',(0.,-1.,0.)) ;
#93180=DIRECTION('center_axis',(0.,-1.,0.)) ;
#93181=DIRECTION('ref_axis',(0.,0.,1.)) ;
#93182=DIRECTION('center_axis',(0.,0.,-1.)) ;
#93183=DIRECTION('ref_axis',(-1.,0.,0.)) ;
#93184=DIRECTION('center_axis',(0.,0.,-1.)) ;
#93185=DIRECTION('ref_axis',(-1.,0.,0.)) ;
#93186=DIRECTION('center_axis',(1.,1.53063836115601E-16,-3.06472600140763E-33)) ;
#93187=DIRECTION('ref_axis',(-1.53063836115601E-16,1.,4.69098718418678E-49)) ;
#93188=DIRECTION('center_axis',(-1.,0.,0.)) ;
#93189=DIRECTION('ref_axis',(0.,0.,1.)) ;
#93190=DIRECTION('center_axis',(-1.53063836115601E-16,1.,-1.020425574104E-16)) ;
#93191=DIRECTION('ref_axis',(-1.,-1.53063836115601E-16,1.3684555315672E-47)) ;
#93192=DIRECTION('',(1.53063836115601E-16,-1.,1.020425574104E-16)) ;
#93193=DIRECTION('center_axis',(0.,-1.,0.)) ;
#93194=DIRECTION('ref_axis',(0.,0.,-1.)) ;
#93195=DIRECTION('center_axis',(-1.53063836115601E-16,1.,-1.30104260698261E-16)) ;
#93196=DIRECTION('ref_axis',(-1.,-1.53063836115601E-16,1.99142572374599E-32)) ;
#93197=DIRECTION('center_axis',(0.,-1.,0.)) ;
#93198=DIRECTION('ref_axis',(0.,0.,-1.)) ;
#93199=DIRECTION('center_axis',(-1.,-1.53063836115601E-16,2.73691106313441E-48)) ;
#93200=DIRECTION('ref_axis',(1.53063836115601E-16,-1.,-4.18922106430579E-64)) ;
#93201=DIRECTION('center_axis',(1.,2.16840434497101E-16,0.)) ;
#93202=DIRECTION('ref_axis',(2.16840434497101E-16,-1.,0.)) ;
#93203=DIRECTION('center_axis',(-1.,0.,2.16840434497102E-15)) ;
#93204=DIRECTION('ref_axis',(2.16840434497102E-15,0.,1.)) ;
#93205=DIRECTION('center_axis',(-1.,-2.16840434497101E-16,0.)) ;
#93206=DIRECTION('ref_axis',(0.,-1.,0.)) ;
#93207=DIRECTION('center_axis',(0.,0.,1.)) ;
#93208=DIRECTION('ref_axis',(-1.,0.,0.)) ;
#93209=DIRECTION('center_axis',(0.,1.,0.)) ;
#93210=DIRECTION('ref_axis',(1.,0.,0.)) ;
#93211=DIRECTION('center_axis',(0.,1.,0.)) ;
#93212=DIRECTION('ref_axis',(0.,0.,-1.)) ;
#93213=DIRECTION('center_axis',(1.,0.,0.)) ;
#93214=DIRECTION('ref_axis',(0.,-1.,0.)) ;
#93215=DIRECTION('center_axis',(1.,6.50521303491304E-15,0.)) ;
#93216=DIRECTION('ref_axis',(-6.50521303491304E-15,1.,0.)) ;
#93217=DIRECTION('center_axis',(8.67361737988403E-15,1.,0.)) ;
#93218=DIRECTION('ref_axis',(-1.,8.67361737988403E-15,0.)) ;
#93219=DIRECTION('center_axis',(1.2303003375722E-16,-1.,1.020425574104E-16)) ;
#93220=DIRECTION('ref_axis',(1.,1.2303003375722E-16,-1.25542992828747E-32)) ;
#93221=DIRECTION('center_axis',(0.,1.,0.)) ;
#93222=DIRECTION('ref_axis',(0.,0.,1.)) ;
#93223=DIRECTION('center_axis',(0.,1.,0.)) ;
#93224=DIRECTION('ref_axis',(1.,0.,0.)) ;
#93225=DIRECTION('center_axis',(1.,1.2303003375722E-16,0.)) ;
#93226=DIRECTION('ref_axis',(1.2303003375722E-16,-1.,0.)) ;
#93227=DIRECTION('center_axis',(0.,0.,1.)) ;
#93228=DIRECTION('ref_axis',(-1.,0.,0.)) ;
#93229=DIRECTION('center_axis',(0.,1.,0.)) ;
#93230=DIRECTION('ref_axis',(1.,0.,0.)) ;
#93231=DIRECTION('center_axis',(0.,0.,-1.)) ;
#93232=DIRECTION('ref_axis',(1.,0.,0.)) ;
#93233=DIRECTION('center_axis',(0.,0.,-1.)) ;
#93234=DIRECTION('ref_axis',(-1.,0.,0.)) ;
#93235=DIRECTION('center_axis',(0.,0.,1.)) ;
#93236=DIRECTION('ref_axis',(1.,0.,0.)) ;
#93237=DIRECTION('center_axis',(-2.16840434497101E-16,1.,-1.020425574104E-16)) ;
#93238=DIRECTION('ref_axis',(-1.,-2.16840434497101E-16,5.47382212626882E-48)) ;
#93239=DIRECTION('center_axis',(0.,1.,0.)) ;
#93240=DIRECTION('ref_axis',(0.,0.,-1.)) ;
#93241=DIRECTION('center_axis',(1.,0.,1.25542992828747E-32)) ;
#93242=DIRECTION('ref_axis',(1.25542992828747E-32,0.,-1.)) ;
#93243=DIRECTION('center_axis',(1.,0.,0.)) ;
#93244=DIRECTION('ref_axis',(0.,0.,-1.)) ;
#93245=DIRECTION('center_axis',(-1.,-1.2303003375722E-16,0.)) ;
#93246=DIRECTION('ref_axis',(0.,-1.,0.)) ;
#93247=DIRECTION('center_axis',(0.,0.,-1.)) ;
#93248=DIRECTION('ref_axis',(1.,0.,0.)) ;
#93249=DIRECTION('center_axis',(0.,0.,-1.)) ;
#93250=DIRECTION('ref_axis',(-1.,0.,0.)) ;
#93251=DIRECTION('',(0.,0.,1.)) ;
#93252=DIRECTION('center_axis',(0.,0.,1.)) ;
#93253=DIRECTION('ref_axis',(1.,0.,0.)) ;
#93254=DIRECTION('center_axis',(0.,0.,1.)) ;
#93255=DIRECTION('ref_axis',(1.,0.,0.)) ;
#93256=DIRECTION('center_axis',(6.27714964143733E-33,-5.10212787052002E-17,
-1.)) ;
#93257=DIRECTION('ref_axis',(3.20268201330022E-49,1.,-5.10212787052002E-17)) ;
#93258=DIRECTION('center_axis',(1.,1.53063836115601E-16,-1.53236300070382E-33)) ;
#93259=DIRECTION('ref_axis',(-1.53063836115601E-16,1.,2.34549359209339E-49)) ;
#93260=DIRECTION('center_axis',(-1.,0.,0.)) ;
#93261=DIRECTION('ref_axis',(0.,0.,1.)) ;
#93262=DIRECTION('center_axis',(1.,0.,0.)) ;
#93263=DIRECTION('ref_axis',(0.,0.,-1.)) ;
#93264=DIRECTION('center_axis',(0.,1.,0.)) ;
#93265=DIRECTION('ref_axis',(1.,0.,0.)) ;
#93266=DIRECTION('center_axis',(-4.33680868994202E-15,1.,0.)) ;
#93267=DIRECTION('ref_axis',(1.,4.33680868994202E-15,0.)) ;
#93268=DIRECTION('center_axis',(0.,-1.,0.)) ;
#93269=DIRECTION('ref_axis',(0.,0.,-1.)) ;
#93270=DIRECTION('center_axis',(0.,0.,-1.)) ;
#93271=DIRECTION('ref_axis',(1.,0.,0.)) ;
#93272=DIRECTION('center_axis',(0.,0.,1.)) ;
#93273=DIRECTION('ref_axis',(1.,0.,0.)) ;
#93274=DIRECTION('center_axis',(0.,0.,-1.)) ;
#93275=DIRECTION('ref_axis',(-1.,0.,0.)) ;
#93276=DIRECTION('center_axis',(0.,1.,0.)) ;
#93277=DIRECTION('ref_axis',(1.,0.,0.)) ;
#93278=DIRECTION('center_axis',(1.,1.2303003375722E-16,0.)) ;
#93279=DIRECTION('ref_axis',(1.2303003375722E-16,-1.,0.)) ;
#93280=DIRECTION('center_axis',(0.,1.,0.)) ;
#93281=DIRECTION('ref_axis',(-6.50521303491307E-15,0.,-1.)) ;
#93282=DIRECTION('center_axis',(6.27714964143733E-33,-5.10212787052002E-17,
-1.)) ;
#93283=DIRECTION('ref_axis',(0.,1.,0.)) ;
#93284=DIRECTION('center_axis',(0.,-1.,0.)) ;
#93285=DIRECTION('ref_axis',(0.,0.,1.)) ;
#93286=DIRECTION('center_axis',(2.16840434497101E-16,-1.,5.10212787052002E-17)) ;
#93287=DIRECTION('ref_axis',(1.,2.16840434497101E-16,-5.47382212626882E-48)) ;
#93288=DIRECTION('center_axis',(0.,1.,0.)) ;
#93289=DIRECTION('ref_axis',(0.,0.,-1.)) ;
#93290=DIRECTION('center_axis',(0.,0.,1.)) ;
#93291=DIRECTION('ref_axis',(1.,0.,0.)) ;
#93292=DIRECTION('center_axis',(0.,0.,-1.)) ;
#93293=DIRECTION('ref_axis',(-1.,0.,0.)) ;
#93294=DIRECTION('center_axis',(-1.,-1.2303003375722E-16,0.)) ;
#93295=DIRECTION('ref_axis',(0.,-1.,0.)) ;
#93296=DIRECTION('center_axis',(0.,-1.,0.)) ;
#93297=DIRECTION('ref_axis',(0.,0.,1.)) ;
#93298=DIRECTION('center_axis',(1.53063836115601E-16,-1.,5.10212787052002E-17)) ;
#93299=DIRECTION('ref_axis',(1.,1.53063836115601E-16,-6.84227765783602E-48)) ;
#93300=DIRECTION('',(-1.53063836115601E-16,1.,-5.10212787052002E-17)) ;
#93301=DIRECTION('center_axis',(0.,-1.,0.)) ;
#93302=DIRECTION('ref_axis',(0.,0.,-1.)) ;
#93303=DIRECTION('center_axis',(-1.,0.,0.)) ;
#93304=DIRECTION('ref_axis',(0.,0.,-1.)) ;
#93305=DIRECTION('center_axis',(-1.2303003375722E-16,1.,-5.10212787052002E-17)) ;
#93306=DIRECTION('ref_axis',(-1.,-1.2303003375722E-16,6.27714964143733E-33)) ;
#93307=DIRECTION('center_axis',(-8.67361737988403E-15,-1.,0.)) ;
#93308=DIRECTION('ref_axis',(1.,-8.67361737988403E-15,0.)) ;
#93309=DIRECTION('center_axis',(1.,0.,6.27714964143733E-33)) ;
#93310=DIRECTION('ref_axis',(6.27714964143733E-33,0.,-1.)) ;
#93311=DIRECTION('center_axis',(-1.,0.,-6.50521303491318E-15)) ;
#93312=DIRECTION('ref_axis',(-6.50521303491318E-15,0.,1.)) ;
#93313=DIRECTION('center_axis',(1.,0.,0.)) ;
#93314=DIRECTION('ref_axis',(0.,1.,0.)) ;
#93315=DIRECTION('center_axis',(0.,0.,-1.)) ;
#93316=DIRECTION('ref_axis',(-1.,0.,0.)) ;
#93317=DIRECTION('center_axis',(0.,0.,1.)) ;
#93318=DIRECTION('ref_axis',(1.,0.,0.)) ;
#93319=DIRECTION('center_axis',(0.,0.,-1.)) ;
#93320=DIRECTION('ref_axis',(-1.,0.,0.)) ;
#93321=DIRECTION('center_axis',(-1.,0.,0.)) ;
#93322=DIRECTION('ref_axis',(0.,0.,1.)) ;
#93323=DIRECTION('center_axis',(0.,-1.,0.)) ;
#93324=DIRECTION('ref_axis',(0.,0.,-1.)) ;
#93325=DIRECTION('center_axis',(0.,1.,0.)) ;
#93326=DIRECTION('ref_axis',(0.,0.,1.)) ;
#93327=DIRECTION('center_axis',(0.,1.,-6.50521303491307E-15)) ;
#93328=DIRECTION('ref_axis',(0.,6.50521303491307E-15,1.)) ;
#93329=DIRECTION('center_axis',(0.,-1.,0.)) ;
#93330=DIRECTION('ref_axis',(0.,0.,-1.)) ;
#93331=DIRECTION('center_axis',(0.,-1.,0.)) ;
#93332=DIRECTION('ref_axis',(0.,0.,-1.)) ;
#93333=DIRECTION('center_axis',(0.,-1.,-1.07081696047951E-16)) ;
#93334=DIRECTION('ref_axis',(0.,1.07081696047951E-16,-1.)) ;
#93335=DIRECTION('center_axis',(0.,1.,0.)) ;
#93336=DIRECTION('ref_axis',(0.,0.,1.)) ;
#93337=DIRECTION('center_axis',(-1.,0.,0.)) ;
#93338=DIRECTION('ref_axis',(0.,0.,1.)) ;
#93339=DIRECTION('center_axis',(0.,0.,1.)) ;
#93340=DIRECTION('ref_axis',(1.,0.,0.)) ;
#93341=DIRECTION('center_axis',(0.,1.,0.)) ;
#93342=DIRECTION('ref_axis',(0.,0.,1.)) ;
#93343=DIRECTION('center_axis',(0.,-1.73472347597681E-14,-1.)) ;
#93344=DIRECTION('ref_axis',(0.,1.,-1.73472347597681E-14)) ;
#93345=DIRECTION('center_axis',(0.,0.,1.)) ;
#93346=DIRECTION('ref_axis',(1.,0.,0.)) ;
#93347=DIRECTION('center_axis',(0.,0.,1.)) ;
#93348=DIRECTION('ref_axis',(1.,0.,0.)) ;
#93349=DIRECTION('center_axis',(0.,0.,1.)) ;
#93350=DIRECTION('ref_axis',(1.,0.,0.)) ;
#93351=DIRECTION('center_axis',(0.,0.,-1.)) ;
#93352=DIRECTION('ref_axis',(-1.,0.,0.)) ;
#93353=DIRECTION('center_axis',(0.,1.,0.)) ;
#93354=DIRECTION('ref_axis',(0.,0.,1.)) ;
#93355=DIRECTION('center_axis',(0.,-0.707106781186545,0.70710678118655)) ;
#93356=DIRECTION('ref_axis',(0.,-0.70710678118655,-0.707106781186545)) ;
#93357=DIRECTION('center_axis',(0.,1.,0.)) ;
#93358=DIRECTION('ref_axis',(0.,0.,1.)) ;
#93359=DIRECTION('center_axis',(0.,-0.514231796959109,-0.857651245551597)) ;
#93360=DIRECTION('ref_axis',(0.,0.857651245551597,-0.514231796959109)) ;
#93361=DIRECTION('center_axis',(0.,-0.707106781186548,0.707106781186547)) ;
#93362=DIRECTION('ref_axis',(0.,-0.707106781186547,-0.707106781186548)) ;
#93363=DIRECTION('center_axis',(0.,-0.707106781186548,0.707106781186548)) ;
#93364=DIRECTION('ref_axis',(0.,-0.707106781186548,-0.707106781186548)) ;
#93365=DIRECTION('center_axis',(-1.,0.,0.)) ;
#93366=DIRECTION('ref_axis',(0.,0.,1.)) ;
#93367=DIRECTION('center_axis',(0.,0.514231796959101,-0.857651245551602)) ;
#93368=DIRECTION('ref_axis',(0.,0.857651245551602,0.514231796959101)) ;
#93369=DIRECTION('center_axis',(0.,1.,0.)) ;
#93370=DIRECTION('ref_axis',(0.,0.,1.)) ;
#93371=DIRECTION('center_axis',(0.,0.,-1.)) ;
#93372=DIRECTION('ref_axis',(-1.,0.,0.)) ;
#93373=DIRECTION('center_axis',(0.,1.,0.)) ;
#93374=DIRECTION('ref_axis',(0.,0.,1.)) ;
#93375=DIRECTION('center_axis',(0.,0.,-1.)) ;
#93376=DIRECTION('ref_axis',(-1.,0.,0.)) ;
#93377=DIRECTION('center_axis',(0.,0.,-1.)) ;
#93378=DIRECTION('ref_axis',(-1.,0.,0.)) ;
#93379=DIRECTION('center_axis',(0.,0.,1.)) ;
#93380=DIRECTION('ref_axis',(1.,0.,0.)) ;
#93381=DIRECTION('center_axis',(0.,0.,-1.)) ;
#93382=DIRECTION('ref_axis',(-1.,0.,0.)) ;
#93383=DIRECTION('center_axis',(0.,1.,0.)) ;
#93384=DIRECTION('ref_axis',(0.,0.,1.)) ;
#93385=DIRECTION('center_axis',(0.,-1.,8.67361737988401E-15)) ;
#93386=DIRECTION('ref_axis',(0.,-8.67361737988401E-15,-1.)) ;
#93387=DIRECTION('center_axis',(0.,0.707106781186546,0.707106781186549)) ;
#93388=DIRECTION('ref_axis',(0.,-0.707106781186549,0.707106781186546)) ;
#93389=DIRECTION('center_axis',(0.,0.707106781186548,0.707106781186548)) ;
#93390=DIRECTION('ref_axis',(0.,-0.707106781186548,0.707106781186548)) ;
#93391=DIRECTION('center_axis',(0.,1.,1.07081696047951E-16)) ;
#93392=DIRECTION('ref_axis',(0.,-1.07081696047951E-16,1.)) ;
#93393=DIRECTION('center_axis',(0.,-1.,0.)) ;
#93394=DIRECTION('ref_axis',(0.,0.,-1.)) ;
#93395=DIRECTION('center_axis',(0.,1.,0.)) ;
#93396=DIRECTION('ref_axis',(0.,0.,1.)) ;
#93397=DIRECTION('center_axis',(0.,-8.67361737988409E-15,1.)) ;
#93398=DIRECTION('ref_axis',(0.,-1.,-8.67361737988409E-15)) ;
#93399=DIRECTION('center_axis',(0.,1.,0.)) ;
#93400=DIRECTION('ref_axis',(0.,0.,1.)) ;
#93401=DIRECTION('center_axis',(0.,8.67361737988403E-15,1.)) ;
#93402=DIRECTION('ref_axis',(0.,-1.,8.67361737988403E-15)) ;
#93403=DIRECTION('center_axis',(0.,3.99416362155027E-15,1.)) ;
#93404=DIRECTION('ref_axis',(0.,-1.,3.99416362155027E-15)) ;
#93405=DIRECTION('center_axis',(0.,0.,1.)) ;
#93406=DIRECTION('ref_axis',(1.,0.,0.)) ;
#93407=DIRECTION('center_axis',(0.,0.,-1.)) ;
#93408=DIRECTION('ref_axis',(-1.,0.,0.)) ;
#93409=DIRECTION('center_axis',(0.,0.,1.)) ;
#93410=DIRECTION('ref_axis',(1.,0.,0.)) ;
#93411=DIRECTION('center_axis',(-1.,0.,0.)) ;
#93412=DIRECTION('ref_axis',(0.,0.,1.)) ;
#93413=DIRECTION('center_axis',(0.,1.,0.)) ;
#93414=DIRECTION('ref_axis',(0.,0.,1.)) ;
#93415=DIRECTION('center_axis',(-1.,0.,0.)) ;
#93416=DIRECTION('ref_axis',(0.,0.,1.)) ;
#93417=DIRECTION('center_axis',(0.,-1.,0.)) ;
#93418=DIRECTION('ref_axis',(0.,0.,-1.)) ;
#93419=DIRECTION('center_axis',(0.,1.,0.)) ;
#93420=DIRECTION('ref_axis',(0.,0.,1.)) ;
#93421=DIRECTION('center_axis',(1.53063836115601E-16,-1.,-1.30104260698261E-16)) ;
#93422=DIRECTION('ref_axis',(1.,1.53063836115601E-16,1.99142572374599E-32)) ;
#93423=DIRECTION('center_axis',(0.,1.,0.)) ;
#93424=DIRECTION('ref_axis',(0.,0.,1.)) ;
#93425=DIRECTION('center_axis',(0.,-1.,0.)) ;
#93426=DIRECTION('ref_axis',(0.,0.,-1.)) ;
#93427=DIRECTION('center_axis',(1.,1.53063836115601E-16,2.73691106313441E-48)) ;
#93428=DIRECTION('ref_axis',(-1.53063836115601E-16,1.,-4.18922106430579E-64)) ;
#93429=DIRECTION('center_axis',(-1.,0.,0.)) ;
#93430=DIRECTION('ref_axis',(0.,0.,1.)) ;
#93431=DIRECTION('center_axis',(1.,1.53063836115601E-16,0.)) ;
#93432=DIRECTION('ref_axis',(1.53063836115601E-16,-1.,0.)) ;
#93433=DIRECTION('center_axis',(0.,1.,0.)) ;
#93434=DIRECTION('ref_axis',(1.,0.,0.)) ;
#93435=DIRECTION('center_axis',(0.,1.,0.)) ;
#93436=DIRECTION('ref_axis',(0.,0.,-1.)) ;
#93437=DIRECTION('center_axis',(0.,0.,1.)) ;
#93438=DIRECTION('ref_axis',(-1.,0.,0.)) ;
#93439=DIRECTION('center_axis',(0.,1.,0.)) ;
#93440=DIRECTION('ref_axis',(1.,0.,0.)) ;
#93441=DIRECTION('center_axis',(0.,0.,1.)) ;
#93442=DIRECTION('ref_axis',(-1.,0.,0.)) ;
#93443=DIRECTION('center_axis',(1.,1.0842021724855E-15,0.)) ;
#93444=DIRECTION('ref_axis',(1.0842021724855E-15,-1.,0.)) ;
#93445=DIRECTION('center_axis',(-1.,-1.53063836115601E-16,0.)) ;
#93446=DIRECTION('ref_axis',(0.,-1.,0.)) ;
#93447=DIRECTION('center_axis',(0.,0.,-1.)) ;
#93448=DIRECTION('ref_axis',(1.,0.,0.)) ;
#93449=DIRECTION('center_axis',(0.,0.,-1.)) ;
#93450=DIRECTION('ref_axis',(0.804034447892625,0.594582716366698,0.)) ;
#93451=DIRECTION('center_axis',(0.,0.,1.)) ;
#93452=DIRECTION('ref_axis',(1.,0.,0.)) ;
#93453=DIRECTION('',(0.,0.,-1.)) ;
#93454=DIRECTION('center_axis',(-2.16840434497101E-16,1.,1.30104260698261E-16)) ;
#93455=DIRECTION('ref_axis',(1.,2.16840434497101E-16,1.22464679914735E-16)) ;
#93456=DIRECTION('',(-2.16840434497101E-16,1.,1.30104260698261E-16)) ;
#93457=DIRECTION('center_axis',(0.,1.,0.)) ;
#93458=DIRECTION('ref_axis',(0.,0.,1.)) ;
#93459=DIRECTION('center_axis',(-1.,-1.53063836115601E-16,-2.73691106313441E-48)) ;
#93460=DIRECTION('ref_axis',(1.53063836115601E-16,-1.,4.18922106430579E-64)) ;
#93461=DIRECTION('center_axis',(1.,2.16840434497101E-16,0.)) ;
#93462=DIRECTION('ref_axis',(2.16840434497101E-16,-1.,0.)) ;
#93463=DIRECTION('center_axis',(0.,0.,1.)) ;
#93464=DIRECTION('ref_axis',(1.,0.,0.)) ;
#93465=DIRECTION('center_axis',(-1.25542992828747E-32,1.020425574104E-16,
1.)) ;
#93466=DIRECTION('ref_axis',(-1.28107280532009E-48,-1.,1.020425574104E-16)) ;
#93467=DIRECTION('center_axis',(0.,0.,1.)) ;
#93468=DIRECTION('ref_axis',(1.,0.,0.)) ;
#93469=DIRECTION('center_axis',(0.,0.,-1.)) ;
#93470=DIRECTION('ref_axis',(-1.,0.,0.)) ;
#93471=DIRECTION('center_axis',(1.,1.53063836115601E-16,-2.73691106313441E-48)) ;
#93472=DIRECTION('ref_axis',(-1.53063836115601E-16,1.,4.18922106430579E-64)) ;
#93473=DIRECTION('center_axis',(-1.,0.,0.)) ;
#93474=DIRECTION('ref_axis',(0.,0.,1.)) ;
#93475=DIRECTION('center_axis',(1.,1.53063836115601E-16,0.)) ;
#93476=DIRECTION('ref_axis',(1.53063836115601E-16,-1.,0.)) ;
#93477=DIRECTION('center_axis',(0.,1.,0.)) ;
#93478=DIRECTION('ref_axis',(1.,0.,0.)) ;
#93479=DIRECTION('center_axis',(-1.,-2.16840434497101E-16,0.)) ;
#93480=DIRECTION('ref_axis',(0.,-1.,0.)) ;
#93481=DIRECTION('center_axis',(0.,0.,-1.)) ;
#93482=DIRECTION('ref_axis',(1.,0.,0.)) ;
#93483=DIRECTION('center_axis',(-1.25542992828747E-32,1.020425574104E-16,
1.)) ;
#93484=DIRECTION('ref_axis',(0.,-1.,0.)) ;
#93485=DIRECTION('center_axis',(0.,-1.,0.)) ;
#93486=DIRECTION('ref_axis',(-6.50521303491307E-15,0.,1.)) ;
#93487=DIRECTION('center_axis',(-1.,0.,0.)) ;
#93488=DIRECTION('ref_axis',(0.,0.,-1.)) ;
#93489=DIRECTION('center_axis',(-1.,-1.53063836115601E-16,0.)) ;
#93490=DIRECTION('ref_axis',(0.,-1.,0.)) ;
#93491=DIRECTION('center_axis',(0.,-1.,0.)) ;
#93492=DIRECTION('ref_axis',(0.,0.,1.)) ;
#93493=DIRECTION('center_axis',(0.,0.,-1.)) ;
#93494=DIRECTION('ref_axis',(-1.,0.,0.)) ;
#93495=DIRECTION('center_axis',(0.,0.,-1.)) ;
#93496=DIRECTION('ref_axis',(-1.,0.,0.)) ;
#93497=DIRECTION('center_axis',(1.,1.53063836115601E-16,-3.06472600140763E-33)) ;
#93498=DIRECTION('ref_axis',(-1.53063836115601E-16,1.,4.69098718418678E-49)) ;
#93499=DIRECTION('center_axis',(-1.,0.,0.)) ;
#93500=DIRECTION('ref_axis',(0.,0.,1.)) ;
#93501=DIRECTION('center_axis',(-1.53063836115601E-16,1.,-1.020425574104E-16)) ;
#93502=DIRECTION('ref_axis',(-1.,-1.53063836115601E-16,1.3684555315672E-47)) ;
#93503=DIRECTION('',(1.53063836115601E-16,-1.,1.020425574104E-16)) ;
#93504=DIRECTION('center_axis',(0.,-1.,0.)) ;
#93505=DIRECTION('ref_axis',(0.,0.,-1.)) ;
#93506=DIRECTION('center_axis',(-1.53063836115601E-16,1.,-1.30104260698261E-16)) ;
#93507=DIRECTION('ref_axis',(-1.,-1.53063836115601E-16,1.99142572374599E-32)) ;
#93508=DIRECTION('center_axis',(0.,-1.,0.)) ;
#93509=DIRECTION('ref_axis',(0.,0.,-1.)) ;
#93510=DIRECTION('center_axis',(-1.,-1.53063836115601E-16,2.73691106313441E-48)) ;
#93511=DIRECTION('ref_axis',(1.53063836115601E-16,-1.,-4.18922106430579E-64)) ;
#93512=DIRECTION('center_axis',(1.,2.16840434497101E-16,0.)) ;
#93513=DIRECTION('ref_axis',(2.16840434497101E-16,-1.,0.)) ;
#93514=DIRECTION('center_axis',(-1.,0.,2.16840434497102E-15)) ;
#93515=DIRECTION('ref_axis',(2.16840434497102E-15,0.,1.)) ;
#93516=DIRECTION('center_axis',(-1.,-2.16840434497101E-16,0.)) ;
#93517=DIRECTION('ref_axis',(0.,-1.,0.)) ;
#93518=DIRECTION('center_axis',(0.,0.,1.)) ;
#93519=DIRECTION('ref_axis',(-1.,0.,0.)) ;
#93520=DIRECTION('center_axis',(0.,1.,0.)) ;
#93521=DIRECTION('ref_axis',(1.,0.,0.)) ;
#93522=DIRECTION('center_axis',(0.,1.,0.)) ;
#93523=DIRECTION('ref_axis',(0.,0.,-1.)) ;
#93524=DIRECTION('center_axis',(1.,0.,0.)) ;
#93525=DIRECTION('ref_axis',(0.,-1.,0.)) ;
#93526=DIRECTION('center_axis',(1.,6.50521303491304E-15,0.)) ;
#93527=DIRECTION('ref_axis',(-6.50521303491304E-15,1.,0.)) ;
#93528=DIRECTION('center_axis',(8.67361737988403E-15,1.,0.)) ;
#93529=DIRECTION('ref_axis',(-1.,8.67361737988403E-15,0.)) ;
#93530=DIRECTION('center_axis',(1.2303003375722E-16,-1.,1.020425574104E-16)) ;
#93531=DIRECTION('ref_axis',(1.,1.2303003375722E-16,-1.25542992828747E-32)) ;
#93532=DIRECTION('center_axis',(0.,1.,0.)) ;
#93533=DIRECTION('ref_axis',(0.,0.,1.)) ;
#93534=DIRECTION('center_axis',(0.,1.,0.)) ;
#93535=DIRECTION('ref_axis',(1.,0.,0.)) ;
#93536=DIRECTION('center_axis',(1.,1.2303003375722E-16,0.)) ;
#93537=DIRECTION('ref_axis',(1.2303003375722E-16,-1.,0.)) ;
#93538=DIRECTION('center_axis',(0.,0.,1.)) ;
#93539=DIRECTION('ref_axis',(-1.,0.,0.)) ;
#93540=DIRECTION('center_axis',(0.,1.,0.)) ;
#93541=DIRECTION('ref_axis',(1.,0.,0.)) ;
#93542=DIRECTION('center_axis',(0.,0.,-1.)) ;
#93543=DIRECTION('ref_axis',(1.,0.,0.)) ;
#93544=DIRECTION('center_axis',(0.,0.,-1.)) ;
#93545=DIRECTION('ref_axis',(-1.,0.,0.)) ;
#93546=DIRECTION('center_axis',(0.,0.,1.)) ;
#93547=DIRECTION('ref_axis',(1.,0.,0.)) ;
#93548=DIRECTION('center_axis',(-2.16840434497101E-16,1.,-1.020425574104E-16)) ;
#93549=DIRECTION('ref_axis',(-1.,-2.16840434497101E-16,5.47382212626882E-48)) ;
#93550=DIRECTION('center_axis',(0.,1.,0.)) ;
#93551=DIRECTION('ref_axis',(0.,0.,-1.)) ;
#93552=DIRECTION('center_axis',(1.,0.,1.25542992828747E-32)) ;
#93553=DIRECTION('ref_axis',(1.25542992828747E-32,0.,-1.)) ;
#93554=DIRECTION('center_axis',(1.,0.,0.)) ;
#93555=DIRECTION('ref_axis',(0.,0.,-1.)) ;
#93556=DIRECTION('center_axis',(-1.,-1.2303003375722E-16,0.)) ;
#93557=DIRECTION('ref_axis',(0.,-1.,0.)) ;
#93558=DIRECTION('center_axis',(0.,0.,-1.)) ;
#93559=DIRECTION('ref_axis',(1.,0.,0.)) ;
#93560=DIRECTION('center_axis',(0.,0.,-1.)) ;
#93561=DIRECTION('ref_axis',(-1.,0.,0.)) ;
#93562=DIRECTION('',(0.,0.,1.)) ;
#93563=DIRECTION('center_axis',(0.,0.,1.)) ;
#93564=DIRECTION('ref_axis',(1.,0.,0.)) ;
#93565=DIRECTION('center_axis',(0.,0.,1.)) ;
#93566=DIRECTION('ref_axis',(1.,0.,0.)) ;
#93567=DIRECTION('center_axis',(6.27714964143733E-33,-5.10212787052002E-17,
-1.)) ;
#93568=DIRECTION('ref_axis',(3.20268201330022E-49,1.,-5.10212787052002E-17)) ;
#93569=DIRECTION('center_axis',(1.,1.53063836115601E-16,-1.53236300070382E-33)) ;
#93570=DIRECTION('ref_axis',(-1.53063836115601E-16,1.,2.34549359209339E-49)) ;
#93571=DIRECTION('center_axis',(-1.,0.,0.)) ;
#93572=DIRECTION('ref_axis',(0.,0.,1.)) ;
#93573=DIRECTION('center_axis',(1.,0.,0.)) ;
#93574=DIRECTION('ref_axis',(0.,0.,-1.)) ;
#93575=DIRECTION('center_axis',(0.,1.,0.)) ;
#93576=DIRECTION('ref_axis',(1.,0.,0.)) ;
#93577=DIRECTION('center_axis',(-4.33680868994202E-15,1.,0.)) ;
#93578=DIRECTION('ref_axis',(1.,4.33680868994202E-15,0.)) ;
#93579=DIRECTION('center_axis',(0.,-1.,0.)) ;
#93580=DIRECTION('ref_axis',(0.,0.,-1.)) ;
#93581=DIRECTION('center_axis',(0.,0.,-1.)) ;
#93582=DIRECTION('ref_axis',(1.,0.,0.)) ;
#93583=DIRECTION('center_axis',(0.,0.,1.)) ;
#93584=DIRECTION('ref_axis',(1.,0.,0.)) ;
#93585=DIRECTION('center_axis',(0.,0.,-1.)) ;
#93586=DIRECTION('ref_axis',(-1.,0.,0.)) ;
#93587=DIRECTION('center_axis',(0.,1.,0.)) ;
#93588=DIRECTION('ref_axis',(1.,0.,0.)) ;
#93589=DIRECTION('center_axis',(1.,1.2303003375722E-16,0.)) ;
#93590=DIRECTION('ref_axis',(1.2303003375722E-16,-1.,0.)) ;
#93591=DIRECTION('center_axis',(0.,1.,0.)) ;
#93592=DIRECTION('ref_axis',(-6.50521303491307E-15,0.,-1.)) ;
#93593=DIRECTION('center_axis',(6.27714964143733E-33,-5.10212787052002E-17,
-1.)) ;
#93594=DIRECTION('ref_axis',(0.,1.,0.)) ;
#93595=DIRECTION('center_axis',(0.,-1.,0.)) ;
#93596=DIRECTION('ref_axis',(0.,0.,1.)) ;
#93597=DIRECTION('center_axis',(2.16840434497101E-16,-1.,5.10212787052002E-17)) ;
#93598=DIRECTION('ref_axis',(1.,2.16840434497101E-16,-5.47382212626882E-48)) ;
#93599=DIRECTION('center_axis',(0.,1.,0.)) ;
#93600=DIRECTION('ref_axis',(0.,0.,-1.)) ;
#93601=DIRECTION('center_axis',(0.,0.,1.)) ;
#93602=DIRECTION('ref_axis',(1.,0.,0.)) ;
#93603=DIRECTION('center_axis',(0.,0.,-1.)) ;
#93604=DIRECTION('ref_axis',(-1.,0.,0.)) ;
#93605=DIRECTION('center_axis',(-1.,-1.2303003375722E-16,0.)) ;
#93606=DIRECTION('ref_axis',(0.,-1.,0.)) ;
#93607=DIRECTION('center_axis',(0.,-1.,0.)) ;
#93608=DIRECTION('ref_axis',(0.,0.,1.)) ;
#93609=DIRECTION('center_axis',(1.53063836115601E-16,-1.,5.10212787052002E-17)) ;
#93610=DIRECTION('ref_axis',(1.,1.53063836115601E-16,-6.84227765783602E-48)) ;
#93611=DIRECTION('',(-1.53063836115601E-16,1.,-5.10212787052002E-17)) ;
#93612=DIRECTION('center_axis',(0.,-1.,0.)) ;
#93613=DIRECTION('ref_axis',(0.,0.,-1.)) ;
#93614=DIRECTION('center_axis',(-1.,0.,0.)) ;
#93615=DIRECTION('ref_axis',(0.,0.,-1.)) ;
#93616=DIRECTION('center_axis',(-1.2303003375722E-16,1.,-5.10212787052002E-17)) ;
#93617=DIRECTION('ref_axis',(-1.,-1.2303003375722E-16,6.27714964143733E-33)) ;
#93618=DIRECTION('center_axis',(-8.67361737988403E-15,-1.,0.)) ;
#93619=DIRECTION('ref_axis',(1.,-8.67361737988403E-15,0.)) ;
#93620=DIRECTION('center_axis',(1.,0.,6.27714964143733E-33)) ;
#93621=DIRECTION('ref_axis',(6.27714964143733E-33,0.,-1.)) ;
#93622=DIRECTION('center_axis',(-1.,0.,-6.50521303491307E-15)) ;
#93623=DIRECTION('ref_axis',(-6.50521303491307E-15,0.,1.)) ;
#93624=DIRECTION('center_axis',(1.,0.,0.)) ;
#93625=DIRECTION('ref_axis',(0.,1.,0.)) ;
#93626=DIRECTION('center_axis',(0.,0.,-1.)) ;
#93627=DIRECTION('ref_axis',(-1.,0.,0.)) ;
#93628=DIRECTION('center_axis',(0.,0.,1.)) ;
#93629=DIRECTION('ref_axis',(1.,0.,0.)) ;
#93630=DIRECTION('center_axis',(0.,0.,-1.)) ;
#93631=DIRECTION('ref_axis',(-1.,0.,0.)) ;
#93632=DIRECTION('center_axis',(-1.,0.,0.)) ;
#93633=DIRECTION('ref_axis',(0.,0.,1.)) ;
#93634=DIRECTION('center_axis',(0.,-1.,0.)) ;
#93635=DIRECTION('ref_axis',(0.,0.,-1.)) ;
#93636=DIRECTION('center_axis',(0.,1.,0.)) ;
#93637=DIRECTION('ref_axis',(0.,0.,1.)) ;
#93638=DIRECTION('center_axis',(0.,1.,-6.50521303491307E-15)) ;
#93639=DIRECTION('ref_axis',(0.,6.50521303491307E-15,1.)) ;
#93640=DIRECTION('center_axis',(0.,-1.,0.)) ;
#93641=DIRECTION('ref_axis',(0.,0.,-1.)) ;
#93642=DIRECTION('center_axis',(0.,-1.,0.)) ;
#93643=DIRECTION('ref_axis',(0.,0.,-1.)) ;
#93644=DIRECTION('center_axis',(0.,-1.,-1.07081696047951E-16)) ;
#93645=DIRECTION('ref_axis',(0.,1.07081696047951E-16,-1.)) ;
#93646=DIRECTION('center_axis',(0.,1.,0.)) ;
#93647=DIRECTION('ref_axis',(0.,0.,1.)) ;
#93648=DIRECTION('center_axis',(-1.,0.,0.)) ;
#93649=DIRECTION('ref_axis',(0.,0.,1.)) ;
#93650=DIRECTION('center_axis',(0.,0.,1.)) ;
#93651=DIRECTION('ref_axis',(1.,0.,0.)) ;
#93652=DIRECTION('center_axis',(0.,1.,0.)) ;
#93653=DIRECTION('ref_axis',(0.,0.,1.)) ;
#93654=DIRECTION('center_axis',(0.,-1.73472347597681E-14,-1.)) ;
#93655=DIRECTION('ref_axis',(0.,1.,-1.73472347597681E-14)) ;
#93656=DIRECTION('center_axis',(0.,0.,1.)) ;
#93657=DIRECTION('ref_axis',(1.,0.,0.)) ;
#93658=DIRECTION('center_axis',(0.,0.,1.)) ;
#93659=DIRECTION('ref_axis',(1.,0.,0.)) ;
#93660=DIRECTION('center_axis',(0.,0.,1.)) ;
#93661=DIRECTION('ref_axis',(1.,0.,0.)) ;
#93662=DIRECTION('center_axis',(0.,0.,-1.)) ;
#93663=DIRECTION('ref_axis',(-1.,0.,0.)) ;
#93664=DIRECTION('center_axis',(0.,1.,0.)) ;
#93665=DIRECTION('ref_axis',(0.,0.,1.)) ;
#93666=DIRECTION('center_axis',(0.,-0.707106781186545,0.70710678118655)) ;
#93667=DIRECTION('ref_axis',(0.,-0.70710678118655,-0.707106781186545)) ;
#93668=DIRECTION('center_axis',(0.,1.,0.)) ;
#93669=DIRECTION('ref_axis',(0.,0.,1.)) ;
#93670=DIRECTION('center_axis',(0.,-0.514231796959109,-0.857651245551597)) ;
#93671=DIRECTION('ref_axis',(0.,0.857651245551597,-0.514231796959109)) ;
#93672=DIRECTION('center_axis',(0.,-0.707106781186548,0.707106781186547)) ;
#93673=DIRECTION('ref_axis',(0.,-0.707106781186547,-0.707106781186548)) ;
#93674=DIRECTION('center_axis',(0.,-0.707106781186548,0.707106781186548)) ;
#93675=DIRECTION('ref_axis',(0.,-0.707106781186548,-0.707106781186548)) ;
#93676=DIRECTION('center_axis',(-1.,0.,0.)) ;
#93677=DIRECTION('ref_axis',(0.,0.,1.)) ;
#93678=DIRECTION('center_axis',(-2.23012492569676E-15,0.514231796959107,
-0.857651245551598)) ;
#93679=DIRECTION('ref_axis',(-5.69910941180089E-30,0.857651245551598,0.514231796959107)) ;
#93680=DIRECTION('center_axis',(0.,1.,0.)) ;
#93681=DIRECTION('ref_axis',(0.,0.,1.)) ;
#93682=DIRECTION('center_axis',(0.,0.,-1.)) ;
#93683=DIRECTION('ref_axis',(-1.,0.,0.)) ;
#93684=DIRECTION('center_axis',(0.,1.,0.)) ;
#93685=DIRECTION('ref_axis',(0.,0.,1.)) ;
#93686=DIRECTION('center_axis',(0.,0.,-1.)) ;
#93687=DIRECTION('ref_axis',(-1.,0.,0.)) ;
#93688=DIRECTION('center_axis',(0.,0.,-1.)) ;
#93689=DIRECTION('ref_axis',(-1.,0.,0.)) ;
#93690=DIRECTION('center_axis',(0.,0.,1.)) ;
#93691=DIRECTION('ref_axis',(1.,0.,0.)) ;
#93692=DIRECTION('center_axis',(0.,0.,-1.)) ;
#93693=DIRECTION('ref_axis',(-1.,0.,0.)) ;
#93694=DIRECTION('center_axis',(0.,1.,0.)) ;
#93695=DIRECTION('ref_axis',(0.,0.,1.)) ;
#93696=DIRECTION('center_axis',(0.,-1.,8.67361737988409E-15)) ;
#93697=DIRECTION('ref_axis',(0.,-8.67361737988409E-15,-1.)) ;
#93698=DIRECTION('center_axis',(0.,0.707106781186546,0.707106781186549)) ;
#93699=DIRECTION('ref_axis',(0.,-0.707106781186549,0.707106781186546)) ;
#93700=DIRECTION('center_axis',(0.,0.707106781186541,0.707106781186554)) ;
#93701=DIRECTION('ref_axis',(0.,-0.707106781186554,0.707106781186541)) ;
#93702=DIRECTION('center_axis',(0.,1.,1.07081696047951E-16)) ;
#93703=DIRECTION('ref_axis',(0.,-1.07081696047951E-16,1.)) ;
#93704=DIRECTION('center_axis',(0.,-1.,0.)) ;
#93705=DIRECTION('ref_axis',(0.,0.,-1.)) ;
#93706=DIRECTION('center_axis',(0.,1.,0.)) ;
#93707=DIRECTION('ref_axis',(0.,0.,1.)) ;
#93708=DIRECTION('center_axis',(0.,0.,1.)) ;
#93709=DIRECTION('ref_axis',(1.,0.,0.)) ;
#93710=DIRECTION('center_axis',(0.,1.,0.)) ;
#93711=DIRECTION('ref_axis',(0.,0.,1.)) ;
#93712=DIRECTION('center_axis',(0.,0.,1.)) ;
#93713=DIRECTION('ref_axis',(1.,0.,0.)) ;
#93714=DIRECTION('center_axis',(0.,3.99416362155027E-15,1.)) ;
#93715=DIRECTION('ref_axis',(0.,-1.,3.99416362155027E-15)) ;
#93716=DIRECTION('center_axis',(0.,0.,1.)) ;
#93717=DIRECTION('ref_axis',(1.,0.,0.)) ;
#93718=DIRECTION('center_axis',(0.,0.,-1.)) ;
#93719=DIRECTION('ref_axis',(-1.,0.,0.)) ;
#93720=DIRECTION('center_axis',(0.,0.,1.)) ;
#93721=DIRECTION('ref_axis',(1.,0.,0.)) ;
#93722=DIRECTION('center_axis',(-1.,0.,0.)) ;
#93723=DIRECTION('ref_axis',(0.,0.,1.)) ;
#93724=DIRECTION('center_axis',(0.,1.,0.)) ;
#93725=DIRECTION('ref_axis',(0.,0.,1.)) ;
#93726=DIRECTION('center_axis',(-1.,0.,0.)) ;
#93727=DIRECTION('ref_axis',(0.,0.,1.)) ;
#93728=DIRECTION('center_axis',(0.,-1.,0.)) ;
#93729=DIRECTION('ref_axis',(0.,0.,-1.)) ;
#93730=DIRECTION('center_axis',(0.,1.,0.)) ;
#93731=DIRECTION('ref_axis',(0.,0.,1.)) ;
#93732=DIRECTION('center_axis',(1.53063836115601E-16,-1.,-1.30104260698261E-16)) ;
#93733=DIRECTION('ref_axis',(1.,1.53063836115601E-16,1.99142572374599E-32)) ;
#93734=DIRECTION('center_axis',(0.,1.,0.)) ;
#93735=DIRECTION('ref_axis',(0.,0.,1.)) ;
#93736=DIRECTION('center_axis',(0.,-1.,0.)) ;
#93737=DIRECTION('ref_axis',(0.,0.,-1.)) ;
#93738=DIRECTION('center_axis',(1.,1.53063836115601E-16,2.73691106313441E-48)) ;
#93739=DIRECTION('ref_axis',(-1.53063836115601E-16,1.,-4.18922106430579E-64)) ;
#93740=DIRECTION('center_axis',(-1.,0.,0.)) ;
#93741=DIRECTION('ref_axis',(0.,0.,1.)) ;
#93742=DIRECTION('center_axis',(1.,1.53063836115601E-16,0.)) ;
#93743=DIRECTION('ref_axis',(1.53063836115601E-16,-1.,0.)) ;
#93744=DIRECTION('center_axis',(0.,1.,0.)) ;
#93745=DIRECTION('ref_axis',(1.,0.,0.)) ;
#93746=DIRECTION('center_axis',(0.,1.,0.)) ;
#93747=DIRECTION('ref_axis',(0.,0.,-1.)) ;
#93748=DIRECTION('center_axis',(0.,0.,1.)) ;
#93749=DIRECTION('ref_axis',(-1.,0.,0.)) ;
#93750=DIRECTION('center_axis',(0.,1.,0.)) ;
#93751=DIRECTION('ref_axis',(1.,0.,0.)) ;
#93752=DIRECTION('center_axis',(0.,0.,1.)) ;
#93753=DIRECTION('ref_axis',(-1.,0.,0.)) ;
#93754=DIRECTION('center_axis',(1.,1.0842021724855E-15,0.)) ;
#93755=DIRECTION('ref_axis',(1.0842021724855E-15,-1.,0.)) ;
#93756=DIRECTION('center_axis',(-1.,-1.53063836115601E-16,0.)) ;
#93757=DIRECTION('ref_axis',(0.,-1.,0.)) ;
#93758=DIRECTION('center_axis',(0.,0.,-1.)) ;
#93759=DIRECTION('ref_axis',(1.,0.,0.)) ;
#93760=DIRECTION('center_axis',(0.,0.,-1.)) ;
#93761=DIRECTION('ref_axis',(0.804034447892618,0.594582716366708,0.)) ;
#93762=DIRECTION('center_axis',(0.,0.,1.)) ;
#93763=DIRECTION('ref_axis',(1.,0.,0.)) ;
#93764=DIRECTION('',(0.,0.,-1.)) ;
#93765=DIRECTION('center_axis',(-2.16840434497101E-16,1.,1.30104260698261E-16)) ;
#93766=DIRECTION('ref_axis',(1.,2.16840434497101E-16,1.22464679914735E-16)) ;
#93767=DIRECTION('',(-2.16840434497101E-16,1.,1.30104260698261E-16)) ;
#93768=DIRECTION('center_axis',(0.,1.,0.)) ;
#93769=DIRECTION('ref_axis',(0.,0.,1.)) ;
#93770=DIRECTION('center_axis',(-1.,-1.53063836115601E-16,-2.73691106313441E-48)) ;
#93771=DIRECTION('ref_axis',(1.53063836115601E-16,-1.,4.18922106430579E-64)) ;
#93772=DIRECTION('center_axis',(1.,2.16840434497101E-16,0.)) ;
#93773=DIRECTION('ref_axis',(2.16840434497101E-16,-1.,0.)) ;
#93774=DIRECTION('center_axis',(0.,0.,1.)) ;
#93775=DIRECTION('ref_axis',(1.,0.,0.)) ;
#93776=DIRECTION('center_axis',(-1.25542992828747E-32,1.020425574104E-16,
1.)) ;
#93777=DIRECTION('ref_axis',(-1.28107280532009E-48,-1.,1.020425574104E-16)) ;
#93778=DIRECTION('center_axis',(0.,0.,1.)) ;
#93779=DIRECTION('ref_axis',(1.,0.,0.)) ;
#93780=DIRECTION('center_axis',(0.,0.,-1.)) ;
#93781=DIRECTION('ref_axis',(-1.,0.,0.)) ;
#93782=DIRECTION('center_axis',(1.,1.53063836115601E-16,-2.73691106313441E-48)) ;
#93783=DIRECTION('ref_axis',(-1.53063836115601E-16,1.,4.18922106430579E-64)) ;
#93784=DIRECTION('center_axis',(-1.,0.,0.)) ;
#93785=DIRECTION('ref_axis',(0.,0.,1.)) ;
#93786=DIRECTION('center_axis',(1.,1.53063836115601E-16,0.)) ;
#93787=DIRECTION('ref_axis',(1.53063836115601E-16,-1.,0.)) ;
#93788=DIRECTION('center_axis',(0.,1.,0.)) ;
#93789=DIRECTION('ref_axis',(1.,0.,0.)) ;
#93790=DIRECTION('center_axis',(-1.,-2.16840434497101E-16,0.)) ;
#93791=DIRECTION('ref_axis',(0.,-1.,0.)) ;
#93792=DIRECTION('center_axis',(0.,0.,-1.)) ;
#93793=DIRECTION('ref_axis',(1.,0.,0.)) ;
#93794=DIRECTION('center_axis',(-1.25542992828747E-32,1.020425574104E-16,
1.)) ;
#93795=DIRECTION('ref_axis',(0.,-1.,0.)) ;
#93796=DIRECTION('center_axis',(0.,-1.,0.)) ;
#93797=DIRECTION('ref_axis',(-6.50521303491307E-15,0.,1.)) ;
#93798=DIRECTION('center_axis',(-1.,0.,0.)) ;
#93799=DIRECTION('ref_axis',(0.,0.,-1.)) ;
#93800=DIRECTION('center_axis',(-1.,-1.53063836115601E-16,0.)) ;
#93801=DIRECTION('ref_axis',(0.,-1.,0.)) ;
#93802=DIRECTION('center_axis',(0.,-1.,0.)) ;
#93803=DIRECTION('ref_axis',(0.,0.,1.)) ;
#93804=DIRECTION('center_axis',(0.,0.,-1.)) ;
#93805=DIRECTION('ref_axis',(-1.,0.,0.)) ;
#93806=DIRECTION('center_axis',(0.,0.,-1.)) ;
#93807=DIRECTION('ref_axis',(-1.,0.,0.)) ;
#93808=DIRECTION('center_axis',(1.,1.53063836115601E-16,-3.06472600140763E-33)) ;
#93809=DIRECTION('ref_axis',(-1.53063836115601E-16,1.,4.69098718418678E-49)) ;
#93810=DIRECTION('center_axis',(-1.,0.,0.)) ;
#93811=DIRECTION('ref_axis',(0.,0.,1.)) ;
#93812=DIRECTION('center_axis',(-1.53063836115601E-16,1.,-1.020425574104E-16)) ;
#93813=DIRECTION('ref_axis',(-1.,-1.53063836115601E-16,1.3684555315672E-47)) ;
#93814=DIRECTION('',(1.53063836115601E-16,-1.,1.020425574104E-16)) ;
#93815=DIRECTION('center_axis',(0.,-1.,0.)) ;
#93816=DIRECTION('ref_axis',(0.,0.,-1.)) ;
#93817=DIRECTION('center_axis',(-1.53063836115601E-16,1.,-1.30104260698261E-16)) ;
#93818=DIRECTION('ref_axis',(-1.,-1.53063836115601E-16,1.99142572374599E-32)) ;
#93819=DIRECTION('center_axis',(0.,-1.,0.)) ;
#93820=DIRECTION('ref_axis',(0.,0.,-1.)) ;
#93821=DIRECTION('center_axis',(-1.,-1.53063836115601E-16,2.73691106313441E-48)) ;
#93822=DIRECTION('ref_axis',(1.53063836115601E-16,-1.,-4.18922106430579E-64)) ;
#93823=DIRECTION('center_axis',(1.,2.16840434497101E-16,0.)) ;
#93824=DIRECTION('ref_axis',(2.16840434497101E-16,-1.,0.)) ;
#93825=DIRECTION('center_axis',(-1.,0.,2.16840434497102E-15)) ;
#93826=DIRECTION('ref_axis',(2.16840434497102E-15,0.,1.)) ;
#93827=DIRECTION('center_axis',(-1.,-2.16840434497101E-16,0.)) ;
#93828=DIRECTION('ref_axis',(0.,-1.,0.)) ;
#93829=DIRECTION('center_axis',(0.,0.,1.)) ;
#93830=DIRECTION('ref_axis',(-1.,0.,0.)) ;
#93831=DIRECTION('center_axis',(0.,1.,0.)) ;
#93832=DIRECTION('ref_axis',(1.,0.,0.)) ;
#93833=DIRECTION('center_axis',(0.,1.,0.)) ;
#93834=DIRECTION('ref_axis',(0.,0.,-1.)) ;
#93835=DIRECTION('center_axis',(1.,0.,0.)) ;
#93836=DIRECTION('ref_axis',(0.,-1.,0.)) ;
#93837=DIRECTION('center_axis',(1.,6.50521303491304E-15,0.)) ;
#93838=DIRECTION('ref_axis',(-6.50521303491304E-15,1.,0.)) ;
#93839=DIRECTION('center_axis',(8.67361737988403E-15,1.,0.)) ;
#93840=DIRECTION('ref_axis',(-1.,8.67361737988403E-15,0.)) ;
#93841=DIRECTION('center_axis',(1.2303003375722E-16,-1.,1.020425574104E-16)) ;
#93842=DIRECTION('ref_axis',(1.,1.2303003375722E-16,-1.25542992828747E-32)) ;
#93843=DIRECTION('center_axis',(0.,1.,0.)) ;
#93844=DIRECTION('ref_axis',(0.,0.,1.)) ;
#93845=DIRECTION('center_axis',(0.,1.,0.)) ;
#93846=DIRECTION('ref_axis',(1.,0.,0.)) ;
#93847=DIRECTION('center_axis',(1.,1.2303003375722E-16,0.)) ;
#93848=DIRECTION('ref_axis',(1.2303003375722E-16,-1.,0.)) ;
#93849=DIRECTION('center_axis',(0.,0.,1.)) ;
#93850=DIRECTION('ref_axis',(-1.,0.,0.)) ;
#93851=DIRECTION('center_axis',(0.,1.,0.)) ;
#93852=DIRECTION('ref_axis',(1.,0.,0.)) ;
#93853=DIRECTION('center_axis',(0.,0.,-1.)) ;
#93854=DIRECTION('ref_axis',(1.,0.,0.)) ;
#93855=DIRECTION('center_axis',(0.,0.,-1.)) ;
#93856=DIRECTION('ref_axis',(-1.,0.,0.)) ;
#93857=DIRECTION('center_axis',(0.,0.,1.)) ;
#93858=DIRECTION('ref_axis',(1.,0.,0.)) ;
#93859=DIRECTION('center_axis',(-2.16840434497101E-16,1.,-1.020425574104E-16)) ;
#93860=DIRECTION('ref_axis',(-1.,-2.16840434497101E-16,5.47382212626882E-48)) ;
#93861=DIRECTION('center_axis',(0.,1.,0.)) ;
#93862=DIRECTION('ref_axis',(0.,0.,-1.)) ;
#93863=DIRECTION('center_axis',(1.,0.,1.25542992828747E-32)) ;
#93864=DIRECTION('ref_axis',(1.25542992828747E-32,0.,-1.)) ;
#93865=DIRECTION('center_axis',(1.,0.,0.)) ;
#93866=DIRECTION('ref_axis',(0.,0.,-1.)) ;
#93867=DIRECTION('center_axis',(-1.,-1.2303003375722E-16,0.)) ;
#93868=DIRECTION('ref_axis',(0.,-1.,0.)) ;
#93869=DIRECTION('center_axis',(0.,0.,-1.)) ;
#93870=DIRECTION('ref_axis',(1.,0.,0.)) ;
#93871=DIRECTION('center_axis',(0.,0.,-1.)) ;
#93872=DIRECTION('ref_axis',(-1.,0.,0.)) ;
#93873=DIRECTION('',(0.,0.,1.)) ;
#93874=DIRECTION('center_axis',(0.,0.,1.)) ;
#93875=DIRECTION('ref_axis',(1.,0.,0.)) ;
#93876=DIRECTION('center_axis',(0.,0.,1.)) ;
#93877=DIRECTION('ref_axis',(1.,0.,0.)) ;
#93878=DIRECTION('center_axis',(6.27714964143733E-33,-5.10212787052002E-17,
-1.)) ;
#93879=DIRECTION('ref_axis',(3.20268201330022E-49,1.,-5.10212787052002E-17)) ;
#93880=DIRECTION('center_axis',(1.,1.53063836115601E-16,-1.53236300070382E-33)) ;
#93881=DIRECTION('ref_axis',(-1.53063836115601E-16,1.,2.34549359209339E-49)) ;
#93882=DIRECTION('center_axis',(-1.,0.,0.)) ;
#93883=DIRECTION('ref_axis',(0.,0.,1.)) ;
#93884=DIRECTION('center_axis',(1.,0.,0.)) ;
#93885=DIRECTION('ref_axis',(0.,0.,-1.)) ;
#93886=DIRECTION('center_axis',(0.,1.,0.)) ;
#93887=DIRECTION('ref_axis',(1.,0.,0.)) ;
#93888=DIRECTION('center_axis',(-4.33680868994202E-15,1.,0.)) ;
#93889=DIRECTION('ref_axis',(1.,4.33680868994202E-15,0.)) ;
#93890=DIRECTION('center_axis',(0.,-1.,0.)) ;
#93891=DIRECTION('ref_axis',(0.,0.,-1.)) ;
#93892=DIRECTION('center_axis',(0.,0.,-1.)) ;
#93893=DIRECTION('ref_axis',(1.,0.,0.)) ;
#93894=DIRECTION('center_axis',(0.,0.,1.)) ;
#93895=DIRECTION('ref_axis',(1.,0.,0.)) ;
#93896=DIRECTION('center_axis',(0.,0.,-1.)) ;
#93897=DIRECTION('ref_axis',(-1.,0.,0.)) ;
#93898=DIRECTION('center_axis',(0.,1.,0.)) ;
#93899=DIRECTION('ref_axis',(1.,0.,0.)) ;
#93900=DIRECTION('center_axis',(1.,1.2303003375722E-16,0.)) ;
#93901=DIRECTION('ref_axis',(1.2303003375722E-16,-1.,0.)) ;
#93902=DIRECTION('center_axis',(0.,1.,0.)) ;
#93903=DIRECTION('ref_axis',(-6.50521303491307E-15,0.,-1.)) ;
#93904=DIRECTION('center_axis',(6.27714964143733E-33,-5.10212787052002E-17,
-1.)) ;
#93905=DIRECTION('ref_axis',(0.,1.,0.)) ;
#93906=DIRECTION('center_axis',(0.,-1.,0.)) ;
#93907=DIRECTION('ref_axis',(0.,0.,1.)) ;
#93908=DIRECTION('center_axis',(2.16840434497101E-16,-1.,5.10212787052002E-17)) ;
#93909=DIRECTION('ref_axis',(1.,2.16840434497101E-16,-5.47382212626882E-48)) ;
#93910=DIRECTION('center_axis',(0.,1.,0.)) ;
#93911=DIRECTION('ref_axis',(0.,0.,-1.)) ;
#93912=DIRECTION('center_axis',(0.,0.,1.)) ;
#93913=DIRECTION('ref_axis',(1.,0.,0.)) ;
#93914=DIRECTION('center_axis',(0.,0.,-1.)) ;
#93915=DIRECTION('ref_axis',(-1.,0.,0.)) ;
#93916=DIRECTION('center_axis',(-1.,-1.2303003375722E-16,0.)) ;
#93917=DIRECTION('ref_axis',(0.,-1.,0.)) ;
#93918=DIRECTION('center_axis',(0.,-1.,0.)) ;
#93919=DIRECTION('ref_axis',(0.,0.,1.)) ;
#93920=DIRECTION('center_axis',(1.53063836115601E-16,-1.,5.10212787052002E-17)) ;
#93921=DIRECTION('ref_axis',(1.,1.53063836115601E-16,-6.84227765783602E-48)) ;
#93922=DIRECTION('',(-1.53063836115601E-16,1.,-5.10212787052002E-17)) ;
#93923=DIRECTION('center_axis',(0.,-1.,0.)) ;
#93924=DIRECTION('ref_axis',(0.,0.,-1.)) ;
#93925=DIRECTION('center_axis',(-1.,0.,0.)) ;
#93926=DIRECTION('ref_axis',(0.,0.,-1.)) ;
#93927=DIRECTION('center_axis',(-1.2303003375722E-16,1.,-5.10212787052002E-17)) ;
#93928=DIRECTION('ref_axis',(-1.,-1.2303003375722E-16,6.27714964143733E-33)) ;
#93929=DIRECTION('center_axis',(-8.67361737988403E-15,-1.,0.)) ;
#93930=DIRECTION('ref_axis',(1.,-8.67361737988403E-15,0.)) ;
#93931=DIRECTION('center_axis',(1.,0.,6.27714964143733E-33)) ;
#93932=DIRECTION('ref_axis',(6.27714964143733E-33,0.,-1.)) ;
#93933=DIRECTION('center_axis',(-1.,0.,-6.50521303491307E-15)) ;
#93934=DIRECTION('ref_axis',(-6.50521303491307E-15,0.,1.)) ;
#93935=DIRECTION('center_axis',(1.,0.,0.)) ;
#93936=DIRECTION('ref_axis',(0.,1.,0.)) ;
#93937=DIRECTION('center_axis',(0.,0.,-1.)) ;
#93938=DIRECTION('ref_axis',(-1.,0.,0.)) ;
#93939=DIRECTION('center_axis',(0.,0.,1.)) ;
#93940=DIRECTION('ref_axis',(1.,0.,0.)) ;
#93941=DIRECTION('center_axis',(0.,0.,-1.)) ;
#93942=DIRECTION('ref_axis',(-1.,0.,0.)) ;
#93943=DIRECTION('center_axis',(-1.,0.,0.)) ;
#93944=DIRECTION('ref_axis',(0.,0.,1.)) ;
#93945=DIRECTION('center_axis',(0.,-1.,0.)) ;
#93946=DIRECTION('ref_axis',(0.,0.,-1.)) ;
#93947=DIRECTION('center_axis',(0.,1.,0.)) ;
#93948=DIRECTION('ref_axis',(0.,0.,1.)) ;
#93949=DIRECTION('center_axis',(0.,1.,-6.50521303491307E-15)) ;
#93950=DIRECTION('ref_axis',(0.,6.50521303491307E-15,1.)) ;
#93951=DIRECTION('center_axis',(0.,-1.,0.)) ;
#93952=DIRECTION('ref_axis',(0.,0.,-1.)) ;
#93953=DIRECTION('center_axis',(0.,-1.,0.)) ;
#93954=DIRECTION('ref_axis',(0.,0.,-1.)) ;
#93955=DIRECTION('center_axis',(0.,-1.,-1.07081696047951E-16)) ;
#93956=DIRECTION('ref_axis',(0.,1.07081696047951E-16,-1.)) ;
#93957=DIRECTION('center_axis',(0.,1.,0.)) ;
#93958=DIRECTION('ref_axis',(0.,0.,1.)) ;
#93959=DIRECTION('center_axis',(-1.,0.,0.)) ;
#93960=DIRECTION('ref_axis',(0.,0.,1.)) ;
#93961=DIRECTION('center_axis',(0.,0.,1.)) ;
#93962=DIRECTION('ref_axis',(1.,0.,0.)) ;
#93963=DIRECTION('center_axis',(0.,1.,0.)) ;
#93964=DIRECTION('ref_axis',(0.,0.,1.)) ;
#93965=DIRECTION('center_axis',(0.,0.,-1.)) ;
#93966=DIRECTION('ref_axis',(-1.,0.,0.)) ;
#93967=DIRECTION('center_axis',(0.,0.,1.)) ;
#93968=DIRECTION('ref_axis',(1.,0.,0.)) ;
#93969=DIRECTION('center_axis',(0.,0.,1.)) ;
#93970=DIRECTION('ref_axis',(1.,0.,0.)) ;
#93971=DIRECTION('center_axis',(0.,0.,1.)) ;
#93972=DIRECTION('ref_axis',(1.,0.,0.)) ;
#93973=DIRECTION('center_axis',(0.,0.,-1.)) ;
#93974=DIRECTION('ref_axis',(-1.,0.,0.)) ;
#93975=DIRECTION('center_axis',(0.,1.,0.)) ;
#93976=DIRECTION('ref_axis',(0.,0.,1.)) ;
#93977=DIRECTION('center_axis',(0.,-0.707106781186558,0.707106781186537)) ;
#93978=DIRECTION('ref_axis',(0.,-0.707106781186537,-0.707106781186558)) ;
#93979=DIRECTION('center_axis',(0.,1.,0.)) ;
#93980=DIRECTION('ref_axis',(0.,0.,1.)) ;
#93981=DIRECTION('center_axis',(0.,-0.514231796959093,-0.857651245551607)) ;
#93982=DIRECTION('ref_axis',(0.,0.857651245551607,-0.514231796959093)) ;
#93983=DIRECTION('center_axis',(0.,-0.707106781186548,0.707106781186547)) ;
#93984=DIRECTION('ref_axis',(0.,-0.707106781186547,-0.707106781186548)) ;
#93985=DIRECTION('center_axis',(0.,-0.70710678118655,0.707106781186545)) ;
#93986=DIRECTION('ref_axis',(0.,-0.707106781186545,-0.70710678118655)) ;
#93987=DIRECTION('center_axis',(-1.,0.,0.)) ;
#93988=DIRECTION('ref_axis',(0.,0.,1.)) ;
#93989=DIRECTION('center_axis',(-2.23012492569676E-15,0.514231796959107,
-0.857651245551598)) ;
#93990=DIRECTION('ref_axis',(-5.69910941180089E-30,0.857651245551598,0.514231796959107)) ;
#93991=DIRECTION('center_axis',(0.,1.,0.)) ;
#93992=DIRECTION('ref_axis',(0.,0.,1.)) ;
#93993=DIRECTION('center_axis',(0.,0.,-1.)) ;
#93994=DIRECTION('ref_axis',(-1.,0.,0.)) ;
#93995=DIRECTION('center_axis',(0.,1.,0.)) ;
#93996=DIRECTION('ref_axis',(0.,0.,1.)) ;
#93997=DIRECTION('center_axis',(0.,0.,-1.)) ;
#93998=DIRECTION('ref_axis',(-1.,0.,0.)) ;
#93999=DIRECTION('center_axis',(0.,0.,-1.)) ;
#94000=DIRECTION('ref_axis',(-1.,0.,0.)) ;
#94001=DIRECTION('center_axis',(0.,0.,1.)) ;
#94002=DIRECTION('ref_axis',(1.,0.,0.)) ;
#94003=DIRECTION('center_axis',(0.,0.,-1.)) ;
#94004=DIRECTION('ref_axis',(-1.,0.,0.)) ;
#94005=DIRECTION('center_axis',(0.,1.,0.)) ;
#94006=DIRECTION('ref_axis',(0.,0.,1.)) ;
#94007=DIRECTION('center_axis',(0.,-1.,8.67361737988409E-15)) ;
#94008=DIRECTION('ref_axis',(0.,-8.67361737988409E-15,-1.)) ;
#94009=DIRECTION('center_axis',(0.,0.707106781186546,0.707106781186549)) ;
#94010=DIRECTION('ref_axis',(0.,-0.707106781186549,0.707106781186546)) ;
#94011=DIRECTION('center_axis',(0.,0.707106781186541,0.707106781186554)) ;
#94012=DIRECTION('ref_axis',(0.,-0.707106781186554,0.707106781186541)) ;
#94013=DIRECTION('center_axis',(0.,1.,1.07081696047951E-16)) ;
#94014=DIRECTION('ref_axis',(0.,-1.07081696047951E-16,1.)) ;
#94015=DIRECTION('center_axis',(0.,-1.,0.)) ;
#94016=DIRECTION('ref_axis',(0.,0.,-1.)) ;
#94017=DIRECTION('center_axis',(0.,1.,0.)) ;
#94018=DIRECTION('ref_axis',(0.,0.,1.)) ;
#94019=DIRECTION('center_axis',(0.,0.,1.)) ;
#94020=DIRECTION('ref_axis',(1.,0.,0.)) ;
#94021=DIRECTION('center_axis',(0.,1.,0.)) ;
#94022=DIRECTION('ref_axis',(0.,0.,1.)) ;
#94023=DIRECTION('center_axis',(0.,0.,1.)) ;
#94024=DIRECTION('ref_axis',(1.,0.,0.)) ;
#94025=DIRECTION('center_axis',(0.,3.99416362155027E-15,1.)) ;
#94026=DIRECTION('ref_axis',(0.,-1.,3.99416362155027E-15)) ;
#94027=DIRECTION('center_axis',(0.,0.,1.)) ;
#94028=DIRECTION('ref_axis',(1.,0.,0.)) ;
#94029=DIRECTION('center_axis',(0.,0.,-1.)) ;
#94030=DIRECTION('ref_axis',(-1.,0.,0.)) ;
#94031=DIRECTION('center_axis',(0.,0.,1.)) ;
#94032=DIRECTION('ref_axis',(1.,0.,0.)) ;
#94033=DIRECTION('center_axis',(-1.,0.,0.)) ;
#94034=DIRECTION('ref_axis',(0.,0.,1.)) ;
#94035=DIRECTION('center_axis',(0.,1.,0.)) ;
#94036=DIRECTION('ref_axis',(0.,0.,1.)) ;
#94037=DIRECTION('center_axis',(-1.,0.,0.)) ;
#94038=DIRECTION('ref_axis',(0.,0.,1.)) ;
#94039=DIRECTION('center_axis',(0.,-1.,0.)) ;
#94040=DIRECTION('ref_axis',(0.,0.,-1.)) ;
#94041=DIRECTION('center_axis',(0.,1.,0.)) ;
#94042=DIRECTION('ref_axis',(0.,0.,1.)) ;
#94043=DIRECTION('center_axis',(1.53063836115601E-16,-1.,-1.30104260698261E-16)) ;
#94044=DIRECTION('ref_axis',(1.,1.53063836115601E-16,1.99142572374599E-32)) ;
#94045=DIRECTION('center_axis',(0.,1.,0.)) ;
#94046=DIRECTION('ref_axis',(0.,0.,1.)) ;
#94047=DIRECTION('center_axis',(0.,-1.,0.)) ;
#94048=DIRECTION('ref_axis',(0.,0.,-1.)) ;
#94049=DIRECTION('center_axis',(1.,1.53063836115601E-16,2.73691106313441E-48)) ;
#94050=DIRECTION('ref_axis',(-1.53063836115601E-16,1.,-4.18922106430579E-64)) ;
#94051=DIRECTION('center_axis',(-1.,0.,0.)) ;
#94052=DIRECTION('ref_axis',(0.,0.,1.)) ;
#94053=DIRECTION('center_axis',(1.,1.53063836115601E-16,0.)) ;
#94054=DIRECTION('ref_axis',(1.53063836115601E-16,-1.,0.)) ;
#94055=DIRECTION('center_axis',(0.,1.,0.)) ;
#94056=DIRECTION('ref_axis',(1.,0.,0.)) ;
#94057=DIRECTION('center_axis',(0.,1.,0.)) ;
#94058=DIRECTION('ref_axis',(0.,0.,-1.)) ;
#94059=DIRECTION('center_axis',(0.,0.,1.)) ;
#94060=DIRECTION('ref_axis',(-1.,0.,0.)) ;
#94061=DIRECTION('center_axis',(0.,1.,0.)) ;
#94062=DIRECTION('ref_axis',(1.,0.,0.)) ;
#94063=DIRECTION('center_axis',(0.,0.,1.)) ;
#94064=DIRECTION('ref_axis',(-1.,0.,0.)) ;
#94065=DIRECTION('center_axis',(1.,1.0842021724855E-15,0.)) ;
#94066=DIRECTION('ref_axis',(1.0842021724855E-15,-1.,0.)) ;
#94067=DIRECTION('center_axis',(-1.,-1.53063836115601E-16,0.)) ;
#94068=DIRECTION('ref_axis',(0.,-1.,0.)) ;
#94069=DIRECTION('center_axis',(0.,0.,-1.)) ;
#94070=DIRECTION('ref_axis',(1.,0.,0.)) ;
#94071=DIRECTION('center_axis',(0.,0.,-1.)) ;
#94072=DIRECTION('ref_axis',(0.804034447892622,0.594582716366702,0.)) ;
#94073=DIRECTION('center_axis',(0.,0.,1.)) ;
#94074=DIRECTION('ref_axis',(1.,0.,0.)) ;
#94075=DIRECTION('',(0.,0.,-1.)) ;
#94076=DIRECTION('center_axis',(-2.16840434497101E-16,1.,1.30104260698261E-16)) ;
#94077=DIRECTION('ref_axis',(1.,2.16840434497101E-16,1.22464679914735E-16)) ;
#94078=DIRECTION('',(-2.16840434497101E-16,1.,1.30104260698261E-16)) ;
#94079=DIRECTION('center_axis',(0.,1.,0.)) ;
#94080=DIRECTION('ref_axis',(0.,0.,1.)) ;
#94081=DIRECTION('center_axis',(-1.,-1.53063836115601E-16,-2.73691106313441E-48)) ;
#94082=DIRECTION('ref_axis',(1.53063836115601E-16,-1.,4.18922106430579E-64)) ;
#94083=DIRECTION('center_axis',(1.,2.16840434497101E-16,0.)) ;
#94084=DIRECTION('ref_axis',(2.16840434497101E-16,-1.,0.)) ;
#94085=DIRECTION('center_axis',(0.,0.,1.)) ;
#94086=DIRECTION('ref_axis',(1.,0.,0.)) ;
#94087=DIRECTION('center_axis',(-1.25542992828747E-32,1.020425574104E-16,
1.)) ;
#94088=DIRECTION('ref_axis',(-1.28107280532009E-48,-1.,1.020425574104E-16)) ;
#94089=DIRECTION('center_axis',(0.,0.,1.)) ;
#94090=DIRECTION('ref_axis',(1.,0.,0.)) ;
#94091=DIRECTION('center_axis',(0.,0.,-1.)) ;
#94092=DIRECTION('ref_axis',(-1.,0.,0.)) ;
#94093=DIRECTION('center_axis',(1.,1.53063836115601E-16,-2.73691106313441E-48)) ;
#94094=DIRECTION('ref_axis',(-1.53063836115601E-16,1.,4.18922106430579E-64)) ;
#94095=DIRECTION('center_axis',(-1.,0.,0.)) ;
#94096=DIRECTION('ref_axis',(0.,0.,1.)) ;
#94097=DIRECTION('center_axis',(1.,1.53063836115601E-16,0.)) ;
#94098=DIRECTION('ref_axis',(1.53063836115601E-16,-1.,0.)) ;
#94099=DIRECTION('center_axis',(0.,1.,0.)) ;
#94100=DIRECTION('ref_axis',(1.,0.,0.)) ;
#94101=DIRECTION('center_axis',(-1.,-2.16840434497101E-16,0.)) ;
#94102=DIRECTION('ref_axis',(0.,-1.,0.)) ;
#94103=DIRECTION('center_axis',(0.,0.,-1.)) ;
#94104=DIRECTION('ref_axis',(1.,0.,0.)) ;
#94105=DIRECTION('center_axis',(-1.25542992828747E-32,1.020425574104E-16,
1.)) ;
#94106=DIRECTION('ref_axis',(0.,-1.,0.)) ;
#94107=DIRECTION('center_axis',(0.,-1.,0.)) ;
#94108=DIRECTION('ref_axis',(-6.50521303491307E-15,0.,1.)) ;
#94109=DIRECTION('center_axis',(-1.,0.,0.)) ;
#94110=DIRECTION('ref_axis',(0.,0.,-1.)) ;
#94111=DIRECTION('center_axis',(-1.,-1.53063836115601E-16,0.)) ;
#94112=DIRECTION('ref_axis',(0.,-1.,0.)) ;
#94113=DIRECTION('center_axis',(0.,-1.,0.)) ;
#94114=DIRECTION('ref_axis',(0.,0.,1.)) ;
#94115=DIRECTION('center_axis',(0.,0.,-1.)) ;
#94116=DIRECTION('ref_axis',(-1.,0.,0.)) ;
#94117=DIRECTION('center_axis',(0.,0.,-1.)) ;
#94118=DIRECTION('ref_axis',(-1.,0.,0.)) ;
#94119=DIRECTION('center_axis',(1.,1.53063836115601E-16,-3.06472600140763E-33)) ;
#94120=DIRECTION('ref_axis',(-1.53063836115601E-16,1.,4.69098718418678E-49)) ;
#94121=DIRECTION('center_axis',(-1.,0.,0.)) ;
#94122=DIRECTION('ref_axis',(0.,0.,1.)) ;
#94123=DIRECTION('center_axis',(-1.53063836115601E-16,1.,-1.020425574104E-16)) ;
#94124=DIRECTION('ref_axis',(-1.,-1.53063836115601E-16,1.3684555315672E-47)) ;
#94125=DIRECTION('',(1.53063836115601E-16,-1.,1.020425574104E-16)) ;
#94126=DIRECTION('center_axis',(0.,-1.,0.)) ;
#94127=DIRECTION('ref_axis',(0.,0.,-1.)) ;
#94128=DIRECTION('center_axis',(-1.53063836115601E-16,1.,-1.30104260698261E-16)) ;
#94129=DIRECTION('ref_axis',(-1.,-1.53063836115601E-16,1.99142572374599E-32)) ;
#94130=DIRECTION('center_axis',(0.,-1.,0.)) ;
#94131=DIRECTION('ref_axis',(0.,0.,-1.)) ;
#94132=DIRECTION('center_axis',(-1.,-1.53063836115601E-16,2.73691106313441E-48)) ;
#94133=DIRECTION('ref_axis',(1.53063836115601E-16,-1.,-4.18922106430579E-64)) ;
#94134=DIRECTION('center_axis',(1.,2.16840434497101E-16,0.)) ;
#94135=DIRECTION('ref_axis',(2.16840434497101E-16,-1.,0.)) ;
#94136=DIRECTION('center_axis',(-1.,0.,2.16840434497102E-15)) ;
#94137=DIRECTION('ref_axis',(2.16840434497102E-15,0.,1.)) ;
#94138=DIRECTION('center_axis',(-1.,-2.16840434497101E-16,0.)) ;
#94139=DIRECTION('ref_axis',(0.,-1.,0.)) ;
#94140=DIRECTION('center_axis',(0.,0.,1.)) ;
#94141=DIRECTION('ref_axis',(-1.,0.,0.)) ;
#94142=DIRECTION('center_axis',(0.,1.,0.)) ;
#94143=DIRECTION('ref_axis',(1.,0.,0.)) ;
#94144=DIRECTION('center_axis',(0.,1.,0.)) ;
#94145=DIRECTION('ref_axis',(0.,0.,-1.)) ;
#94146=DIRECTION('center_axis',(1.,0.,0.)) ;
#94147=DIRECTION('ref_axis',(0.,-1.,0.)) ;
#94148=DIRECTION('center_axis',(1.,6.50521303491304E-15,0.)) ;
#94149=DIRECTION('ref_axis',(-6.50521303491304E-15,1.,0.)) ;
#94150=DIRECTION('center_axis',(8.67361737988403E-15,1.,0.)) ;
#94151=DIRECTION('ref_axis',(-1.,8.67361737988403E-15,0.)) ;
#94152=DIRECTION('center_axis',(1.2303003375722E-16,-1.,1.020425574104E-16)) ;
#94153=DIRECTION('ref_axis',(1.,1.2303003375722E-16,-1.25542992828747E-32)) ;
#94154=DIRECTION('center_axis',(0.,1.,0.)) ;
#94155=DIRECTION('ref_axis',(0.,0.,1.)) ;
#94156=DIRECTION('center_axis',(0.,1.,0.)) ;
#94157=DIRECTION('ref_axis',(1.,0.,0.)) ;
#94158=DIRECTION('center_axis',(1.,1.2303003375722E-16,0.)) ;
#94159=DIRECTION('ref_axis',(1.2303003375722E-16,-1.,0.)) ;
#94160=DIRECTION('center_axis',(0.,0.,1.)) ;
#94161=DIRECTION('ref_axis',(-1.,0.,0.)) ;
#94162=DIRECTION('center_axis',(0.,1.,0.)) ;
#94163=DIRECTION('ref_axis',(1.,0.,0.)) ;
#94164=DIRECTION('center_axis',(0.,0.,-1.)) ;
#94165=DIRECTION('ref_axis',(1.,0.,0.)) ;
#94166=DIRECTION('center_axis',(0.,0.,-1.)) ;
#94167=DIRECTION('ref_axis',(-1.,0.,0.)) ;
#94168=DIRECTION('center_axis',(0.,0.,1.)) ;
#94169=DIRECTION('ref_axis',(1.,0.,0.)) ;
#94170=DIRECTION('center_axis',(-2.16840434497101E-16,1.,-1.020425574104E-16)) ;
#94171=DIRECTION('ref_axis',(-1.,-2.16840434497101E-16,5.47382212626882E-48)) ;
#94172=DIRECTION('center_axis',(0.,1.,0.)) ;
#94173=DIRECTION('ref_axis',(0.,0.,-1.)) ;
#94174=DIRECTION('center_axis',(1.,0.,1.25542992828747E-32)) ;
#94175=DIRECTION('ref_axis',(1.25542992828747E-32,0.,-1.)) ;
#94176=DIRECTION('center_axis',(1.,0.,0.)) ;
#94177=DIRECTION('ref_axis',(0.,0.,-1.)) ;
#94178=DIRECTION('center_axis',(-1.,-1.2303003375722E-16,0.)) ;
#94179=DIRECTION('ref_axis',(0.,-1.,0.)) ;
#94180=DIRECTION('center_axis',(0.,0.,-1.)) ;
#94181=DIRECTION('ref_axis',(1.,0.,0.)) ;
#94182=DIRECTION('center_axis',(0.,0.,-1.)) ;
#94183=DIRECTION('ref_axis',(-1.,0.,0.)) ;
#94184=DIRECTION('',(0.,0.,1.)) ;
#94185=DIRECTION('center_axis',(0.,0.,1.)) ;
#94186=DIRECTION('ref_axis',(1.,0.,0.)) ;
#94187=DIRECTION('center_axis',(0.,0.,1.)) ;
#94188=DIRECTION('ref_axis',(1.,0.,0.)) ;
#94189=DIRECTION('center_axis',(6.27714964143733E-33,-5.10212787052002E-17,
-1.)) ;
#94190=DIRECTION('ref_axis',(3.20268201330022E-49,1.,-5.10212787052002E-17)) ;
#94191=DIRECTION('center_axis',(1.,1.53063836115601E-16,-1.53236300070382E-33)) ;
#94192=DIRECTION('ref_axis',(-1.53063836115601E-16,1.,2.34549359209339E-49)) ;
#94193=DIRECTION('center_axis',(-1.,0.,0.)) ;
#94194=DIRECTION('ref_axis',(0.,0.,1.)) ;
#94195=DIRECTION('center_axis',(1.,0.,0.)) ;
#94196=DIRECTION('ref_axis',(0.,0.,-1.)) ;
#94197=DIRECTION('center_axis',(0.,1.,0.)) ;
#94198=DIRECTION('ref_axis',(1.,0.,0.)) ;
#94199=DIRECTION('center_axis',(-4.33680868994202E-15,1.,0.)) ;
#94200=DIRECTION('ref_axis',(1.,4.33680868994202E-15,0.)) ;
#94201=DIRECTION('center_axis',(0.,-1.,0.)) ;
#94202=DIRECTION('ref_axis',(0.,0.,-1.)) ;
#94203=DIRECTION('center_axis',(0.,0.,-1.)) ;
#94204=DIRECTION('ref_axis',(1.,0.,0.)) ;
#94205=DIRECTION('center_axis',(0.,0.,1.)) ;
#94206=DIRECTION('ref_axis',(1.,0.,0.)) ;
#94207=DIRECTION('center_axis',(0.,0.,-1.)) ;
#94208=DIRECTION('ref_axis',(-1.,0.,0.)) ;
#94209=DIRECTION('center_axis',(0.,1.,0.)) ;
#94210=DIRECTION('ref_axis',(1.,0.,0.)) ;
#94211=DIRECTION('center_axis',(1.,1.2303003375722E-16,0.)) ;
#94212=DIRECTION('ref_axis',(1.2303003375722E-16,-1.,0.)) ;
#94213=DIRECTION('center_axis',(0.,1.,0.)) ;
#94214=DIRECTION('ref_axis',(-6.50521303491307E-15,0.,-1.)) ;
#94215=DIRECTION('center_axis',(6.27714964143733E-33,-5.10212787052002E-17,
-1.)) ;
#94216=DIRECTION('ref_axis',(0.,1.,0.)) ;
#94217=DIRECTION('center_axis',(0.,-1.,0.)) ;
#94218=DIRECTION('ref_axis',(0.,0.,1.)) ;
#94219=DIRECTION('center_axis',(2.16840434497101E-16,-1.,5.10212787052002E-17)) ;
#94220=DIRECTION('ref_axis',(1.,2.16840434497101E-16,-5.47382212626882E-48)) ;
#94221=DIRECTION('center_axis',(0.,1.,0.)) ;
#94222=DIRECTION('ref_axis',(0.,0.,-1.)) ;
#94223=DIRECTION('center_axis',(0.,0.,1.)) ;
#94224=DIRECTION('ref_axis',(1.,0.,0.)) ;
#94225=DIRECTION('center_axis',(0.,0.,-1.)) ;
#94226=DIRECTION('ref_axis',(-1.,0.,0.)) ;
#94227=DIRECTION('center_axis',(-1.,-1.2303003375722E-16,0.)) ;
#94228=DIRECTION('ref_axis',(0.,-1.,0.)) ;
#94229=DIRECTION('center_axis',(0.,-1.,0.)) ;
#94230=DIRECTION('ref_axis',(0.,0.,1.)) ;
#94231=DIRECTION('center_axis',(1.53063836115601E-16,-1.,5.10212787052002E-17)) ;
#94232=DIRECTION('ref_axis',(1.,1.53063836115601E-16,-6.84227765783602E-48)) ;
#94233=DIRECTION('',(-1.53063836115601E-16,1.,-5.10212787052002E-17)) ;
#94234=DIRECTION('center_axis',(0.,-1.,0.)) ;
#94235=DIRECTION('ref_axis',(0.,0.,-1.)) ;
#94236=DIRECTION('center_axis',(-1.,0.,0.)) ;
#94237=DIRECTION('ref_axis',(0.,0.,-1.)) ;
#94238=DIRECTION('center_axis',(-1.2303003375722E-16,1.,-5.10212787052002E-17)) ;
#94239=DIRECTION('ref_axis',(-1.,-1.2303003375722E-16,6.27714964143733E-33)) ;
#94240=DIRECTION('center_axis',(-8.67361737988403E-15,-1.,0.)) ;
#94241=DIRECTION('ref_axis',(1.,-8.67361737988403E-15,0.)) ;
#94242=DIRECTION('center_axis',(1.,0.,6.27714964143733E-33)) ;
#94243=DIRECTION('ref_axis',(6.27714964143733E-33,0.,-1.)) ;
#94244=DIRECTION('center_axis',(-1.,0.,-6.50521303491307E-15)) ;
#94245=DIRECTION('ref_axis',(-6.50521303491307E-15,0.,1.)) ;
#94246=DIRECTION('center_axis',(1.,0.,0.)) ;
#94247=DIRECTION('ref_axis',(0.,1.,0.)) ;
#94248=DIRECTION('center_axis',(0.,0.,-1.)) ;
#94249=DIRECTION('ref_axis',(-1.,0.,0.)) ;
#94250=DIRECTION('center_axis',(0.,0.,1.)) ;
#94251=DIRECTION('ref_axis',(1.,0.,0.)) ;
#94252=DIRECTION('center_axis',(0.,0.,-1.)) ;
#94253=DIRECTION('ref_axis',(-1.,0.,0.)) ;
#94254=DIRECTION('center_axis',(-1.,0.,0.)) ;
#94255=DIRECTION('ref_axis',(0.,0.,1.)) ;
#94256=DIRECTION('center_axis',(0.,-1.,0.)) ;
#94257=DIRECTION('ref_axis',(0.,0.,-1.)) ;
#94258=DIRECTION('center_axis',(0.,1.,0.)) ;
#94259=DIRECTION('ref_axis',(0.,0.,1.)) ;
#94260=DIRECTION('center_axis',(0.,1.,-6.50521303491307E-15)) ;
#94261=DIRECTION('ref_axis',(0.,6.50521303491307E-15,1.)) ;
#94262=DIRECTION('center_axis',(0.,-1.,0.)) ;
#94263=DIRECTION('ref_axis',(0.,0.,-1.)) ;
#94264=DIRECTION('center_axis',(0.,-1.,0.)) ;
#94265=DIRECTION('ref_axis',(0.,0.,-1.)) ;
#94266=DIRECTION('center_axis',(0.,-1.,-1.07081696047951E-16)) ;
#94267=DIRECTION('ref_axis',(0.,1.07081696047951E-16,-1.)) ;
#94268=DIRECTION('center_axis',(0.,1.,0.)) ;
#94269=DIRECTION('ref_axis',(0.,0.,1.)) ;
#94270=DIRECTION('center_axis',(-1.,0.,0.)) ;
#94271=DIRECTION('ref_axis',(0.,0.,1.)) ;
#94272=DIRECTION('center_axis',(0.,0.,1.)) ;
#94273=DIRECTION('ref_axis',(1.,0.,0.)) ;
#94274=DIRECTION('center_axis',(0.,1.,0.)) ;
#94275=DIRECTION('ref_axis',(0.,0.,1.)) ;
#94276=DIRECTION('center_axis',(0.,0.,-1.)) ;
#94277=DIRECTION('ref_axis',(-1.,0.,0.)) ;
#94278=DIRECTION('center_axis',(0.,0.,1.)) ;
#94279=DIRECTION('ref_axis',(1.,0.,0.)) ;
#94280=DIRECTION('center_axis',(0.,0.,1.)) ;
#94281=DIRECTION('ref_axis',(1.,0.,0.)) ;
#94282=DIRECTION('center_axis',(0.,0.,1.)) ;
#94283=DIRECTION('ref_axis',(1.,0.,0.)) ;
#94284=DIRECTION('center_axis',(0.,0.,-1.)) ;
#94285=DIRECTION('ref_axis',(-1.,0.,0.)) ;
#94286=DIRECTION('center_axis',(0.,1.,0.)) ;
#94287=DIRECTION('ref_axis',(0.,0.,1.)) ;
#94288=DIRECTION('center_axis',(0.,-0.707106781186558,0.707106781186537)) ;
#94289=DIRECTION('ref_axis',(0.,-0.707106781186537,-0.707106781186558)) ;
#94290=DIRECTION('center_axis',(0.,1.,0.)) ;
#94291=DIRECTION('ref_axis',(0.,0.,1.)) ;
#94292=DIRECTION('center_axis',(0.,-0.514231796959093,-0.857651245551607)) ;
#94293=DIRECTION('ref_axis',(0.,0.857651245551607,-0.514231796959093)) ;
#94294=DIRECTION('center_axis',(0.,-0.707106781186548,0.707106781186547)) ;
#94295=DIRECTION('ref_axis',(0.,-0.707106781186547,-0.707106781186548)) ;
#94296=DIRECTION('center_axis',(0.,-0.707106781186548,0.707106781186548)) ;
#94297=DIRECTION('ref_axis',(0.,-0.707106781186548,-0.707106781186548)) ;
#94298=DIRECTION('center_axis',(-1.,0.,0.)) ;
#94299=DIRECTION('ref_axis',(0.,0.,1.)) ;
#94300=DIRECTION('center_axis',(0.,0.514231796959095,-0.857651245551606)) ;
#94301=DIRECTION('ref_axis',(0.,0.857651245551606,0.514231796959095)) ;
#94302=DIRECTION('center_axis',(0.,1.,0.)) ;
#94303=DIRECTION('ref_axis',(0.,0.,1.)) ;
#94304=DIRECTION('center_axis',(0.,0.,-1.)) ;
#94305=DIRECTION('ref_axis',(-1.,0.,0.)) ;
#94306=DIRECTION('center_axis',(0.,1.,0.)) ;
#94307=DIRECTION('ref_axis',(0.,0.,1.)) ;
#94308=DIRECTION('center_axis',(0.,0.,-1.)) ;
#94309=DIRECTION('ref_axis',(-1.,0.,0.)) ;
#94310=DIRECTION('center_axis',(0.,0.,-1.)) ;
#94311=DIRECTION('ref_axis',(-1.,0.,0.)) ;
#94312=DIRECTION('center_axis',(0.,0.,1.)) ;
#94313=DIRECTION('ref_axis',(1.,0.,0.)) ;
#94314=DIRECTION('center_axis',(0.,0.,-1.)) ;
#94315=DIRECTION('ref_axis',(-1.,0.,0.)) ;
#94316=DIRECTION('center_axis',(0.,1.,0.)) ;
#94317=DIRECTION('ref_axis',(0.,0.,1.)) ;
#94318=DIRECTION('center_axis',(0.,-1.,8.67361737988409E-15)) ;
#94319=DIRECTION('ref_axis',(0.,-8.67361737988409E-15,-1.)) ;
#94320=DIRECTION('center_axis',(0.,0.707106781186546,0.707106781186549)) ;
#94321=DIRECTION('ref_axis',(0.,-0.707106781186549,0.707106781186546)) ;
#94322=DIRECTION('center_axis',(0.,0.707106781186537,0.707106781186558)) ;
#94323=DIRECTION('ref_axis',(0.,-0.707106781186558,0.707106781186537)) ;
#94324=DIRECTION('center_axis',(0.,1.,1.07081696047951E-16)) ;
#94325=DIRECTION('ref_axis',(0.,-1.07081696047951E-16,1.)) ;
#94326=DIRECTION('center_axis',(0.,-1.,0.)) ;
#94327=DIRECTION('ref_axis',(0.,0.,-1.)) ;
#94328=DIRECTION('center_axis',(0.,1.,0.)) ;
#94329=DIRECTION('ref_axis',(0.,0.,1.)) ;
#94330=DIRECTION('center_axis',(0.,0.,1.)) ;
#94331=DIRECTION('ref_axis',(1.,0.,0.)) ;
#94332=DIRECTION('center_axis',(0.,1.,0.)) ;
#94333=DIRECTION('ref_axis',(0.,0.,1.)) ;
#94334=DIRECTION('center_axis',(0.,0.,1.)) ;
#94335=DIRECTION('ref_axis',(1.,0.,0.)) ;
#94336=DIRECTION('center_axis',(0.,3.99416362155027E-15,1.)) ;
#94337=DIRECTION('ref_axis',(0.,-1.,3.99416362155027E-15)) ;
#94338=DIRECTION('center_axis',(0.,0.,1.)) ;
#94339=DIRECTION('ref_axis',(1.,0.,0.)) ;
#94340=DIRECTION('center_axis',(0.,0.,-1.)) ;
#94341=DIRECTION('ref_axis',(-1.,0.,0.)) ;
#94342=DIRECTION('center_axis',(0.,0.,1.)) ;
#94343=DIRECTION('ref_axis',(1.,0.,0.)) ;
#94344=DIRECTION('center_axis',(-1.,0.,0.)) ;
#94345=DIRECTION('ref_axis',(0.,0.,1.)) ;
#94346=DIRECTION('center_axis',(0.,1.,0.)) ;
#94347=DIRECTION('ref_axis',(0.,0.,1.)) ;
#94348=DIRECTION('center_axis',(-1.,0.,0.)) ;
#94349=DIRECTION('ref_axis',(0.,0.,1.)) ;
#94350=DIRECTION('center_axis',(0.,-1.,0.)) ;
#94351=DIRECTION('ref_axis',(0.,0.,-1.)) ;
#94352=DIRECTION('center_axis',(0.,1.,0.)) ;
#94353=DIRECTION('ref_axis',(0.,0.,1.)) ;
#94354=DIRECTION('center_axis',(1.53063836115601E-16,-1.,-1.30104260698261E-16)) ;
#94355=DIRECTION('ref_axis',(1.,1.53063836115601E-16,1.99142572374599E-32)) ;
#94356=DIRECTION('center_axis',(0.,1.,0.)) ;
#94357=DIRECTION('ref_axis',(0.,0.,1.)) ;
#94358=DIRECTION('center_axis',(0.,-1.,0.)) ;
#94359=DIRECTION('ref_axis',(0.,0.,-1.)) ;
#94360=DIRECTION('center_axis',(1.,1.53063836115601E-16,2.73691106313441E-48)) ;
#94361=DIRECTION('ref_axis',(-1.53063836115601E-16,1.,-4.18922106430579E-64)) ;
#94362=DIRECTION('center_axis',(-1.,0.,0.)) ;
#94363=DIRECTION('ref_axis',(0.,0.,1.)) ;
#94364=DIRECTION('center_axis',(1.,1.53063836115601E-16,0.)) ;
#94365=DIRECTION('ref_axis',(1.53063836115601E-16,-1.,0.)) ;
#94366=DIRECTION('center_axis',(0.,1.,0.)) ;
#94367=DIRECTION('ref_axis',(1.,0.,0.)) ;
#94368=DIRECTION('center_axis',(0.,1.,0.)) ;
#94369=DIRECTION('ref_axis',(0.,0.,-1.)) ;
#94370=DIRECTION('center_axis',(0.,0.,1.)) ;
#94371=DIRECTION('ref_axis',(-1.,0.,0.)) ;
#94372=DIRECTION('center_axis',(0.,1.,0.)) ;
#94373=DIRECTION('ref_axis',(1.,0.,0.)) ;
#94374=DIRECTION('center_axis',(0.,0.,1.)) ;
#94375=DIRECTION('ref_axis',(-1.,0.,0.)) ;
#94376=DIRECTION('center_axis',(1.,1.0842021724855E-15,0.)) ;
#94377=DIRECTION('ref_axis',(1.0842021724855E-15,-1.,0.)) ;
#94378=DIRECTION('center_axis',(-1.,-1.53063836115601E-16,0.)) ;
#94379=DIRECTION('ref_axis',(0.,-1.,0.)) ;
#94380=DIRECTION('center_axis',(0.,0.,-1.)) ;
#94381=DIRECTION('ref_axis',(1.,0.,0.)) ;
#94382=DIRECTION('center_axis',(0.,0.,-1.)) ;
#94383=DIRECTION('ref_axis',(0.804034447892617,0.594582716366709,0.)) ;
#94384=DIRECTION('center_axis',(0.,0.,1.)) ;
#94385=DIRECTION('ref_axis',(1.,0.,0.)) ;
#94386=DIRECTION('',(0.,0.,-1.)) ;
#94387=DIRECTION('center_axis',(-2.16840434497101E-16,1.,1.30104260698261E-16)) ;
#94388=DIRECTION('ref_axis',(1.,2.16840434497101E-16,1.22464679914735E-16)) ;
#94389=DIRECTION('',(-2.16840434497101E-16,1.,1.30104260698261E-16)) ;
#94390=DIRECTION('center_axis',(0.,1.,0.)) ;
#94391=DIRECTION('ref_axis',(0.,0.,1.)) ;
#94392=DIRECTION('center_axis',(-1.,-1.53063836115601E-16,-2.73691106313441E-48)) ;
#94393=DIRECTION('ref_axis',(1.53063836115601E-16,-1.,4.18922106430579E-64)) ;
#94394=DIRECTION('center_axis',(1.,2.16840434497101E-16,0.)) ;
#94395=DIRECTION('ref_axis',(2.16840434497101E-16,-1.,0.)) ;
#94396=DIRECTION('center_axis',(0.,0.,1.)) ;
#94397=DIRECTION('ref_axis',(1.,0.,0.)) ;
#94398=DIRECTION('center_axis',(-1.25542992828747E-32,1.020425574104E-16,
1.)) ;
#94399=DIRECTION('ref_axis',(-1.28107280532009E-48,-1.,1.020425574104E-16)) ;
#94400=DIRECTION('center_axis',(0.,0.,1.)) ;
#94401=DIRECTION('ref_axis',(1.,0.,0.)) ;
#94402=DIRECTION('center_axis',(0.,0.,-1.)) ;
#94403=DIRECTION('ref_axis',(-1.,0.,0.)) ;
#94404=DIRECTION('center_axis',(1.,1.53063836115601E-16,-2.73691106313441E-48)) ;
#94405=DIRECTION('ref_axis',(-1.53063836115601E-16,1.,4.18922106430579E-64)) ;
#94406=DIRECTION('center_axis',(-1.,0.,0.)) ;
#94407=DIRECTION('ref_axis',(0.,0.,1.)) ;
#94408=DIRECTION('center_axis',(1.,1.53063836115601E-16,0.)) ;
#94409=DIRECTION('ref_axis',(1.53063836115601E-16,-1.,0.)) ;
#94410=DIRECTION('center_axis',(0.,1.,0.)) ;
#94411=DIRECTION('ref_axis',(1.,0.,0.)) ;
#94412=DIRECTION('center_axis',(-1.,-2.16840434497101E-16,0.)) ;
#94413=DIRECTION('ref_axis',(0.,-1.,0.)) ;
#94414=DIRECTION('center_axis',(0.,0.,-1.)) ;
#94415=DIRECTION('ref_axis',(1.,0.,0.)) ;
#94416=DIRECTION('center_axis',(-1.25542992828747E-32,1.020425574104E-16,
1.)) ;
#94417=DIRECTION('ref_axis',(0.,-1.,0.)) ;
#94418=DIRECTION('center_axis',(0.,-1.,0.)) ;
#94419=DIRECTION('ref_axis',(-6.50521303491307E-15,0.,1.)) ;
#94420=DIRECTION('center_axis',(-1.,0.,0.)) ;
#94421=DIRECTION('ref_axis',(0.,0.,-1.)) ;
#94422=DIRECTION('center_axis',(-1.,-1.53063836115601E-16,0.)) ;
#94423=DIRECTION('ref_axis',(0.,-1.,0.)) ;
#94424=DIRECTION('center_axis',(0.,-1.,0.)) ;
#94425=DIRECTION('ref_axis',(0.,0.,1.)) ;
#94426=DIRECTION('center_axis',(0.,0.,-1.)) ;
#94427=DIRECTION('ref_axis',(-1.,0.,0.)) ;
#94428=DIRECTION('center_axis',(0.,0.,-1.)) ;
#94429=DIRECTION('ref_axis',(-1.,0.,0.)) ;
#94430=DIRECTION('center_axis',(1.,1.53063836115601E-16,-3.06472600140763E-33)) ;
#94431=DIRECTION('ref_axis',(-1.53063836115601E-16,1.,4.69098718418678E-49)) ;
#94432=DIRECTION('center_axis',(-1.,0.,0.)) ;
#94433=DIRECTION('ref_axis',(0.,0.,1.)) ;
#94434=DIRECTION('center_axis',(-1.53063836115601E-16,1.,-1.020425574104E-16)) ;
#94435=DIRECTION('ref_axis',(-1.,-1.53063836115601E-16,1.3684555315672E-47)) ;
#94436=DIRECTION('',(1.53063836115601E-16,-1.,1.020425574104E-16)) ;
#94437=DIRECTION('center_axis',(0.,-1.,0.)) ;
#94438=DIRECTION('ref_axis',(0.,0.,-1.)) ;
#94439=DIRECTION('center_axis',(-1.53063836115601E-16,1.,-1.30104260698261E-16)) ;
#94440=DIRECTION('ref_axis',(-1.,-1.53063836115601E-16,1.99142572374599E-32)) ;
#94441=DIRECTION('center_axis',(0.,-1.,0.)) ;
#94442=DIRECTION('ref_axis',(0.,0.,-1.)) ;
#94443=DIRECTION('center_axis',(-1.,-1.53063836115601E-16,2.73691106313441E-48)) ;
#94444=DIRECTION('ref_axis',(1.53063836115601E-16,-1.,-4.18922106430579E-64)) ;
#94445=DIRECTION('center_axis',(1.,2.16840434497101E-16,0.)) ;
#94446=DIRECTION('ref_axis',(2.16840434497101E-16,-1.,0.)) ;
#94447=DIRECTION('center_axis',(-1.,0.,2.16840434497102E-15)) ;
#94448=DIRECTION('ref_axis',(2.16840434497102E-15,0.,1.)) ;
#94449=DIRECTION('center_axis',(-1.,-2.16840434497101E-16,0.)) ;
#94450=DIRECTION('ref_axis',(0.,-1.,0.)) ;
#94451=DIRECTION('center_axis',(0.,0.,1.)) ;
#94452=DIRECTION('ref_axis',(-1.,0.,0.)) ;
#94453=DIRECTION('center_axis',(0.,1.,0.)) ;
#94454=DIRECTION('ref_axis',(1.,0.,0.)) ;
#94455=DIRECTION('center_axis',(0.,1.,0.)) ;
#94456=DIRECTION('ref_axis',(0.,0.,-1.)) ;
#94457=DIRECTION('center_axis',(1.,0.,0.)) ;
#94458=DIRECTION('ref_axis',(0.,-1.,0.)) ;
#94459=DIRECTION('center_axis',(1.,6.50521303491304E-15,0.)) ;
#94460=DIRECTION('ref_axis',(-6.50521303491304E-15,1.,0.)) ;
#94461=DIRECTION('center_axis',(8.67361737988403E-15,1.,0.)) ;
#94462=DIRECTION('ref_axis',(-1.,8.67361737988403E-15,0.)) ;
#94463=DIRECTION('center_axis',(1.2303003375722E-16,-1.,1.020425574104E-16)) ;
#94464=DIRECTION('ref_axis',(1.,1.2303003375722E-16,-1.25542992828747E-32)) ;
#94465=DIRECTION('center_axis',(0.,1.,0.)) ;
#94466=DIRECTION('ref_axis',(0.,0.,1.)) ;
#94467=DIRECTION('center_axis',(0.,1.,0.)) ;
#94468=DIRECTION('ref_axis',(1.,0.,0.)) ;
#94469=DIRECTION('center_axis',(1.,1.2303003375722E-16,0.)) ;
#94470=DIRECTION('ref_axis',(1.2303003375722E-16,-1.,0.)) ;
#94471=DIRECTION('center_axis',(0.,0.,1.)) ;
#94472=DIRECTION('ref_axis',(-1.,0.,0.)) ;
#94473=DIRECTION('center_axis',(0.,1.,0.)) ;
#94474=DIRECTION('ref_axis',(1.,0.,0.)) ;
#94475=DIRECTION('center_axis',(0.,0.,-1.)) ;
#94476=DIRECTION('ref_axis',(1.,0.,0.)) ;
#94477=DIRECTION('center_axis',(0.,0.,-1.)) ;
#94478=DIRECTION('ref_axis',(-1.,0.,0.)) ;
#94479=DIRECTION('center_axis',(0.,0.,1.)) ;
#94480=DIRECTION('ref_axis',(1.,0.,0.)) ;
#94481=DIRECTION('center_axis',(-2.16840434497101E-16,1.,-1.020425574104E-16)) ;
#94482=DIRECTION('ref_axis',(-1.,-2.16840434497101E-16,5.47382212626882E-48)) ;
#94483=DIRECTION('center_axis',(0.,1.,0.)) ;
#94484=DIRECTION('ref_axis',(0.,0.,-1.)) ;
#94485=DIRECTION('center_axis',(1.,0.,1.25542992828747E-32)) ;
#94486=DIRECTION('ref_axis',(1.25542992828747E-32,0.,-1.)) ;
#94487=DIRECTION('center_axis',(1.,0.,0.)) ;
#94488=DIRECTION('ref_axis',(0.,0.,-1.)) ;
#94489=DIRECTION('center_axis',(-1.,-1.2303003375722E-16,0.)) ;
#94490=DIRECTION('ref_axis',(0.,-1.,0.)) ;
#94491=DIRECTION('center_axis',(0.,0.,-1.)) ;
#94492=DIRECTION('ref_axis',(1.,0.,0.)) ;
#94493=DIRECTION('center_axis',(0.,0.,-1.)) ;
#94494=DIRECTION('ref_axis',(-1.,0.,0.)) ;
#94495=DIRECTION('',(0.,0.,1.)) ;
#94496=DIRECTION('center_axis',(0.,0.,1.)) ;
#94497=DIRECTION('ref_axis',(1.,0.,0.)) ;
#94498=DIRECTION('center_axis',(0.,0.,1.)) ;
#94499=DIRECTION('ref_axis',(1.,0.,0.)) ;
#94500=DIRECTION('center_axis',(6.27714964143733E-33,-5.10212787052002E-17,
-1.)) ;
#94501=DIRECTION('ref_axis',(3.20268201330022E-49,1.,-5.10212787052002E-17)) ;
#94502=DIRECTION('center_axis',(1.,1.53063836115601E-16,-1.53236300070382E-33)) ;
#94503=DIRECTION('ref_axis',(-1.53063836115601E-16,1.,2.34549359209339E-49)) ;
#94504=DIRECTION('center_axis',(-1.,0.,0.)) ;
#94505=DIRECTION('ref_axis',(0.,0.,1.)) ;
#94506=DIRECTION('center_axis',(1.,0.,0.)) ;
#94507=DIRECTION('ref_axis',(0.,0.,-1.)) ;
#94508=DIRECTION('center_axis',(0.,1.,0.)) ;
#94509=DIRECTION('ref_axis',(1.,0.,0.)) ;
#94510=DIRECTION('center_axis',(-4.33680868994202E-15,1.,0.)) ;
#94511=DIRECTION('ref_axis',(1.,4.33680868994202E-15,0.)) ;
#94512=DIRECTION('center_axis',(0.,-1.,0.)) ;
#94513=DIRECTION('ref_axis',(0.,0.,-1.)) ;
#94514=DIRECTION('center_axis',(0.,0.,-1.)) ;
#94515=DIRECTION('ref_axis',(1.,0.,0.)) ;
#94516=DIRECTION('center_axis',(0.,0.,1.)) ;
#94517=DIRECTION('ref_axis',(1.,0.,0.)) ;
#94518=DIRECTION('center_axis',(0.,0.,-1.)) ;
#94519=DIRECTION('ref_axis',(-1.,0.,0.)) ;
#94520=DIRECTION('center_axis',(0.,1.,0.)) ;
#94521=DIRECTION('ref_axis',(1.,0.,0.)) ;
#94522=DIRECTION('center_axis',(1.,1.2303003375722E-16,0.)) ;
#94523=DIRECTION('ref_axis',(1.2303003375722E-16,-1.,0.)) ;
#94524=DIRECTION('center_axis',(0.,1.,0.)) ;
#94525=DIRECTION('ref_axis',(-6.50521303491307E-15,0.,-1.)) ;
#94526=DIRECTION('center_axis',(6.27714964143733E-33,-5.10212787052002E-17,
-1.)) ;
#94527=DIRECTION('ref_axis',(0.,1.,0.)) ;
#94528=DIRECTION('center_axis',(0.,-1.,0.)) ;
#94529=DIRECTION('ref_axis',(0.,0.,1.)) ;
#94530=DIRECTION('center_axis',(2.16840434497101E-16,-1.,5.10212787052002E-17)) ;
#94531=DIRECTION('ref_axis',(1.,2.16840434497101E-16,-5.47382212626882E-48)) ;
#94532=DIRECTION('center_axis',(0.,1.,0.)) ;
#94533=DIRECTION('ref_axis',(0.,0.,-1.)) ;
#94534=DIRECTION('center_axis',(0.,0.,1.)) ;
#94535=DIRECTION('ref_axis',(1.,0.,0.)) ;
#94536=DIRECTION('center_axis',(0.,0.,-1.)) ;
#94537=DIRECTION('ref_axis',(-1.,0.,0.)) ;
#94538=DIRECTION('center_axis',(-1.,-1.2303003375722E-16,0.)) ;
#94539=DIRECTION('ref_axis',(0.,-1.,0.)) ;
#94540=DIRECTION('center_axis',(0.,-1.,0.)) ;
#94541=DIRECTION('ref_axis',(0.,0.,1.)) ;
#94542=DIRECTION('center_axis',(1.53063836115601E-16,-1.,5.10212787052002E-17)) ;
#94543=DIRECTION('ref_axis',(1.,1.53063836115601E-16,-6.84227765783602E-48)) ;
#94544=DIRECTION('',(-1.53063836115601E-16,1.,-5.10212787052002E-17)) ;
#94545=DIRECTION('center_axis',(0.,-1.,0.)) ;
#94546=DIRECTION('ref_axis',(0.,0.,-1.)) ;
#94547=DIRECTION('center_axis',(-1.,0.,0.)) ;
#94548=DIRECTION('ref_axis',(0.,0.,-1.)) ;
#94549=DIRECTION('center_axis',(-1.2303003375722E-16,1.,-5.10212787052002E-17)) ;
#94550=DIRECTION('ref_axis',(-1.,-1.2303003375722E-16,6.27714964143733E-33)) ;
#94551=DIRECTION('center_axis',(-8.67361737988403E-15,-1.,0.)) ;
#94552=DIRECTION('ref_axis',(1.,-8.67361737988403E-15,0.)) ;
#94553=DIRECTION('center_axis',(1.,0.,6.27714964143733E-33)) ;
#94554=DIRECTION('ref_axis',(6.27714964143733E-33,0.,-1.)) ;
#94555=DIRECTION('center_axis',(-1.,0.,-6.50521303491307E-15)) ;
#94556=DIRECTION('ref_axis',(-6.50521303491307E-15,0.,1.)) ;
#94557=DIRECTION('center_axis',(1.,0.,0.)) ;
#94558=DIRECTION('ref_axis',(0.,1.,0.)) ;
#94559=DIRECTION('center_axis',(0.,0.,-1.)) ;
#94560=DIRECTION('ref_axis',(-1.,0.,0.)) ;
#94561=DIRECTION('center_axis',(0.,0.,1.)) ;
#94562=DIRECTION('ref_axis',(1.,0.,0.)) ;
#94563=DIRECTION('center_axis',(0.,0.,-1.)) ;
#94564=DIRECTION('ref_axis',(-1.,0.,0.)) ;
#94565=DIRECTION('center_axis',(-1.,0.,0.)) ;
#94566=DIRECTION('ref_axis',(0.,0.,1.)) ;
#94567=DIRECTION('center_axis',(0.,-1.,0.)) ;
#94568=DIRECTION('ref_axis',(0.,0.,-1.)) ;
#94569=DIRECTION('center_axis',(0.,1.,0.)) ;
#94570=DIRECTION('ref_axis',(0.,0.,1.)) ;
#94571=DIRECTION('center_axis',(0.,1.,-6.50521303491307E-15)) ;
#94572=DIRECTION('ref_axis',(0.,6.50521303491307E-15,1.)) ;
#94573=DIRECTION('center_axis',(0.,-1.,0.)) ;
#94574=DIRECTION('ref_axis',(0.,0.,-1.)) ;
#94575=DIRECTION('center_axis',(0.,-1.,0.)) ;
#94576=DIRECTION('ref_axis',(0.,0.,-1.)) ;
#94577=DIRECTION('center_axis',(0.,-1.,-1.07081696047951E-16)) ;
#94578=DIRECTION('ref_axis',(0.,1.07081696047951E-16,-1.)) ;
#94579=DIRECTION('center_axis',(0.,1.,0.)) ;
#94580=DIRECTION('ref_axis',(0.,0.,1.)) ;
#94581=DIRECTION('center_axis',(-1.,0.,0.)) ;
#94582=DIRECTION('ref_axis',(0.,0.,1.)) ;
#94583=DIRECTION('center_axis',(0.,0.,1.)) ;
#94584=DIRECTION('ref_axis',(1.,0.,0.)) ;
#94585=DIRECTION('center_axis',(0.,1.,0.)) ;
#94586=DIRECTION('ref_axis',(0.,0.,1.)) ;
#94587=DIRECTION('center_axis',(0.,0.,-1.)) ;
#94588=DIRECTION('ref_axis',(-1.,0.,0.)) ;
#94589=DIRECTION('center_axis',(0.,0.,1.)) ;
#94590=DIRECTION('ref_axis',(1.,0.,0.)) ;
#94591=DIRECTION('center_axis',(0.,0.,1.)) ;
#94592=DIRECTION('ref_axis',(1.,0.,0.)) ;
#94593=DIRECTION('center_axis',(0.,0.,1.)) ;
#94594=DIRECTION('ref_axis',(1.,0.,0.)) ;
#94595=DIRECTION('center_axis',(0.,0.,-1.)) ;
#94596=DIRECTION('ref_axis',(-1.,0.,0.)) ;
#94597=DIRECTION('center_axis',(0.,1.,0.)) ;
#94598=DIRECTION('ref_axis',(0.,0.,1.)) ;
#94599=DIRECTION('center_axis',(0.,-0.707106781186558,0.707106781186537)) ;
#94600=DIRECTION('ref_axis',(0.,-0.707106781186537,-0.707106781186558)) ;
#94601=DIRECTION('center_axis',(0.,1.,0.)) ;
#94602=DIRECTION('ref_axis',(0.,0.,1.)) ;
#94603=DIRECTION('center_axis',(0.,-0.514231796959093,-0.857651245551607)) ;
#94604=DIRECTION('ref_axis',(0.,0.857651245551607,-0.514231796959093)) ;
#94605=DIRECTION('center_axis',(0.,-0.707106781186548,0.707106781186547)) ;
#94606=DIRECTION('ref_axis',(0.,-0.707106781186547,-0.707106781186548)) ;
#94607=DIRECTION('center_axis',(0.,-0.707106781186548,0.707106781186548)) ;
#94608=DIRECTION('ref_axis',(0.,-0.707106781186548,-0.707106781186548)) ;
#94609=DIRECTION('center_axis',(-1.,0.,0.)) ;
#94610=DIRECTION('ref_axis',(0.,0.,1.)) ;
#94611=DIRECTION('center_axis',(0.,0.514231796959095,-0.857651245551606)) ;
#94612=DIRECTION('ref_axis',(0.,0.857651245551606,0.514231796959095)) ;
#94613=DIRECTION('center_axis',(0.,1.,0.)) ;
#94614=DIRECTION('ref_axis',(0.,0.,1.)) ;
#94615=DIRECTION('center_axis',(0.,0.,-1.)) ;
#94616=DIRECTION('ref_axis',(-1.,0.,0.)) ;
#94617=DIRECTION('center_axis',(0.,1.,0.)) ;
#94618=DIRECTION('ref_axis',(0.,0.,1.)) ;
#94619=DIRECTION('center_axis',(0.,0.,-1.)) ;
#94620=DIRECTION('ref_axis',(-1.,0.,0.)) ;
#94621=DIRECTION('center_axis',(0.,0.,-1.)) ;
#94622=DIRECTION('ref_axis',(-1.,0.,0.)) ;
#94623=DIRECTION('center_axis',(0.,0.,1.)) ;
#94624=DIRECTION('ref_axis',(1.,0.,0.)) ;
#94625=DIRECTION('center_axis',(0.,0.,-1.)) ;
#94626=DIRECTION('ref_axis',(-1.,0.,0.)) ;
#94627=DIRECTION('center_axis',(0.,1.,0.)) ;
#94628=DIRECTION('ref_axis',(0.,0.,1.)) ;
#94629=DIRECTION('center_axis',(0.,-1.,8.67361737988409E-15)) ;
#94630=DIRECTION('ref_axis',(0.,-8.67361737988409E-15,-1.)) ;
#94631=DIRECTION('center_axis',(0.,0.707106781186546,0.707106781186549)) ;
#94632=DIRECTION('ref_axis',(0.,-0.707106781186549,0.707106781186546)) ;
#94633=DIRECTION('center_axis',(0.,0.707106781186537,0.707106781186558)) ;
#94634=DIRECTION('ref_axis',(0.,-0.707106781186558,0.707106781186537)) ;
#94635=DIRECTION('center_axis',(0.,1.,1.07081696047951E-16)) ;
#94636=DIRECTION('ref_axis',(0.,-1.07081696047951E-16,1.)) ;
#94637=DIRECTION('center_axis',(0.,-1.,0.)) ;
#94638=DIRECTION('ref_axis',(0.,0.,-1.)) ;
#94639=DIRECTION('center_axis',(0.,1.,0.)) ;
#94640=DIRECTION('ref_axis',(0.,0.,1.)) ;
#94641=DIRECTION('center_axis',(0.,0.,1.)) ;
#94642=DIRECTION('ref_axis',(1.,0.,0.)) ;
#94643=DIRECTION('center_axis',(0.,1.,0.)) ;
#94644=DIRECTION('ref_axis',(0.,0.,1.)) ;
#94645=DIRECTION('center_axis',(0.,0.,1.)) ;
#94646=DIRECTION('ref_axis',(1.,0.,0.)) ;
#94647=DIRECTION('center_axis',(0.,3.99416362155027E-15,1.)) ;
#94648=DIRECTION('ref_axis',(0.,-1.,3.99416362155027E-15)) ;
#94649=DIRECTION('center_axis',(0.,0.,1.)) ;
#94650=DIRECTION('ref_axis',(1.,0.,0.)) ;
#94651=DIRECTION('center_axis',(0.,0.,-1.)) ;
#94652=DIRECTION('ref_axis',(-1.,0.,0.)) ;
#94653=DIRECTION('center_axis',(0.,0.,1.)) ;
#94654=DIRECTION('ref_axis',(1.,0.,0.)) ;
#94655=DIRECTION('center_axis',(-1.,0.,0.)) ;
#94656=DIRECTION('ref_axis',(0.,0.,1.)) ;
#94657=DIRECTION('center_axis',(0.,1.,0.)) ;
#94658=DIRECTION('ref_axis',(0.,0.,1.)) ;
#94659=DIRECTION('center_axis',(-1.,0.,0.)) ;
#94660=DIRECTION('ref_axis',(0.,0.,1.)) ;
#94661=DIRECTION('center_axis',(0.,-1.,0.)) ;
#94662=DIRECTION('ref_axis',(0.,0.,-1.)) ;
#94663=DIRECTION('center_axis',(0.,1.,0.)) ;
#94664=DIRECTION('ref_axis',(0.,0.,1.)) ;
#94665=DIRECTION('center_axis',(1.53063836115601E-16,-1.,-1.30104260698261E-16)) ;
#94666=DIRECTION('ref_axis',(1.,1.53063836115601E-16,1.99142572374599E-32)) ;
#94667=DIRECTION('center_axis',(0.,1.,0.)) ;
#94668=DIRECTION('ref_axis',(0.,0.,1.)) ;
#94669=DIRECTION('center_axis',(0.,-1.,0.)) ;
#94670=DIRECTION('ref_axis',(0.,0.,-1.)) ;
#94671=DIRECTION('center_axis',(1.,1.53063836115601E-16,2.73691106313441E-48)) ;
#94672=DIRECTION('ref_axis',(-1.53063836115601E-16,1.,-4.18922106430579E-64)) ;
#94673=DIRECTION('center_axis',(-1.,0.,0.)) ;
#94674=DIRECTION('ref_axis',(0.,0.,1.)) ;
#94675=DIRECTION('center_axis',(1.,1.53063836115601E-16,0.)) ;
#94676=DIRECTION('ref_axis',(1.53063836115601E-16,-1.,0.)) ;
#94677=DIRECTION('center_axis',(0.,1.,0.)) ;
#94678=DIRECTION('ref_axis',(1.,0.,0.)) ;
#94679=DIRECTION('center_axis',(0.,1.,0.)) ;
#94680=DIRECTION('ref_axis',(0.,0.,-1.)) ;
#94681=DIRECTION('center_axis',(0.,0.,1.)) ;
#94682=DIRECTION('ref_axis',(-1.,0.,0.)) ;
#94683=DIRECTION('center_axis',(0.,1.,0.)) ;
#94684=DIRECTION('ref_axis',(1.,0.,0.)) ;
#94685=DIRECTION('center_axis',(0.,0.,1.)) ;
#94686=DIRECTION('ref_axis',(-1.,0.,0.)) ;
#94687=DIRECTION('center_axis',(1.,1.0842021724855E-15,0.)) ;
#94688=DIRECTION('ref_axis',(1.0842021724855E-15,-1.,0.)) ;
#94689=DIRECTION('center_axis',(-1.,-1.53063836115601E-16,0.)) ;
#94690=DIRECTION('ref_axis',(0.,-1.,0.)) ;
#94691=DIRECTION('center_axis',(0.,0.,-1.)) ;
#94692=DIRECTION('ref_axis',(1.,0.,0.)) ;
#94693=DIRECTION('center_axis',(0.,0.,-1.)) ;
#94694=DIRECTION('ref_axis',(0.804034447892626,0.594582716366697,0.)) ;
#94695=DIRECTION('center_axis',(0.,0.,1.)) ;
#94696=DIRECTION('ref_axis',(1.,0.,0.)) ;
#94697=DIRECTION('',(0.,0.,-1.)) ;
#94698=DIRECTION('center_axis',(-2.16840434497101E-16,1.,1.30104260698261E-16)) ;
#94699=DIRECTION('ref_axis',(1.,2.16840434497101E-16,1.22464679914735E-16)) ;
#94700=DIRECTION('',(-2.16840434497101E-16,1.,1.30104260698261E-16)) ;
#94701=DIRECTION('center_axis',(0.,1.,0.)) ;
#94702=DIRECTION('ref_axis',(0.,0.,1.)) ;
#94703=DIRECTION('center_axis',(-1.,-1.53063836115601E-16,-2.73691106313441E-48)) ;
#94704=DIRECTION('ref_axis',(1.53063836115601E-16,-1.,4.18922106430579E-64)) ;
#94705=DIRECTION('center_axis',(1.,2.16840434497101E-16,0.)) ;
#94706=DIRECTION('ref_axis',(2.16840434497101E-16,-1.,0.)) ;
#94707=DIRECTION('center_axis',(0.,0.,1.)) ;
#94708=DIRECTION('ref_axis',(1.,0.,0.)) ;
#94709=DIRECTION('center_axis',(-1.25542992828747E-32,1.020425574104E-16,
1.)) ;
#94710=DIRECTION('ref_axis',(-1.28107280532009E-48,-1.,1.020425574104E-16)) ;
#94711=DIRECTION('center_axis',(0.,0.,1.)) ;
#94712=DIRECTION('ref_axis',(1.,0.,0.)) ;
#94713=DIRECTION('center_axis',(0.,0.,-1.)) ;
#94714=DIRECTION('ref_axis',(-1.,0.,0.)) ;
#94715=DIRECTION('center_axis',(1.,1.53063836115601E-16,-2.73691106313441E-48)) ;
#94716=DIRECTION('ref_axis',(-1.53063836115601E-16,1.,4.18922106430579E-64)) ;
#94717=DIRECTION('center_axis',(-1.,0.,0.)) ;
#94718=DIRECTION('ref_axis',(0.,0.,1.)) ;
#94719=DIRECTION('center_axis',(1.,1.53063836115601E-16,0.)) ;
#94720=DIRECTION('ref_axis',(1.53063836115601E-16,-1.,0.)) ;
#94721=DIRECTION('center_axis',(0.,1.,0.)) ;
#94722=DIRECTION('ref_axis',(1.,0.,0.)) ;
#94723=DIRECTION('center_axis',(-1.,-2.16840434497101E-16,0.)) ;
#94724=DIRECTION('ref_axis',(0.,-1.,0.)) ;
#94725=DIRECTION('center_axis',(0.,0.,-1.)) ;
#94726=DIRECTION('ref_axis',(1.,0.,0.)) ;
#94727=DIRECTION('center_axis',(-1.25542992828747E-32,1.020425574104E-16,
1.)) ;
#94728=DIRECTION('ref_axis',(0.,-1.,0.)) ;
#94729=DIRECTION('center_axis',(0.,-1.,0.)) ;
#94730=DIRECTION('ref_axis',(-6.50521303491307E-15,0.,1.)) ;
#94731=DIRECTION('center_axis',(-1.,0.,0.)) ;
#94732=DIRECTION('ref_axis',(0.,0.,-1.)) ;
#94733=DIRECTION('center_axis',(-1.,-1.53063836115601E-16,0.)) ;
#94734=DIRECTION('ref_axis',(0.,-1.,0.)) ;
#94735=DIRECTION('center_axis',(0.,-1.,0.)) ;
#94736=DIRECTION('ref_axis',(0.,0.,1.)) ;
#94737=DIRECTION('center_axis',(0.,0.,-1.)) ;
#94738=DIRECTION('ref_axis',(-1.,0.,0.)) ;
#94739=DIRECTION('center_axis',(0.,0.,-1.)) ;
#94740=DIRECTION('ref_axis',(-1.,0.,0.)) ;
#94741=DIRECTION('center_axis',(1.,1.53063836115601E-16,-3.06472600140763E-33)) ;
#94742=DIRECTION('ref_axis',(-1.53063836115601E-16,1.,4.69098718418678E-49)) ;
#94743=DIRECTION('center_axis',(-1.,0.,0.)) ;
#94744=DIRECTION('ref_axis',(0.,0.,1.)) ;
#94745=DIRECTION('center_axis',(-1.53063836115601E-16,1.,-1.020425574104E-16)) ;
#94746=DIRECTION('ref_axis',(-1.,-1.53063836115601E-16,1.3684555315672E-47)) ;
#94747=DIRECTION('',(1.53063836115601E-16,-1.,1.020425574104E-16)) ;
#94748=DIRECTION('center_axis',(0.,-1.,0.)) ;
#94749=DIRECTION('ref_axis',(0.,0.,-1.)) ;
#94750=DIRECTION('center_axis',(-1.53063836115601E-16,1.,-1.30104260698261E-16)) ;
#94751=DIRECTION('ref_axis',(-1.,-1.53063836115601E-16,1.99142572374599E-32)) ;
#94752=DIRECTION('center_axis',(0.,-1.,0.)) ;
#94753=DIRECTION('ref_axis',(0.,0.,-1.)) ;
#94754=DIRECTION('center_axis',(-1.,-1.53063836115601E-16,2.73691106313441E-48)) ;
#94755=DIRECTION('ref_axis',(1.53063836115601E-16,-1.,-4.18922106430579E-64)) ;
#94756=DIRECTION('center_axis',(1.,2.16840434497101E-16,0.)) ;
#94757=DIRECTION('ref_axis',(2.16840434497101E-16,-1.,0.)) ;
#94758=DIRECTION('center_axis',(-1.,0.,2.16840434497102E-15)) ;
#94759=DIRECTION('ref_axis',(2.16840434497102E-15,0.,1.)) ;
#94760=DIRECTION('center_axis',(-1.,-2.16840434497101E-16,0.)) ;
#94761=DIRECTION('ref_axis',(0.,-1.,0.)) ;
#94762=DIRECTION('center_axis',(0.,0.,1.)) ;
#94763=DIRECTION('ref_axis',(-1.,0.,0.)) ;
#94764=DIRECTION('center_axis',(0.,1.,0.)) ;
#94765=DIRECTION('ref_axis',(1.,0.,0.)) ;
#94766=DIRECTION('center_axis',(0.,1.,0.)) ;
#94767=DIRECTION('ref_axis',(0.,0.,-1.)) ;
#94768=DIRECTION('center_axis',(1.,0.,0.)) ;
#94769=DIRECTION('ref_axis',(0.,-1.,0.)) ;
#94770=DIRECTION('center_axis',(1.,6.50521303491304E-15,0.)) ;
#94771=DIRECTION('ref_axis',(-6.50521303491304E-15,1.,0.)) ;
#94772=DIRECTION('center_axis',(8.67361737988403E-15,1.,0.)) ;
#94773=DIRECTION('ref_axis',(-1.,8.67361737988403E-15,0.)) ;
#94774=DIRECTION('center_axis',(1.2303003375722E-16,-1.,1.020425574104E-16)) ;
#94775=DIRECTION('ref_axis',(1.,1.2303003375722E-16,-1.25542992828747E-32)) ;
#94776=DIRECTION('center_axis',(0.,1.,0.)) ;
#94777=DIRECTION('ref_axis',(0.,0.,1.)) ;
#94778=DIRECTION('center_axis',(0.,1.,0.)) ;
#94779=DIRECTION('ref_axis',(1.,0.,0.)) ;
#94780=DIRECTION('center_axis',(1.,1.2303003375722E-16,0.)) ;
#94781=DIRECTION('ref_axis',(1.2303003375722E-16,-1.,0.)) ;
#94782=DIRECTION('center_axis',(0.,0.,1.)) ;
#94783=DIRECTION('ref_axis',(-1.,0.,0.)) ;
#94784=DIRECTION('center_axis',(0.,1.,0.)) ;
#94785=DIRECTION('ref_axis',(1.,0.,0.)) ;
#94786=DIRECTION('center_axis',(0.,0.,-1.)) ;
#94787=DIRECTION('ref_axis',(1.,0.,0.)) ;
#94788=DIRECTION('center_axis',(0.,0.,-1.)) ;
#94789=DIRECTION('ref_axis',(-1.,0.,0.)) ;
#94790=DIRECTION('center_axis',(0.,0.,1.)) ;
#94791=DIRECTION('ref_axis',(1.,0.,0.)) ;
#94792=DIRECTION('center_axis',(-2.16840434497101E-16,1.,-1.020425574104E-16)) ;
#94793=DIRECTION('ref_axis',(-1.,-2.16840434497101E-16,5.47382212626882E-48)) ;
#94794=DIRECTION('center_axis',(0.,1.,0.)) ;
#94795=DIRECTION('ref_axis',(0.,0.,-1.)) ;
#94796=DIRECTION('center_axis',(1.,0.,1.25542992828747E-32)) ;
#94797=DIRECTION('ref_axis',(1.25542992828747E-32,0.,-1.)) ;
#94798=DIRECTION('center_axis',(1.,0.,0.)) ;
#94799=DIRECTION('ref_axis',(0.,0.,-1.)) ;
#94800=DIRECTION('center_axis',(-1.,-1.2303003375722E-16,0.)) ;
#94801=DIRECTION('ref_axis',(0.,-1.,0.)) ;
#94802=DIRECTION('center_axis',(0.,0.,-1.)) ;
#94803=DIRECTION('ref_axis',(1.,0.,0.)) ;
#94804=DIRECTION('center_axis',(0.,0.,-1.)) ;
#94805=DIRECTION('ref_axis',(-1.,0.,0.)) ;
#94806=DIRECTION('',(0.,0.,1.)) ;
#94807=DIRECTION('center_axis',(0.,0.,1.)) ;
#94808=DIRECTION('ref_axis',(1.,0.,0.)) ;
#94809=DIRECTION('center_axis',(0.,0.,1.)) ;
#94810=DIRECTION('ref_axis',(1.,0.,0.)) ;
#94811=DIRECTION('center_axis',(6.27714964143733E-33,-5.10212787052002E-17,
-1.)) ;
#94812=DIRECTION('ref_axis',(3.20268201330022E-49,1.,-5.10212787052002E-17)) ;
#94813=DIRECTION('center_axis',(1.,1.53063836115601E-16,-1.53236300070382E-33)) ;
#94814=DIRECTION('ref_axis',(-1.53063836115601E-16,1.,2.34549359209339E-49)) ;
#94815=DIRECTION('center_axis',(-1.,0.,0.)) ;
#94816=DIRECTION('ref_axis',(0.,0.,1.)) ;
#94817=DIRECTION('center_axis',(1.,0.,0.)) ;
#94818=DIRECTION('ref_axis',(0.,0.,-1.)) ;
#94819=DIRECTION('center_axis',(0.,1.,0.)) ;
#94820=DIRECTION('ref_axis',(1.,0.,0.)) ;
#94821=DIRECTION('center_axis',(-4.33680868994202E-15,1.,0.)) ;
#94822=DIRECTION('ref_axis',(1.,4.33680868994202E-15,0.)) ;
#94823=DIRECTION('center_axis',(0.,-1.,0.)) ;
#94824=DIRECTION('ref_axis',(0.,0.,-1.)) ;
#94825=DIRECTION('center_axis',(0.,0.,-1.)) ;
#94826=DIRECTION('ref_axis',(1.,0.,0.)) ;
#94827=DIRECTION('center_axis',(0.,0.,1.)) ;
#94828=DIRECTION('ref_axis',(1.,0.,0.)) ;
#94829=DIRECTION('center_axis',(0.,0.,-1.)) ;
#94830=DIRECTION('ref_axis',(-1.,0.,0.)) ;
#94831=DIRECTION('center_axis',(0.,1.,0.)) ;
#94832=DIRECTION('ref_axis',(1.,0.,0.)) ;
#94833=DIRECTION('center_axis',(1.,1.2303003375722E-16,0.)) ;
#94834=DIRECTION('ref_axis',(1.2303003375722E-16,-1.,0.)) ;
#94835=DIRECTION('center_axis',(0.,1.,0.)) ;
#94836=DIRECTION('ref_axis',(-6.50521303491307E-15,0.,-1.)) ;
#94837=DIRECTION('center_axis',(6.27714964143733E-33,-5.10212787052002E-17,
-1.)) ;
#94838=DIRECTION('ref_axis',(0.,1.,0.)) ;
#94839=DIRECTION('center_axis',(0.,-1.,0.)) ;
#94840=DIRECTION('ref_axis',(0.,0.,1.)) ;
#94841=DIRECTION('center_axis',(2.16840434497101E-16,-1.,5.10212787052002E-17)) ;
#94842=DIRECTION('ref_axis',(1.,2.16840434497101E-16,-5.47382212626882E-48)) ;
#94843=DIRECTION('center_axis',(0.,1.,0.)) ;
#94844=DIRECTION('ref_axis',(0.,0.,-1.)) ;
#94845=DIRECTION('center_axis',(0.,0.,1.)) ;
#94846=DIRECTION('ref_axis',(1.,0.,0.)) ;
#94847=DIRECTION('center_axis',(0.,0.,-1.)) ;
#94848=DIRECTION('ref_axis',(-1.,0.,0.)) ;
#94849=DIRECTION('center_axis',(-1.,-1.2303003375722E-16,0.)) ;
#94850=DIRECTION('ref_axis',(0.,-1.,0.)) ;
#94851=DIRECTION('center_axis',(0.,-1.,0.)) ;
#94852=DIRECTION('ref_axis',(0.,0.,1.)) ;
#94853=DIRECTION('center_axis',(1.53063836115601E-16,-1.,5.10212787052002E-17)) ;
#94854=DIRECTION('ref_axis',(1.,1.53063836115601E-16,-6.84227765783602E-48)) ;
#94855=DIRECTION('',(-1.53063836115601E-16,1.,-5.10212787052002E-17)) ;
#94856=DIRECTION('center_axis',(0.,-1.,0.)) ;
#94857=DIRECTION('ref_axis',(0.,0.,-1.)) ;
#94858=DIRECTION('center_axis',(-1.,0.,0.)) ;
#94859=DIRECTION('ref_axis',(0.,0.,-1.)) ;
#94860=DIRECTION('center_axis',(-1.2303003375722E-16,1.,-5.10212787052002E-17)) ;
#94861=DIRECTION('ref_axis',(-1.,-1.2303003375722E-16,6.27714964143733E-33)) ;
#94862=DIRECTION('center_axis',(-8.67361737988403E-15,-1.,0.)) ;
#94863=DIRECTION('ref_axis',(1.,-8.67361737988403E-15,0.)) ;
#94864=DIRECTION('center_axis',(1.,0.,6.27714964143733E-33)) ;
#94865=DIRECTION('ref_axis',(6.27714964143733E-33,0.,-1.)) ;
#94866=DIRECTION('center_axis',(-1.,0.,-6.50521303491307E-15)) ;
#94867=DIRECTION('ref_axis',(-6.50521303491307E-15,0.,1.)) ;
#94868=DIRECTION('center_axis',(1.,0.,0.)) ;
#94869=DIRECTION('ref_axis',(0.,1.,0.)) ;
#94870=DIRECTION('center_axis',(0.,0.,-1.)) ;
#94871=DIRECTION('ref_axis',(-1.,0.,0.)) ;
#94872=DIRECTION('center_axis',(0.,0.,1.)) ;
#94873=DIRECTION('ref_axis',(1.,0.,0.)) ;
#94874=DIRECTION('center_axis',(0.,0.,-1.)) ;
#94875=DIRECTION('ref_axis',(-1.,0.,0.)) ;
#94876=DIRECTION('center_axis',(-1.,0.,0.)) ;
#94877=DIRECTION('ref_axis',(0.,0.,1.)) ;
#94878=DIRECTION('center_axis',(0.,-1.,0.)) ;
#94879=DIRECTION('ref_axis',(0.,0.,-1.)) ;
#94880=DIRECTION('center_axis',(0.,1.,0.)) ;
#94881=DIRECTION('ref_axis',(0.,0.,1.)) ;
#94882=DIRECTION('center_axis',(0.,1.,-6.50521303491307E-15)) ;
#94883=DIRECTION('ref_axis',(0.,6.50521303491307E-15,1.)) ;
#94884=DIRECTION('center_axis',(0.,-1.,0.)) ;
#94885=DIRECTION('ref_axis',(0.,0.,-1.)) ;
#94886=DIRECTION('center_axis',(0.,-1.,0.)) ;
#94887=DIRECTION('ref_axis',(0.,0.,-1.)) ;
#94888=DIRECTION('center_axis',(0.,-1.,-1.07081696047951E-16)) ;
#94889=DIRECTION('ref_axis',(0.,1.07081696047951E-16,-1.)) ;
#94890=DIRECTION('center_axis',(0.,1.,0.)) ;
#94891=DIRECTION('ref_axis',(0.,0.,1.)) ;
#94892=DIRECTION('center_axis',(-1.,0.,0.)) ;
#94893=DIRECTION('ref_axis',(0.,0.,1.)) ;
#94894=DIRECTION('center_axis',(0.,0.,1.)) ;
#94895=DIRECTION('ref_axis',(1.,0.,0.)) ;
#94896=DIRECTION('center_axis',(0.,1.,0.)) ;
#94897=DIRECTION('ref_axis',(0.,0.,1.)) ;
#94898=DIRECTION('center_axis',(0.,0.,-1.)) ;
#94899=DIRECTION('ref_axis',(-1.,0.,0.)) ;
#94900=DIRECTION('center_axis',(0.,0.,1.)) ;
#94901=DIRECTION('ref_axis',(1.,0.,0.)) ;
#94902=DIRECTION('center_axis',(0.,0.,1.)) ;
#94903=DIRECTION('ref_axis',(1.,0.,0.)) ;
#94904=DIRECTION('center_axis',(0.,0.,1.)) ;
#94905=DIRECTION('ref_axis',(1.,0.,0.)) ;
#94906=DIRECTION('center_axis',(0.,0.,-1.)) ;
#94907=DIRECTION('ref_axis',(-1.,0.,0.)) ;
#94908=DIRECTION('center_axis',(0.,1.,0.)) ;
#94909=DIRECTION('ref_axis',(0.,0.,1.)) ;
#94910=DIRECTION('center_axis',(0.,-0.707106781186558,0.707106781186537)) ;
#94911=DIRECTION('ref_axis',(0.,-0.707106781186537,-0.707106781186558)) ;
#94912=DIRECTION('center_axis',(0.,1.,0.)) ;
#94913=DIRECTION('ref_axis',(0.,0.,1.)) ;
#94914=DIRECTION('center_axis',(0.,-0.514231796959093,-0.857651245551607)) ;
#94915=DIRECTION('ref_axis',(0.,0.857651245551607,-0.514231796959093)) ;
#94916=DIRECTION('center_axis',(0.,-0.707106781186548,0.707106781186547)) ;
#94917=DIRECTION('ref_axis',(0.,-0.707106781186547,-0.707106781186548)) ;
#94918=DIRECTION('center_axis',(0.,-0.707106781186548,0.707106781186548)) ;
#94919=DIRECTION('ref_axis',(0.,-0.707106781186548,-0.707106781186548)) ;
#94920=DIRECTION('center_axis',(-1.,0.,0.)) ;
#94921=DIRECTION('ref_axis',(0.,0.,1.)) ;
#94922=DIRECTION('center_axis',(0.,0.514231796959095,-0.857651245551606)) ;
#94923=DIRECTION('ref_axis',(0.,0.857651245551606,0.514231796959095)) ;
#94924=DIRECTION('center_axis',(0.,1.,0.)) ;
#94925=DIRECTION('ref_axis',(0.,0.,1.)) ;
#94926=DIRECTION('center_axis',(0.,0.,-1.)) ;
#94927=DIRECTION('ref_axis',(-1.,0.,0.)) ;
#94928=DIRECTION('center_axis',(0.,1.,0.)) ;
#94929=DIRECTION('ref_axis',(0.,0.,1.)) ;
#94930=DIRECTION('center_axis',(0.,0.,-1.)) ;
#94931=DIRECTION('ref_axis',(-1.,0.,0.)) ;
#94932=DIRECTION('center_axis',(0.,0.,-1.)) ;
#94933=DIRECTION('ref_axis',(-1.,0.,0.)) ;
#94934=DIRECTION('center_axis',(0.,0.,1.)) ;
#94935=DIRECTION('ref_axis',(1.,0.,0.)) ;
#94936=DIRECTION('center_axis',(0.,0.,-1.)) ;
#94937=DIRECTION('ref_axis',(-1.,0.,0.)) ;
#94938=DIRECTION('center_axis',(0.,1.,0.)) ;
#94939=DIRECTION('ref_axis',(0.,0.,1.)) ;
#94940=DIRECTION('center_axis',(0.,-1.,8.67361737988409E-15)) ;
#94941=DIRECTION('ref_axis',(0.,-8.67361737988409E-15,-1.)) ;
#94942=DIRECTION('center_axis',(0.,0.707106781186546,0.707106781186549)) ;
#94943=DIRECTION('ref_axis',(0.,-0.707106781186549,0.707106781186546)) ;
#94944=DIRECTION('center_axis',(0.,0.707106781186537,0.707106781186558)) ;
#94945=DIRECTION('ref_axis',(0.,-0.707106781186558,0.707106781186537)) ;
#94946=DIRECTION('center_axis',(0.,1.,1.07081696047951E-16)) ;
#94947=DIRECTION('ref_axis',(0.,-1.07081696047951E-16,1.)) ;
#94948=DIRECTION('center_axis',(0.,-1.,0.)) ;
#94949=DIRECTION('ref_axis',(0.,0.,-1.)) ;
#94950=DIRECTION('center_axis',(0.,1.,0.)) ;
#94951=DIRECTION('ref_axis',(0.,0.,1.)) ;
#94952=DIRECTION('center_axis',(0.,0.,1.)) ;
#94953=DIRECTION('ref_axis',(1.,0.,0.)) ;
#94954=DIRECTION('center_axis',(0.,1.,0.)) ;
#94955=DIRECTION('ref_axis',(0.,0.,1.)) ;
#94956=DIRECTION('center_axis',(0.,0.,1.)) ;
#94957=DIRECTION('ref_axis',(1.,0.,0.)) ;
#94958=DIRECTION('center_axis',(0.,3.99416362155027E-15,1.)) ;
#94959=DIRECTION('ref_axis',(0.,-1.,3.99416362155027E-15)) ;
#94960=DIRECTION('center_axis',(0.,0.,1.)) ;
#94961=DIRECTION('ref_axis',(1.,0.,0.)) ;
#94962=DIRECTION('center_axis',(0.,0.,-1.)) ;
#94963=DIRECTION('ref_axis',(-1.,0.,0.)) ;
#94964=DIRECTION('center_axis',(0.,0.,1.)) ;
#94965=DIRECTION('ref_axis',(1.,0.,0.)) ;
#94966=DIRECTION('center_axis',(-1.,0.,0.)) ;
#94967=DIRECTION('ref_axis',(0.,0.,1.)) ;
#94968=DIRECTION('center_axis',(0.,1.,0.)) ;
#94969=DIRECTION('ref_axis',(0.,0.,1.)) ;
#94970=DIRECTION('center_axis',(-1.,0.,0.)) ;
#94971=DIRECTION('ref_axis',(0.,0.,1.)) ;
#94972=DIRECTION('center_axis',(0.,-1.,0.)) ;
#94973=DIRECTION('ref_axis',(0.,0.,-1.)) ;
#94974=DIRECTION('center_axis',(0.,1.,0.)) ;
#94975=DIRECTION('ref_axis',(0.,0.,1.)) ;
#94976=DIRECTION('center_axis',(1.53063836115601E-16,-1.,-1.30104260698261E-16)) ;
#94977=DIRECTION('ref_axis',(1.,1.53063836115601E-16,1.99142572374599E-32)) ;
#94978=DIRECTION('center_axis',(0.,1.,0.)) ;
#94979=DIRECTION('ref_axis',(0.,0.,1.)) ;
#94980=DIRECTION('center_axis',(0.,-1.,0.)) ;
#94981=DIRECTION('ref_axis',(0.,0.,-1.)) ;
#94982=DIRECTION('center_axis',(1.,1.53063836115601E-16,2.73691106313441E-48)) ;
#94983=DIRECTION('ref_axis',(-1.53063836115601E-16,1.,-4.18922106430579E-64)) ;
#94984=DIRECTION('center_axis',(-1.,0.,0.)) ;
#94985=DIRECTION('ref_axis',(0.,0.,1.)) ;
#94986=DIRECTION('center_axis',(1.,1.53063836115601E-16,0.)) ;
#94987=DIRECTION('ref_axis',(1.53063836115601E-16,-1.,0.)) ;
#94988=DIRECTION('center_axis',(0.,1.,0.)) ;
#94989=DIRECTION('ref_axis',(1.,0.,0.)) ;
#94990=DIRECTION('center_axis',(0.,1.,0.)) ;
#94991=DIRECTION('ref_axis',(0.,0.,-1.)) ;
#94992=DIRECTION('center_axis',(0.,0.,1.)) ;
#94993=DIRECTION('ref_axis',(-1.,0.,0.)) ;
#94994=DIRECTION('center_axis',(0.,1.,0.)) ;
#94995=DIRECTION('ref_axis',(1.,0.,0.)) ;
#94996=DIRECTION('center_axis',(0.,0.,1.)) ;
#94997=DIRECTION('ref_axis',(-1.,0.,0.)) ;
#94998=DIRECTION('center_axis',(1.,1.0842021724855E-15,0.)) ;
#94999=DIRECTION('ref_axis',(1.0842021724855E-15,-1.,0.)) ;
#95000=DIRECTION('center_axis',(-1.,-1.53063836115601E-16,0.)) ;
#95001=DIRECTION('ref_axis',(0.,-1.,0.)) ;
#95002=DIRECTION('center_axis',(0.,0.,-1.)) ;
#95003=DIRECTION('ref_axis',(1.,0.,0.)) ;
#95004=DIRECTION('center_axis',(0.,0.,-1.)) ;
#95005=DIRECTION('ref_axis',(0.804034447892627,0.594582716366695,0.)) ;
#95006=DIRECTION('center_axis',(0.,0.,1.)) ;
#95007=DIRECTION('ref_axis',(1.,0.,0.)) ;
#95008=DIRECTION('',(0.,0.,-1.)) ;
#95009=DIRECTION('center_axis',(-2.16840434497101E-16,1.,1.30104260698261E-16)) ;
#95010=DIRECTION('ref_axis',(1.,2.16840434497101E-16,1.22464679914735E-16)) ;
#95011=DIRECTION('',(-2.16840434497101E-16,1.,1.30104260698261E-16)) ;
#95012=DIRECTION('center_axis',(0.,1.,0.)) ;
#95013=DIRECTION('ref_axis',(0.,0.,1.)) ;
#95014=DIRECTION('center_axis',(-1.,-1.53063836115601E-16,-2.73691106313441E-48)) ;
#95015=DIRECTION('ref_axis',(1.53063836115601E-16,-1.,4.18922106430579E-64)) ;
#95016=DIRECTION('center_axis',(1.,2.16840434497101E-16,0.)) ;
#95017=DIRECTION('ref_axis',(2.16840434497101E-16,-1.,0.)) ;
#95018=DIRECTION('center_axis',(0.,0.,1.)) ;
#95019=DIRECTION('ref_axis',(1.,0.,0.)) ;
#95020=DIRECTION('center_axis',(-1.25542992828747E-32,1.020425574104E-16,
1.)) ;
#95021=DIRECTION('ref_axis',(-1.28107280532009E-48,-1.,1.020425574104E-16)) ;
#95022=DIRECTION('center_axis',(0.,0.,1.)) ;
#95023=DIRECTION('ref_axis',(1.,0.,0.)) ;
#95024=DIRECTION('center_axis',(0.,0.,-1.)) ;
#95025=DIRECTION('ref_axis',(-1.,0.,0.)) ;
#95026=DIRECTION('center_axis',(1.,1.53063836115601E-16,-2.73691106313441E-48)) ;
#95027=DIRECTION('ref_axis',(-1.53063836115601E-16,1.,4.18922106430579E-64)) ;
#95028=DIRECTION('center_axis',(-1.,0.,0.)) ;
#95029=DIRECTION('ref_axis',(0.,0.,1.)) ;
#95030=DIRECTION('center_axis',(1.,1.53063836115601E-16,0.)) ;
#95031=DIRECTION('ref_axis',(1.53063836115601E-16,-1.,0.)) ;
#95032=DIRECTION('center_axis',(0.,1.,0.)) ;
#95033=DIRECTION('ref_axis',(1.,0.,0.)) ;
#95034=DIRECTION('center_axis',(-1.,-2.16840434497101E-16,0.)) ;
#95035=DIRECTION('ref_axis',(0.,-1.,0.)) ;
#95036=DIRECTION('center_axis',(0.,0.,-1.)) ;
#95037=DIRECTION('ref_axis',(1.,0.,0.)) ;
#95038=DIRECTION('center_axis',(-1.25542992828747E-32,1.020425574104E-16,
1.)) ;
#95039=DIRECTION('ref_axis',(0.,-1.,0.)) ;
#95040=DIRECTION('center_axis',(0.,-1.,0.)) ;
#95041=DIRECTION('ref_axis',(-6.50521303491307E-15,0.,1.)) ;
#95042=DIRECTION('center_axis',(-1.,0.,0.)) ;
#95043=DIRECTION('ref_axis',(0.,0.,-1.)) ;
#95044=DIRECTION('center_axis',(-1.,-1.53063836115601E-16,0.)) ;
#95045=DIRECTION('ref_axis',(0.,-1.,0.)) ;
#95046=DIRECTION('center_axis',(0.,-1.,0.)) ;
#95047=DIRECTION('ref_axis',(0.,0.,1.)) ;
#95048=DIRECTION('center_axis',(0.,0.,-1.)) ;
#95049=DIRECTION('ref_axis',(-1.,0.,0.)) ;
#95050=DIRECTION('center_axis',(0.,0.,-1.)) ;
#95051=DIRECTION('ref_axis',(-1.,0.,0.)) ;
#95052=DIRECTION('center_axis',(1.,1.53063836115601E-16,-3.06472600140763E-33)) ;
#95053=DIRECTION('ref_axis',(-1.53063836115601E-16,1.,4.69098718418678E-49)) ;
#95054=DIRECTION('center_axis',(-1.,0.,0.)) ;
#95055=DIRECTION('ref_axis',(0.,0.,1.)) ;
#95056=DIRECTION('center_axis',(-1.53063836115601E-16,1.,-1.020425574104E-16)) ;
#95057=DIRECTION('ref_axis',(-1.,-1.53063836115601E-16,1.3684555315672E-47)) ;
#95058=DIRECTION('',(1.53063836115601E-16,-1.,1.020425574104E-16)) ;
#95059=DIRECTION('center_axis',(0.,-1.,0.)) ;
#95060=DIRECTION('ref_axis',(0.,0.,-1.)) ;
#95061=DIRECTION('center_axis',(-1.53063836115601E-16,1.,-1.30104260698261E-16)) ;
#95062=DIRECTION('ref_axis',(-1.,-1.53063836115601E-16,1.99142572374599E-32)) ;
#95063=DIRECTION('center_axis',(0.,-1.,0.)) ;
#95064=DIRECTION('ref_axis',(0.,0.,-1.)) ;
#95065=DIRECTION('center_axis',(-1.,-1.53063836115601E-16,2.73691106313441E-48)) ;
#95066=DIRECTION('ref_axis',(1.53063836115601E-16,-1.,-4.18922106430579E-64)) ;
#95067=DIRECTION('center_axis',(1.,2.16840434497101E-16,0.)) ;
#95068=DIRECTION('ref_axis',(2.16840434497101E-16,-1.,0.)) ;
#95069=DIRECTION('center_axis',(-1.,0.,2.16840434497102E-15)) ;
#95070=DIRECTION('ref_axis',(2.16840434497102E-15,0.,1.)) ;
#95071=DIRECTION('center_axis',(-1.,-2.16840434497101E-16,0.)) ;
#95072=DIRECTION('ref_axis',(0.,-1.,0.)) ;
#95073=DIRECTION('center_axis',(0.,0.,1.)) ;
#95074=DIRECTION('ref_axis',(-1.,0.,0.)) ;
#95075=DIRECTION('center_axis',(0.,1.,0.)) ;
#95076=DIRECTION('ref_axis',(1.,0.,0.)) ;
#95077=DIRECTION('center_axis',(0.,1.,0.)) ;
#95078=DIRECTION('ref_axis',(0.,0.,-1.)) ;
#95079=DIRECTION('center_axis',(1.,0.,0.)) ;
#95080=DIRECTION('ref_axis',(0.,-1.,0.)) ;
#95081=DIRECTION('center_axis',(1.,6.50521303491304E-15,0.)) ;
#95082=DIRECTION('ref_axis',(-6.50521303491304E-15,1.,0.)) ;
#95083=DIRECTION('center_axis',(8.67361737988403E-15,1.,0.)) ;
#95084=DIRECTION('ref_axis',(-1.,8.67361737988403E-15,0.)) ;
#95085=DIRECTION('center_axis',(1.2303003375722E-16,-1.,1.020425574104E-16)) ;
#95086=DIRECTION('ref_axis',(1.,1.2303003375722E-16,-1.25542992828747E-32)) ;
#95087=DIRECTION('center_axis',(0.,1.,0.)) ;
#95088=DIRECTION('ref_axis',(0.,0.,1.)) ;
#95089=DIRECTION('center_axis',(0.,1.,0.)) ;
#95090=DIRECTION('ref_axis',(1.,0.,0.)) ;
#95091=DIRECTION('center_axis',(1.,1.2303003375722E-16,0.)) ;
#95092=DIRECTION('ref_axis',(1.2303003375722E-16,-1.,0.)) ;
#95093=DIRECTION('center_axis',(0.,0.,1.)) ;
#95094=DIRECTION('ref_axis',(-1.,0.,0.)) ;
#95095=DIRECTION('center_axis',(0.,1.,0.)) ;
#95096=DIRECTION('ref_axis',(1.,0.,0.)) ;
#95097=DIRECTION('center_axis',(0.,0.,-1.)) ;
#95098=DIRECTION('ref_axis',(1.,0.,0.)) ;
#95099=DIRECTION('center_axis',(0.,0.,-1.)) ;
#95100=DIRECTION('ref_axis',(-1.,0.,0.)) ;
#95101=DIRECTION('center_axis',(0.,0.,1.)) ;
#95102=DIRECTION('ref_axis',(1.,0.,0.)) ;
#95103=DIRECTION('center_axis',(-2.16840434497101E-16,1.,-1.020425574104E-16)) ;
#95104=DIRECTION('ref_axis',(-1.,-2.16840434497101E-16,5.47382212626882E-48)) ;
#95105=DIRECTION('center_axis',(0.,1.,0.)) ;
#95106=DIRECTION('ref_axis',(0.,0.,-1.)) ;
#95107=DIRECTION('center_axis',(1.,0.,1.25542992828747E-32)) ;
#95108=DIRECTION('ref_axis',(1.25542992828747E-32,0.,-1.)) ;
#95109=DIRECTION('center_axis',(1.,0.,0.)) ;
#95110=DIRECTION('ref_axis',(0.,0.,-1.)) ;
#95111=DIRECTION('center_axis',(-1.,-1.2303003375722E-16,0.)) ;
#95112=DIRECTION('ref_axis',(0.,-1.,0.)) ;
#95113=DIRECTION('center_axis',(0.,0.,-1.)) ;
#95114=DIRECTION('ref_axis',(1.,0.,0.)) ;
#95115=DIRECTION('center_axis',(0.,0.,-1.)) ;
#95116=DIRECTION('ref_axis',(-1.,0.,0.)) ;
#95117=DIRECTION('',(0.,0.,1.)) ;
#95118=DIRECTION('center_axis',(0.,0.,1.)) ;
#95119=DIRECTION('ref_axis',(1.,0.,0.)) ;
#95120=DIRECTION('center_axis',(0.,0.,1.)) ;
#95121=DIRECTION('ref_axis',(1.,0.,0.)) ;
#95122=DIRECTION('center_axis',(6.27714964143733E-33,-5.10212787052002E-17,
-1.)) ;
#95123=DIRECTION('ref_axis',(3.20268201330022E-49,1.,-5.10212787052002E-17)) ;
#95124=DIRECTION('center_axis',(1.,1.53063836115601E-16,-1.53236300070382E-33)) ;
#95125=DIRECTION('ref_axis',(-1.53063836115601E-16,1.,2.34549359209339E-49)) ;
#95126=DIRECTION('center_axis',(-1.,0.,0.)) ;
#95127=DIRECTION('ref_axis',(0.,0.,1.)) ;
#95128=DIRECTION('center_axis',(1.,0.,0.)) ;
#95129=DIRECTION('ref_axis',(0.,0.,-1.)) ;
#95130=DIRECTION('center_axis',(0.,1.,0.)) ;
#95131=DIRECTION('ref_axis',(1.,0.,0.)) ;
#95132=DIRECTION('center_axis',(-4.33680868994202E-15,1.,0.)) ;
#95133=DIRECTION('ref_axis',(1.,4.33680868994202E-15,0.)) ;
#95134=DIRECTION('center_axis',(0.,-1.,0.)) ;
#95135=DIRECTION('ref_axis',(0.,0.,-1.)) ;
#95136=DIRECTION('center_axis',(0.,0.,-1.)) ;
#95137=DIRECTION('ref_axis',(1.,0.,0.)) ;
#95138=DIRECTION('center_axis',(0.,0.,1.)) ;
#95139=DIRECTION('ref_axis',(1.,0.,0.)) ;
#95140=DIRECTION('center_axis',(0.,0.,-1.)) ;
#95141=DIRECTION('ref_axis',(-1.,0.,0.)) ;
#95142=DIRECTION('center_axis',(0.,1.,0.)) ;
#95143=DIRECTION('ref_axis',(1.,0.,0.)) ;
#95144=DIRECTION('center_axis',(1.,1.2303003375722E-16,0.)) ;
#95145=DIRECTION('ref_axis',(1.2303003375722E-16,-1.,0.)) ;
#95146=DIRECTION('center_axis',(0.,1.,0.)) ;
#95147=DIRECTION('ref_axis',(-6.50521303491284E-15,0.,-1.)) ;
#95148=DIRECTION('center_axis',(6.27714964143733E-33,-5.10212787052002E-17,
-1.)) ;
#95149=DIRECTION('ref_axis',(0.,1.,0.)) ;
#95150=DIRECTION('center_axis',(0.,-1.,0.)) ;
#95151=DIRECTION('ref_axis',(0.,0.,1.)) ;
#95152=DIRECTION('center_axis',(2.16840434497101E-16,-1.,5.10212787052002E-17)) ;
#95153=DIRECTION('ref_axis',(1.,2.16840434497101E-16,-5.47382212626882E-48)) ;
#95154=DIRECTION('center_axis',(0.,1.,0.)) ;
#95155=DIRECTION('ref_axis',(0.,0.,-1.)) ;
#95156=DIRECTION('center_axis',(0.,0.,1.)) ;
#95157=DIRECTION('ref_axis',(1.,0.,0.)) ;
#95158=DIRECTION('center_axis',(0.,0.,-1.)) ;
#95159=DIRECTION('ref_axis',(-1.,0.,0.)) ;
#95160=DIRECTION('center_axis',(-1.,-1.2303003375722E-16,0.)) ;
#95161=DIRECTION('ref_axis',(0.,-1.,0.)) ;
#95162=DIRECTION('center_axis',(0.,-1.,0.)) ;
#95163=DIRECTION('ref_axis',(0.,0.,1.)) ;
#95164=DIRECTION('center_axis',(1.53063836115601E-16,-1.,5.10212787052002E-17)) ;
#95165=DIRECTION('ref_axis',(1.,1.53063836115601E-16,-6.84227765783602E-48)) ;
#95166=DIRECTION('',(-1.53063836115601E-16,1.,-5.10212787052002E-17)) ;
#95167=DIRECTION('center_axis',(0.,-1.,0.)) ;
#95168=DIRECTION('ref_axis',(0.,0.,-1.)) ;
#95169=DIRECTION('center_axis',(-1.,0.,0.)) ;
#95170=DIRECTION('ref_axis',(0.,0.,-1.)) ;
#95171=DIRECTION('center_axis',(-1.2303003375722E-16,1.,-5.10212787052002E-17)) ;
#95172=DIRECTION('ref_axis',(-1.,-1.2303003375722E-16,6.27714964143733E-33)) ;
#95173=DIRECTION('center_axis',(-8.67361737988403E-15,-1.,0.)) ;
#95174=DIRECTION('ref_axis',(1.,-8.67361737988403E-15,0.)) ;
#95175=DIRECTION('center_axis',(1.,0.,6.27714964143733E-33)) ;
#95176=DIRECTION('ref_axis',(6.27714964143733E-33,0.,-1.)) ;
#95177=DIRECTION('center_axis',(-1.,0.,-6.50521303491284E-15)) ;
#95178=DIRECTION('ref_axis',(-6.50521303491284E-15,0.,1.)) ;
#95179=DIRECTION('center_axis',(1.,0.,0.)) ;
#95180=DIRECTION('ref_axis',(0.,1.,0.)) ;
#95181=DIRECTION('center_axis',(0.,0.,-1.)) ;
#95182=DIRECTION('ref_axis',(-1.,0.,0.)) ;
#95183=DIRECTION('center_axis',(0.,0.,1.)) ;
#95184=DIRECTION('ref_axis',(1.,0.,0.)) ;
#95185=DIRECTION('center_axis',(0.,0.,-1.)) ;
#95186=DIRECTION('ref_axis',(-1.,0.,0.)) ;
#95187=DIRECTION('center_axis',(-1.,0.,0.)) ;
#95188=DIRECTION('ref_axis',(0.,0.,1.)) ;
#95189=DIRECTION('center_axis',(0.,-1.,0.)) ;
#95190=DIRECTION('ref_axis',(0.,0.,-1.)) ;
#95191=DIRECTION('center_axis',(0.,1.,0.)) ;
#95192=DIRECTION('ref_axis',(0.,0.,1.)) ;
#95193=DIRECTION('center_axis',(0.,1.,-6.50521303491284E-15)) ;
#95194=DIRECTION('ref_axis',(0.,6.50521303491284E-15,1.)) ;
#95195=DIRECTION('center_axis',(0.,-1.,0.)) ;
#95196=DIRECTION('ref_axis',(0.,0.,-1.)) ;
#95197=DIRECTION('center_axis',(0.,-1.,0.)) ;
#95198=DIRECTION('ref_axis',(0.,0.,-1.)) ;
#95199=DIRECTION('center_axis',(0.,-1.,-1.07081696047951E-16)) ;
#95200=DIRECTION('ref_axis',(0.,1.07081696047951E-16,-1.)) ;
#95201=DIRECTION('center_axis',(0.,1.,0.)) ;
#95202=DIRECTION('ref_axis',(0.,0.,1.)) ;
#95203=DIRECTION('center_axis',(-1.,0.,0.)) ;
#95204=DIRECTION('ref_axis',(0.,0.,1.)) ;
#95205=DIRECTION('center_axis',(0.,0.,1.)) ;
#95206=DIRECTION('ref_axis',(1.,0.,0.)) ;
#95207=DIRECTION('center_axis',(0.,1.,0.)) ;
#95208=DIRECTION('ref_axis',(0.,0.,1.)) ;
#95209=DIRECTION('center_axis',(0.,0.,-1.)) ;
#95210=DIRECTION('ref_axis',(-1.,0.,0.)) ;
#95211=DIRECTION('center_axis',(0.,0.,1.)) ;
#95212=DIRECTION('ref_axis',(1.,0.,0.)) ;
#95213=DIRECTION('center_axis',(0.,0.,1.)) ;
#95214=DIRECTION('ref_axis',(1.,0.,0.)) ;
#95215=DIRECTION('center_axis',(0.,0.,1.)) ;
#95216=DIRECTION('ref_axis',(1.,0.,0.)) ;
#95217=DIRECTION('center_axis',(0.,0.,-1.)) ;
#95218=DIRECTION('ref_axis',(-1.,0.,0.)) ;
#95219=DIRECTION('center_axis',(0.,1.,0.)) ;
#95220=DIRECTION('ref_axis',(0.,0.,1.)) ;
#95221=DIRECTION('center_axis',(0.,-0.707106781186532,0.707106781186563)) ;
#95222=DIRECTION('ref_axis',(0.,-0.707106781186563,-0.707106781186532)) ;
#95223=DIRECTION('center_axis',(0.,1.,0.)) ;
#95224=DIRECTION('ref_axis',(0.,0.,1.)) ;
#95225=DIRECTION('center_axis',(2.23012492569655E-15,-0.51423179695906,
-0.857651245551627)) ;
#95226=DIRECTION('ref_axis',(2.6714619735869E-30,0.857651245551626,-0.51423179695906)) ;
#95227=DIRECTION('center_axis',(0.,-0.707106781186548,0.707106781186547)) ;
#95228=DIRECTION('ref_axis',(0.,-0.707106781186547,-0.707106781186548)) ;
#95229=DIRECTION('center_axis',(0.,-0.707106781186541,0.707106781186554)) ;
#95230=DIRECTION('ref_axis',(0.,-0.707106781186554,-0.707106781186541)) ;
#95231=DIRECTION('center_axis',(-1.,0.,0.)) ;
#95232=DIRECTION('ref_axis',(0.,0.,1.)) ;
#95233=DIRECTION('center_axis',(0.,0.514231796959095,-0.857651245551606)) ;
#95234=DIRECTION('ref_axis',(0.,0.857651245551606,0.514231796959095)) ;
#95235=DIRECTION('center_axis',(0.,1.,0.)) ;
#95236=DIRECTION('ref_axis',(0.,0.,1.)) ;
#95237=DIRECTION('center_axis',(0.,0.,-1.)) ;
#95238=DIRECTION('ref_axis',(-1.,0.,0.)) ;
#95239=DIRECTION('center_axis',(0.,1.,0.)) ;
#95240=DIRECTION('ref_axis',(0.,0.,1.)) ;
#95241=DIRECTION('center_axis',(0.,0.,-1.)) ;
#95242=DIRECTION('ref_axis',(-1.,0.,0.)) ;
#95243=DIRECTION('center_axis',(0.,0.,-1.)) ;
#95244=DIRECTION('ref_axis',(-1.,0.,0.)) ;
#95245=DIRECTION('center_axis',(0.,0.,1.)) ;
#95246=DIRECTION('ref_axis',(1.,0.,0.)) ;
#95247=DIRECTION('center_axis',(0.,0.,-1.)) ;
#95248=DIRECTION('ref_axis',(-1.,0.,0.)) ;
#95249=DIRECTION('center_axis',(0.,1.,0.)) ;
#95250=DIRECTION('ref_axis',(0.,0.,1.)) ;
#95251=DIRECTION('center_axis',(0.,-1.,8.67361737988409E-15)) ;
#95252=DIRECTION('ref_axis',(0.,-8.67361737988409E-15,-1.)) ;
#95253=DIRECTION('center_axis',(0.,0.707106781186546,0.707106781186549)) ;
#95254=DIRECTION('ref_axis',(0.,-0.707106781186549,0.707106781186546)) ;
#95255=DIRECTION('center_axis',(0.,0.707106781186537,0.707106781186558)) ;
#95256=DIRECTION('ref_axis',(0.,-0.707106781186558,0.707106781186537)) ;
#95257=DIRECTION('center_axis',(0.,1.,1.07081696047951E-16)) ;
#95258=DIRECTION('ref_axis',(0.,-1.07081696047951E-16,1.)) ;
#95259=DIRECTION('center_axis',(0.,-1.,0.)) ;
#95260=DIRECTION('ref_axis',(0.,0.,-1.)) ;
#95261=DIRECTION('center_axis',(0.,1.,0.)) ;
#95262=DIRECTION('ref_axis',(0.,0.,1.)) ;
#95263=DIRECTION('center_axis',(0.,0.,1.)) ;
#95264=DIRECTION('ref_axis',(1.,0.,0.)) ;
#95265=DIRECTION('center_axis',(0.,1.,0.)) ;
#95266=DIRECTION('ref_axis',(0.,0.,1.)) ;
#95267=DIRECTION('center_axis',(0.,0.,1.)) ;
#95268=DIRECTION('ref_axis',(1.,0.,0.)) ;
#95269=DIRECTION('center_axis',(0.,3.99416362155027E-15,1.)) ;
#95270=DIRECTION('ref_axis',(0.,-1.,3.99416362155027E-15)) ;
#95271=DIRECTION('center_axis',(0.,0.,1.)) ;
#95272=DIRECTION('ref_axis',(1.,0.,0.)) ;
#95273=DIRECTION('center_axis',(0.,0.,-1.)) ;
#95274=DIRECTION('ref_axis',(-1.,0.,0.)) ;
#95275=DIRECTION('center_axis',(0.,0.,1.)) ;
#95276=DIRECTION('ref_axis',(1.,0.,0.)) ;
#95277=DIRECTION('center_axis',(-1.,0.,0.)) ;
#95278=DIRECTION('ref_axis',(0.,0.,1.)) ;
#95279=DIRECTION('center_axis',(0.,1.,0.)) ;
#95280=DIRECTION('ref_axis',(0.,0.,1.)) ;
#95281=DIRECTION('center_axis',(-1.,0.,0.)) ;
#95282=DIRECTION('ref_axis',(0.,0.,1.)) ;
#95283=DIRECTION('center_axis',(0.,-1.,0.)) ;
#95284=DIRECTION('ref_axis',(0.,0.,-1.)) ;
#95285=DIRECTION('center_axis',(0.,1.,0.)) ;
#95286=DIRECTION('ref_axis',(0.,0.,1.)) ;
#95287=DIRECTION('center_axis',(1.53063836115601E-16,-1.,-1.30104260698261E-16)) ;
#95288=DIRECTION('ref_axis',(1.,1.53063836115601E-16,1.99142572374599E-32)) ;
#95289=DIRECTION('center_axis',(0.,1.,0.)) ;
#95290=DIRECTION('ref_axis',(0.,0.,1.)) ;
#95291=DIRECTION('center_axis',(0.,-1.,0.)) ;
#95292=DIRECTION('ref_axis',(0.,0.,-1.)) ;
#95293=DIRECTION('center_axis',(1.,1.53063836115601E-16,2.73691106313441E-48)) ;
#95294=DIRECTION('ref_axis',(-1.53063836115601E-16,1.,-4.18922106430579E-64)) ;
#95295=DIRECTION('center_axis',(-1.,0.,0.)) ;
#95296=DIRECTION('ref_axis',(0.,0.,1.)) ;
#95297=DIRECTION('center_axis',(1.,1.53063836115601E-16,0.)) ;
#95298=DIRECTION('ref_axis',(1.53063836115601E-16,-1.,0.)) ;
#95299=DIRECTION('center_axis',(0.,1.,0.)) ;
#95300=DIRECTION('ref_axis',(1.,0.,0.)) ;
#95301=DIRECTION('center_axis',(0.,1.,0.)) ;
#95302=DIRECTION('ref_axis',(0.,0.,-1.)) ;
#95303=DIRECTION('center_axis',(0.,0.,1.)) ;
#95304=DIRECTION('ref_axis',(-1.,0.,0.)) ;
#95305=DIRECTION('center_axis',(0.,1.,0.)) ;
#95306=DIRECTION('ref_axis',(1.,0.,0.)) ;
#95307=DIRECTION('center_axis',(0.,0.,1.)) ;
#95308=DIRECTION('ref_axis',(-1.,0.,0.)) ;
#95309=DIRECTION('center_axis',(1.,1.0842021724855E-15,0.)) ;
#95310=DIRECTION('ref_axis',(1.0842021724855E-15,-1.,0.)) ;
#95311=DIRECTION('center_axis',(-1.,-1.53063836115601E-16,0.)) ;
#95312=DIRECTION('ref_axis',(0.,-1.,0.)) ;
#95313=DIRECTION('center_axis',(0.,0.,-1.)) ;
#95314=DIRECTION('ref_axis',(1.,0.,0.)) ;
#95315=DIRECTION('center_axis',(0.,0.,-1.)) ;
#95316=DIRECTION('ref_axis',(0.804034447892622,0.594582716366703,0.)) ;
#95317=DIRECTION('center_axis',(0.,0.,1.)) ;
#95318=DIRECTION('ref_axis',(1.,0.,0.)) ;
#95319=DIRECTION('',(0.,0.,-1.)) ;
#95320=DIRECTION('center_axis',(-2.16840434497101E-16,1.,1.30104260698261E-16)) ;
#95321=DIRECTION('ref_axis',(1.,2.16840434497101E-16,1.22464679914735E-16)) ;
#95322=DIRECTION('',(-2.16840434497101E-16,1.,1.30104260698261E-16)) ;
#95323=DIRECTION('center_axis',(0.,1.,0.)) ;
#95324=DIRECTION('ref_axis',(0.,0.,1.)) ;
#95325=DIRECTION('center_axis',(-1.,-1.53063836115601E-16,-2.73691106313441E-48)) ;
#95326=DIRECTION('ref_axis',(1.53063836115601E-16,-1.,4.18922106430579E-64)) ;
#95327=DIRECTION('center_axis',(1.,2.16840434497101E-16,0.)) ;
#95328=DIRECTION('ref_axis',(2.16840434497101E-16,-1.,0.)) ;
#95329=DIRECTION('center_axis',(0.,0.,1.)) ;
#95330=DIRECTION('ref_axis',(1.,0.,0.)) ;
#95331=DIRECTION('center_axis',(-1.25542992828747E-32,1.020425574104E-16,
1.)) ;
#95332=DIRECTION('ref_axis',(-1.28107280532009E-48,-1.,1.020425574104E-16)) ;
#95333=DIRECTION('center_axis',(0.,0.,1.)) ;
#95334=DIRECTION('ref_axis',(1.,0.,0.)) ;
#95335=DIRECTION('center_axis',(0.,0.,-1.)) ;
#95336=DIRECTION('ref_axis',(-1.,0.,0.)) ;
#95337=DIRECTION('center_axis',(1.,1.53063836115601E-16,-2.73691106313441E-48)) ;
#95338=DIRECTION('ref_axis',(-1.53063836115601E-16,1.,4.18922106430579E-64)) ;
#95339=DIRECTION('center_axis',(-1.,0.,0.)) ;
#95340=DIRECTION('ref_axis',(0.,0.,1.)) ;
#95341=DIRECTION('center_axis',(1.,1.53063836115601E-16,0.)) ;
#95342=DIRECTION('ref_axis',(1.53063836115601E-16,-1.,0.)) ;
#95343=DIRECTION('center_axis',(0.,1.,0.)) ;
#95344=DIRECTION('ref_axis',(1.,0.,0.)) ;
#95345=DIRECTION('center_axis',(-1.,-2.16840434497101E-16,0.)) ;
#95346=DIRECTION('ref_axis',(0.,-1.,0.)) ;
#95347=DIRECTION('center_axis',(0.,0.,-1.)) ;
#95348=DIRECTION('ref_axis',(1.,0.,0.)) ;
#95349=DIRECTION('center_axis',(-1.25542992828747E-32,1.020425574104E-16,
1.)) ;
#95350=DIRECTION('ref_axis',(0.,-1.,0.)) ;
#95351=DIRECTION('center_axis',(0.,-1.,0.)) ;
#95352=DIRECTION('ref_axis',(-6.50521303491284E-15,0.,1.)) ;
#95353=DIRECTION('center_axis',(-1.,0.,0.)) ;
#95354=DIRECTION('ref_axis',(0.,0.,-1.)) ;
#95355=DIRECTION('center_axis',(-1.,-1.53063836115601E-16,0.)) ;
#95356=DIRECTION('ref_axis',(0.,-1.,0.)) ;
#95357=DIRECTION('center_axis',(0.,-1.,0.)) ;
#95358=DIRECTION('ref_axis',(0.,0.,1.)) ;
#95359=DIRECTION('center_axis',(0.,0.,-1.)) ;
#95360=DIRECTION('ref_axis',(-1.,0.,0.)) ;
#95361=DIRECTION('center_axis',(0.,0.,-1.)) ;
#95362=DIRECTION('ref_axis',(-1.,0.,0.)) ;
#95363=DIRECTION('center_axis',(1.,1.53063836115601E-16,-3.06472600140763E-33)) ;
#95364=DIRECTION('ref_axis',(-1.53063836115601E-16,1.,4.69098718418678E-49)) ;
#95365=DIRECTION('center_axis',(-1.,0.,0.)) ;
#95366=DIRECTION('ref_axis',(0.,0.,1.)) ;
#95367=DIRECTION('center_axis',(-1.53063836115601E-16,1.,-1.020425574104E-16)) ;
#95368=DIRECTION('ref_axis',(-1.,-1.53063836115601E-16,1.3684555315672E-47)) ;
#95369=DIRECTION('',(1.53063836115601E-16,-1.,1.020425574104E-16)) ;
#95370=DIRECTION('center_axis',(0.,-1.,0.)) ;
#95371=DIRECTION('ref_axis',(0.,0.,-1.)) ;
#95372=DIRECTION('center_axis',(-1.53063836115601E-16,1.,-1.30104260698261E-16)) ;
#95373=DIRECTION('ref_axis',(-1.,-1.53063836115601E-16,1.99142572374599E-32)) ;
#95374=DIRECTION('center_axis',(0.,-1.,0.)) ;
#95375=DIRECTION('ref_axis',(0.,0.,-1.)) ;
#95376=DIRECTION('center_axis',(-1.,-1.53063836115601E-16,2.73691106313441E-48)) ;
#95377=DIRECTION('ref_axis',(1.53063836115601E-16,-1.,-4.18922106430579E-64)) ;
#95378=DIRECTION('center_axis',(1.,2.16840434497101E-16,0.)) ;
#95379=DIRECTION('ref_axis',(2.16840434497101E-16,-1.,0.)) ;
#95380=DIRECTION('center_axis',(-1.,0.,2.16840434497095E-15)) ;
#95381=DIRECTION('ref_axis',(2.16840434497095E-15,0.,1.)) ;
#95382=DIRECTION('center_axis',(-1.,-2.16840434497101E-16,0.)) ;
#95383=DIRECTION('ref_axis',(0.,-1.,0.)) ;
#95384=DIRECTION('center_axis',(0.,0.,1.)) ;
#95385=DIRECTION('ref_axis',(-1.,0.,0.)) ;
#95386=DIRECTION('center_axis',(0.,1.,0.)) ;
#95387=DIRECTION('ref_axis',(1.,0.,0.)) ;
#95388=DIRECTION('center_axis',(0.,1.,0.)) ;
#95389=DIRECTION('ref_axis',(0.,0.,-1.)) ;
#95390=DIRECTION('center_axis',(1.,0.,0.)) ;
#95391=DIRECTION('ref_axis',(0.,-1.,0.)) ;
#95392=DIRECTION('center_axis',(1.,6.50521303491304E-15,0.)) ;
#95393=DIRECTION('ref_axis',(-6.50521303491304E-15,1.,0.)) ;
#95394=DIRECTION('center_axis',(8.67361737988403E-15,1.,0.)) ;
#95395=DIRECTION('ref_axis',(-1.,8.67361737988403E-15,0.)) ;
#95396=DIRECTION('center_axis',(1.2303003375722E-16,-1.,1.020425574104E-16)) ;
#95397=DIRECTION('ref_axis',(1.,1.2303003375722E-16,-1.25542992828747E-32)) ;
#95398=DIRECTION('center_axis',(0.,1.,0.)) ;
#95399=DIRECTION('ref_axis',(0.,0.,1.)) ;
#95400=DIRECTION('center_axis',(0.,1.,0.)) ;
#95401=DIRECTION('ref_axis',(1.,0.,0.)) ;
#95402=DIRECTION('center_axis',(1.,1.2303003375722E-16,0.)) ;
#95403=DIRECTION('ref_axis',(1.2303003375722E-16,-1.,0.)) ;
#95404=DIRECTION('center_axis',(0.,0.,1.)) ;
#95405=DIRECTION('ref_axis',(-1.,0.,0.)) ;
#95406=DIRECTION('center_axis',(0.,1.,0.)) ;
#95407=DIRECTION('ref_axis',(1.,0.,0.)) ;
#95408=DIRECTION('center_axis',(0.,0.,-1.)) ;
#95409=DIRECTION('ref_axis',(1.,0.,0.)) ;
#95410=DIRECTION('center_axis',(0.,0.,-1.)) ;
#95411=DIRECTION('ref_axis',(-1.,0.,0.)) ;
#95412=DIRECTION('center_axis',(0.,0.,1.)) ;
#95413=DIRECTION('ref_axis',(1.,0.,0.)) ;
#95414=DIRECTION('center_axis',(-2.16840434497101E-16,1.,-1.020425574104E-16)) ;
#95415=DIRECTION('ref_axis',(-1.,-2.16840434497101E-16,5.47382212626882E-48)) ;
#95416=DIRECTION('center_axis',(0.,1.,0.)) ;
#95417=DIRECTION('ref_axis',(0.,0.,-1.)) ;
#95418=DIRECTION('center_axis',(1.,0.,1.25542992828747E-32)) ;
#95419=DIRECTION('ref_axis',(1.25542992828747E-32,0.,-1.)) ;
#95420=DIRECTION('center_axis',(1.,0.,0.)) ;
#95421=DIRECTION('ref_axis',(0.,0.,-1.)) ;
#95422=DIRECTION('center_axis',(-1.,-1.2303003375722E-16,0.)) ;
#95423=DIRECTION('ref_axis',(0.,-1.,0.)) ;
#95424=DIRECTION('center_axis',(0.,0.,-1.)) ;
#95425=DIRECTION('ref_axis',(1.,0.,0.)) ;
#95426=DIRECTION('center_axis',(0.,0.,-1.)) ;
#95427=DIRECTION('ref_axis',(-1.,0.,0.)) ;
#95428=DIRECTION('',(0.,0.,1.)) ;
#95429=DIRECTION('center_axis',(0.,0.,1.)) ;
#95430=DIRECTION('ref_axis',(1.,0.,0.)) ;
#95431=DIRECTION('center_axis',(0.,0.,1.)) ;
#95432=DIRECTION('ref_axis',(1.,0.,0.)) ;
#95433=DIRECTION('center_axis',(6.27714964143733E-33,-5.10212787052002E-17,
-1.)) ;
#95434=DIRECTION('ref_axis',(3.20268201330022E-49,1.,-5.10212787052002E-17)) ;
#95435=DIRECTION('center_axis',(1.,1.53063836115601E-16,-1.53236300070382E-33)) ;
#95436=DIRECTION('ref_axis',(-1.53063836115601E-16,1.,2.34549359209339E-49)) ;
#95437=DIRECTION('center_axis',(-1.,0.,0.)) ;
#95438=DIRECTION('ref_axis',(0.,0.,1.)) ;
#95439=DIRECTION('center_axis',(1.,0.,0.)) ;
#95440=DIRECTION('ref_axis',(0.,0.,-1.)) ;
#95441=DIRECTION('center_axis',(0.,1.,0.)) ;
#95442=DIRECTION('ref_axis',(1.,0.,0.)) ;
#95443=DIRECTION('center_axis',(-4.33680868994202E-15,1.,0.)) ;
#95444=DIRECTION('ref_axis',(1.,4.33680868994202E-15,0.)) ;
#95445=DIRECTION('center_axis',(0.,-1.,0.)) ;
#95446=DIRECTION('ref_axis',(0.,0.,-1.)) ;
#95447=DIRECTION('center_axis',(0.,0.,-1.)) ;
#95448=DIRECTION('ref_axis',(1.,0.,0.)) ;
#95449=DIRECTION('center_axis',(0.,0.,1.)) ;
#95450=DIRECTION('ref_axis',(1.,0.,0.)) ;
#95451=DIRECTION('center_axis',(0.,0.,-1.)) ;
#95452=DIRECTION('ref_axis',(-1.,0.,0.)) ;
#95453=DIRECTION('center_axis',(0.,1.,0.)) ;
#95454=DIRECTION('ref_axis',(1.,0.,0.)) ;
#95455=DIRECTION('center_axis',(1.,1.2303003375722E-16,0.)) ;
#95456=DIRECTION('ref_axis',(1.2303003375722E-16,-1.,0.)) ;
#95457=DIRECTION('center_axis',(0.,1.,0.)) ;
#95458=DIRECTION('ref_axis',(-6.50521303491284E-15,0.,-1.)) ;
#95459=DIRECTION('center_axis',(6.27714964143733E-33,-5.10212787052002E-17,
-1.)) ;
#95460=DIRECTION('ref_axis',(0.,1.,0.)) ;
#95461=DIRECTION('center_axis',(0.,-1.,0.)) ;
#95462=DIRECTION('ref_axis',(0.,0.,1.)) ;
#95463=DIRECTION('center_axis',(2.16840434497101E-16,-1.,5.10212787052002E-17)) ;
#95464=DIRECTION('ref_axis',(1.,2.16840434497101E-16,-5.47382212626882E-48)) ;
#95465=DIRECTION('center_axis',(0.,1.,0.)) ;
#95466=DIRECTION('ref_axis',(0.,0.,-1.)) ;
#95467=DIRECTION('center_axis',(0.,0.,1.)) ;
#95468=DIRECTION('ref_axis',(1.,0.,0.)) ;
#95469=DIRECTION('center_axis',(0.,0.,-1.)) ;
#95470=DIRECTION('ref_axis',(-1.,0.,0.)) ;
#95471=DIRECTION('center_axis',(-1.,-1.2303003375722E-16,0.)) ;
#95472=DIRECTION('ref_axis',(0.,-1.,0.)) ;
#95473=DIRECTION('center_axis',(0.,-1.,0.)) ;
#95474=DIRECTION('ref_axis',(0.,0.,1.)) ;
#95475=DIRECTION('center_axis',(1.53063836115601E-16,-1.,5.10212787052002E-17)) ;
#95476=DIRECTION('ref_axis',(1.,1.53063836115601E-16,-6.84227765783602E-48)) ;
#95477=DIRECTION('',(-1.53063836115601E-16,1.,-5.10212787052002E-17)) ;
#95478=DIRECTION('center_axis',(0.,-1.,0.)) ;
#95479=DIRECTION('ref_axis',(0.,0.,-1.)) ;
#95480=DIRECTION('center_axis',(-1.,0.,0.)) ;
#95481=DIRECTION('ref_axis',(0.,0.,-1.)) ;
#95482=DIRECTION('center_axis',(-1.2303003375722E-16,1.,-5.10212787052002E-17)) ;
#95483=DIRECTION('ref_axis',(-1.,-1.2303003375722E-16,6.27714964143733E-33)) ;
#95484=DIRECTION('center_axis',(-8.67361737988403E-15,-1.,0.)) ;
#95485=DIRECTION('ref_axis',(1.,-8.67361737988403E-15,0.)) ;
#95486=DIRECTION('center_axis',(1.,0.,6.27714964143733E-33)) ;
#95487=DIRECTION('ref_axis',(6.27714964143733E-33,0.,-1.)) ;
#95488=DIRECTION('center_axis',(-1.,0.,-6.50521303491284E-15)) ;
#95489=DIRECTION('ref_axis',(-6.50521303491284E-15,0.,1.)) ;
#95490=DIRECTION('center_axis',(1.,0.,0.)) ;
#95491=DIRECTION('ref_axis',(0.,1.,0.)) ;
#95492=DIRECTION('center_axis',(0.,0.,-1.)) ;
#95493=DIRECTION('ref_axis',(-1.,0.,0.)) ;
#95494=DIRECTION('center_axis',(0.,0.,1.)) ;
#95495=DIRECTION('ref_axis',(1.,0.,0.)) ;
#95496=DIRECTION('center_axis',(0.,0.,-1.)) ;
#95497=DIRECTION('ref_axis',(-1.,0.,0.)) ;
#95498=DIRECTION('center_axis',(-1.,0.,0.)) ;
#95499=DIRECTION('ref_axis',(0.,0.,1.)) ;
#95500=DIRECTION('center_axis',(0.,-1.,0.)) ;
#95501=DIRECTION('ref_axis',(0.,0.,-1.)) ;
#95502=DIRECTION('center_axis',(0.,1.,0.)) ;
#95503=DIRECTION('ref_axis',(0.,0.,1.)) ;
#95504=DIRECTION('center_axis',(0.,1.,-6.50521303491284E-15)) ;
#95505=DIRECTION('ref_axis',(0.,6.50521303491284E-15,1.)) ;
#95506=DIRECTION('center_axis',(0.,-1.,0.)) ;
#95507=DIRECTION('ref_axis',(0.,0.,-1.)) ;
#95508=DIRECTION('center_axis',(0.,-1.,0.)) ;
#95509=DIRECTION('ref_axis',(0.,0.,-1.)) ;
#95510=DIRECTION('center_axis',(0.,-1.,-1.07081696047951E-16)) ;
#95511=DIRECTION('ref_axis',(0.,1.07081696047951E-16,-1.)) ;
#95512=DIRECTION('center_axis',(0.,1.,0.)) ;
#95513=DIRECTION('ref_axis',(0.,0.,1.)) ;
#95514=DIRECTION('center_axis',(-1.,0.,0.)) ;
#95515=DIRECTION('ref_axis',(0.,0.,1.)) ;
#95516=DIRECTION('center_axis',(0.,0.,1.)) ;
#95517=DIRECTION('ref_axis',(1.,0.,0.)) ;
#95518=DIRECTION('center_axis',(0.,1.,0.)) ;
#95519=DIRECTION('ref_axis',(0.,0.,1.)) ;
#95520=DIRECTION('center_axis',(0.,0.,-1.)) ;
#95521=DIRECTION('ref_axis',(-1.,0.,0.)) ;
#95522=DIRECTION('center_axis',(0.,0.,1.)) ;
#95523=DIRECTION('ref_axis',(1.,0.,0.)) ;
#95524=DIRECTION('center_axis',(0.,0.,1.)) ;
#95525=DIRECTION('ref_axis',(1.,0.,0.)) ;
#95526=DIRECTION('center_axis',(0.,0.,1.)) ;
#95527=DIRECTION('ref_axis',(1.,0.,0.)) ;
#95528=DIRECTION('center_axis',(0.,0.,-1.)) ;
#95529=DIRECTION('ref_axis',(-1.,0.,0.)) ;
#95530=DIRECTION('center_axis',(0.,1.,0.)) ;
#95531=DIRECTION('ref_axis',(0.,0.,1.)) ;
#95532=DIRECTION('center_axis',(0.,-0.707106781186532,0.707106781186563)) ;
#95533=DIRECTION('ref_axis',(0.,-0.707106781186563,-0.707106781186532)) ;
#95534=DIRECTION('center_axis',(0.,1.,0.)) ;
#95535=DIRECTION('ref_axis',(0.,0.,1.)) ;
#95536=DIRECTION('center_axis',(2.23012492569655E-15,-0.51423179695906,
-0.857651245551627)) ;
#95537=DIRECTION('ref_axis',(2.6714619735869E-30,0.857651245551626,-0.51423179695906)) ;
#95538=DIRECTION('center_axis',(0.,-0.707106781186548,0.707106781186547)) ;
#95539=DIRECTION('ref_axis',(0.,-0.707106781186547,-0.707106781186548)) ;
#95540=DIRECTION('center_axis',(0.,-0.707106781186543,0.707106781186552)) ;
#95541=DIRECTION('ref_axis',(0.,-0.707106781186552,-0.707106781186543)) ;
#95542=DIRECTION('center_axis',(-1.,0.,0.)) ;
#95543=DIRECTION('ref_axis',(0.,0.,1.)) ;
#95544=DIRECTION('center_axis',(-6.69037477709043E-15,0.51423179695912,
-0.85765124555159)) ;
#95545=DIRECTION('ref_axis',(-4.44487660401203E-29,0.85765124555159,0.51423179695912)) ;
#95546=DIRECTION('center_axis',(0.,1.,0.)) ;
#95547=DIRECTION('ref_axis',(0.,0.,1.)) ;
#95548=DIRECTION('center_axis',(0.,0.,-1.)) ;
#95549=DIRECTION('ref_axis',(-1.,0.,0.)) ;
#95550=DIRECTION('center_axis',(0.,1.,0.)) ;
#95551=DIRECTION('ref_axis',(0.,0.,1.)) ;
#95552=DIRECTION('center_axis',(0.,0.,-1.)) ;
#95553=DIRECTION('ref_axis',(-1.,0.,0.)) ;
#95554=DIRECTION('center_axis',(0.,0.,-1.)) ;
#95555=DIRECTION('ref_axis',(-1.,0.,0.)) ;
#95556=DIRECTION('center_axis',(0.,0.,1.)) ;
#95557=DIRECTION('ref_axis',(1.,0.,0.)) ;
#95558=DIRECTION('center_axis',(0.,0.,-1.)) ;
#95559=DIRECTION('ref_axis',(-1.,0.,0.)) ;
#95560=DIRECTION('center_axis',(0.,1.,0.)) ;
#95561=DIRECTION('ref_axis',(0.,0.,1.)) ;
#95562=DIRECTION('center_axis',(0.,-1.,8.67361737988379E-15)) ;
#95563=DIRECTION('ref_axis',(0.,-8.67361737988379E-15,-1.)) ;
#95564=DIRECTION('center_axis',(0.,0.707106781186546,0.707106781186549)) ;
#95565=DIRECTION('ref_axis',(0.,-0.707106781186549,0.707106781186546)) ;
#95566=DIRECTION('center_axis',(0.,0.707106781186534,0.707106781186561)) ;
#95567=DIRECTION('ref_axis',(0.,-0.707106781186561,0.707106781186534)) ;
#95568=DIRECTION('center_axis',(0.,1.,1.07081696047951E-16)) ;
#95569=DIRECTION('ref_axis',(0.,-1.07081696047951E-16,1.)) ;
#95570=DIRECTION('center_axis',(0.,-1.,0.)) ;
#95571=DIRECTION('ref_axis',(0.,0.,-1.)) ;
#95572=DIRECTION('center_axis',(0.,1.,0.)) ;
#95573=DIRECTION('ref_axis',(0.,0.,1.)) ;
#95574=DIRECTION('center_axis',(0.,0.,1.)) ;
#95575=DIRECTION('ref_axis',(1.,0.,0.)) ;
#95576=DIRECTION('center_axis',(0.,1.,0.)) ;
#95577=DIRECTION('ref_axis',(0.,0.,1.)) ;
#95578=DIRECTION('center_axis',(0.,6.93889390390723E-14,1.)) ;
#95579=DIRECTION('ref_axis',(0.,-1.,6.93889390390723E-14)) ;
#95580=DIRECTION('center_axis',(0.,3.99416362155027E-15,1.)) ;
#95581=DIRECTION('ref_axis',(0.,-1.,3.99416362155027E-15)) ;
#95582=DIRECTION('center_axis',(0.,0.,1.)) ;
#95583=DIRECTION('ref_axis',(1.,0.,0.)) ;
#95584=DIRECTION('center_axis',(0.,0.,-1.)) ;
#95585=DIRECTION('ref_axis',(-1.,0.,0.)) ;
#95586=DIRECTION('center_axis',(0.,0.,1.)) ;
#95587=DIRECTION('ref_axis',(1.,0.,0.)) ;
#95588=DIRECTION('center_axis',(-1.,0.,0.)) ;
#95589=DIRECTION('ref_axis',(0.,0.,1.)) ;
#95590=DIRECTION('center_axis',(0.,1.,0.)) ;
#95591=DIRECTION('ref_axis',(0.,0.,1.)) ;
#95592=DIRECTION('center_axis',(-1.,0.,0.)) ;
#95593=DIRECTION('ref_axis',(0.,0.,1.)) ;
#95594=DIRECTION('center_axis',(0.,-1.,0.)) ;
#95595=DIRECTION('ref_axis',(0.,0.,-1.)) ;
#95596=DIRECTION('center_axis',(0.,1.,0.)) ;
#95597=DIRECTION('ref_axis',(0.,0.,1.)) ;
#95598=DIRECTION('center_axis',(1.,-9.85638338623186E-18,0.)) ;
#95599=DIRECTION('ref_axis',(9.85638338623186E-18,1.,0.)) ;
#95600=DIRECTION('',(0.,0.,-1.)) ;
#95601=DIRECTION('',(-9.85638338623186E-18,-1.,0.)) ;
#95602=DIRECTION('',(0.,0.,1.)) ;
#95603=DIRECTION('',(9.85638338623186E-18,1.,0.)) ;
#95604=DIRECTION('center_axis',(0.707106781186548,0.707106781186548,0.)) ;
#95605=DIRECTION('ref_axis',(-0.707106781186548,0.707106781186548,0.)) ;
#95606=DIRECTION('',(0.,0.,1.)) ;
#95607=DIRECTION('',(-0.577350269189625,0.577350269189625,0.577350269189627)) ;
#95608=DIRECTION('',(0.,0.,-1.)) ;
#95609=DIRECTION('',(0.577350269189625,-0.577350269189625,0.577350269189627)) ;
#95610=DIRECTION('center_axis',(0.,1.,0.)) ;
#95611=DIRECTION('ref_axis',(0.,0.,1.)) ;
#95612=DIRECTION('',(0.,0.,1.)) ;
#95613=DIRECTION('',(-1.,0.,-9.8563833862319E-18)) ;
#95614=DIRECTION('',(0.,0.,-1.)) ;
#95615=DIRECTION('',(1.,0.,-9.8563833862319E-18)) ;
#95616=DIRECTION('center_axis',(-0.707106781186548,0.707106781186548,0.)) ;
#95617=DIRECTION('ref_axis',(-0.707106781186548,-0.707106781186548,0.)) ;
#95618=DIRECTION('',(0.,0.,1.)) ;
#95619=DIRECTION('',(-0.577350269189625,-0.577350269189625,-0.577350269189627)) ;
#95620=DIRECTION('',(0.,0.,-1.)) ;
#95621=DIRECTION('',(0.577350269189625,0.577350269189625,-0.577350269189627)) ;
#95622=DIRECTION('center_axis',(-1.,9.85638338623186E-18,0.)) ;
#95623=DIRECTION('ref_axis',(-9.85638338623186E-18,-1.,0.)) ;
#95624=DIRECTION('',(0.,0.,-1.)) ;
#95625=DIRECTION('',(9.85638338623186E-18,1.,0.)) ;
#95626=DIRECTION('',(0.,0.,-1.)) ;
#95627=DIRECTION('',(-9.85638338623186E-18,-1.,0.)) ;
#95628=DIRECTION('center_axis',(0.,0.,1.)) ;
#95629=DIRECTION('ref_axis',(1.,0.,0.)) ;
#95630=DIRECTION('',(9.85638338623186E-18,1.,0.)) ;
#95631=DIRECTION('center_axis',(0.,0.,-1.)) ;
#95632=DIRECTION('ref_axis',(1.,0.,0.)) ;
#95633=DIRECTION('center_axis',(0.,0.,1.)) ;
#95634=DIRECTION('ref_axis',(1.,0.,0.)) ;
#95635=DIRECTION('',(-9.85638338623186E-18,-1.,0.)) ;
#95636=DIRECTION('',(1.,-9.85638338623186E-18,0.)) ;
#95637=DIRECTION('center_axis',(0.,0.,1.)) ;
#95638=DIRECTION('ref_axis',(1.,0.,0.)) ;
#95639=DIRECTION('',(9.85638338623186E-18,1.,0.)) ;
#95640=DIRECTION('center_axis',(0.,0.,-1.)) ;
#95641=DIRECTION('ref_axis',(1.,0.,0.)) ;
#95642=DIRECTION('center_axis',(0.,0.,1.)) ;
#95643=DIRECTION('ref_axis',(1.,0.,0.)) ;
#95644=DIRECTION('',(-9.85638338623186E-18,-1.,0.)) ;
#95645=DIRECTION('',(-1.,9.85638338623186E-18,0.)) ;
#95646=DIRECTION('center_axis',(0.,0.,-1.)) ;
#95647=DIRECTION('ref_axis',(-1.,0.,0.)) ;
#95648=DIRECTION('center_axis',(0.,0.,1.)) ;
#95649=DIRECTION('ref_axis',(1.,0.,0.)) ;
#95650=DIRECTION('center_axis',(0.,0.,-1.)) ;
#95651=DIRECTION('ref_axis',(1.,0.,0.)) ;
#95652=DIRECTION('center_axis',(0.,0.,-1.)) ;
#95653=DIRECTION('ref_axis',(-1.,0.,0.)) ;
#95654=DIRECTION('center_axis',(0.,0.,-1.)) ;
#95655=DIRECTION('ref_axis',(1.,0.,0.)) ;
#95656=DIRECTION('center_axis',(0.,0.,1.)) ;
#95657=DIRECTION('ref_axis',(1.,0.,0.)) ;
#95658=DIRECTION('center_axis',(-0.707106781186548,-0.707106781186547,0.)) ;
#95659=DIRECTION('ref_axis',(0.707106781186547,-0.707106781186548,0.)) ;
#95660=DIRECTION('',(0.,0.,1.)) ;
#95661=DIRECTION('',(0.577350269189625,-0.577350269189626,-0.577350269189626)) ;
#95662=DIRECTION('',(0.,0.,-1.)) ;
#95663=DIRECTION('',(-0.577350269189625,0.577350269189626,-0.577350269189626)) ;
#95664=DIRECTION('center_axis',(1.95511867169517E-16,-1.,0.)) ;
#95665=DIRECTION('ref_axis',(1.,1.95511867169517E-16,0.)) ;
#95666=DIRECTION('',(0.,0.,-1.)) ;
#95667=DIRECTION('',(-1.,-1.95511867169517E-16,0.)) ;
#95668=DIRECTION('',(1.,1.95511867169517E-16,0.)) ;
#95669=DIRECTION('center_axis',(1.06642836637918E-16,1.,0.)) ;
#95670=DIRECTION('ref_axis',(-1.,1.06642836637918E-16,0.)) ;
#95671=DIRECTION('',(1.,-1.06642836637919E-16,0.)) ;
#95672=DIRECTION('',(0.,0.,1.)) ;
#95673=DIRECTION('',(-1.,1.06642836637919E-16,0.)) ;
#95674=DIRECTION('center_axis',(-0.707106781186548,0.707106781186547,0.)) ;
#95675=DIRECTION('ref_axis',(-0.707106781186547,-0.707106781186548,0.)) ;
#95676=DIRECTION('',(0.,0.,1.)) ;
#95677=DIRECTION('',(-0.577350269189625,-0.577350269189626,0.577350269189627)) ;
#95678=DIRECTION('',(0.,0.,-1.)) ;
#95679=DIRECTION('',(0.577350269189625,0.577350269189626,0.577350269189627)) ;
#95680=DIRECTION('center_axis',(-1.,0.,0.)) ;
#95681=DIRECTION('ref_axis',(0.,0.,1.)) ;
#95682=DIRECTION('',(0.,0.,-1.)) ;
#95683=DIRECTION('',(0.,1.,1.95511867169518E-16)) ;
#95684=DIRECTION('',(0.,0.,1.)) ;
#95685=DIRECTION('',(0.,-1.,1.95511867169518E-16)) ;
#95686=DIRECTION('center_axis',(0.,0.,1.)) ;
#95687=DIRECTION('ref_axis',(1.,0.,0.)) ;
#95688=DIRECTION('',(-1.95511867169517E-16,1.,0.)) ;
#95689=DIRECTION('',(-1.,-1.95511867169517E-16,0.)) ;
#95690=DIRECTION('',(1.,-1.06642836637919E-16,0.)) ;
#95691=DIRECTION('center_axis',(0.,0.,1.)) ;
#95692=DIRECTION('ref_axis',(1.,0.,0.)) ;
#95693=DIRECTION('',(1.,1.95511867169517E-16,0.)) ;
#95694=DIRECTION('',(1.95511867169517E-16,-1.,0.)) ;
#95695=DIRECTION('',(-1.,1.06642836637919E-16,0.)) ;
#95696=DIRECTION('center_axis',(1.,-9.85638338623186E-18,0.)) ;
#95697=DIRECTION('ref_axis',(9.85638338623186E-18,1.,0.)) ;
#95698=DIRECTION('',(0.,0.,-1.)) ;
#95699=DIRECTION('',(-9.85638338623186E-18,-1.,0.)) ;
#95700=DIRECTION('',(0.,0.,1.)) ;
#95701=DIRECTION('',(9.85638338623186E-18,1.,0.)) ;
#95702=DIRECTION('center_axis',(0.707106781186548,0.707106781186548,0.)) ;
#95703=DIRECTION('ref_axis',(-0.707106781186548,0.707106781186548,0.)) ;
#95704=DIRECTION('',(0.,0.,1.)) ;
#95705=DIRECTION('',(-0.577350269189625,0.577350269189625,0.577350269189627)) ;
#95706=DIRECTION('',(0.,0.,-1.)) ;
#95707=DIRECTION('',(0.577350269189625,-0.577350269189625,0.577350269189627)) ;
#95708=DIRECTION('center_axis',(0.,1.,0.)) ;
#95709=DIRECTION('ref_axis',(0.,0.,1.)) ;
#95710=DIRECTION('',(0.,0.,1.)) ;
#95711=DIRECTION('',(-1.,0.,-9.8563833862319E-18)) ;
#95712=DIRECTION('',(0.,0.,-1.)) ;
#95713=DIRECTION('',(1.,0.,-9.8563833862319E-18)) ;
#95714=DIRECTION('center_axis',(-0.707106781186548,0.707106781186548,0.)) ;
#95715=DIRECTION('ref_axis',(-0.707106781186548,-0.707106781186548,0.)) ;
#95716=DIRECTION('',(0.,0.,1.)) ;
#95717=DIRECTION('',(-0.577350269189625,-0.577350269189625,-0.577350269189627)) ;
#95718=DIRECTION('',(0.,0.,-1.)) ;
#95719=DIRECTION('',(0.577350269189625,0.577350269189625,-0.577350269189627)) ;
#95720=DIRECTION('center_axis',(-1.,9.85638338623186E-18,0.)) ;
#95721=DIRECTION('ref_axis',(-9.85638338623186E-18,-1.,0.)) ;
#95722=DIRECTION('',(0.,0.,-1.)) ;
#95723=DIRECTION('',(9.85638338623186E-18,1.,0.)) ;
#95724=DIRECTION('',(0.,0.,-1.)) ;
#95725=DIRECTION('',(-9.85638338623186E-18,-1.,0.)) ;
#95726=DIRECTION('center_axis',(0.,0.,1.)) ;
#95727=DIRECTION('ref_axis',(1.,0.,0.)) ;
#95728=DIRECTION('',(9.85638338623186E-18,1.,0.)) ;
#95729=DIRECTION('center_axis',(0.,0.,-1.)) ;
#95730=DIRECTION('ref_axis',(1.,0.,0.)) ;
#95731=DIRECTION('center_axis',(0.,0.,1.)) ;
#95732=DIRECTION('ref_axis',(1.,0.,0.)) ;
#95733=DIRECTION('',(-9.85638338623186E-18,-1.,0.)) ;
#95734=DIRECTION('',(1.,-9.85638338623186E-18,0.)) ;
#95735=DIRECTION('center_axis',(0.,0.,1.)) ;
#95736=DIRECTION('ref_axis',(1.,0.,0.)) ;
#95737=DIRECTION('',(9.85638338623186E-18,1.,0.)) ;
#95738=DIRECTION('center_axis',(0.,0.,-1.)) ;
#95739=DIRECTION('ref_axis',(1.,0.,0.)) ;
#95740=DIRECTION('center_axis',(0.,0.,1.)) ;
#95741=DIRECTION('ref_axis',(1.,0.,0.)) ;
#95742=DIRECTION('',(-9.85638338623186E-18,-1.,0.)) ;
#95743=DIRECTION('',(-1.,9.85638338623186E-18,0.)) ;
#95744=DIRECTION('center_axis',(0.,0.,-1.)) ;
#95745=DIRECTION('ref_axis',(-1.,0.,0.)) ;
#95746=DIRECTION('center_axis',(0.,0.,1.)) ;
#95747=DIRECTION('ref_axis',(1.,0.,0.)) ;
#95748=DIRECTION('center_axis',(0.,0.,-1.)) ;
#95749=DIRECTION('ref_axis',(1.,0.,0.)) ;
#95750=DIRECTION('center_axis',(0.,0.,-1.)) ;
#95751=DIRECTION('ref_axis',(-1.,0.,0.)) ;
#95752=DIRECTION('center_axis',(0.,0.,-1.)) ;
#95753=DIRECTION('ref_axis',(1.,0.,0.)) ;
#95754=DIRECTION('center_axis',(0.,0.,1.)) ;
#95755=DIRECTION('ref_axis',(1.,0.,0.)) ;
#95756=DIRECTION('center_axis',(-0.707106781186548,-0.707106781186547,0.)) ;
#95757=DIRECTION('ref_axis',(0.707106781186547,-0.707106781186548,0.)) ;
#95758=DIRECTION('',(0.,0.,1.)) ;
#95759=DIRECTION('',(0.577350269189625,-0.577350269189626,-0.577350269189626)) ;
#95760=DIRECTION('',(0.,0.,-1.)) ;
#95761=DIRECTION('',(-0.577350269189625,0.577350269189626,-0.577350269189626)) ;
#95762=DIRECTION('center_axis',(1.95511867169517E-16,-1.,0.)) ;
#95763=DIRECTION('ref_axis',(1.,1.95511867169517E-16,0.)) ;
#95764=DIRECTION('',(0.,0.,-1.)) ;
#95765=DIRECTION('',(-1.,-1.95511867169517E-16,0.)) ;
#95766=DIRECTION('',(1.,1.95511867169517E-16,0.)) ;
#95767=DIRECTION('center_axis',(1.06642836637918E-16,1.,0.)) ;
#95768=DIRECTION('ref_axis',(-1.,1.06642836637918E-16,0.)) ;
#95769=DIRECTION('',(1.,-1.06642836637919E-16,0.)) ;
#95770=DIRECTION('',(0.,0.,1.)) ;
#95771=DIRECTION('',(-1.,1.06642836637919E-16,0.)) ;
#95772=DIRECTION('center_axis',(-0.707106781186548,0.707106781186547,0.)) ;
#95773=DIRECTION('ref_axis',(-0.707106781186547,-0.707106781186548,0.)) ;
#95774=DIRECTION('',(0.,0.,1.)) ;
#95775=DIRECTION('',(-0.577350269189625,-0.577350269189626,0.577350269189627)) ;
#95776=DIRECTION('',(0.,0.,-1.)) ;
#95777=DIRECTION('',(0.577350269189625,0.577350269189626,0.577350269189627)) ;
#95778=DIRECTION('center_axis',(-1.,0.,0.)) ;
#95779=DIRECTION('ref_axis',(0.,0.,1.)) ;
#95780=DIRECTION('',(0.,0.,-1.)) ;
#95781=DIRECTION('',(0.,1.,1.95511867169518E-16)) ;
#95782=DIRECTION('',(0.,0.,1.)) ;
#95783=DIRECTION('',(0.,-1.,1.95511867169518E-16)) ;
#95784=DIRECTION('center_axis',(0.,0.,1.)) ;
#95785=DIRECTION('ref_axis',(1.,0.,0.)) ;
#95786=DIRECTION('',(-1.95511867169517E-16,1.,0.)) ;
#95787=DIRECTION('',(-1.,-1.95511867169517E-16,0.)) ;
#95788=DIRECTION('',(1.,-1.06642836637919E-16,0.)) ;
#95789=DIRECTION('center_axis',(0.,0.,1.)) ;
#95790=DIRECTION('ref_axis',(1.,0.,0.)) ;
#95791=DIRECTION('',(1.,1.95511867169517E-16,0.)) ;
#95792=DIRECTION('',(1.95511867169517E-16,-1.,0.)) ;
#95793=DIRECTION('',(-1.,1.06642836637919E-16,0.)) ;
#95794=DIRECTION('center_axis',(1.,-9.85638338623186E-18,0.)) ;
#95795=DIRECTION('ref_axis',(9.85638338623186E-18,1.,0.)) ;
#95796=DIRECTION('',(0.,0.,-1.)) ;
#95797=DIRECTION('',(-9.85638338623186E-18,-1.,0.)) ;
#95798=DIRECTION('',(0.,0.,1.)) ;
#95799=DIRECTION('',(9.85638338623186E-18,1.,0.)) ;
#95800=DIRECTION('center_axis',(0.707106781186548,0.707106781186548,0.)) ;
#95801=DIRECTION('ref_axis',(-0.707106781186548,0.707106781186548,0.)) ;
#95802=DIRECTION('',(0.,0.,1.)) ;
#95803=DIRECTION('',(-0.577350269189625,0.577350269189625,0.577350269189627)) ;
#95804=DIRECTION('',(0.,0.,-1.)) ;
#95805=DIRECTION('',(0.577350269189625,-0.577350269189625,0.577350269189627)) ;
#95806=DIRECTION('center_axis',(0.,1.,0.)) ;
#95807=DIRECTION('ref_axis',(0.,0.,1.)) ;
#95808=DIRECTION('',(0.,0.,1.)) ;
#95809=DIRECTION('',(-1.,0.,-9.8563833862319E-18)) ;
#95810=DIRECTION('',(0.,0.,-1.)) ;
#95811=DIRECTION('',(1.,0.,-9.8563833862319E-18)) ;
#95812=DIRECTION('center_axis',(-0.707106781186548,0.707106781186548,0.)) ;
#95813=DIRECTION('ref_axis',(-0.707106781186548,-0.707106781186548,0.)) ;
#95814=DIRECTION('',(0.,0.,1.)) ;
#95815=DIRECTION('',(-0.577350269189625,-0.577350269189625,-0.577350269189627)) ;
#95816=DIRECTION('',(0.,0.,-1.)) ;
#95817=DIRECTION('',(0.577350269189625,0.577350269189625,-0.577350269189627)) ;
#95818=DIRECTION('center_axis',(-1.,9.85638338623186E-18,0.)) ;
#95819=DIRECTION('ref_axis',(-9.85638338623186E-18,-1.,0.)) ;
#95820=DIRECTION('',(0.,0.,-1.)) ;
#95821=DIRECTION('',(9.85638338623186E-18,1.,0.)) ;
#95822=DIRECTION('',(0.,0.,-1.)) ;
#95823=DIRECTION('',(-9.85638338623186E-18,-1.,0.)) ;
#95824=DIRECTION('center_axis',(0.,0.,1.)) ;
#95825=DIRECTION('ref_axis',(1.,0.,0.)) ;
#95826=DIRECTION('',(9.85638338623186E-18,1.,0.)) ;
#95827=DIRECTION('center_axis',(0.,0.,-1.)) ;
#95828=DIRECTION('ref_axis',(1.,0.,0.)) ;
#95829=DIRECTION('center_axis',(0.,0.,1.)) ;
#95830=DIRECTION('ref_axis',(1.,0.,0.)) ;
#95831=DIRECTION('',(-9.85638338623186E-18,-1.,0.)) ;
#95832=DIRECTION('',(1.,-9.85638338623186E-18,0.)) ;
#95833=DIRECTION('center_axis',(0.,0.,1.)) ;
#95834=DIRECTION('ref_axis',(1.,0.,0.)) ;
#95835=DIRECTION('',(9.85638338623186E-18,1.,0.)) ;
#95836=DIRECTION('center_axis',(0.,0.,-1.)) ;
#95837=DIRECTION('ref_axis',(1.,0.,0.)) ;
#95838=DIRECTION('center_axis',(0.,0.,1.)) ;
#95839=DIRECTION('ref_axis',(1.,0.,0.)) ;
#95840=DIRECTION('',(-9.85638338623186E-18,-1.,0.)) ;
#95841=DIRECTION('',(-1.,9.85638338623186E-18,0.)) ;
#95842=DIRECTION('center_axis',(0.,0.,-1.)) ;
#95843=DIRECTION('ref_axis',(-1.,0.,0.)) ;
#95844=DIRECTION('center_axis',(0.,0.,1.)) ;
#95845=DIRECTION('ref_axis',(1.,0.,0.)) ;
#95846=DIRECTION('center_axis',(0.,0.,-1.)) ;
#95847=DIRECTION('ref_axis',(1.,0.,0.)) ;
#95848=DIRECTION('center_axis',(0.,0.,-1.)) ;
#95849=DIRECTION('ref_axis',(-1.,0.,0.)) ;
#95850=DIRECTION('center_axis',(0.,0.,-1.)) ;
#95851=DIRECTION('ref_axis',(1.,0.,0.)) ;
#95852=DIRECTION('center_axis',(0.,0.,1.)) ;
#95853=DIRECTION('ref_axis',(1.,0.,0.)) ;
#95854=DIRECTION('center_axis',(-0.707106781186548,-0.707106781186547,0.)) ;
#95855=DIRECTION('ref_axis',(0.707106781186547,-0.707106781186548,0.)) ;
#95856=DIRECTION('',(0.,0.,1.)) ;
#95857=DIRECTION('',(0.577350269189625,-0.577350269189626,-0.577350269189626)) ;
#95858=DIRECTION('',(0.,0.,-1.)) ;
#95859=DIRECTION('',(-0.577350269189625,0.577350269189626,-0.577350269189626)) ;
#95860=DIRECTION('center_axis',(1.95511867169517E-16,-1.,0.)) ;
#95861=DIRECTION('ref_axis',(1.,1.95511867169517E-16,0.)) ;
#95862=DIRECTION('',(0.,0.,-1.)) ;
#95863=DIRECTION('',(-1.,-1.95511867169517E-16,0.)) ;
#95864=DIRECTION('',(1.,1.95511867169517E-16,0.)) ;
#95865=DIRECTION('center_axis',(1.06642836637918E-16,1.,0.)) ;
#95866=DIRECTION('ref_axis',(-1.,1.06642836637918E-16,0.)) ;
#95867=DIRECTION('',(1.,-1.06642836637919E-16,0.)) ;
#95868=DIRECTION('',(0.,0.,1.)) ;
#95869=DIRECTION('',(-1.,1.06642836637919E-16,0.)) ;
#95870=DIRECTION('center_axis',(-0.707106781186548,0.707106781186547,0.)) ;
#95871=DIRECTION('ref_axis',(-0.707106781186547,-0.707106781186548,0.)) ;
#95872=DIRECTION('',(0.,0.,1.)) ;
#95873=DIRECTION('',(-0.577350269189625,-0.577350269189626,0.577350269189627)) ;
#95874=DIRECTION('',(0.,0.,-1.)) ;
#95875=DIRECTION('',(0.577350269189625,0.577350269189626,0.577350269189627)) ;
#95876=DIRECTION('center_axis',(-1.,0.,0.)) ;
#95877=DIRECTION('ref_axis',(0.,0.,1.)) ;
#95878=DIRECTION('',(0.,0.,-1.)) ;
#95879=DIRECTION('',(0.,1.,1.95511867169518E-16)) ;
#95880=DIRECTION('',(0.,0.,1.)) ;
#95881=DIRECTION('',(0.,-1.,1.95511867169518E-16)) ;
#95882=DIRECTION('center_axis',(0.,0.,1.)) ;
#95883=DIRECTION('ref_axis',(1.,0.,0.)) ;
#95884=DIRECTION('',(-1.95511867169517E-16,1.,0.)) ;
#95885=DIRECTION('',(-1.,-1.95511867169517E-16,0.)) ;
#95886=DIRECTION('',(1.,-1.06642836637919E-16,0.)) ;
#95887=DIRECTION('center_axis',(0.,0.,1.)) ;
#95888=DIRECTION('ref_axis',(1.,0.,0.)) ;
#95889=DIRECTION('',(1.,1.95511867169517E-16,0.)) ;
#95890=DIRECTION('',(1.95511867169517E-16,-1.,0.)) ;
#95891=DIRECTION('',(-1.,1.06642836637919E-16,0.)) ;
#95892=DIRECTION('center_axis',(1.,-9.85638338623186E-18,0.)) ;
#95893=DIRECTION('ref_axis',(9.85638338623186E-18,1.,0.)) ;
#95894=DIRECTION('',(0.,0.,-1.)) ;
#95895=DIRECTION('',(-9.85638338623186E-18,-1.,0.)) ;
#95896=DIRECTION('',(0.,0.,1.)) ;
#95897=DIRECTION('',(9.85638338623186E-18,1.,0.)) ;
#95898=DIRECTION('center_axis',(0.707106781186548,0.707106781186548,0.)) ;
#95899=DIRECTION('ref_axis',(-0.707106781186548,0.707106781186548,0.)) ;
#95900=DIRECTION('',(0.,0.,1.)) ;
#95901=DIRECTION('',(-0.577350269189625,0.577350269189625,0.577350269189627)) ;
#95902=DIRECTION('',(0.,0.,-1.)) ;
#95903=DIRECTION('',(0.577350269189625,-0.577350269189625,0.577350269189627)) ;
#95904=DIRECTION('center_axis',(0.,1.,0.)) ;
#95905=DIRECTION('ref_axis',(0.,0.,1.)) ;
#95906=DIRECTION('',(0.,0.,1.)) ;
#95907=DIRECTION('',(-1.,0.,-9.8563833862319E-18)) ;
#95908=DIRECTION('',(0.,0.,-1.)) ;
#95909=DIRECTION('',(1.,0.,-9.8563833862319E-18)) ;
#95910=DIRECTION('center_axis',(-0.707106781186548,0.707106781186548,0.)) ;
#95911=DIRECTION('ref_axis',(-0.707106781186548,-0.707106781186548,0.)) ;
#95912=DIRECTION('',(0.,0.,1.)) ;
#95913=DIRECTION('',(-0.577350269189625,-0.577350269189625,-0.577350269189627)) ;
#95914=DIRECTION('',(0.,0.,-1.)) ;
#95915=DIRECTION('',(0.577350269189625,0.577350269189625,-0.577350269189627)) ;
#95916=DIRECTION('center_axis',(-1.,9.85638338623186E-18,0.)) ;
#95917=DIRECTION('ref_axis',(-9.85638338623186E-18,-1.,0.)) ;
#95918=DIRECTION('',(0.,0.,-1.)) ;
#95919=DIRECTION('',(9.85638338623186E-18,1.,0.)) ;
#95920=DIRECTION('',(0.,0.,-1.)) ;
#95921=DIRECTION('',(-9.85638338623186E-18,-1.,0.)) ;
#95922=DIRECTION('center_axis',(0.,0.,1.)) ;
#95923=DIRECTION('ref_axis',(1.,0.,0.)) ;
#95924=DIRECTION('',(9.85638338623186E-18,1.,0.)) ;
#95925=DIRECTION('center_axis',(0.,0.,-1.)) ;
#95926=DIRECTION('ref_axis',(1.,0.,0.)) ;
#95927=DIRECTION('center_axis',(0.,0.,1.)) ;
#95928=DIRECTION('ref_axis',(1.,0.,0.)) ;
#95929=DIRECTION('',(-9.85638338623186E-18,-1.,0.)) ;
#95930=DIRECTION('',(1.,-9.85638338623186E-18,0.)) ;
#95931=DIRECTION('center_axis',(0.,0.,1.)) ;
#95932=DIRECTION('ref_axis',(1.,0.,0.)) ;
#95933=DIRECTION('',(9.85638338623186E-18,1.,0.)) ;
#95934=DIRECTION('center_axis',(0.,0.,-1.)) ;
#95935=DIRECTION('ref_axis',(1.,0.,0.)) ;
#95936=DIRECTION('center_axis',(0.,0.,1.)) ;
#95937=DIRECTION('ref_axis',(1.,0.,0.)) ;
#95938=DIRECTION('',(-9.85638338623186E-18,-1.,0.)) ;
#95939=DIRECTION('',(-1.,9.85638338623186E-18,0.)) ;
#95940=DIRECTION('center_axis',(0.,0.,-1.)) ;
#95941=DIRECTION('ref_axis',(-1.,0.,0.)) ;
#95942=DIRECTION('center_axis',(0.,0.,1.)) ;
#95943=DIRECTION('ref_axis',(1.,0.,0.)) ;
#95944=DIRECTION('center_axis',(0.,0.,-1.)) ;
#95945=DIRECTION('ref_axis',(1.,0.,0.)) ;
#95946=DIRECTION('center_axis',(0.,0.,-1.)) ;
#95947=DIRECTION('ref_axis',(-1.,0.,0.)) ;
#95948=DIRECTION('center_axis',(0.,0.,-1.)) ;
#95949=DIRECTION('ref_axis',(1.,0.,0.)) ;
#95950=DIRECTION('center_axis',(0.,0.,1.)) ;
#95951=DIRECTION('ref_axis',(1.,0.,0.)) ;
#95952=DIRECTION('center_axis',(-0.707106781186548,-0.707106781186547,0.)) ;
#95953=DIRECTION('ref_axis',(0.707106781186547,-0.707106781186548,0.)) ;
#95954=DIRECTION('',(0.,0.,1.)) ;
#95955=DIRECTION('',(0.577350269189625,-0.577350269189626,-0.577350269189626)) ;
#95956=DIRECTION('',(0.,0.,-1.)) ;
#95957=DIRECTION('',(-0.577350269189625,0.577350269189626,-0.577350269189626)) ;
#95958=DIRECTION('center_axis',(1.95511867169517E-16,-1.,0.)) ;
#95959=DIRECTION('ref_axis',(1.,1.95511867169517E-16,0.)) ;
#95960=DIRECTION('',(0.,0.,-1.)) ;
#95961=DIRECTION('',(-1.,-1.95511867169517E-16,0.)) ;
#95962=DIRECTION('',(1.,1.95511867169517E-16,0.)) ;
#95963=DIRECTION('center_axis',(1.06642836637918E-16,1.,0.)) ;
#95964=DIRECTION('ref_axis',(-1.,1.06642836637918E-16,0.)) ;
#95965=DIRECTION('',(1.,-1.06642836637919E-16,0.)) ;
#95966=DIRECTION('',(0.,0.,1.)) ;
#95967=DIRECTION('',(-1.,1.06642836637919E-16,0.)) ;
#95968=DIRECTION('center_axis',(-0.707106781186548,0.707106781186547,0.)) ;
#95969=DIRECTION('ref_axis',(-0.707106781186547,-0.707106781186548,0.)) ;
#95970=DIRECTION('',(0.,0.,1.)) ;
#95971=DIRECTION('',(-0.577350269189625,-0.577350269189626,0.577350269189627)) ;
#95972=DIRECTION('',(0.,0.,-1.)) ;
#95973=DIRECTION('',(0.577350269189625,0.577350269189626,0.577350269189627)) ;
#95974=DIRECTION('center_axis',(-1.,0.,0.)) ;
#95975=DIRECTION('ref_axis',(0.,0.,1.)) ;
#95976=DIRECTION('',(0.,0.,-1.)) ;
#95977=DIRECTION('',(0.,1.,1.95511867169518E-16)) ;
#95978=DIRECTION('',(0.,0.,1.)) ;
#95979=DIRECTION('',(0.,-1.,1.95511867169518E-16)) ;
#95980=DIRECTION('center_axis',(0.,0.,1.)) ;
#95981=DIRECTION('ref_axis',(1.,0.,0.)) ;
#95982=DIRECTION('',(-1.95511867169517E-16,1.,0.)) ;
#95983=DIRECTION('',(-1.,-1.95511867169517E-16,0.)) ;
#95984=DIRECTION('',(1.,-1.06642836637919E-16,0.)) ;
#95985=DIRECTION('center_axis',(0.,0.,1.)) ;
#95986=DIRECTION('ref_axis',(1.,0.,0.)) ;
#95987=DIRECTION('',(1.,1.95511867169517E-16,0.)) ;
#95988=DIRECTION('',(1.95511867169517E-16,-1.,0.)) ;
#95989=DIRECTION('',(-1.,1.06642836637919E-16,0.)) ;
#95990=DIRECTION('center_axis',(1.,-9.85638338623186E-18,0.)) ;
#95991=DIRECTION('ref_axis',(9.85638338623186E-18,1.,0.)) ;
#95992=DIRECTION('',(0.,0.,-1.)) ;
#95993=DIRECTION('',(-9.85638338623186E-18,-1.,0.)) ;
#95994=DIRECTION('',(0.,0.,1.)) ;
#95995=DIRECTION('',(9.85638338623186E-18,1.,0.)) ;
#95996=DIRECTION('center_axis',(0.707106781186548,0.707106781186548,0.)) ;
#95997=DIRECTION('ref_axis',(-0.707106781186548,0.707106781186548,0.)) ;
#95998=DIRECTION('',(0.,0.,1.)) ;
#95999=DIRECTION('',(-0.577350269189625,0.577350269189625,0.577350269189627)) ;
#96000=DIRECTION('',(0.,0.,-1.)) ;
#96001=DIRECTION('',(0.577350269189625,-0.577350269189625,0.577350269189627)) ;
#96002=DIRECTION('center_axis',(0.,1.,0.)) ;
#96003=DIRECTION('ref_axis',(0.,0.,1.)) ;
#96004=DIRECTION('',(0.,0.,1.)) ;
#96005=DIRECTION('',(-1.,0.,-9.8563833862319E-18)) ;
#96006=DIRECTION('',(0.,0.,-1.)) ;
#96007=DIRECTION('',(1.,0.,-9.8563833862319E-18)) ;
#96008=DIRECTION('center_axis',(-0.707106781186548,0.707106781186548,0.)) ;
#96009=DIRECTION('ref_axis',(-0.707106781186548,-0.707106781186548,0.)) ;
#96010=DIRECTION('',(0.,0.,1.)) ;
#96011=DIRECTION('',(-0.577350269189625,-0.577350269189625,-0.577350269189627)) ;
#96012=DIRECTION('',(0.,0.,-1.)) ;
#96013=DIRECTION('',(0.577350269189625,0.577350269189625,-0.577350269189627)) ;
#96014=DIRECTION('center_axis',(-1.,9.85638338623186E-18,0.)) ;
#96015=DIRECTION('ref_axis',(-9.85638338623186E-18,-1.,0.)) ;
#96016=DIRECTION('',(0.,0.,-1.)) ;
#96017=DIRECTION('',(9.85638338623186E-18,1.,0.)) ;
#96018=DIRECTION('',(0.,0.,-1.)) ;
#96019=DIRECTION('',(-9.85638338623186E-18,-1.,0.)) ;
#96020=DIRECTION('center_axis',(0.,0.,1.)) ;
#96021=DIRECTION('ref_axis',(1.,0.,0.)) ;
#96022=DIRECTION('',(9.85638338623186E-18,1.,0.)) ;
#96023=DIRECTION('center_axis',(0.,0.,-1.)) ;
#96024=DIRECTION('ref_axis',(1.,0.,0.)) ;
#96025=DIRECTION('center_axis',(0.,0.,1.)) ;
#96026=DIRECTION('ref_axis',(1.,0.,0.)) ;
#96027=DIRECTION('',(-9.85638338623186E-18,-1.,0.)) ;
#96028=DIRECTION('',(1.,-9.85638338623186E-18,0.)) ;
#96029=DIRECTION('center_axis',(0.,0.,1.)) ;
#96030=DIRECTION('ref_axis',(1.,0.,0.)) ;
#96031=DIRECTION('',(9.85638338623186E-18,1.,0.)) ;
#96032=DIRECTION('center_axis',(0.,0.,-1.)) ;
#96033=DIRECTION('ref_axis',(1.,0.,0.)) ;
#96034=DIRECTION('center_axis',(0.,0.,1.)) ;
#96035=DIRECTION('ref_axis',(1.,0.,0.)) ;
#96036=DIRECTION('',(-9.85638338623186E-18,-1.,0.)) ;
#96037=DIRECTION('',(-1.,9.85638338623186E-18,0.)) ;
#96038=DIRECTION('center_axis',(0.,0.,-1.)) ;
#96039=DIRECTION('ref_axis',(-1.,0.,0.)) ;
#96040=DIRECTION('center_axis',(0.,0.,1.)) ;
#96041=DIRECTION('ref_axis',(1.,0.,0.)) ;
#96042=DIRECTION('center_axis',(0.,0.,-1.)) ;
#96043=DIRECTION('ref_axis',(1.,0.,0.)) ;
#96044=DIRECTION('center_axis',(0.,0.,-1.)) ;
#96045=DIRECTION('ref_axis',(-1.,0.,0.)) ;
#96046=DIRECTION('center_axis',(0.,0.,-1.)) ;
#96047=DIRECTION('ref_axis',(1.,0.,0.)) ;
#96048=DIRECTION('center_axis',(0.,0.,1.)) ;
#96049=DIRECTION('ref_axis',(1.,0.,0.)) ;
#96050=DIRECTION('center_axis',(-0.707106781186548,-0.707106781186547,0.)) ;
#96051=DIRECTION('ref_axis',(0.707106781186547,-0.707106781186548,0.)) ;
#96052=DIRECTION('',(0.,0.,1.)) ;
#96053=DIRECTION('',(0.577350269189625,-0.577350269189626,-0.577350269189626)) ;
#96054=DIRECTION('',(0.,0.,-1.)) ;
#96055=DIRECTION('',(-0.577350269189625,0.577350269189626,-0.577350269189626)) ;
#96056=DIRECTION('center_axis',(1.95511867169517E-16,-1.,0.)) ;
#96057=DIRECTION('ref_axis',(1.,1.95511867169517E-16,0.)) ;
#96058=DIRECTION('',(0.,0.,-1.)) ;
#96059=DIRECTION('',(-1.,-1.95511867169517E-16,0.)) ;
#96060=DIRECTION('',(1.,1.95511867169517E-16,0.)) ;
#96061=DIRECTION('center_axis',(1.06642836637918E-16,1.,0.)) ;
#96062=DIRECTION('ref_axis',(-1.,1.06642836637918E-16,0.)) ;
#96063=DIRECTION('',(1.,-1.06642836637919E-16,0.)) ;
#96064=DIRECTION('',(0.,0.,1.)) ;
#96065=DIRECTION('',(-1.,1.06642836637919E-16,0.)) ;
#96066=DIRECTION('center_axis',(-0.707106781186548,0.707106781186547,0.)) ;
#96067=DIRECTION('ref_axis',(-0.707106781186547,-0.707106781186548,0.)) ;
#96068=DIRECTION('',(0.,0.,1.)) ;
#96069=DIRECTION('',(-0.577350269189625,-0.577350269189626,0.577350269189627)) ;
#96070=DIRECTION('',(0.,0.,-1.)) ;
#96071=DIRECTION('',(0.577350269189625,0.577350269189626,0.577350269189627)) ;
#96072=DIRECTION('center_axis',(-1.,0.,0.)) ;
#96073=DIRECTION('ref_axis',(0.,0.,1.)) ;
#96074=DIRECTION('',(0.,0.,-1.)) ;
#96075=DIRECTION('',(0.,1.,1.95511867169518E-16)) ;
#96076=DIRECTION('',(0.,0.,1.)) ;
#96077=DIRECTION('',(0.,-1.,1.95511867169518E-16)) ;
#96078=DIRECTION('center_axis',(0.,0.,1.)) ;
#96079=DIRECTION('ref_axis',(1.,0.,0.)) ;
#96080=DIRECTION('',(-1.95511867169517E-16,1.,0.)) ;
#96081=DIRECTION('',(-1.,-1.95511867169517E-16,0.)) ;
#96082=DIRECTION('',(1.,-1.06642836637919E-16,0.)) ;
#96083=DIRECTION('center_axis',(0.,0.,1.)) ;
#96084=DIRECTION('ref_axis',(1.,0.,0.)) ;
#96085=DIRECTION('',(1.,1.95511867169517E-16,0.)) ;
#96086=DIRECTION('',(1.95511867169517E-16,-1.,0.)) ;
#96087=DIRECTION('',(-1.,1.06642836637919E-16,0.)) ;
#96088=DIRECTION('center_axis',(1.,-9.85638338623186E-18,0.)) ;
#96089=DIRECTION('ref_axis',(9.85638338623186E-18,1.,0.)) ;
#96090=DIRECTION('',(0.,0.,-1.)) ;
#96091=DIRECTION('',(-9.85638338623186E-18,-1.,0.)) ;
#96092=DIRECTION('',(0.,0.,1.)) ;
#96093=DIRECTION('',(9.85638338623186E-18,1.,0.)) ;
#96094=DIRECTION('center_axis',(0.707106781186548,0.707106781186548,0.)) ;
#96095=DIRECTION('ref_axis',(-0.707106781186548,0.707106781186548,0.)) ;
#96096=DIRECTION('',(0.,0.,1.)) ;
#96097=DIRECTION('',(-0.577350269189625,0.577350269189625,0.577350269189627)) ;
#96098=DIRECTION('',(0.,0.,-1.)) ;
#96099=DIRECTION('',(0.577350269189625,-0.577350269189625,0.577350269189627)) ;
#96100=DIRECTION('center_axis',(0.,1.,0.)) ;
#96101=DIRECTION('ref_axis',(0.,0.,1.)) ;
#96102=DIRECTION('',(0.,0.,1.)) ;
#96103=DIRECTION('',(-1.,0.,-9.8563833862319E-18)) ;
#96104=DIRECTION('',(0.,0.,-1.)) ;
#96105=DIRECTION('',(1.,0.,-9.8563833862319E-18)) ;
#96106=DIRECTION('center_axis',(-0.707106781186548,0.707106781186548,0.)) ;
#96107=DIRECTION('ref_axis',(-0.707106781186548,-0.707106781186548,0.)) ;
#96108=DIRECTION('',(0.,0.,1.)) ;
#96109=DIRECTION('',(-0.577350269189625,-0.577350269189625,-0.577350269189627)) ;
#96110=DIRECTION('',(0.,0.,-1.)) ;
#96111=DIRECTION('',(0.577350269189625,0.577350269189625,-0.577350269189627)) ;
#96112=DIRECTION('center_axis',(-1.,9.85638338623186E-18,0.)) ;
#96113=DIRECTION('ref_axis',(-9.85638338623186E-18,-1.,0.)) ;
#96114=DIRECTION('',(0.,0.,-1.)) ;
#96115=DIRECTION('',(9.85638338623186E-18,1.,0.)) ;
#96116=DIRECTION('',(0.,0.,-1.)) ;
#96117=DIRECTION('',(-9.85638338623186E-18,-1.,0.)) ;
#96118=DIRECTION('center_axis',(0.,0.,1.)) ;
#96119=DIRECTION('ref_axis',(1.,0.,0.)) ;
#96120=DIRECTION('',(9.85638338623186E-18,1.,0.)) ;
#96121=DIRECTION('center_axis',(0.,0.,-1.)) ;
#96122=DIRECTION('ref_axis',(1.,0.,0.)) ;
#96123=DIRECTION('center_axis',(0.,0.,1.)) ;
#96124=DIRECTION('ref_axis',(1.,0.,0.)) ;
#96125=DIRECTION('',(-9.85638338623186E-18,-1.,0.)) ;
#96126=DIRECTION('',(1.,-9.85638338623186E-18,0.)) ;
#96127=DIRECTION('center_axis',(0.,0.,1.)) ;
#96128=DIRECTION('ref_axis',(1.,0.,0.)) ;
#96129=DIRECTION('',(9.85638338623186E-18,1.,0.)) ;
#96130=DIRECTION('center_axis',(0.,0.,-1.)) ;
#96131=DIRECTION('ref_axis',(1.,0.,0.)) ;
#96132=DIRECTION('center_axis',(0.,0.,1.)) ;
#96133=DIRECTION('ref_axis',(1.,0.,0.)) ;
#96134=DIRECTION('',(-9.85638338623186E-18,-1.,0.)) ;
#96135=DIRECTION('',(-1.,9.85638338623186E-18,0.)) ;
#96136=DIRECTION('center_axis',(0.,0.,-1.)) ;
#96137=DIRECTION('ref_axis',(-1.,0.,0.)) ;
#96138=DIRECTION('center_axis',(0.,0.,1.)) ;
#96139=DIRECTION('ref_axis',(1.,0.,0.)) ;
#96140=DIRECTION('center_axis',(0.,0.,-1.)) ;
#96141=DIRECTION('ref_axis',(1.,0.,0.)) ;
#96142=DIRECTION('center_axis',(0.,0.,-1.)) ;
#96143=DIRECTION('ref_axis',(-1.,0.,0.)) ;
#96144=DIRECTION('center_axis',(0.,0.,-1.)) ;
#96145=DIRECTION('ref_axis',(1.,0.,0.)) ;
#96146=DIRECTION('center_axis',(0.,0.,1.)) ;
#96147=DIRECTION('ref_axis',(1.,0.,0.)) ;
#96148=DIRECTION('center_axis',(-0.707106781186548,-0.707106781186547,0.)) ;
#96149=DIRECTION('ref_axis',(0.707106781186547,-0.707106781186548,0.)) ;
#96150=DIRECTION('',(0.,0.,1.)) ;
#96151=DIRECTION('',(0.577350269189625,-0.577350269189626,-0.577350269189626)) ;
#96152=DIRECTION('',(0.,0.,-1.)) ;
#96153=DIRECTION('',(-0.577350269189625,0.577350269189626,-0.577350269189626)) ;
#96154=DIRECTION('center_axis',(1.95511867169517E-16,-1.,0.)) ;
#96155=DIRECTION('ref_axis',(1.,1.95511867169517E-16,0.)) ;
#96156=DIRECTION('',(0.,0.,-1.)) ;
#96157=DIRECTION('',(-1.,-1.95511867169517E-16,0.)) ;
#96158=DIRECTION('',(1.,1.95511867169517E-16,0.)) ;
#96159=DIRECTION('center_axis',(1.06642836637918E-16,1.,0.)) ;
#96160=DIRECTION('ref_axis',(-1.,1.06642836637918E-16,0.)) ;
#96161=DIRECTION('',(1.,-1.06642836637919E-16,0.)) ;
#96162=DIRECTION('',(0.,0.,1.)) ;
#96163=DIRECTION('',(-1.,1.06642836637919E-16,0.)) ;
#96164=DIRECTION('center_axis',(-0.707106781186548,0.707106781186547,0.)) ;
#96165=DIRECTION('ref_axis',(-0.707106781186547,-0.707106781186548,0.)) ;
#96166=DIRECTION('',(0.,0.,1.)) ;
#96167=DIRECTION('',(-0.577350269189625,-0.577350269189626,0.577350269189627)) ;
#96168=DIRECTION('',(0.,0.,-1.)) ;
#96169=DIRECTION('',(0.577350269189625,0.577350269189626,0.577350269189627)) ;
#96170=DIRECTION('center_axis',(-1.,0.,0.)) ;
#96171=DIRECTION('ref_axis',(0.,0.,1.)) ;
#96172=DIRECTION('',(0.,0.,-1.)) ;
#96173=DIRECTION('',(0.,1.,1.95511867169518E-16)) ;
#96174=DIRECTION('',(0.,0.,1.)) ;
#96175=DIRECTION('',(0.,-1.,1.95511867169518E-16)) ;
#96176=DIRECTION('center_axis',(0.,0.,1.)) ;
#96177=DIRECTION('ref_axis',(1.,0.,0.)) ;
#96178=DIRECTION('',(-1.95511867169517E-16,1.,0.)) ;
#96179=DIRECTION('',(-1.,-1.95511867169517E-16,0.)) ;
#96180=DIRECTION('',(1.,-1.06642836637919E-16,0.)) ;
#96181=DIRECTION('center_axis',(0.,0.,1.)) ;
#96182=DIRECTION('ref_axis',(1.,0.,0.)) ;
#96183=DIRECTION('',(1.,1.95511867169517E-16,0.)) ;
#96184=DIRECTION('',(1.95511867169517E-16,-1.,0.)) ;
#96185=DIRECTION('',(-1.,1.06642836637919E-16,0.)) ;
#96186=DIRECTION('center_axis',(1.,-9.85638338623186E-18,0.)) ;
#96187=DIRECTION('ref_axis',(9.85638338623186E-18,1.,0.)) ;
#96188=DIRECTION('',(0.,0.,-1.)) ;
#96189=DIRECTION('',(-9.85638338623186E-18,-1.,0.)) ;
#96190=DIRECTION('',(0.,0.,1.)) ;
#96191=DIRECTION('',(9.85638338623186E-18,1.,0.)) ;
#96192=DIRECTION('center_axis',(0.707106781186548,0.707106781186548,0.)) ;
#96193=DIRECTION('ref_axis',(-0.707106781186548,0.707106781186548,0.)) ;
#96194=DIRECTION('',(0.,0.,1.)) ;
#96195=DIRECTION('',(-0.577350269189625,0.577350269189625,0.577350269189627)) ;
#96196=DIRECTION('',(0.,0.,-1.)) ;
#96197=DIRECTION('',(0.577350269189625,-0.577350269189625,0.577350269189627)) ;
#96198=DIRECTION('center_axis',(0.,1.,0.)) ;
#96199=DIRECTION('ref_axis',(0.,0.,1.)) ;
#96200=DIRECTION('',(0.,0.,1.)) ;
#96201=DIRECTION('',(-1.,0.,-9.8563833862319E-18)) ;
#96202=DIRECTION('',(0.,0.,-1.)) ;
#96203=DIRECTION('',(1.,0.,-9.8563833862319E-18)) ;
#96204=DIRECTION('center_axis',(-0.707106781186548,0.707106781186548,0.)) ;
#96205=DIRECTION('ref_axis',(-0.707106781186548,-0.707106781186548,0.)) ;
#96206=DIRECTION('',(0.,0.,1.)) ;
#96207=DIRECTION('',(-0.577350269189625,-0.577350269189625,-0.577350269189627)) ;
#96208=DIRECTION('',(0.,0.,-1.)) ;
#96209=DIRECTION('',(0.577350269189625,0.577350269189625,-0.577350269189627)) ;
#96210=DIRECTION('center_axis',(-1.,9.85638338623186E-18,0.)) ;
#96211=DIRECTION('ref_axis',(-9.85638338623186E-18,-1.,0.)) ;
#96212=DIRECTION('',(0.,0.,-1.)) ;
#96213=DIRECTION('',(9.85638338623186E-18,1.,0.)) ;
#96214=DIRECTION('',(0.,0.,-1.)) ;
#96215=DIRECTION('',(-9.85638338623186E-18,-1.,0.)) ;
#96216=DIRECTION('center_axis',(0.,0.,1.)) ;
#96217=DIRECTION('ref_axis',(1.,0.,0.)) ;
#96218=DIRECTION('',(9.85638338623186E-18,1.,0.)) ;
#96219=DIRECTION('center_axis',(0.,0.,-1.)) ;
#96220=DIRECTION('ref_axis',(1.,0.,0.)) ;
#96221=DIRECTION('center_axis',(0.,0.,1.)) ;
#96222=DIRECTION('ref_axis',(1.,0.,0.)) ;
#96223=DIRECTION('',(-9.85638338623186E-18,-1.,0.)) ;
#96224=DIRECTION('',(1.,-9.85638338623186E-18,0.)) ;
#96225=DIRECTION('center_axis',(0.,0.,1.)) ;
#96226=DIRECTION('ref_axis',(1.,0.,0.)) ;
#96227=DIRECTION('',(9.85638338623186E-18,1.,0.)) ;
#96228=DIRECTION('center_axis',(0.,0.,-1.)) ;
#96229=DIRECTION('ref_axis',(1.,0.,0.)) ;
#96230=DIRECTION('center_axis',(0.,0.,1.)) ;
#96231=DIRECTION('ref_axis',(1.,0.,0.)) ;
#96232=DIRECTION('',(-9.85638338623186E-18,-1.,0.)) ;
#96233=DIRECTION('',(-1.,9.85638338623186E-18,0.)) ;
#96234=DIRECTION('center_axis',(0.,0.,-1.)) ;
#96235=DIRECTION('ref_axis',(-1.,0.,0.)) ;
#96236=DIRECTION('center_axis',(0.,0.,1.)) ;
#96237=DIRECTION('ref_axis',(1.,0.,0.)) ;
#96238=DIRECTION('center_axis',(0.,0.,-1.)) ;
#96239=DIRECTION('ref_axis',(1.,0.,0.)) ;
#96240=DIRECTION('center_axis',(0.,0.,-1.)) ;
#96241=DIRECTION('ref_axis',(-1.,0.,0.)) ;
#96242=DIRECTION('center_axis',(0.,0.,-1.)) ;
#96243=DIRECTION('ref_axis',(1.,0.,0.)) ;
#96244=DIRECTION('center_axis',(0.,0.,1.)) ;
#96245=DIRECTION('ref_axis',(1.,0.,0.)) ;
#96246=DIRECTION('center_axis',(-0.707106781186548,-0.707106781186547,0.)) ;
#96247=DIRECTION('ref_axis',(0.707106781186547,-0.707106781186548,0.)) ;
#96248=DIRECTION('',(0.,0.,1.)) ;
#96249=DIRECTION('',(0.577350269189625,-0.577350269189626,-0.577350269189626)) ;
#96250=DIRECTION('',(0.,0.,-1.)) ;
#96251=DIRECTION('',(-0.577350269189625,0.577350269189626,-0.577350269189626)) ;
#96252=DIRECTION('center_axis',(1.95511867169517E-16,-1.,0.)) ;
#96253=DIRECTION('ref_axis',(1.,1.95511867169517E-16,0.)) ;
#96254=DIRECTION('',(0.,0.,-1.)) ;
#96255=DIRECTION('',(-1.,-1.95511867169517E-16,0.)) ;
#96256=DIRECTION('',(1.,1.95511867169517E-16,0.)) ;
#96257=DIRECTION('center_axis',(1.06642836637918E-16,1.,0.)) ;
#96258=DIRECTION('ref_axis',(-1.,1.06642836637918E-16,0.)) ;
#96259=DIRECTION('',(1.,-1.06642836637919E-16,0.)) ;
#96260=DIRECTION('',(0.,0.,1.)) ;
#96261=DIRECTION('',(-1.,1.06642836637919E-16,0.)) ;
#96262=DIRECTION('center_axis',(-0.707106781186548,0.707106781186547,0.)) ;
#96263=DIRECTION('ref_axis',(-0.707106781186547,-0.707106781186548,0.)) ;
#96264=DIRECTION('',(0.,0.,1.)) ;
#96265=DIRECTION('',(-0.577350269189625,-0.577350269189626,0.577350269189627)) ;
#96266=DIRECTION('',(0.,0.,-1.)) ;
#96267=DIRECTION('',(0.577350269189625,0.577350269189626,0.577350269189627)) ;
#96268=DIRECTION('center_axis',(-1.,0.,0.)) ;
#96269=DIRECTION('ref_axis',(0.,0.,1.)) ;
#96270=DIRECTION('',(0.,0.,-1.)) ;
#96271=DIRECTION('',(0.,1.,1.95511867169518E-16)) ;
#96272=DIRECTION('',(0.,0.,1.)) ;
#96273=DIRECTION('',(0.,-1.,1.95511867169518E-16)) ;
#96274=DIRECTION('center_axis',(0.,0.,1.)) ;
#96275=DIRECTION('ref_axis',(1.,0.,0.)) ;
#96276=DIRECTION('',(-1.95511867169517E-16,1.,0.)) ;
#96277=DIRECTION('',(-1.,-1.95511867169517E-16,0.)) ;
#96278=DIRECTION('',(1.,-1.06642836637919E-16,0.)) ;
#96279=DIRECTION('center_axis',(0.,0.,1.)) ;
#96280=DIRECTION('ref_axis',(1.,0.,0.)) ;
#96281=DIRECTION('',(1.,1.95511867169517E-16,0.)) ;
#96282=DIRECTION('',(1.95511867169517E-16,-1.,0.)) ;
#96283=DIRECTION('',(-1.,1.06642836637919E-16,0.)) ;
#96284=DIRECTION('center_axis',(1.,-9.85638338623186E-18,0.)) ;
#96285=DIRECTION('ref_axis',(9.85638338623186E-18,1.,0.)) ;
#96286=DIRECTION('',(0.,0.,-1.)) ;
#96287=DIRECTION('',(-9.85638338623186E-18,-1.,0.)) ;
#96288=DIRECTION('',(0.,0.,1.)) ;
#96289=DIRECTION('',(9.85638338623186E-18,1.,0.)) ;
#96290=DIRECTION('center_axis',(0.707106781186548,0.707106781186548,0.)) ;
#96291=DIRECTION('ref_axis',(-0.707106781186548,0.707106781186548,0.)) ;
#96292=DIRECTION('',(0.,0.,1.)) ;
#96293=DIRECTION('',(-0.577350269189625,0.577350269189625,0.577350269189627)) ;
#96294=DIRECTION('',(0.,0.,-1.)) ;
#96295=DIRECTION('',(0.577350269189625,-0.577350269189625,0.577350269189627)) ;
#96296=DIRECTION('center_axis',(0.,1.,0.)) ;
#96297=DIRECTION('ref_axis',(0.,0.,1.)) ;
#96298=DIRECTION('',(0.,0.,1.)) ;
#96299=DIRECTION('',(-1.,0.,-9.8563833862319E-18)) ;
#96300=DIRECTION('',(0.,0.,-1.)) ;
#96301=DIRECTION('',(1.,0.,-9.8563833862319E-18)) ;
#96302=DIRECTION('center_axis',(-0.707106781186548,0.707106781186548,0.)) ;
#96303=DIRECTION('ref_axis',(-0.707106781186548,-0.707106781186548,0.)) ;
#96304=DIRECTION('',(0.,0.,1.)) ;
#96305=DIRECTION('',(-0.577350269189625,-0.577350269189625,-0.577350269189627)) ;
#96306=DIRECTION('',(0.,0.,-1.)) ;
#96307=DIRECTION('',(0.577350269189625,0.577350269189625,-0.577350269189627)) ;
#96308=DIRECTION('center_axis',(-1.,9.85638338623186E-18,0.)) ;
#96309=DIRECTION('ref_axis',(-9.85638338623186E-18,-1.,0.)) ;
#96310=DIRECTION('',(0.,0.,-1.)) ;
#96311=DIRECTION('',(9.85638338623186E-18,1.,0.)) ;
#96312=DIRECTION('',(0.,0.,-1.)) ;
#96313=DIRECTION('',(-9.85638338623186E-18,-1.,0.)) ;
#96314=DIRECTION('center_axis',(0.,0.,1.)) ;
#96315=DIRECTION('ref_axis',(1.,0.,0.)) ;
#96316=DIRECTION('',(9.85638338623186E-18,1.,0.)) ;
#96317=DIRECTION('center_axis',(0.,0.,-1.)) ;
#96318=DIRECTION('ref_axis',(1.,0.,0.)) ;
#96319=DIRECTION('center_axis',(0.,0.,1.)) ;
#96320=DIRECTION('ref_axis',(1.,0.,0.)) ;
#96321=DIRECTION('',(-9.85638338623186E-18,-1.,0.)) ;
#96322=DIRECTION('',(1.,-9.85638338623186E-18,0.)) ;
#96323=DIRECTION('center_axis',(0.,0.,1.)) ;
#96324=DIRECTION('ref_axis',(1.,0.,0.)) ;
#96325=DIRECTION('',(9.85638338623186E-18,1.,0.)) ;
#96326=DIRECTION('center_axis',(0.,0.,-1.)) ;
#96327=DIRECTION('ref_axis',(1.,0.,0.)) ;
#96328=DIRECTION('center_axis',(0.,0.,1.)) ;
#96329=DIRECTION('ref_axis',(1.,0.,0.)) ;
#96330=DIRECTION('',(-9.85638338623186E-18,-1.,0.)) ;
#96331=DIRECTION('',(-1.,9.85638338623186E-18,0.)) ;
#96332=DIRECTION('center_axis',(0.,0.,-1.)) ;
#96333=DIRECTION('ref_axis',(-1.,0.,0.)) ;
#96334=DIRECTION('center_axis',(0.,0.,1.)) ;
#96335=DIRECTION('ref_axis',(1.,0.,0.)) ;
#96336=DIRECTION('center_axis',(0.,0.,-1.)) ;
#96337=DIRECTION('ref_axis',(1.,0.,0.)) ;
#96338=DIRECTION('center_axis',(0.,0.,-1.)) ;
#96339=DIRECTION('ref_axis',(-1.,0.,0.)) ;
#96340=DIRECTION('center_axis',(0.,0.,-1.)) ;
#96341=DIRECTION('ref_axis',(1.,0.,0.)) ;
#96342=DIRECTION('center_axis',(0.,0.,1.)) ;
#96343=DIRECTION('ref_axis',(1.,0.,0.)) ;
#96344=DIRECTION('center_axis',(-0.707106781186548,-0.707106781186547,0.)) ;
#96345=DIRECTION('ref_axis',(0.707106781186547,-0.707106781186548,0.)) ;
#96346=DIRECTION('',(0.,0.,1.)) ;
#96347=DIRECTION('',(0.577350269189625,-0.577350269189626,-0.577350269189626)) ;
#96348=DIRECTION('',(0.,0.,-1.)) ;
#96349=DIRECTION('',(-0.577350269189625,0.577350269189626,-0.577350269189626)) ;
#96350=DIRECTION('center_axis',(1.95511867169517E-16,-1.,0.)) ;
#96351=DIRECTION('ref_axis',(1.,1.95511867169517E-16,0.)) ;
#96352=DIRECTION('',(0.,0.,-1.)) ;
#96353=DIRECTION('',(-1.,-1.95511867169517E-16,0.)) ;
#96354=DIRECTION('',(1.,1.95511867169517E-16,0.)) ;
#96355=DIRECTION('center_axis',(1.06642836637918E-16,1.,0.)) ;
#96356=DIRECTION('ref_axis',(-1.,1.06642836637918E-16,0.)) ;
#96357=DIRECTION('',(1.,-1.06642836637919E-16,0.)) ;
#96358=DIRECTION('',(0.,0.,1.)) ;
#96359=DIRECTION('',(-1.,1.06642836637919E-16,0.)) ;
#96360=DIRECTION('center_axis',(-0.707106781186548,0.707106781186547,0.)) ;
#96361=DIRECTION('ref_axis',(-0.707106781186547,-0.707106781186548,0.)) ;
#96362=DIRECTION('',(0.,0.,1.)) ;
#96363=DIRECTION('',(-0.577350269189625,-0.577350269189626,0.577350269189627)) ;
#96364=DIRECTION('',(0.,0.,-1.)) ;
#96365=DIRECTION('',(0.577350269189625,0.577350269189626,0.577350269189627)) ;
#96366=DIRECTION('center_axis',(-1.,0.,0.)) ;
#96367=DIRECTION('ref_axis',(0.,0.,1.)) ;
#96368=DIRECTION('',(0.,0.,-1.)) ;
#96369=DIRECTION('',(0.,1.,1.95511867169518E-16)) ;
#96370=DIRECTION('',(0.,0.,1.)) ;
#96371=DIRECTION('',(0.,-1.,1.95511867169518E-16)) ;
#96372=DIRECTION('center_axis',(0.,0.,1.)) ;
#96373=DIRECTION('ref_axis',(1.,0.,0.)) ;
#96374=DIRECTION('',(-1.95511867169517E-16,1.,0.)) ;
#96375=DIRECTION('',(-1.,-1.95511867169517E-16,0.)) ;
#96376=DIRECTION('',(1.,-1.06642836637919E-16,0.)) ;
#96377=DIRECTION('center_axis',(0.,0.,1.)) ;
#96378=DIRECTION('ref_axis',(1.,0.,0.)) ;
#96379=DIRECTION('',(1.,1.95511867169517E-16,0.)) ;
#96380=DIRECTION('',(1.95511867169517E-16,-1.,0.)) ;
#96381=DIRECTION('',(-1.,1.06642836637919E-16,0.)) ;
#96382=DIRECTION('center_axis',(1.,-9.85638338623186E-18,0.)) ;
#96383=DIRECTION('ref_axis',(9.85638338623186E-18,1.,0.)) ;
#96384=DIRECTION('',(0.,0.,-1.)) ;
#96385=DIRECTION('',(-9.85638338623186E-18,-1.,0.)) ;
#96386=DIRECTION('',(0.,0.,1.)) ;
#96387=DIRECTION('',(9.85638338623186E-18,1.,0.)) ;
#96388=DIRECTION('center_axis',(0.707106781186548,0.707106781186548,0.)) ;
#96389=DIRECTION('ref_axis',(-0.707106781186548,0.707106781186548,0.)) ;
#96390=DIRECTION('',(0.,0.,1.)) ;
#96391=DIRECTION('',(-0.577350269189625,0.577350269189625,0.577350269189627)) ;
#96392=DIRECTION('',(0.,0.,-1.)) ;
#96393=DIRECTION('',(0.577350269189625,-0.577350269189625,0.577350269189627)) ;
#96394=DIRECTION('center_axis',(0.,1.,0.)) ;
#96395=DIRECTION('ref_axis',(0.,0.,1.)) ;
#96396=DIRECTION('',(0.,0.,1.)) ;
#96397=DIRECTION('',(-1.,0.,-9.8563833862319E-18)) ;
#96398=DIRECTION('',(0.,0.,-1.)) ;
#96399=DIRECTION('',(1.,0.,-9.8563833862319E-18)) ;
#96400=DIRECTION('center_axis',(-0.707106781186548,0.707106781186548,0.)) ;
#96401=DIRECTION('ref_axis',(-0.707106781186548,-0.707106781186548,0.)) ;
#96402=DIRECTION('',(0.,0.,1.)) ;
#96403=DIRECTION('',(-0.577350269189625,-0.577350269189625,-0.577350269189627)) ;
#96404=DIRECTION('',(0.,0.,-1.)) ;
#96405=DIRECTION('',(0.577350269189625,0.577350269189625,-0.577350269189627)) ;
#96406=DIRECTION('center_axis',(-1.,9.85638338623186E-18,0.)) ;
#96407=DIRECTION('ref_axis',(-9.85638338623186E-18,-1.,0.)) ;
#96408=DIRECTION('',(0.,0.,-1.)) ;
#96409=DIRECTION('',(9.85638338623186E-18,1.,0.)) ;
#96410=DIRECTION('',(0.,0.,-1.)) ;
#96411=DIRECTION('',(-9.85638338623186E-18,-1.,0.)) ;
#96412=DIRECTION('center_axis',(0.,0.,1.)) ;
#96413=DIRECTION('ref_axis',(1.,0.,0.)) ;
#96414=DIRECTION('',(9.85638338623186E-18,1.,0.)) ;
#96415=DIRECTION('center_axis',(0.,0.,-1.)) ;
#96416=DIRECTION('ref_axis',(1.,0.,0.)) ;
#96417=DIRECTION('center_axis',(0.,0.,1.)) ;
#96418=DIRECTION('ref_axis',(1.,0.,0.)) ;
#96419=DIRECTION('',(-9.85638338623186E-18,-1.,0.)) ;
#96420=DIRECTION('',(1.,-9.85638338623186E-18,0.)) ;
#96421=DIRECTION('center_axis',(0.,0.,1.)) ;
#96422=DIRECTION('ref_axis',(1.,0.,0.)) ;
#96423=DIRECTION('',(9.85638338623186E-18,1.,0.)) ;
#96424=DIRECTION('center_axis',(0.,0.,-1.)) ;
#96425=DIRECTION('ref_axis',(1.,0.,0.)) ;
#96426=DIRECTION('center_axis',(0.,0.,1.)) ;
#96427=DIRECTION('ref_axis',(1.,0.,0.)) ;
#96428=DIRECTION('',(-9.85638338623186E-18,-1.,0.)) ;
#96429=DIRECTION('',(-1.,9.85638338623186E-18,0.)) ;
#96430=DIRECTION('center_axis',(0.,0.,-1.)) ;
#96431=DIRECTION('ref_axis',(-1.,0.,0.)) ;
#96432=DIRECTION('center_axis',(0.,0.,1.)) ;
#96433=DIRECTION('ref_axis',(1.,0.,0.)) ;
#96434=DIRECTION('center_axis',(0.,0.,-1.)) ;
#96435=DIRECTION('ref_axis',(1.,0.,0.)) ;
#96436=DIRECTION('center_axis',(0.,0.,-1.)) ;
#96437=DIRECTION('ref_axis',(-1.,0.,0.)) ;
#96438=DIRECTION('center_axis',(0.,0.,-1.)) ;
#96439=DIRECTION('ref_axis',(1.,0.,0.)) ;
#96440=DIRECTION('center_axis',(0.,0.,1.)) ;
#96441=DIRECTION('ref_axis',(1.,0.,0.)) ;
#96442=DIRECTION('center_axis',(-0.707106781186548,-0.707106781186547,0.)) ;
#96443=DIRECTION('ref_axis',(0.707106781186547,-0.707106781186548,0.)) ;
#96444=DIRECTION('',(0.,0.,1.)) ;
#96445=DIRECTION('',(0.577350269189625,-0.577350269189626,-0.577350269189626)) ;
#96446=DIRECTION('',(0.,0.,-1.)) ;
#96447=DIRECTION('',(-0.577350269189625,0.577350269189626,-0.577350269189626)) ;
#96448=DIRECTION('center_axis',(1.95511867169517E-16,-1.,0.)) ;
#96449=DIRECTION('ref_axis',(1.,1.95511867169517E-16,0.)) ;
#96450=DIRECTION('',(0.,0.,-1.)) ;
#96451=DIRECTION('',(-1.,-1.95511867169517E-16,0.)) ;
#96452=DIRECTION('',(1.,1.95511867169517E-16,0.)) ;
#96453=DIRECTION('center_axis',(1.06642836637918E-16,1.,0.)) ;
#96454=DIRECTION('ref_axis',(-1.,1.06642836637918E-16,0.)) ;
#96455=DIRECTION('',(1.,-1.06642836637919E-16,0.)) ;
#96456=DIRECTION('',(0.,0.,1.)) ;
#96457=DIRECTION('',(-1.,1.06642836637919E-16,0.)) ;
#96458=DIRECTION('center_axis',(-0.707106781186548,0.707106781186547,0.)) ;
#96459=DIRECTION('ref_axis',(-0.707106781186547,-0.707106781186548,0.)) ;
#96460=DIRECTION('',(0.,0.,1.)) ;
#96461=DIRECTION('',(-0.577350269189625,-0.577350269189626,0.577350269189627)) ;
#96462=DIRECTION('',(0.,0.,-1.)) ;
#96463=DIRECTION('',(0.577350269189625,0.577350269189626,0.577350269189627)) ;
#96464=DIRECTION('center_axis',(-1.,0.,0.)) ;
#96465=DIRECTION('ref_axis',(0.,0.,1.)) ;
#96466=DIRECTION('',(0.,0.,-1.)) ;
#96467=DIRECTION('',(0.,1.,1.95511867169518E-16)) ;
#96468=DIRECTION('',(0.,0.,1.)) ;
#96469=DIRECTION('',(0.,-1.,1.95511867169518E-16)) ;
#96470=DIRECTION('center_axis',(0.,0.,1.)) ;
#96471=DIRECTION('ref_axis',(1.,0.,0.)) ;
#96472=DIRECTION('',(-1.95511867169517E-16,1.,0.)) ;
#96473=DIRECTION('',(-1.,-1.95511867169517E-16,0.)) ;
#96474=DIRECTION('',(1.,-1.06642836637919E-16,0.)) ;
#96475=DIRECTION('center_axis',(0.,0.,1.)) ;
#96476=DIRECTION('ref_axis',(1.,0.,0.)) ;
#96477=DIRECTION('',(1.,1.95511867169517E-16,0.)) ;
#96478=DIRECTION('',(1.95511867169517E-16,-1.,0.)) ;
#96479=DIRECTION('',(-1.,1.06642836637919E-16,0.)) ;
#96480=DIRECTION('center_axis',(6.96951553037899E-18,0.707106781186549,
0.707106781186546)) ;
#96481=DIRECTION('ref_axis',(-8.6424177776148E-34,-0.707106781186546,0.707106781186549)) ;
#96482=DIRECTION('',(-0.577350269189625,0.577350269189625,-0.577350269189627)) ;
#96483=DIRECTION('',(1.,-9.85638338623186E-18,0.)) ;
#96484=DIRECTION('',(-0.577350269189625,-0.577350269189625,0.577350269189627)) ;
#96485=DIRECTION('',(-1.,7.70371977754894E-34,9.8563833862319E-18)) ;
#96486=DIRECTION('center_axis',(6.96951553037899E-18,0.707106781186549,
-0.707106781186546)) ;
#96487=DIRECTION('ref_axis',(8.6424177776148E-34,0.707106781186546,0.707106781186549)) ;
#96488=DIRECTION('',(0.577350269189625,0.577350269189625,0.577350269189627)) ;
#96489=DIRECTION('',(-1.,9.85638338623186E-18,0.)) ;
#96490=DIRECTION('',(0.577350269189625,-0.577350269189625,-0.577350269189627)) ;
#96491=DIRECTION('',(1.,-7.70371977754894E-34,9.8563833862319E-18)) ;
#96492=DIRECTION('center_axis',(6.96951553037899E-18,0.707106781186549,
0.707106781186546)) ;
#96493=DIRECTION('ref_axis',(-8.6424177776148E-34,-0.707106781186546,0.707106781186549)) ;
#96494=DIRECTION('',(-0.577350269189625,0.577350269189625,-0.577350269189627)) ;
#96495=DIRECTION('',(1.,-9.85638338623186E-18,0.)) ;
#96496=DIRECTION('',(-0.577350269189625,-0.577350269189625,0.577350269189627)) ;
#96497=DIRECTION('',(-1.,7.70371977754894E-34,9.8563833862319E-18)) ;
#96498=DIRECTION('center_axis',(6.96951553037899E-18,0.707106781186549,
-0.707106781186546)) ;
#96499=DIRECTION('ref_axis',(8.6424177776148E-34,0.707106781186546,0.707106781186549)) ;
#96500=DIRECTION('',(0.577350269189625,0.577350269189625,0.577350269189627)) ;
#96501=DIRECTION('',(-1.,9.85638338623186E-18,0.)) ;
#96502=DIRECTION('',(0.577350269189625,-0.577350269189625,-0.577350269189627)) ;
#96503=DIRECTION('',(1.,-7.70371977754894E-34,9.8563833862319E-18)) ;
#96504=DIRECTION('center_axis',(6.96951553037899E-18,0.707106781186549,
0.707106781186546)) ;
#96505=DIRECTION('ref_axis',(-8.6424177776148E-34,-0.707106781186546,0.707106781186549)) ;
#96506=DIRECTION('',(-0.577350269189625,0.577350269189625,-0.577350269189627)) ;
#96507=DIRECTION('',(1.,-9.85638338623186E-18,0.)) ;
#96508=DIRECTION('',(-0.577350269189625,-0.577350269189625,0.577350269189627)) ;
#96509=DIRECTION('',(-1.,7.70371977754894E-34,9.8563833862319E-18)) ;
#96510=DIRECTION('center_axis',(6.96951553037899E-18,0.707106781186549,
-0.707106781186546)) ;
#96511=DIRECTION('ref_axis',(8.6424177776148E-34,0.707106781186546,0.707106781186549)) ;
#96512=DIRECTION('',(0.577350269189625,0.577350269189625,0.577350269189627)) ;
#96513=DIRECTION('',(-1.,9.85638338623186E-18,0.)) ;
#96514=DIRECTION('',(0.577350269189625,-0.577350269189625,-0.577350269189627)) ;
#96515=DIRECTION('',(1.,-7.70371977754894E-34,9.8563833862319E-18)) ;
#96516=DIRECTION('center_axis',(6.96951553037899E-18,0.707106781186549,
0.707106781186546)) ;
#96517=DIRECTION('ref_axis',(-8.6424177776148E-34,-0.707106781186546,0.707106781186549)) ;
#96518=DIRECTION('',(-0.577350269189625,0.577350269189625,-0.577350269189627)) ;
#96519=DIRECTION('',(1.,-9.85638338623186E-18,0.)) ;
#96520=DIRECTION('',(-0.577350269189625,-0.577350269189625,0.577350269189627)) ;
#96521=DIRECTION('',(-1.,7.70371977754894E-34,9.8563833862319E-18)) ;
#96522=DIRECTION('center_axis',(6.96951553037899E-18,0.707106781186549,
-0.707106781186546)) ;
#96523=DIRECTION('ref_axis',(8.6424177776148E-34,0.707106781186546,0.707106781186549)) ;
#96524=DIRECTION('',(0.577350269189625,0.577350269189625,0.577350269189627)) ;
#96525=DIRECTION('',(-1.,9.85638338623186E-18,0.)) ;
#96526=DIRECTION('',(0.577350269189625,-0.577350269189625,-0.577350269189627)) ;
#96527=DIRECTION('',(1.,-7.70371977754894E-34,9.8563833862319E-18)) ;
#96528=DIRECTION('center_axis',(6.96951553037899E-18,0.707106781186549,
0.707106781186546)) ;
#96529=DIRECTION('ref_axis',(-8.6424177776148E-34,-0.707106781186546,0.707106781186549)) ;
#96530=DIRECTION('',(-0.577350269189625,0.577350269189625,-0.577350269189627)) ;
#96531=DIRECTION('',(1.,-9.85638338623186E-18,0.)) ;
#96532=DIRECTION('',(-0.577350269189625,-0.577350269189625,0.577350269189627)) ;
#96533=DIRECTION('',(-1.,7.70371977754894E-34,9.8563833862319E-18)) ;
#96534=DIRECTION('center_axis',(6.96951553037899E-18,0.707106781186549,
-0.707106781186546)) ;
#96535=DIRECTION('ref_axis',(8.6424177776148E-34,0.707106781186546,0.707106781186549)) ;
#96536=DIRECTION('',(0.577350269189625,0.577350269189625,0.577350269189627)) ;
#96537=DIRECTION('',(-1.,9.85638338623186E-18,0.)) ;
#96538=DIRECTION('',(0.577350269189625,-0.577350269189625,-0.577350269189627)) ;
#96539=DIRECTION('',(1.,-7.70371977754894E-34,9.8563833862319E-18)) ;
#96540=DIRECTION('center_axis',(6.96951553037899E-18,0.707106781186549,
0.707106781186546)) ;
#96541=DIRECTION('ref_axis',(-8.6424177776148E-34,-0.707106781186546,0.707106781186549)) ;
#96542=DIRECTION('',(-0.577350269189625,0.577350269189625,-0.577350269189627)) ;
#96543=DIRECTION('',(1.,-9.85638338623186E-18,0.)) ;
#96544=DIRECTION('',(-0.577350269189625,-0.577350269189625,0.577350269189627)) ;
#96545=DIRECTION('',(-1.,7.70371977754894E-34,9.8563833862319E-18)) ;
#96546=DIRECTION('center_axis',(6.96951553037899E-18,0.707106781186549,
-0.707106781186546)) ;
#96547=DIRECTION('ref_axis',(8.6424177776148E-34,0.707106781186546,0.707106781186549)) ;
#96548=DIRECTION('',(0.577350269189625,0.577350269189625,0.577350269189627)) ;
#96549=DIRECTION('',(-1.,9.85638338623186E-18,0.)) ;
#96550=DIRECTION('',(0.577350269189625,-0.577350269189625,-0.577350269189627)) ;
#96551=DIRECTION('',(1.,-7.70371977754894E-34,9.8563833862319E-18)) ;
#96552=DIRECTION('center_axis',(6.96951553037899E-18,0.707106781186549,
0.707106781186546)) ;
#96553=DIRECTION('ref_axis',(-8.6424177776148E-34,-0.707106781186546,0.707106781186549)) ;
#96554=DIRECTION('',(-0.577350269189625,0.577350269189625,-0.577350269189627)) ;
#96555=DIRECTION('',(1.,-9.85638338623186E-18,0.)) ;
#96556=DIRECTION('',(-0.577350269189625,-0.577350269189625,0.577350269189627)) ;
#96557=DIRECTION('',(-1.,7.70371977754894E-34,9.8563833862319E-18)) ;
#96558=DIRECTION('center_axis',(6.96951553037899E-18,0.707106781186549,
-0.707106781186546)) ;
#96559=DIRECTION('ref_axis',(8.6424177776148E-34,0.707106781186546,0.707106781186549)) ;
#96560=DIRECTION('',(0.577350269189625,0.577350269189625,0.577350269189627)) ;
#96561=DIRECTION('',(-1.,9.85638338623186E-18,0.)) ;
#96562=DIRECTION('',(0.577350269189625,-0.577350269189625,-0.577350269189627)) ;
#96563=DIRECTION('',(1.,-7.70371977754894E-34,9.8563833862319E-18)) ;
#96564=DIRECTION('center_axis',(6.96951553037899E-18,0.707106781186549,
0.707106781186546)) ;
#96565=DIRECTION('ref_axis',(-8.6424177776148E-34,-0.707106781186546,0.707106781186549)) ;
#96566=DIRECTION('',(-0.577350269189625,0.577350269189625,-0.577350269189627)) ;
#96567=DIRECTION('',(1.,-9.85638338623186E-18,0.)) ;
#96568=DIRECTION('',(-0.577350269189625,-0.577350269189625,0.577350269189627)) ;
#96569=DIRECTION('',(-1.,7.70371977754894E-34,9.8563833862319E-18)) ;
#96570=DIRECTION('center_axis',(6.96951553037899E-18,0.707106781186549,
-0.707106781186546)) ;
#96571=DIRECTION('ref_axis',(8.6424177776148E-34,0.707106781186546,0.707106781186549)) ;
#96572=DIRECTION('',(0.577350269189625,0.577350269189625,0.577350269189627)) ;
#96573=DIRECTION('',(-1.,9.85638338623186E-18,0.)) ;
#96574=DIRECTION('',(0.577350269189625,-0.577350269189625,-0.577350269189627)) ;
#96575=DIRECTION('',(1.,-7.70371977754894E-34,9.8563833862319E-18)) ;
#96576=DIRECTION('center_axis',(6.96951553037899E-18,0.707106781186549,
0.707106781186546)) ;
#96577=DIRECTION('ref_axis',(-8.6424177776148E-34,-0.707106781186546,0.707106781186549)) ;
#96578=DIRECTION('',(-0.577350269189625,0.577350269189625,-0.577350269189627)) ;
#96579=DIRECTION('',(1.,-9.85638338623186E-18,0.)) ;
#96580=DIRECTION('',(-0.577350269189625,-0.577350269189625,0.577350269189627)) ;
#96581=DIRECTION('',(-1.,7.70371977754894E-34,9.8563833862319E-18)) ;
#96582=DIRECTION('center_axis',(6.96951553037899E-18,0.707106781186549,
-0.707106781186546)) ;
#96583=DIRECTION('ref_axis',(8.6424177776148E-34,0.707106781186546,0.707106781186549)) ;
#96584=DIRECTION('',(0.577350269189625,0.577350269189625,0.577350269189627)) ;
#96585=DIRECTION('',(-1.,9.85638338623186E-18,0.)) ;
#96586=DIRECTION('',(0.577350269189625,-0.577350269189625,-0.577350269189627)) ;
#96587=DIRECTION('',(1.,-7.70371977754894E-34,9.8563833862319E-18)) ;
#96588=DIRECTION('center_axis',(-0.707106781186548,-1.38247767078009E-16,
0.707106781186547)) ;
#96589=DIRECTION('ref_axis',(0.707106781186547,8.815972061965E-34,0.707106781186548)) ;
#96590=DIRECTION('',(-0.577350269189625,-0.577350269189626,-0.577350269189626)) ;
#96591=DIRECTION('',(-1.95511867169517E-16,1.,0.)) ;
#96592=DIRECTION('',(0.577350269189625,-0.577350269189626,0.577350269189626)) ;
#96593=DIRECTION('',(0.,-1.,-1.95511867169518E-16)) ;
#96594=DIRECTION('center_axis',(-0.707106781186548,-1.38247767078009E-16,
-0.707106781186547)) ;
#96595=DIRECTION('ref_axis',(-0.707106781186547,-8.815972061965E-34,0.707106781186548)) ;
#96596=DIRECTION('',(-0.577350269189625,0.577350269189626,0.577350269189626)) ;
#96597=DIRECTION('',(1.95511867169517E-16,-1.,0.)) ;
#96598=DIRECTION('',(0.577350269189625,0.577350269189626,-0.577350269189626)) ;
#96599=DIRECTION('',(0.,1.,-1.95511867169518E-16)) ;
#96600=DIRECTION('center_axis',(-0.707106781186548,-1.38247767078009E-16,
0.707106781186547)) ;
#96601=DIRECTION('ref_axis',(0.707106781186547,8.815972061965E-34,0.707106781186548)) ;
#96602=DIRECTION('',(-0.577350269189625,-0.577350269189626,-0.577350269189626)) ;
#96603=DIRECTION('',(-1.95511867169517E-16,1.,0.)) ;
#96604=DIRECTION('',(0.577350269189625,-0.577350269189626,0.577350269189626)) ;
#96605=DIRECTION('',(0.,-1.,-1.95511867169518E-16)) ;
#96606=DIRECTION('center_axis',(-0.707106781186548,-1.38247767078009E-16,
-0.707106781186547)) ;
#96607=DIRECTION('ref_axis',(-0.707106781186547,-8.815972061965E-34,0.707106781186548)) ;
#96608=DIRECTION('',(-0.577350269189625,0.577350269189626,0.577350269189626)) ;
#96609=DIRECTION('',(1.95511867169517E-16,-1.,0.)) ;
#96610=DIRECTION('',(0.577350269189625,0.577350269189626,-0.577350269189626)) ;
#96611=DIRECTION('',(0.,1.,-1.95511867169518E-16)) ;
#96612=DIRECTION('center_axis',(-0.707106781186548,-1.38247767078009E-16,
0.707106781186547)) ;
#96613=DIRECTION('ref_axis',(0.707106781186547,8.815972061965E-34,0.707106781186548)) ;
#96614=DIRECTION('',(-0.577350269189625,-0.577350269189626,-0.577350269189626)) ;
#96615=DIRECTION('',(-1.95511867169517E-16,1.,0.)) ;
#96616=DIRECTION('',(0.577350269189625,-0.577350269189626,0.577350269189626)) ;
#96617=DIRECTION('',(0.,-1.,-1.95511867169518E-16)) ;
#96618=DIRECTION('center_axis',(-0.707106781186548,-1.38247767078009E-16,
-0.707106781186547)) ;
#96619=DIRECTION('ref_axis',(-0.707106781186547,-8.815972061965E-34,0.707106781186548)) ;
#96620=DIRECTION('',(-0.577350269189625,0.577350269189626,0.577350269189626)) ;
#96621=DIRECTION('',(1.95511867169517E-16,-1.,0.)) ;
#96622=DIRECTION('',(0.577350269189625,0.577350269189626,-0.577350269189626)) ;
#96623=DIRECTION('',(0.,1.,-1.95511867169518E-16)) ;
#96624=DIRECTION('center_axis',(-0.707106781186548,-1.38247767078009E-16,
0.707106781186547)) ;
#96625=DIRECTION('ref_axis',(0.707106781186547,8.815972061965E-34,0.707106781186548)) ;
#96626=DIRECTION('',(-0.577350269189625,-0.577350269189626,-0.577350269189626)) ;
#96627=DIRECTION('',(-1.95511867169517E-16,1.,0.)) ;
#96628=DIRECTION('',(0.577350269189625,-0.577350269189626,0.577350269189626)) ;
#96629=DIRECTION('',(0.,-1.,-1.95511867169518E-16)) ;
#96630=DIRECTION('center_axis',(-0.707106781186548,-1.38247767078009E-16,
-0.707106781186547)) ;
#96631=DIRECTION('ref_axis',(-0.707106781186547,-8.815972061965E-34,0.707106781186548)) ;
#96632=DIRECTION('',(-0.577350269189625,0.577350269189626,0.577350269189626)) ;
#96633=DIRECTION('',(1.95511867169517E-16,-1.,0.)) ;
#96634=DIRECTION('',(0.577350269189625,0.577350269189626,-0.577350269189626)) ;
#96635=DIRECTION('',(0.,1.,-1.95511867169518E-16)) ;
#96636=DIRECTION('center_axis',(-0.707106781186548,-1.38247767078009E-16,
0.707106781186547)) ;
#96637=DIRECTION('ref_axis',(0.707106781186547,8.815972061965E-34,0.707106781186548)) ;
#96638=DIRECTION('',(-0.577350269189625,-0.577350269189626,-0.577350269189626)) ;
#96639=DIRECTION('',(-1.95511867169517E-16,1.,0.)) ;
#96640=DIRECTION('',(0.577350269189625,-0.577350269189626,0.577350269189626)) ;
#96641=DIRECTION('',(0.,-1.,-1.95511867169518E-16)) ;
#96642=DIRECTION('center_axis',(-0.707106781186548,-1.38247767078009E-16,
-0.707106781186547)) ;
#96643=DIRECTION('ref_axis',(-0.707106781186547,-8.815972061965E-34,0.707106781186548)) ;
#96644=DIRECTION('',(-0.577350269189625,0.577350269189626,0.577350269189626)) ;
#96645=DIRECTION('',(1.95511867169517E-16,-1.,0.)) ;
#96646=DIRECTION('',(0.577350269189625,0.577350269189626,-0.577350269189626)) ;
#96647=DIRECTION('',(0.,1.,-1.95511867169518E-16)) ;
#96648=DIRECTION('center_axis',(-0.707106781186548,-1.38247767078009E-16,
0.707106781186547)) ;
#96649=DIRECTION('ref_axis',(0.707106781186547,8.815972061965E-34,0.707106781186548)) ;
#96650=DIRECTION('',(-0.577350269189625,-0.577350269189626,-0.577350269189626)) ;
#96651=DIRECTION('',(-1.95511867169517E-16,1.,0.)) ;
#96652=DIRECTION('',(0.577350269189625,-0.577350269189626,0.577350269189626)) ;
#96653=DIRECTION('',(0.,-1.,-1.95511867169518E-16)) ;
#96654=DIRECTION('center_axis',(-0.707106781186548,-1.38247767078009E-16,
-0.707106781186547)) ;
#96655=DIRECTION('ref_axis',(-0.707106781186547,-8.815972061965E-34,0.707106781186548)) ;
#96656=DIRECTION('',(-0.577350269189625,0.577350269189626,0.577350269189626)) ;
#96657=DIRECTION('',(1.95511867169517E-16,-1.,0.)) ;
#96658=DIRECTION('',(0.577350269189625,0.577350269189626,-0.577350269189626)) ;
#96659=DIRECTION('',(0.,1.,-1.95511867169518E-16)) ;
#96660=DIRECTION('center_axis',(-0.707106781186548,-1.38247767078009E-16,
0.707106781186547)) ;
#96661=DIRECTION('ref_axis',(0.707106781186547,8.815972061965E-34,0.707106781186548)) ;
#96662=DIRECTION('',(-0.577350269189625,-0.577350269189626,-0.577350269189626)) ;
#96663=DIRECTION('',(-1.95511867169517E-16,1.,0.)) ;
#96664=DIRECTION('',(0.577350269189625,-0.577350269189626,0.577350269189626)) ;
#96665=DIRECTION('',(0.,-1.,-1.95511867169518E-16)) ;
#96666=DIRECTION('center_axis',(-0.707106781186548,-1.38247767078009E-16,
-0.707106781186547)) ;
#96667=DIRECTION('ref_axis',(-0.707106781186547,-8.815972061965E-34,0.707106781186548)) ;
#96668=DIRECTION('',(-0.577350269189625,0.577350269189626,0.577350269189626)) ;
#96669=DIRECTION('',(1.95511867169517E-16,-1.,0.)) ;
#96670=DIRECTION('',(0.577350269189625,0.577350269189626,-0.577350269189626)) ;
#96671=DIRECTION('',(0.,1.,-1.95511867169518E-16)) ;
#96672=DIRECTION('center_axis',(-0.707106781186548,-1.38247767078009E-16,
0.707106781186547)) ;
#96673=DIRECTION('ref_axis',(0.707106781186547,8.815972061965E-34,0.707106781186548)) ;
#96674=DIRECTION('',(-0.577350269189625,-0.577350269189626,-0.577350269189626)) ;
#96675=DIRECTION('',(-1.95511867169517E-16,1.,0.)) ;
#96676=DIRECTION('',(0.577350269189625,-0.577350269189626,0.577350269189626)) ;
#96677=DIRECTION('',(0.,-1.,-1.95511867169518E-16)) ;
#96678=DIRECTION('center_axis',(-0.707106781186548,-1.38247767078009E-16,
-0.707106781186547)) ;
#96679=DIRECTION('ref_axis',(-0.707106781186547,-8.815972061965E-34,0.707106781186548)) ;
#96680=DIRECTION('',(-0.577350269189625,0.577350269189626,0.577350269189626)) ;
#96681=DIRECTION('',(1.95511867169517E-16,-1.,0.)) ;
#96682=DIRECTION('',(0.577350269189625,0.577350269189626,-0.577350269189626)) ;
#96683=DIRECTION('',(0.,1.,-1.95511867169518E-16)) ;
#96684=DIRECTION('center_axis',(-0.707106781186548,-1.38247767078009E-16,
0.707106781186547)) ;
#96685=DIRECTION('ref_axis',(0.707106781186547,8.815972061965E-34,0.707106781186548)) ;
#96686=DIRECTION('',(-0.577350269189625,-0.577350269189626,-0.577350269189626)) ;
#96687=DIRECTION('',(-1.95511867169517E-16,1.,0.)) ;
#96688=DIRECTION('',(0.577350269189625,-0.577350269189626,0.577350269189626)) ;
#96689=DIRECTION('',(0.,-1.,-1.95511867169518E-16)) ;
#96690=DIRECTION('center_axis',(-0.707106781186548,-1.38247767078009E-16,
-0.707106781186547)) ;
#96691=DIRECTION('ref_axis',(-0.707106781186547,-8.815972061965E-34,0.707106781186548)) ;
#96692=DIRECTION('',(-0.577350269189625,0.577350269189626,0.577350269189626)) ;
#96693=DIRECTION('',(1.95511867169517E-16,-1.,0.)) ;
#96694=DIRECTION('',(0.577350269189625,0.577350269189626,-0.577350269189626)) ;
#96695=DIRECTION('',(0.,1.,-1.95511867169518E-16)) ;
#96696=DIRECTION('center_axis',(0.577350269189625,0.577350269189625,-0.577350269189628)) ;
#96697=DIRECTION('ref_axis',(-0.70710678118655,2.50449302218608E-16,-0.707106781186546)) ;
#96698=DIRECTION('center_axis',(-0.577350269189625,-0.577350269189625,0.577350269189628)) ;
#96699=DIRECTION('ref_axis',(-0.707106781186548,-2.12258087602815E-15,-0.707106781186547)) ;
#96700=DIRECTION('center_axis',(-0.577350269189622,-0.577350269189626,0.57735026918963)) ;
#96701=DIRECTION('ref_axis',(4.78608867599257E-17,-0.70710678118655,-0.707106781186545)) ;
#96702=DIRECTION('center_axis',(0.,0.,-1.)) ;
#96703=DIRECTION('ref_axis',(-1.,0.,0.)) ;
#96704=DIRECTION('center_axis',(0.,0.,1.)) ;
#96705=DIRECTION('ref_axis',(-1.,-8.67361737988404E-15,0.)) ;
#96706=DIRECTION('center_axis',(0.,0.,-1.)) ;
#96707=DIRECTION('ref_axis',(-1.,0.,0.)) ;
#96708=DIRECTION('center_axis',(2.08166817117218E-16,1.,0.)) ;
#96709=DIRECTION('ref_axis',(1.,0.,0.)) ;
#96710=DIRECTION('center_axis',(-1.,0.,-4.40821857296472E-15)) ;
#96711=DIRECTION('ref_axis',(4.40821857296472E-15,0.,-1.)) ;
#96712=DIRECTION('center_axis',(8.67361737988402E-15,8.67361737988401E-15,
1.)) ;
#96713=DIRECTION('ref_axis',(-1.,-9.79595207717063E-44,8.67361737988402E-15)) ;
#96714=DIRECTION('center_axis',(-0.577350269189625,-0.577350269189625,-0.577350269189628)) ;
#96715=DIRECTION('ref_axis',(-0.70710678118655,2.50449302218608E-16,0.707106781186546)) ;
#96716=DIRECTION('center_axis',(-0.577350269189625,-0.577350269189625,-0.577350269189628)) ;
#96717=DIRECTION('ref_axis',(-0.70710678118655,2.22693726602979E-16,0.707106781186546)) ;
#96718=DIRECTION('center_axis',(-0.577350269189624,-0.577350269189623,-0.577350269189631)) ;
#96719=DIRECTION('ref_axis',(-0.707106781186552,5.79770761800025E-17,0.707106781186543)) ;
#96720=DIRECTION('center_axis',(0.,0.,-1.)) ;
#96721=DIRECTION('ref_axis',(-1.,0.,0.)) ;
#96722=DIRECTION('center_axis',(-6.1331736667335E-15,0.,1.)) ;
#96723=DIRECTION('ref_axis',(1.,0.,6.1331736667335E-15)) ;
#96724=DIRECTION('center_axis',(-1.,0.,9.8563833862319E-18)) ;
#96725=DIRECTION('ref_axis',(9.8563833862319E-18,0.,1.)) ;
#96726=DIRECTION('center_axis',(-1.,3.93023287525994E-15,-3.93023287525997E-15)) ;
#96727=DIRECTION('ref_axis',(-3.93023287525997E-15,2.80259692864963E-44,
1.)) ;
#96728=DIRECTION('center_axis',(2.08166817117218E-16,1.,0.)) ;
#96729=DIRECTION('ref_axis',(1.,0.,0.)) ;
#96730=DIRECTION('center_axis',(-1.,-8.13151629364126E-16,-8.13151629364131E-16)) ;
#96731=DIRECTION('ref_axis',(8.13151629364131E-16,1.13855500226391E-45,
-1.)) ;
#96732=DIRECTION('center_axis',(2.08166817117218E-16,1.,0.)) ;
#96733=DIRECTION('ref_axis',(1.,0.,0.)) ;
#96734=DIRECTION('center_axis',(-0.577350269189623,0.577350269189622,-0.577350269189633)) ;
#96735=DIRECTION('ref_axis',(0.707106781186554,7.82055407754491E-16,-0.707106781186541)) ;
#96736=DIRECTION('center_axis',(-6.1331736667335E-15,0.,1.)) ;
#96737=DIRECTION('ref_axis',(-1.,0.,-6.1331736667335E-15)) ;
#96738=DIRECTION('center_axis',(-1.,0.,-9.8563833862319E-18)) ;
#96739=DIRECTION('ref_axis',(-9.8563833862319E-18,0.,1.)) ;
#96740=DIRECTION('center_axis',(-1.,0.,-2.10827844793965E-15)) ;
#96741=DIRECTION('ref_axis',(-2.10827844793965E-15,0.,1.)) ;
#96742=DIRECTION('center_axis',(0.,0.,-1.)) ;
#96743=DIRECTION('ref_axis',(-1.,0.,0.)) ;
#96744=DIRECTION('center_axis',(0.,0.,1.)) ;
#96745=DIRECTION('ref_axis',(1.,0.,0.)) ;
#96746=DIRECTION('center_axis',(0.577350269189625,-0.577350269189625,0.577350269189628)) ;
#96747=DIRECTION('ref_axis',(0.707106781186549,-7.23605167296792E-16,-0.707106781186546)) ;
#96748=DIRECTION('center_axis',(0.577350269189625,-0.577350269189625,0.577350269189628)) ;
#96749=DIRECTION('ref_axis',(0.707106781186549,-7.51360742912421E-16,-0.707106781186546)) ;
#96750=DIRECTION('center_axis',(2.08166817117218E-16,1.,0.)) ;
#96751=DIRECTION('ref_axis',(1.,0.,0.)) ;
#96752=DIRECTION('center_axis',(-0.577350269189626,0.577350269189624,0.577350269189628)) ;
#96753=DIRECTION('ref_axis',(-0.707106781186549,-7.24154524606924E-16,-0.707106781186546)) ;
#96754=DIRECTION('center_axis',(0.,0.,-1.)) ;
#96755=DIRECTION('ref_axis',(-1.,0.,0.)) ;
#96756=DIRECTION('center_axis',(0.,0.,1.)) ;
#96757=DIRECTION('ref_axis',(-1.,0.,0.)) ;
#96758=DIRECTION('center_axis',(0.,0.,-1.)) ;
#96759=DIRECTION('ref_axis',(-1.,0.,0.)) ;
#96760=DIRECTION('center_axis',(-0.577350269189625,0.577350269189625,0.577350269189628)) ;
#96761=DIRECTION('ref_axis',(0.70710678118655,2.22693726602979E-16,0.707106781186546)) ;
#96762=DIRECTION('center_axis',(0.577350269189625,-0.577350269189625,-0.577350269189628)) ;
#96763=DIRECTION('ref_axis',(0.707106781186549,-8.43215074740835E-16,0.707106781186546)) ;
#96764=DIRECTION('center_axis',(-0.577350269189625,0.577350269189626,-0.577350269189626)) ;
#96765=DIRECTION('ref_axis',(6.27941990732594E-17,0.707106781186548,0.707106781186548)) ;
#96766=DIRECTION('center_axis',(0.577350269189625,-0.577350269189626,0.577350269189626)) ;
#96767=DIRECTION('ref_axis',(5.0289788758123E-16,0.707106781186548,0.707106781186547)) ;
#96768=DIRECTION('center_axis',(0.577350269189624,-0.57735026918963,0.577350269189624)) ;
#96769=DIRECTION('ref_axis',(0.707106781186551,0.707106781186544,6.33763658455854E-16)) ;
#96770=DIRECTION('center_axis',(0.,0.,-1.)) ;
#96771=DIRECTION('ref_axis',(-1.,0.,0.)) ;
#96772=DIRECTION('center_axis',(0.,0.,1.)) ;
#96773=DIRECTION('ref_axis',(-1.,2.71050543121375E-15,0.)) ;
#96774=DIRECTION('center_axis',(0.,0.,-1.)) ;
#96775=DIRECTION('ref_axis',(-1.,0.,0.)) ;
#96776=DIRECTION('center_axis',(0.,1.,0.)) ;
#96777=DIRECTION('ref_axis',(1.,0.,0.)) ;
#96778=DIRECTION('center_axis',(0.,-1.,-3.25824851045217E-15)) ;
#96779=DIRECTION('ref_axis',(0.,-3.25824851045217E-15,1.)) ;
#96780=DIRECTION('center_axis',(4.33680868994201E-15,-4.33680868994202E-15,
1.)) ;
#96781=DIRECTION('ref_axis',(3.0828566215146E-44,1.,4.33680868994202E-15)) ;
#96782=DIRECTION('center_axis',(0.577350269189625,-0.577350269189626,-0.577350269189626)) ;
#96783=DIRECTION('ref_axis',(6.27941990732594E-17,0.707106781186548,-0.707106781186548)) ;
#96784=DIRECTION('center_axis',(0.577350269189625,-0.577350269189626,-0.577350269189626)) ;
#96785=DIRECTION('ref_axis',(-7.7646791370609E-16,0.707106781186547,-0.707106781186548)) ;
#96786=DIRECTION('center_axis',(0.577350269189625,-0.577350269189626,-0.577350269189627)) ;
#96787=DIRECTION('ref_axis',(-3.31150339748933E-16,0.707106781186548,-0.707106781186547)) ;
#96788=DIRECTION('center_axis',(0.,0.,-1.)) ;
#96789=DIRECTION('ref_axis',(-1.,0.,0.)) ;
#96790=DIRECTION('center_axis',(0.,-6.1331736667335E-15,1.)) ;
#96791=DIRECTION('ref_axis',(0.,-1.,-6.1331736667335E-15)) ;
#96792=DIRECTION('center_axis',(0.,1.,1.95511867169518E-16)) ;
#96793=DIRECTION('ref_axis',(0.,-1.95511867169518E-16,1.)) ;
#96794=DIRECTION('center_axis',(2.71050543121375E-16,-1.,7.93888660359539E-17)) ;
#96795=DIRECTION('ref_axis',(1.,2.71050543121375E-16,0.)) ;
#96796=DIRECTION('center_axis',(0.,1.,0.)) ;
#96797=DIRECTION('ref_axis',(1.,0.,0.)) ;
#96798=DIRECTION('center_axis',(-1.28749007982653E-15,-1.,1.47915175691195E-15)) ;
#96799=DIRECTION('ref_axis',(-1.49686561198851E-32,1.47915175691195E-15,
1.)) ;
#96800=DIRECTION('center_axis',(0.,1.,0.)) ;
#96801=DIRECTION('ref_axis',(1.,0.,0.)) ;
#96802=DIRECTION('center_axis',(-0.577350269189624,-0.577350269189626,-0.577350269189628)) ;
#96803=DIRECTION('ref_axis',(-1.24495925064522E-15,-0.707106781186548,0.707106781186547)) ;
#96804=DIRECTION('center_axis',(0.,-6.1331736667335E-15,1.)) ;
#96805=DIRECTION('ref_axis',(0.,1.,6.1331736667335E-15)) ;
#96806=DIRECTION('center_axis',(0.,1.,-1.95511867169518E-16)) ;
#96807=DIRECTION('ref_axis',(0.,1.95511867169518E-16,1.)) ;
#96808=DIRECTION('center_axis',(0.,-1.,-4.59988025005012E-15)) ;
#96809=DIRECTION('ref_axis',(0.,4.59988025005012E-15,-1.)) ;
#96810=DIRECTION('center_axis',(0.,0.,-1.)) ;
#96811=DIRECTION('ref_axis',(-1.,0.,0.)) ;
#96812=DIRECTION('center_axis',(0.,0.,1.)) ;
#96813=DIRECTION('ref_axis',(1.,0.,0.)) ;
#96814=DIRECTION('center_axis',(0.577350269189625,0.577350269189626,0.577350269189627)) ;
#96815=DIRECTION('ref_axis',(-2.71345386026911E-16,-0.707106781186548,0.707106781186547)) ;
#96816=DIRECTION('center_axis',(0.577350269189625,0.577350269189626,0.577350269189627)) ;
#96817=DIRECTION('ref_axis',(-2.71345386026911E-16,-0.707106781186548,0.707106781186547)) ;
#96818=DIRECTION('center_axis',(0.,1.,0.)) ;
#96819=DIRECTION('ref_axis',(1.,0.,0.)) ;
#96820=DIRECTION('center_axis',(-0.577350269189624,-0.577350269189628,0.577350269189625)) ;
#96821=DIRECTION('ref_axis',(-6.89490688817364E-15,0.707106781186549,0.707106781186546)) ;
#96822=DIRECTION('center_axis',(0.,0.,-1.)) ;
#96823=DIRECTION('ref_axis',(-1.,0.,0.)) ;
#96824=DIRECTION('center_axis',(0.,0.,1.)) ;
#96825=DIRECTION('ref_axis',(-1.,1.0842021724855E-15,0.)) ;
#96826=DIRECTION('center_axis',(0.,0.,-1.)) ;
#96827=DIRECTION('ref_axis',(-1.,0.,0.)) ;
#96828=DIRECTION('center_axis',(-0.577350269189625,-0.577350269189626,0.577350269189627)) ;
#96829=DIRECTION('ref_axis',(-2.71345386026911E-16,-0.707106781186548,-0.707106781186547)) ;
#96830=DIRECTION('center_axis',(0.577350269189625,0.577350269189626,-0.577350269189627)) ;
#96831=DIRECTION('ref_axis',(-9.76085677604559E-15,-0.707106781186543,-0.707106781186552)) ;
#96832=DIRECTION('center_axis',(0.577350269189625,0.577350269189625,-0.577350269189628)) ;
#96833=DIRECTION('ref_axis',(-0.707106781186549,-7.23605167296792E-16,-0.707106781186546)) ;
#96834=DIRECTION('center_axis',(-0.577350269189625,-0.577350269189625,0.577350269189628)) ;
#96835=DIRECTION('ref_axis',(-0.707106781186542,-1.47047746496289E-14,-0.707106781186553)) ;
#96836=DIRECTION('center_axis',(-0.577350269189629,-0.577350269189624,0.577350269189624)) ;
#96837=DIRECTION('ref_axis',(0.707106781186545,-9.59471324968973E-16,0.70710678118655)) ;
#96838=DIRECTION('center_axis',(0.,0.,-1.)) ;
#96839=DIRECTION('ref_axis',(-1.,0.,0.)) ;
#96840=DIRECTION('center_axis',(0.,0.,1.)) ;
#96841=DIRECTION('ref_axis',(-1.,0.,0.)) ;
#96842=DIRECTION('center_axis',(0.,0.,-1.)) ;
#96843=DIRECTION('ref_axis',(-1.,0.,0.)) ;
#96844=DIRECTION('center_axis',(2.08166817117218E-16,1.,0.)) ;
#96845=DIRECTION('ref_axis',(1.,0.,0.)) ;
#96846=DIRECTION('center_axis',(-1.,0.,-5.94151198964807E-15)) ;
#96847=DIRECTION('ref_axis',(5.94151198964807E-15,0.,-1.)) ;
#96848=DIRECTION('center_axis',(0.,0.,1.)) ;
#96849=DIRECTION('ref_axis',(-1.,0.,0.)) ;
#96850=DIRECTION('center_axis',(-0.577350269189625,-0.577350269189625,-0.577350269189628)) ;
#96851=DIRECTION('ref_axis',(-0.707106781186549,-7.23605167296792E-16,0.707106781186546)) ;
#96852=DIRECTION('center_axis',(-0.577350269189625,-0.577350269189625,-0.577350269189628)) ;
#96853=DIRECTION('ref_axis',(-0.707106781186549,-7.51360742912421E-16,0.707106781186546)) ;
#96854=DIRECTION('center_axis',(-0.577350269189629,-0.577350269189628,-0.577350269189621)) ;
#96855=DIRECTION('ref_axis',(0.707106781186547,-0.707106781186548,-9.25270248417546E-17)) ;
#96856=DIRECTION('center_axis',(0.,0.,-1.)) ;
#96857=DIRECTION('ref_axis',(-1.,0.,0.)) ;
#96858=DIRECTION('center_axis',(1.2266347333467E-14,0.,1.)) ;
#96859=DIRECTION('ref_axis',(1.,0.,-1.2266347333467E-14)) ;
#96860=DIRECTION('center_axis',(-1.,0.,9.8563833862319E-18)) ;
#96861=DIRECTION('ref_axis',(9.8563833862319E-18,0.,1.)) ;
#96862=DIRECTION('center_axis',(-1.,1.62630325872825E-15,-1.62630325872825E-15)) ;
#96863=DIRECTION('ref_axis',(-1.62630325872825E-15,0.,1.)) ;
#96864=DIRECTION('center_axis',(2.08166817117218E-16,1.,0.)) ;
#96865=DIRECTION('ref_axis',(1.,0.,0.)) ;
#96866=DIRECTION('center_axis',(-1.,1.35525271560688E-16,1.35525271560688E-16)) ;
#96867=DIRECTION('ref_axis',(-1.35525271560688E-16,0.,-1.)) ;
#96868=DIRECTION('center_axis',(2.08166817117218E-16,1.,0.)) ;
#96869=DIRECTION('ref_axis',(1.,0.,0.)) ;
#96870=DIRECTION('center_axis',(-0.577350269189628,0.577350269189628,-0.577350269189621)) ;
#96871=DIRECTION('ref_axis',(0.707106781186547,0.707106781186548,5.83290435273539E-16)) ;
#96872=DIRECTION('center_axis',(1.2266347333467E-14,0.,1.)) ;
#96873=DIRECTION('ref_axis',(-1.,0.,1.2266347333467E-14)) ;
#96874=DIRECTION('center_axis',(-1.,0.,-9.8563833862319E-18)) ;
#96875=DIRECTION('ref_axis',(-9.8563833862319E-18,0.,1.)) ;
#96876=DIRECTION('center_axis',(-1.,0.,9.58308385427108E-16)) ;
#96877=DIRECTION('ref_axis',(9.58308385427108E-16,0.,1.)) ;
#96878=DIRECTION('center_axis',(0.,0.,-1.)) ;
#96879=DIRECTION('ref_axis',(-1.,0.,0.)) ;
#96880=DIRECTION('center_axis',(-8.67361737988402E-15,8.67361737988401E-15,
1.)) ;
#96881=DIRECTION('ref_axis',(1.,-9.79595207717063E-44,8.67361737988402E-15)) ;
#96882=DIRECTION('center_axis',(0.577350269189625,-0.577350269189625,0.577350269189628)) ;
#96883=DIRECTION('ref_axis',(0.707106781186549,-7.23605167296792E-16,-0.707106781186546)) ;
#96884=DIRECTION('center_axis',(0.577350269189625,-0.577350269189625,0.577350269189628)) ;
#96885=DIRECTION('ref_axis',(0.707106781186549,-7.51360742912421E-16,-0.707106781186546)) ;
#96886=DIRECTION('center_axis',(2.08166817117218E-16,1.,0.)) ;
#96887=DIRECTION('ref_axis',(1.,0.,0.)) ;
#96888=DIRECTION('center_axis',(-0.577350269189631,0.577350269189623,0.577350269189623)) ;
#96889=DIRECTION('ref_axis',(-0.707106781186542,1.43689139429453E-15,-0.707106781186553)) ;
#96890=DIRECTION('center_axis',(0.,0.,-1.)) ;
#96891=DIRECTION('ref_axis',(-1.,0.,0.)) ;
#96892=DIRECTION('center_axis',(0.,0.,1.)) ;
#96893=DIRECTION('ref_axis',(-1.,0.,0.)) ;
#96894=DIRECTION('center_axis',(0.,0.,-1.)) ;
#96895=DIRECTION('ref_axis',(-1.,0.,0.)) ;
#96896=DIRECTION('center_axis',(-0.577350269189625,0.577350269189625,0.577350269189628)) ;
#96897=DIRECTION('ref_axis',(0.707106781186549,-7.51360742912421E-16,0.707106781186546)) ;
#96898=DIRECTION('center_axis',(0.577350269189625,-0.577350269189625,-0.577350269189628)) ;
#96899=DIRECTION('ref_axis',(0.707106781186549,-8.43215074740835E-16,0.707106781186546)) ;
#96900=DIRECTION('center_axis',(-0.577350269189625,0.577350269189626,-0.577350269189626)) ;
#96901=DIRECTION('ref_axis',(6.27941990732594E-17,0.707106781186548,0.707106781186548)) ;
#96902=DIRECTION('center_axis',(0.577350269189625,-0.577350269189626,0.577350269189626)) ;
#96903=DIRECTION('ref_axis',(-4.12932450763554E-14,0.707106781186527,0.707106781186568)) ;
#96904=DIRECTION('center_axis',(0.577350269189626,-0.577350269189626,0.577350269189626)) ;
#96905=DIRECTION('ref_axis',(0.707106781186548,0.707106781186547,-6.70219100485003E-16)) ;
#96906=DIRECTION('center_axis',(0.,0.,-1.)) ;
#96907=DIRECTION('ref_axis',(-1.,0.,0.)) ;
#96908=DIRECTION('center_axis',(0.,0.,1.)) ;
#96909=DIRECTION('ref_axis',(-1.,0.,0.)) ;
#96910=DIRECTION('center_axis',(0.,0.,-1.)) ;
#96911=DIRECTION('ref_axis',(-1.,0.,0.)) ;
#96912=DIRECTION('center_axis',(0.,1.,0.)) ;
#96913=DIRECTION('ref_axis',(1.,0.,0.)) ;
#96914=DIRECTION('center_axis',(0.,-1.,-1.05413922396982E-14)) ;
#96915=DIRECTION('ref_axis',(0.,-1.05413922396982E-14,1.)) ;
#96916=DIRECTION('center_axis',(-8.67361737988401E-15,8.67361737988403E-15,
1.)) ;
#96917=DIRECTION('ref_axis',(-4.48415508583941E-44,1.,-8.67361737988403E-15)) ;
#96918=DIRECTION('center_axis',(0.577350269189625,-0.577350269189626,-0.577350269189626)) ;
#96919=DIRECTION('ref_axis',(6.27941990732594E-17,0.707106781186548,-0.707106781186548)) ;
#96920=DIRECTION('center_axis',(0.577350269189625,-0.577350269189626,-0.577350269189626)) ;
#96921=DIRECTION('ref_axis',(-7.7646791370609E-16,0.707106781186547,-0.707106781186548)) ;
#96922=DIRECTION('center_axis',(0.577350269189627,-0.577350269189628,-0.577350269189622)) ;
#96923=DIRECTION('ref_axis',(0.707106781186548,0.707106781186547,-7.93962717014541E-17)) ;
#96924=DIRECTION('center_axis',(0.,0.,-1.)) ;
#96925=DIRECTION('ref_axis',(-1.,0.,0.)) ;
#96926=DIRECTION('center_axis',(0.,1.2266347333467E-14,1.)) ;
#96927=DIRECTION('ref_axis',(0.,-1.,1.2266347333467E-14)) ;
#96928=DIRECTION('center_axis',(0.,1.,1.95511867169518E-16)) ;
#96929=DIRECTION('ref_axis',(0.,-1.95511867169518E-16,1.)) ;
#96930=DIRECTION('center_axis',(-1.42301535138722E-15,-1.,-1.61467702847264E-15)) ;
#96931=DIRECTION('ref_axis',(-1.65443041324959E-32,1.61467702847264E-15,
-1.)) ;
#96932=DIRECTION('center_axis',(0.,1.,0.)) ;
#96933=DIRECTION('ref_axis',(1.,0.,0.)) ;
#96934=DIRECTION('center_axis',(3.72694496791891E-15,-1.,-3.53528329083349E-15)) ;
#96935=DIRECTION('ref_axis',(-1.,-3.72694496791891E-15,0.)) ;
#96936=DIRECTION('center_axis',(0.,1.,0.)) ;
#96937=DIRECTION('ref_axis',(1.,0.,0.)) ;
#96938=DIRECTION('center_axis',(-0.577350269189623,-0.577350269189624,-0.577350269189631)) ;
#96939=DIRECTION('ref_axis',(1.89964573407132E-15,-0.707106781186553,0.707106781186542)) ;
#96940=DIRECTION('center_axis',(0.,-1.2266347333467E-14,1.)) ;
#96941=DIRECTION('ref_axis',(0.,1.,1.2266347333467E-14)) ;
#96942=DIRECTION('center_axis',(0.,1.,-1.95511867169518E-16)) ;
#96943=DIRECTION('ref_axis',(0.,1.95511867169518E-16,1.)) ;
#96944=DIRECTION('center_axis',(0.,-1.,-7.66646708341686E-16)) ;
#96945=DIRECTION('ref_axis',(0.,7.66646708341686E-16,-1.)) ;
#96946=DIRECTION('center_axis',(0.,0.,-1.)) ;
#96947=DIRECTION('ref_axis',(-1.,0.,0.)) ;
#96948=DIRECTION('center_axis',(0.,0.,1.)) ;
#96949=DIRECTION('ref_axis',(1.,0.,0.)) ;
#96950=DIRECTION('center_axis',(0.577350269189625,0.577350269189626,0.577350269189627)) ;
#96951=DIRECTION('ref_axis',(-2.71345386026911E-16,-0.707106781186548,0.707106781186547)) ;
#96952=DIRECTION('center_axis',(0.577350269189625,0.577350269189626,0.577350269189627)) ;
#96953=DIRECTION('ref_axis',(-2.71345386026911E-16,-0.707106781186548,0.707106781186547)) ;
#96954=DIRECTION('center_axis',(0.,1.,0.)) ;
#96955=DIRECTION('ref_axis',(1.,0.,0.)) ;
#96956=DIRECTION('center_axis',(-0.577350269189625,-0.577350269189627,0.577350269189625)) ;
#96957=DIRECTION('ref_axis',(4.24759239037863E-16,0.707106781186546,0.707106781186549)) ;
#96958=DIRECTION('center_axis',(0.,0.,-1.)) ;
#96959=DIRECTION('ref_axis',(-1.,0.,0.)) ;
#96960=DIRECTION('center_axis',(0.,0.,1.)) ;
#96961=DIRECTION('ref_axis',(-1.,1.0842021724855E-15,0.)) ;
#96962=DIRECTION('center_axis',(0.,0.,-1.)) ;
#96963=DIRECTION('ref_axis',(-1.,0.,0.)) ;
#96964=DIRECTION('center_axis',(-0.577350269189625,-0.577350269189626,0.577350269189627)) ;
#96965=DIRECTION('ref_axis',(-2.71345386026911E-16,-0.707106781186548,-0.707106781186547)) ;
#96966=DIRECTION('center_axis',(0.577350269189625,0.577350269189626,-0.577350269189627)) ;
#96967=DIRECTION('ref_axis',(-8.1269550549169E-15,-0.707106781186544,-0.707106781186551)) ;
#96968=DIRECTION('center_axis',(0.577350269189625,0.577350269189625,-0.577350269189628)) ;
#96969=DIRECTION('ref_axis',(-0.707106781186549,-7.23605167296792E-16,-0.707106781186546)) ;
#96970=DIRECTION('center_axis',(-0.577350269189625,-0.577350269189625,0.577350269189628)) ;
#96971=DIRECTION('ref_axis',(-0.707106781186545,-8.33999502129868E-15,-0.70710678118655)) ;
#96972=DIRECTION('center_axis',(-0.577350269189627,-0.577350269189625,0.577350269189625)) ;
#96973=DIRECTION('ref_axis',(0.707106781186546,1.26631399429469E-16,0.707106781186549)) ;
#96974=DIRECTION('center_axis',(0.,0.,-1.)) ;
#96975=DIRECTION('ref_axis',(-1.,0.,0.)) ;
#96976=DIRECTION('center_axis',(0.,0.,1.)) ;
#96977=DIRECTION('ref_axis',(-1.,0.,0.)) ;
#96978=DIRECTION('center_axis',(0.,0.,-1.)) ;
#96979=DIRECTION('ref_axis',(-1.,0.,0.)) ;
#96980=DIRECTION('center_axis',(2.08166817117218E-16,1.,0.)) ;
#96981=DIRECTION('ref_axis',(1.,0.,0.)) ;
#96982=DIRECTION('center_axis',(-1.,0.,9.58308385427108E-16)) ;
#96983=DIRECTION('ref_axis',(-9.58308385427108E-16,0.,-1.)) ;
#96984=DIRECTION('center_axis',(0.,0.,1.)) ;
#96985=DIRECTION('ref_axis',(-1.,0.,0.)) ;
#96986=DIRECTION('center_axis',(-0.577350269189625,-0.577350269189625,-0.577350269189628)) ;
#96987=DIRECTION('ref_axis',(-0.707106781186549,-7.23605167296792E-16,0.707106781186546)) ;
#96988=DIRECTION('center_axis',(-0.577350269189625,-0.577350269189625,-0.577350269189628)) ;
#96989=DIRECTION('ref_axis',(-0.707106781186549,-7.51360742912421E-16,0.707106781186546)) ;
#96990=DIRECTION('center_axis',(-0.577350269189633,-0.577350269189632,-0.577350269189612)) ;
#96991=DIRECTION('ref_axis',(0.707106781186547,-0.707106781186548,-7.39398349810839E-17)) ;
#96992=DIRECTION('center_axis',(0.,0.,-1.)) ;
#96993=DIRECTION('ref_axis',(-1.,0.,0.)) ;
#96994=DIRECTION('center_axis',(2.4532694666934E-14,0.,1.)) ;
#96995=DIRECTION('ref_axis',(1.,0.,-2.4532694666934E-14)) ;
#96996=DIRECTION('center_axis',(-1.,0.,9.8563833862319E-18)) ;
#96997=DIRECTION('ref_axis',(9.8563833862319E-18,0.,1.)) ;
#96998=DIRECTION('center_axis',(-1.,-8.40256683676264E-15,8.40256683676264E-15)) ;
#96999=DIRECTION('ref_axis',(8.40256683676264E-15,-6.05360936588321E-43,
1.)) ;
#97000=DIRECTION('center_axis',(2.08166817117218E-16,1.,0.)) ;
#97001=DIRECTION('ref_axis',(1.,0.,0.)) ;
#97002=DIRECTION('center_axis',(-1.,4.9466724119651E-15,4.9466724119651E-15)) ;
#97003=DIRECTION('ref_axis',(-4.9466724119651E-15,-2.12997366577372E-43,
-1.)) ;
#97004=DIRECTION('center_axis',(2.08166817117218E-16,1.,0.)) ;
#97005=DIRECTION('ref_axis',(1.,0.,0.)) ;
#97006=DIRECTION('center_axis',(-0.577350269189629,0.577350269189628,-0.577350269189621)) ;
#97007=DIRECTION('ref_axis',(0.707106781186547,0.707106781186548,-3.27220711197328E-17)) ;
#97008=DIRECTION('center_axis',(0.,0.,1.)) ;
#97009=DIRECTION('ref_axis',(-1.,0.,0.)) ;
#97010=DIRECTION('center_axis',(-1.,0.,-9.8563833862319E-18)) ;
#97011=DIRECTION('ref_axis',(-9.8563833862319E-18,0.,1.)) ;
#97012=DIRECTION('center_axis',(-1.,0.,-1.05413922396982E-14)) ;
#97013=DIRECTION('ref_axis',(-1.05413922396982E-14,0.,1.)) ;
#97014=DIRECTION('center_axis',(0.,0.,-1.)) ;
#97015=DIRECTION('ref_axis',(-1.,0.,0.)) ;
#97016=DIRECTION('center_axis',(0.,0.,1.)) ;
#97017=DIRECTION('ref_axis',(1.,0.,0.)) ;
#97018=DIRECTION('center_axis',(0.577350269189625,-0.577350269189625,0.577350269189628)) ;
#97019=DIRECTION('ref_axis',(0.707106781186549,-7.23605167296792E-16,-0.707106781186546)) ;
#97020=DIRECTION('center_axis',(0.577350269189625,-0.577350269189625,0.577350269189628)) ;
#97021=DIRECTION('ref_axis',(0.707106781186549,-7.51360742912421E-16,-0.707106781186546)) ;
#97022=DIRECTION('center_axis',(2.08166817117218E-16,1.,0.)) ;
#97023=DIRECTION('ref_axis',(1.,0.,0.)) ;
#97024=DIRECTION('center_axis',(-0.577350269189631,0.577350269189623,0.577350269189623)) ;
#97025=DIRECTION('ref_axis',(-0.707106781186544,-2.28159610212341E-15,-0.707106781186551)) ;
#97026=DIRECTION('center_axis',(0.,0.,-1.)) ;
#97027=DIRECTION('ref_axis',(-1.,0.,0.)) ;
#97028=DIRECTION('center_axis',(0.,0.,1.)) ;
#97029=DIRECTION('ref_axis',(-1.,0.,0.)) ;
#97030=DIRECTION('center_axis',(0.,0.,-1.)) ;
#97031=DIRECTION('ref_axis',(-1.,0.,0.)) ;
#97032=DIRECTION('center_axis',(-0.577350269189625,0.577350269189625,0.577350269189628)) ;
#97033=DIRECTION('ref_axis',(0.707106781186549,-7.51360742912421E-16,0.707106781186546)) ;
#97034=DIRECTION('center_axis',(0.577350269189625,-0.577350269189625,-0.577350269189628)) ;
#97035=DIRECTION('ref_axis',(0.707106781186548,-2.12258087602815E-15,0.707106781186547)) ;
#97036=DIRECTION('center_axis',(-0.577350269189625,0.577350269189626,-0.577350269189626)) ;
#97037=DIRECTION('ref_axis',(6.27941990732594E-17,0.707106781186548,0.707106781186548)) ;
#97038=DIRECTION('center_axis',(0.577350269189625,-0.577350269189626,0.577350269189626)) ;
#97039=DIRECTION('ref_axis',(-2.74316855014674E-14,0.707106781186534,0.707106781186561)) ;
#97040=DIRECTION('center_axis',(0.577350269189617,-0.577350269189643,0.577350269189617)) ;
#97041=DIRECTION('ref_axis',(0.707106781186564,0.707106781186531,-7.69284786604672E-16)) ;
#97042=DIRECTION('center_axis',(0.,0.,-1.)) ;
#97043=DIRECTION('ref_axis',(-1.,0.,0.)) ;
#97044=DIRECTION('center_axis',(0.,0.,1.)) ;
#97045=DIRECTION('ref_axis',(-1.,0.,0.)) ;
#97046=DIRECTION('center_axis',(0.,0.,-1.)) ;
#97047=DIRECTION('ref_axis',(-1.,0.,0.)) ;
#97048=DIRECTION('center_axis',(0.,1.,0.)) ;
#97049=DIRECTION('ref_axis',(1.,0.,0.)) ;
#97050=DIRECTION('center_axis',(0.,-1.,-1.39913024272358E-14)) ;
#97051=DIRECTION('ref_axis',(0.,-1.39913024272358E-14,1.)) ;
#97052=DIRECTION('center_axis',(1.7347234759768E-14,-1.73472347597681E-14,
1.)) ;
#97053=DIRECTION('ref_axis',(-1.79366203433577E-43,1.,1.73472347597681E-14)) ;
#97054=DIRECTION('center_axis',(0.577350269189625,-0.577350269189626,-0.577350269189626)) ;
#97055=DIRECTION('ref_axis',(6.27941990732594E-17,0.707106781186548,-0.707106781186548)) ;
#97056=DIRECTION('center_axis',(0.577350269189625,-0.577350269189626,-0.577350269189626)) ;
#97057=DIRECTION('ref_axis',(-7.7646791370609E-16,0.707106781186547,-0.707106781186548)) ;
#97058=DIRECTION('center_axis',(0.577350269189636,-0.577350269189637,-0.577350269189605)) ;
#97059=DIRECTION('ref_axis',(0.707106781186548,0.707106781186547,-1.89650892222054E-16)) ;
#97060=DIRECTION('center_axis',(0.,0.,-1.)) ;
#97061=DIRECTION('ref_axis',(-1.,0.,0.)) ;
#97062=DIRECTION('center_axis',(0.,2.4532694666934E-14,1.)) ;
#97063=DIRECTION('ref_axis',(0.,-1.,2.4532694666934E-14)) ;
#97064=DIRECTION('center_axis',(0.,1.,1.95511867169518E-16)) ;
#97065=DIRECTION('ref_axis',(0.,-1.95511867169518E-16,1.)) ;
#97066=DIRECTION('center_axis',(1.21972744404619E-15,-1.,1.02806576696077E-15)) ;
#97067=DIRECTION('ref_axis',(1.,1.21972744404619E-15,0.)) ;
#97068=DIRECTION('center_axis',(0.,1.,0.)) ;
#97069=DIRECTION('ref_axis',(1.,0.,0.)) ;
#97070=DIRECTION('center_axis',(-1.41623908780917E-14,-1.,1.43540525551772E-14)) ;
#97071=DIRECTION('ref_axis',(-1.64655217322172E-31,1.43540525551772E-14,
1.)) ;
#97072=DIRECTION('center_axis',(0.,1.,0.)) ;
#97073=DIRECTION('ref_axis',(1.,0.,0.)) ;
#97074=DIRECTION('center_axis',(-0.577350269189625,-0.577350269189626,-0.577350269189626)) ;
#97075=DIRECTION('ref_axis',(4.43092933859209E-16,-0.707106781186548,0.707106781186547)) ;
#97076=DIRECTION('center_axis',(0.,0.,1.)) ;
#97077=DIRECTION('ref_axis',(-1.,8.87690528722505E-15,0.)) ;
#97078=DIRECTION('center_axis',(0.,1.,-1.95511867169518E-16)) ;
#97079=DIRECTION('ref_axis',(0.,1.95511867169518E-16,1.)) ;
#97080=DIRECTION('center_axis',(0.,-1.,-2.17536003491953E-14)) ;
#97081=DIRECTION('ref_axis',(0.,2.17536003491953E-14,-1.)) ;
#97082=DIRECTION('center_axis',(0.,0.,-1.)) ;
#97083=DIRECTION('ref_axis',(-1.,0.,0.)) ;
#97084=DIRECTION('center_axis',(-1.7347234759768E-14,-1.73472347597681E-14,
1.)) ;
#97085=DIRECTION('ref_axis',(-8.96831017167883E-44,-1.,-1.73472347597681E-14)) ;
#97086=DIRECTION('center_axis',(0.577350269189625,0.577350269189626,0.577350269189627)) ;
#97087=DIRECTION('ref_axis',(-2.71345386026911E-16,-0.707106781186548,0.707106781186547)) ;
#97088=DIRECTION('center_axis',(0.577350269189625,0.577350269189626,0.577350269189627)) ;
#97089=DIRECTION('ref_axis',(-2.71345386026911E-16,-0.707106781186548,0.707106781186547)) ;
#97090=DIRECTION('center_axis',(0.,1.,0.)) ;
#97091=DIRECTION('ref_axis',(1.,0.,0.)) ;
#97092=DIRECTION('center_axis',(-0.577350269189615,-0.577350269189648,0.577350269189615)) ;
#97093=DIRECTION('ref_axis',(-7.65039491896549E-15,0.707106781186531,0.707106781186564)) ;
#97094=DIRECTION('center_axis',(0.,0.,-1.)) ;
#97095=DIRECTION('ref_axis',(-1.,0.,0.)) ;
#97096=DIRECTION('center_axis',(0.,0.,1.)) ;
#97097=DIRECTION('ref_axis',(-1.,1.0842021724855E-15,0.)) ;
#97098=DIRECTION('center_axis',(0.,0.,-1.)) ;
#97099=DIRECTION('ref_axis',(-1.,0.,0.)) ;
#97100=DIRECTION('center_axis',(-0.577350269189625,-0.577350269189626,0.577350269189627)) ;
#97101=DIRECTION('ref_axis',(-2.71345386026911E-16,-0.707106781186548,-0.707106781186547)) ;
#97102=DIRECTION('center_axis',(0.577350269189625,0.577350269189626,-0.577350269189627)) ;
#97103=DIRECTION('ref_axis',(1.27552458785726E-14,-0.707106781186554,-0.707106781186541)) ;
#97104=DIRECTION('center_axis',(0.577350269189625,0.577350269189625,-0.577350269189628)) ;
#97105=DIRECTION('ref_axis',(-0.707106781186549,-7.23605167296792E-16,-0.707106781186546)) ;
#97106=DIRECTION('center_axis',(-0.577350269189625,-0.577350269189625,0.577350269189628)) ;
#97107=DIRECTION('ref_axis',(-0.707106781186545,-8.28019006757666E-15,-0.70710678118655)) ;
#97108=DIRECTION('center_axis',(-0.577350269189628,-0.577350269189625,0.577350269189625)) ;
#97109=DIRECTION('ref_axis',(0.707106781186546,1.58001979428239E-16,0.707106781186549)) ;
#97110=DIRECTION('center_axis',(0.,0.,-1.)) ;
#97111=DIRECTION('ref_axis',(-1.,0.,0.)) ;
#97112=DIRECTION('center_axis',(0.,0.,1.)) ;
#97113=DIRECTION('ref_axis',(-1.,-8.67361737988404E-15,0.)) ;
#97114=DIRECTION('center_axis',(0.,0.,-1.)) ;
#97115=DIRECTION('ref_axis',(-1.,0.,0.)) ;
#97116=DIRECTION('center_axis',(2.08166817117218E-16,1.,0.)) ;
#97117=DIRECTION('ref_axis',(1.,0.,0.)) ;
#97118=DIRECTION('center_axis',(-1.,0.,-4.40821857296469E-15)) ;
#97119=DIRECTION('ref_axis',(4.40821857296469E-15,0.,-1.)) ;
#97120=DIRECTION('center_axis',(0.,0.,1.)) ;
#97121=DIRECTION('ref_axis',(-1.,0.,0.)) ;
#97122=DIRECTION('center_axis',(-0.577350269189625,-0.577350269189625,-0.577350269189628)) ;
#97123=DIRECTION('ref_axis',(-0.707106781186549,-7.23605167296792E-16,0.707106781186546)) ;
#97124=DIRECTION('center_axis',(-0.577350269189625,-0.577350269189625,-0.577350269189628)) ;
#97125=DIRECTION('ref_axis',(-0.707106781186549,-7.51360742912421E-16,0.707106781186546)) ;
#97126=DIRECTION('center_axis',(-0.577350269189624,-0.577350269189624,-0.57735026918963)) ;
#97127=DIRECTION('ref_axis',(-0.70710678118655,-1.90469774984546E-15,0.707106781186545)) ;
#97128=DIRECTION('center_axis',(0.,0.,-1.)) ;
#97129=DIRECTION('ref_axis',(-1.,0.,0.)) ;
#97130=DIRECTION('center_axis',(0.,0.,1.)) ;
#97131=DIRECTION('ref_axis',(1.,0.,0.)) ;
#97132=DIRECTION('center_axis',(-1.,0.,9.8563833862319E-18)) ;
#97133=DIRECTION('ref_axis',(9.8563833862319E-18,0.,1.)) ;
#97134=DIRECTION('center_axis',(-1.,3.93023287525994E-15,-3.93023287525994E-15)) ;
#97135=DIRECTION('ref_axis',(-3.93023287525994E-15,-1.34524652575182E-43,
1.)) ;
#97136=DIRECTION('center_axis',(2.08166817117218E-16,1.,0.)) ;
#97137=DIRECTION('ref_axis',(1.,0.,0.)) ;
#97138=DIRECTION('center_axis',(-1.,-4.33680868994201E-15,-4.33680868994201E-15)) ;
#97139=DIRECTION('ref_axis',(4.33680868994201E-15,-1.59748024933029E-43,
-1.)) ;
#97140=DIRECTION('center_axis',(2.08166817117218E-16,1.,0.)) ;
#97141=DIRECTION('ref_axis',(1.,0.,0.)) ;
#97142=DIRECTION('center_axis',(-0.577350269189625,0.577350269189624,-0.577350269189628)) ;
#97143=DIRECTION('ref_axis',(0.707106781186549,-6.77492742903108E-16,-0.707106781186546)) ;
#97144=DIRECTION('center_axis',(0.,0.,1.)) ;
#97145=DIRECTION('ref_axis',(-1.,0.,0.)) ;
#97146=DIRECTION('center_axis',(-1.,0.,-9.8563833862319E-18)) ;
#97147=DIRECTION('ref_axis',(-9.8563833862319E-18,0.,1.)) ;
#97148=DIRECTION('center_axis',(-1.,0.,-9.00809882301481E-15)) ;
#97149=DIRECTION('ref_axis',(-9.00809882301481E-15,0.,1.)) ;
#97150=DIRECTION('center_axis',(0.,0.,-1.)) ;
#97151=DIRECTION('ref_axis',(-1.,0.,0.)) ;
#97152=DIRECTION('center_axis',(0.,0.,1.)) ;
#97153=DIRECTION('ref_axis',(1.,0.,0.)) ;
#97154=DIRECTION('center_axis',(0.577350269189625,-0.577350269189625,0.577350269189628)) ;
#97155=DIRECTION('ref_axis',(0.707106781186549,-7.23605167296792E-16,-0.707106781186546)) ;
#97156=DIRECTION('center_axis',(0.577350269189625,-0.577350269189625,0.577350269189628)) ;
#97157=DIRECTION('ref_axis',(0.707106781186549,-7.51360742912421E-16,-0.707106781186546)) ;
#97158=DIRECTION('center_axis',(2.08166817117218E-16,1.,0.)) ;
#97159=DIRECTION('ref_axis',(1.,0.,0.)) ;
#97160=DIRECTION('center_axis',(-0.57735026918963,0.577350269189624,0.577350269189624)) ;
#97161=DIRECTION('ref_axis',(-0.707106781186544,-8.1317851962192E-16,-0.707106781186551)) ;
#97162=DIRECTION('center_axis',(0.,0.,-1.)) ;
#97163=DIRECTION('ref_axis',(-1.,0.,0.)) ;
#97164=DIRECTION('center_axis',(0.,0.,1.)) ;
#97165=DIRECTION('ref_axis',(-1.,0.,0.)) ;
#97166=DIRECTION('center_axis',(0.,0.,-1.)) ;
#97167=DIRECTION('ref_axis',(-1.,0.,0.)) ;
#97168=DIRECTION('center_axis',(-0.577350269189625,0.577350269189625,0.577350269189628)) ;
#97169=DIRECTION('ref_axis',(0.707106781186549,-7.51360742912421E-16,0.707106781186546)) ;
#97170=DIRECTION('center_axis',(0.577350269189625,-0.577350269189625,-0.577350269189628)) ;
#97171=DIRECTION('ref_axis',(0.707106781186545,-8.51940988246475E-15,0.70710678118655)) ;
#97172=DIRECTION('center_axis',(-0.577350269189625,0.577350269189626,-0.577350269189626)) ;
#97173=DIRECTION('ref_axis',(6.27941990732594E-17,0.707106781186548,0.707106781186548)) ;
#97174=DIRECTION('center_axis',(0.577350269189625,-0.577350269189626,0.577350269189626)) ;
#97175=DIRECTION('ref_axis',(-6.96183268087023E-15,0.707106781186544,0.707106781186551)) ;
#97176=DIRECTION('center_axis',(0.577350269189619,-0.57735026918964,0.577350269189619)) ;
#97177=DIRECTION('ref_axis',(0.70710678118656,0.707106781186535,9.56388759536482E-16)) ;
#97178=DIRECTION('center_axis',(0.,0.,-1.)) ;
#97179=DIRECTION('ref_axis',(-1.,0.,0.)) ;
#97180=DIRECTION('center_axis',(0.,0.,1.)) ;
#97181=DIRECTION('ref_axis',(-1.,0.,0.)) ;
#97182=DIRECTION('center_axis',(0.,0.,-1.)) ;
#97183=DIRECTION('ref_axis',(-1.,0.,0.)) ;
#97184=DIRECTION('center_axis',(0.,1.,0.)) ;
#97185=DIRECTION('ref_axis',(1.,0.,0.)) ;
#97186=DIRECTION('center_axis',(0.,-1.,-5.94151198964807E-15)) ;
#97187=DIRECTION('ref_axis',(0.,-5.94151198964807E-15,1.)) ;
#97188=DIRECTION('center_axis',(1.7347234759768E-14,-1.73472347597681E-14,
1.)) ;
#97189=DIRECTION('ref_axis',(-1.79366203433577E-43,1.,1.73472347597681E-14)) ;
#97190=DIRECTION('center_axis',(0.577350269189625,-0.577350269189626,-0.577350269189626)) ;
#97191=DIRECTION('ref_axis',(6.27941990732594E-17,0.707106781186548,-0.707106781186548)) ;
#97192=DIRECTION('center_axis',(0.577350269189625,-0.577350269189626,-0.577350269189626)) ;
#97193=DIRECTION('ref_axis',(3.83287980137187E-16,0.707106781186548,-0.707106781186547)) ;
#97194=DIRECTION('center_axis',(0.57735026918963,-0.577350269189631,-0.577350269189617)) ;
#97195=DIRECTION('ref_axis',(0.707106781186548,0.707106781186547,-9.21608659434825E-17)) ;
#97196=DIRECTION('center_axis',(0.,0.,-1.)) ;
#97197=DIRECTION('ref_axis',(-1.,0.,0.)) ;
#97198=DIRECTION('center_axis',(0.,0.,1.)) ;
#97199=DIRECTION('ref_axis',(1.,0.,0.)) ;
#97200=DIRECTION('center_axis',(0.,1.,1.95511867169518E-16)) ;
#97201=DIRECTION('ref_axis',(0.,-1.95511867169518E-16,1.)) ;
#97202=DIRECTION('center_axis',(1.15196480826585E-15,-1.,9.60303131180424E-16)) ;
#97203=DIRECTION('ref_axis',(1.,1.15196480826585E-15,0.)) ;
#97204=DIRECTION('center_axis',(0.,1.,0.)) ;
#97205=DIRECTION('ref_axis',(1.,0.,0.)) ;
#97206=DIRECTION('center_axis',(-7.5216525716181E-15,-1.,7.71331424870352E-15)) ;
#97207=DIRECTION('ref_axis',(-8.74484647013228E-32,7.71331424870352E-15,
1.)) ;
#97208=DIRECTION('center_axis',(0.,1.,0.)) ;
#97209=DIRECTION('ref_axis',(1.,0.,0.)) ;
#97210=DIRECTION('center_axis',(-0.577350269189626,-0.577350269189627,-0.577350269189625)) ;
#97211=DIRECTION('ref_axis',(-0.707106781186548,0.707106781186547,-9.19305248608458E-17)) ;
#97212=DIRECTION('center_axis',(0.,0.,1.)) ;
#97213=DIRECTION('ref_axis',(-1.,1.76182853028894E-15,0.)) ;
#97214=DIRECTION('center_axis',(0.,1.,-1.95511867169518E-16)) ;
#97215=DIRECTION('ref_axis',(0.,1.95511867169518E-16,1.)) ;
#97216=DIRECTION('center_axis',(0.,-1.,-7.95395959904499E-15)) ;
#97217=DIRECTION('ref_axis',(0.,7.95395959904499E-15,-1.)) ;
#97218=DIRECTION('center_axis',(0.,0.,-1.)) ;
#97219=DIRECTION('ref_axis',(-1.,0.,0.)) ;
#97220=DIRECTION('center_axis',(0.,0.,1.)) ;
#97221=DIRECTION('ref_axis',(1.,0.,0.)) ;
#97222=DIRECTION('center_axis',(0.577350269189625,0.577350269189626,0.577350269189627)) ;
#97223=DIRECTION('ref_axis',(-2.71345386026911E-16,-0.707106781186548,0.707106781186547)) ;
#97224=DIRECTION('center_axis',(0.577350269189625,0.577350269189626,0.577350269189627)) ;
#97225=DIRECTION('ref_axis',(-2.71345386026911E-16,-0.707106781186548,0.707106781186547)) ;
#97226=DIRECTION('center_axis',(0.,1.,0.)) ;
#97227=DIRECTION('ref_axis',(1.,0.,0.)) ;
#97228=DIRECTION('center_axis',(-0.577350269189622,-0.577350269189633,0.577350269189622)) ;
#97229=DIRECTION('ref_axis',(-1.42949951585321E-15,0.707106781186542,0.707106781186553)) ;
#97230=DIRECTION('center_axis',(0.,0.,-1.)) ;
#97231=DIRECTION('ref_axis',(-1.,0.,0.)) ;
#97232=DIRECTION('center_axis',(0.,0.,1.)) ;
#97233=DIRECTION('ref_axis',(-1.,1.0842021724855E-15,0.)) ;
#97234=DIRECTION('center_axis',(0.,0.,-1.)) ;
#97235=DIRECTION('ref_axis',(-1.,0.,0.)) ;
#97236=DIRECTION('center_axis',(-0.577350269189625,-0.577350269189626,0.577350269189627)) ;
#97237=DIRECTION('ref_axis',(-2.71345386026911E-16,-0.707106781186548,-0.707106781186547)) ;
#97238=DIRECTION('center_axis',(0.577350269189625,0.577350269189626,-0.577350269189627)) ;
#97239=DIRECTION('ref_axis',(-2.71345386026911E-16,-0.707106781186548,-0.707106781186547)) ;
#97240=DIRECTION('center_axis',(0.577350269189625,0.577350269189625,-0.577350269189628)) ;
#97241=DIRECTION('ref_axis',(-0.707106781186552,5.19478420936363E-15,-0.707106781186543)) ;
#97242=DIRECTION('center_axis',(-0.577350269189625,-0.577350269189625,0.577350269189628)) ;
#97243=DIRECTION('ref_axis',(-0.707106781186566,3.31891725521342E-14,-0.707106781186529)) ;
#97244=DIRECTION('center_axis',(-0.577350269189652,-0.577350269189606,0.57735026918962)) ;
#97245=DIRECTION('ref_axis',(0.707106781186528,-3.96520952299298E-16,0.707106781186567)) ;
#97246=DIRECTION('center_axis',(0.,0.,-1.)) ;
#97247=DIRECTION('ref_axis',(-1.,0.,0.)) ;
#97248=DIRECTION('center_axis',(0.,0.,1.)) ;
#97249=DIRECTION('ref_axis',(-1.,-8.67361737988404E-15,0.)) ;
#97250=DIRECTION('center_axis',(0.,0.,-1.)) ;
#97251=DIRECTION('ref_axis',(-1.,0.,0.)) ;
#97252=DIRECTION('center_axis',(2.08166817117218E-16,1.,0.)) ;
#97253=DIRECTION('ref_axis',(1.,0.,0.)) ;
#97254=DIRECTION('center_axis',(-1.,0.,-1.66745659064321E-14)) ;
#97255=DIRECTION('ref_axis',(1.66745659064321E-14,2.60208521396523E-14,
-1.)) ;
#97256=DIRECTION('center_axis',(-3.46944695195361E-14,-3.4694469519536E-14,
1.)) ;
#97257=DIRECTION('ref_axis',(-1.,-1.68611237719883E-42,-3.46944695195361E-14)) ;
#97258=DIRECTION('center_axis',(-0.577350269189625,-0.577350269189625,-0.577350269189628)) ;
#97259=DIRECTION('ref_axis',(-0.707106781186552,5.19478420936363E-15,0.707106781186543)) ;
#97260=DIRECTION('center_axis',(-0.577350269189625,-0.577350269189625,-0.577350269189628)) ;
#97261=DIRECTION('ref_axis',(-0.707106781186552,5.1349792556416E-15,0.707106781186543)) ;
#97262=DIRECTION('center_axis',(-0.577350269189626,-0.577350269189626,-0.577350269189626)) ;
#97263=DIRECTION('ref_axis',(0.707106781186547,-0.707106781186548,6.36902276417946E-16)) ;
#97264=DIRECTION('center_axis',(0.,0.,-1.)) ;
#97265=DIRECTION('ref_axis',(-1.,0.,0.)) ;
#97266=DIRECTION('center_axis',(0.,0.,1.)) ;
#97267=DIRECTION('ref_axis',(1.,0.,0.)) ;
#97268=DIRECTION('center_axis',(-1.,0.,9.8563833862319E-18)) ;
#97269=DIRECTION('ref_axis',(9.8563833862319E-18,0.,1.)) ;
#97270=DIRECTION('center_axis',(-1.,8.87690528722497E-15,-8.87690528722518E-15)) ;
#97271=DIRECTION('ref_axis',(-8.87690528722518E-15,4.48415508583942E-43,
1.)) ;
#97272=DIRECTION('center_axis',(2.08166817117218E-16,1.,0.)) ;
#97273=DIRECTION('ref_axis',(1.,0.,0.)) ;
#97274=DIRECTION('center_axis',(-1.,8.53809210832325E-15,8.53809210832346E-15)) ;
#97275=DIRECTION('ref_axis',(-8.53809210832339E-15,8.67361737988409E-15,
-1.)) ;
#97276=DIRECTION('center_axis',(2.08166817117218E-16,1.,0.)) ;
#97277=DIRECTION('ref_axis',(1.,0.,0.)) ;
#97278=DIRECTION('center_axis',(-0.577350269189622,0.577350269189621,-0.577350269189634)) ;
#97279=DIRECTION('ref_axis',(0.707106781186563,1.66970714627838E-14,-0.707106781186532)) ;
#97280=DIRECTION('center_axis',(0.,0.,1.)) ;
#97281=DIRECTION('ref_axis',(-1.,0.,0.)) ;
#97282=DIRECTION('center_axis',(-1.,0.,-9.8563833862319E-18)) ;
#97283=DIRECTION('ref_axis',(-9.8563833862319E-18,0.,1.)) ;
#97284=DIRECTION('center_axis',(-1.,0.,-1.34163173959798E-15)) ;
#97285=DIRECTION('ref_axis',(-1.34163173959798E-15,0.,1.)) ;
#97286=DIRECTION('center_axis',(0.,0.,-1.)) ;
#97287=DIRECTION('ref_axis',(-1.,0.,0.)) ;
#97288=DIRECTION('center_axis',(-3.46944695195361E-14,3.4694469519536E-14,
1.)) ;
#97289=DIRECTION('ref_axis',(1.,-1.68611237719883E-42,3.46944695195361E-14)) ;
#97290=DIRECTION('center_axis',(0.577350269189625,-0.577350269189625,0.577350269189628)) ;
#97291=DIRECTION('ref_axis',(0.707106781186552,5.19478420936363E-15,-0.707106781186543)) ;
#97292=DIRECTION('center_axis',(0.577350269189625,-0.577350269189625,0.577350269189628)) ;
#97293=DIRECTION('ref_axis',(0.707106781186552,5.1349792556416E-15,-0.707106781186543)) ;
#97294=DIRECTION('center_axis',(2.08166817117218E-16,1.,0.)) ;
#97295=DIRECTION('ref_axis',(1.,0.,0.)) ;
#97296=DIRECTION('center_axis',(-0.577350269189646,0.577350269189609,0.577350269189623)) ;
#97297=DIRECTION('ref_axis',(-0.707106781186529,8.66006384940495E-15,-0.707106781186566)) ;
#97298=DIRECTION('center_axis',(0.,0.,-1.)) ;
#97299=DIRECTION('ref_axis',(-1.,0.,0.)) ;
#97300=DIRECTION('center_axis',(0.,0.,1.)) ;
#97301=DIRECTION('ref_axis',(-1.,0.,0.)) ;
#97302=DIRECTION('center_axis',(0.,0.,-1.)) ;
#97303=DIRECTION('ref_axis',(-1.,0.,0.)) ;
#97304=DIRECTION('center_axis',(-0.577350269189625,0.577350269189625,0.577350269189628)) ;
#97305=DIRECTION('ref_axis',(0.707106781186552,5.1349792556416E-15,0.707106781186543)) ;
#97306=DIRECTION('center_axis',(0.577350269189625,-0.577350269189625,-0.577350269189628)) ;
#97307=DIRECTION('ref_axis',(0.707106781186559,1.92955635991398E-14,0.707106781186536)) ;
#97308=DIRECTION('center_axis',(-0.577350269189625,0.577350269189626,-0.577350269189626)) ;
#97309=DIRECTION('ref_axis',(5.20172641667636E-15,0.70710678118655,0.707106781186545)) ;
#97310=DIRECTION('center_axis',(0.577350269189625,-0.577350269189626,0.577350269189626)) ;
#97311=DIRECTION('ref_axis',(1.27903606950626E-14,0.707106781186554,0.707106781186541)) ;
#97312=DIRECTION('center_axis',(0.577350269189636,-0.577350269189592,0.57735026918965)) ;
#97313=DIRECTION('ref_axis',(0.707106781186558,3.40611850366138E-15,-0.707106781186537)) ;
#97314=DIRECTION('center_axis',(0.,0.,-1.)) ;
#97315=DIRECTION('ref_axis',(-1.,0.,0.)) ;
#97316=DIRECTION('center_axis',(0.,0.,1.)) ;
#97317=DIRECTION('ref_axis',(-1.,1.57209315010398E-14,0.)) ;
#97318=DIRECTION('center_axis',(0.,0.,-1.)) ;
#97319=DIRECTION('ref_axis',(-1.,0.,0.)) ;
#97320=DIRECTION('center_axis',(0.,1.,0.)) ;
#97321=DIRECTION('ref_axis',(1.,0.,0.)) ;
#97322=DIRECTION('center_axis',(0.,-1.,7.76229792195976E-15)) ;
#97323=DIRECTION('ref_axis',(3.46944695195364E-14,7.76229792195976E-15,
1.)) ;
#97324=DIRECTION('center_axis',(-3.46944695195361E-14,3.46944695195361E-14,
1.)) ;
#97325=DIRECTION('ref_axis',(-7.17464813734306E-43,1.,-3.46944695195361E-14)) ;
#97326=DIRECTION('center_axis',(0.577350269189625,-0.577350269189626,-0.577350269189626)) ;
#97327=DIRECTION('ref_axis',(5.20172641667636E-15,0.70710678118655,-0.707106781186545)) ;
#97328=DIRECTION('center_axis',(0.577350269189625,-0.577350269189626,-0.577350269189626)) ;
#97329=DIRECTION('ref_axis',(5.11416588733871E-15,0.70710678118655,-0.707106781186545)) ;
#97330=DIRECTION('center_axis',(0.577350269189624,-0.577350269189625,-0.577350269189629)) ;
#97331=DIRECTION('ref_axis',(4.29556475679742E-15,0.707106781186552,-0.707106781186543)) ;
#97332=DIRECTION('center_axis',(0.,0.,-1.)) ;
#97333=DIRECTION('ref_axis',(-1.,0.,0.)) ;
#97334=DIRECTION('center_axis',(0.,0.,1.)) ;
#97335=DIRECTION('ref_axis',(1.,0.,0.)) ;
#97336=DIRECTION('center_axis',(0.,1.,1.95511867169518E-16)) ;
#97337=DIRECTION('ref_axis',(0.,-1.95511867169518E-16,1.)) ;
#97338=DIRECTION('center_axis',(-7.65717784317885E-15,-1.,-7.84883952026447E-15)) ;
#97339=DIRECTION('ref_axis',(-8.90241127119925E-32,7.84883952026447E-15,
-1.)) ;
#97340=DIRECTION('center_axis',(0.,1.,0.)) ;
#97341=DIRECTION('ref_axis',(1.,0.,0.)) ;
#97342=DIRECTION('center_axis',(-1.28749007982652E-15,-1.,1.47915175691198E-15)) ;
#97343=DIRECTION('ref_axis',(3.46944695195364E-14,1.47915175691194E-15,
1.)) ;
#97344=DIRECTION('center_axis',(0.,1.,0.)) ;
#97345=DIRECTION('ref_axis',(1.,0.,0.)) ;
#97346=DIRECTION('center_axis',(-0.577350269189619,-0.577350269189621,-0.577350269189638)) ;
#97347=DIRECTION('ref_axis',(1.66660234080318E-14,-0.707106781186566,0.707106781186529)) ;
#97348=DIRECTION('center_axis',(0.,0.,1.)) ;
#97349=DIRECTION('ref_axis',(-1.,-3.52365706057788E-15,0.)) ;
#97350=DIRECTION('center_axis',(0.,1.,-1.95511867169518E-16)) ;
#97351=DIRECTION('ref_axis',(0.,1.95511867169518E-16,1.)) ;
#97352=DIRECTION('center_axis',(0.,-1.,3.06658683336682E-15)) ;
#97353=DIRECTION('ref_axis',(0.,-3.06658683336682E-15,-1.)) ;
#97354=DIRECTION('center_axis',(0.,0.,-1.)) ;
#97355=DIRECTION('ref_axis',(-1.,0.,0.)) ;
#97356=DIRECTION('center_axis',(-3.4694469519536E-14,-3.46944695195361E-14,
1.)) ;
#97357=DIRECTION('ref_axis',(-8.96831017167883E-43,-1.,-3.46944695195361E-14)) ;
#97358=DIRECTION('center_axis',(0.577350269189625,0.577350269189626,0.577350269189627)) ;
#97359=DIRECTION('ref_axis',(5.35231302451417E-15,-0.707106781186551,0.707106781186544)) ;
#97360=DIRECTION('center_axis',(0.577350269189625,0.577350269189626,0.577350269189627)) ;
#97361=DIRECTION('ref_axis',(5.35231302451417E-15,-0.707106781186551,0.707106781186544)) ;
#97362=DIRECTION('center_axis',(0.,1.,0.)) ;
#97363=DIRECTION('ref_axis',(1.,0.,0.)) ;
#97364=DIRECTION('center_axis',(-0.577350269189609,-0.577350269189646,0.577350269189623)) ;
#97365=DIRECTION('ref_axis',(8.91337114590872E-15,0.707106781186529,0.707106781186566)) ;
#97366=DIRECTION('center_axis',(0.,0.,-1.)) ;
#97367=DIRECTION('ref_axis',(-1.,0.,0.)) ;
#97368=DIRECTION('center_axis',(0.,0.,1.)) ;
#97369=DIRECTION('ref_axis',(-1.,1.0842021724855E-15,0.)) ;
#97370=DIRECTION('center_axis',(0.,0.,-1.)) ;
#97371=DIRECTION('ref_axis',(-1.,0.,0.)) ;
#97372=DIRECTION('center_axis',(-0.577350269189625,-0.577350269189626,0.577350269189627)) ;
#97373=DIRECTION('ref_axis',(5.35231302451417E-15,-0.707106781186551,-0.707106781186544)) ;
#97374=DIRECTION('center_axis',(0.577350269189625,0.577350269189626,-0.577350269189627)) ;
#97375=DIRECTION('ref_axis',(-6.40836823623517E-14,-0.707106781186516,-0.707106781186579)) ;
#97376=DIRECTION('center_axis',(0.577350269189625,0.577350269189625,-0.577350269189628)) ;
#97377=DIRECTION('ref_axis',(-0.707106781186552,5.19478420936363E-15,-0.707106781186543)) ;
#97378=DIRECTION('center_axis',(-0.577350269189625,-0.577350269189625,0.577350269189628)) ;
#97379=DIRECTION('ref_axis',(-0.707106781186566,3.31891725521342E-14,-0.707106781186529)) ;
#97380=DIRECTION('center_axis',(-0.577350269189652,-0.577350269189606,0.57735026918962)) ;
#97381=DIRECTION('ref_axis',(0.707106781186528,-3.96520952299298E-16,0.707106781186567)) ;
#97382=DIRECTION('center_axis',(0.,0.,-1.)) ;
#97383=DIRECTION('ref_axis',(-1.,0.,0.)) ;
#97384=DIRECTION('center_axis',(0.,0.,1.)) ;
#97385=DIRECTION('ref_axis',(-1.,-8.67361737988404E-15,0.)) ;
#97386=DIRECTION('center_axis',(0.,0.,-1.)) ;
#97387=DIRECTION('ref_axis',(-1.,0.,0.)) ;
#97388=DIRECTION('center_axis',(2.08166817117218E-16,1.,0.)) ;
#97389=DIRECTION('ref_axis',(1.,0.,0.)) ;
#97390=DIRECTION('center_axis',(-1.,0.,-1.66745659064321E-14)) ;
#97391=DIRECTION('ref_axis',(1.66745659064321E-14,2.60208521396523E-14,
-1.)) ;
#97392=DIRECTION('center_axis',(-3.46944695195361E-14,-3.4694469519536E-14,
1.)) ;
#97393=DIRECTION('ref_axis',(-1.,-1.68611237719883E-42,-3.46944695195361E-14)) ;
#97394=DIRECTION('center_axis',(-0.577350269189625,-0.577350269189625,-0.577350269189628)) ;
#97395=DIRECTION('ref_axis',(-0.707106781186552,5.19478420936363E-15,0.707106781186543)) ;
#97396=DIRECTION('center_axis',(-0.577350269189625,-0.577350269189625,-0.577350269189628)) ;
#97397=DIRECTION('ref_axis',(-0.707106781186552,5.1349792556416E-15,0.707106781186543)) ;
#97398=DIRECTION('center_axis',(-0.577350269189626,-0.577350269189626,-0.577350269189626)) ;
#97399=DIRECTION('ref_axis',(0.707106781186547,-0.707106781186548,6.36902276417946E-16)) ;
#97400=DIRECTION('center_axis',(0.,0.,-1.)) ;
#97401=DIRECTION('ref_axis',(-1.,0.,0.)) ;
#97402=DIRECTION('center_axis',(0.,0.,1.)) ;
#97403=DIRECTION('ref_axis',(1.,0.,0.)) ;
#97404=DIRECTION('center_axis',(-1.,0.,9.8563833862319E-18)) ;
#97405=DIRECTION('ref_axis',(9.8563833862319E-18,0.,1.)) ;
#97406=DIRECTION('center_axis',(-1.,8.87690528722497E-15,-8.87690528722518E-15)) ;
#97407=DIRECTION('ref_axis',(-8.87690528722518E-15,4.48415508583942E-43,
1.)) ;
#97408=DIRECTION('center_axis',(2.08166817117218E-16,1.,0.)) ;
#97409=DIRECTION('ref_axis',(1.,0.,0.)) ;
#97410=DIRECTION('center_axis',(-1.,8.53809210832325E-15,8.53809210832346E-15)) ;
#97411=DIRECTION('ref_axis',(-8.53809210832339E-15,8.67361737988409E-15,
-1.)) ;
#97412=DIRECTION('center_axis',(2.08166817117218E-16,1.,0.)) ;
#97413=DIRECTION('ref_axis',(1.,0.,0.)) ;
#97414=DIRECTION('center_axis',(-0.577350269189622,0.577350269189621,-0.577350269189634)) ;
#97415=DIRECTION('ref_axis',(0.707106781186563,1.66970714627838E-14,-0.707106781186532)) ;
#97416=DIRECTION('center_axis',(0.,0.,1.)) ;
#97417=DIRECTION('ref_axis',(-1.,0.,0.)) ;
#97418=DIRECTION('center_axis',(-1.,0.,-9.8563833862319E-18)) ;
#97419=DIRECTION('ref_axis',(-9.8563833862319E-18,0.,1.)) ;
#97420=DIRECTION('center_axis',(-1.,0.,-1.34163173959798E-15)) ;
#97421=DIRECTION('ref_axis',(-1.34163173959798E-15,0.,1.)) ;
#97422=DIRECTION('center_axis',(0.,0.,-1.)) ;
#97423=DIRECTION('ref_axis',(-1.,0.,0.)) ;
#97424=DIRECTION('center_axis',(-3.46944695195361E-14,3.4694469519536E-14,
1.)) ;
#97425=DIRECTION('ref_axis',(1.,-1.68611237719883E-42,3.46944695195361E-14)) ;
#97426=DIRECTION('center_axis',(0.577350269189625,-0.577350269189625,0.577350269189628)) ;
#97427=DIRECTION('ref_axis',(0.707106781186552,5.19478420936363E-15,-0.707106781186543)) ;
#97428=DIRECTION('center_axis',(0.577350269189625,-0.577350269189625,0.577350269189628)) ;
#97429=DIRECTION('ref_axis',(0.707106781186552,5.1349792556416E-15,-0.707106781186543)) ;
#97430=DIRECTION('center_axis',(2.08166817117218E-16,1.,0.)) ;
#97431=DIRECTION('ref_axis',(1.,0.,0.)) ;
#97432=DIRECTION('center_axis',(-0.577350269189646,0.577350269189609,0.577350269189623)) ;
#97433=DIRECTION('ref_axis',(-0.707106781186529,8.66006384940495E-15,-0.707106781186566)) ;
#97434=DIRECTION('center_axis',(0.,0.,-1.)) ;
#97435=DIRECTION('ref_axis',(-1.,0.,0.)) ;
#97436=DIRECTION('center_axis',(0.,0.,1.)) ;
#97437=DIRECTION('ref_axis',(-1.,0.,0.)) ;
#97438=DIRECTION('center_axis',(0.,0.,-1.)) ;
#97439=DIRECTION('ref_axis',(-1.,0.,0.)) ;
#97440=DIRECTION('center_axis',(-0.577350269189625,0.577350269189625,0.577350269189628)) ;
#97441=DIRECTION('ref_axis',(0.707106781186552,5.1349792556416E-15,0.707106781186543)) ;
#97442=DIRECTION('center_axis',(0.577350269189625,-0.577350269189625,-0.577350269189628)) ;
#97443=DIRECTION('ref_axis',(0.707106781186559,1.92955635991398E-14,0.707106781186536)) ;
#97444=DIRECTION('center_axis',(-0.577350269189625,0.577350269189626,-0.577350269189626)) ;
#97445=DIRECTION('ref_axis',(5.20172641667636E-15,0.70710678118655,0.707106781186545)) ;
#97446=DIRECTION('center_axis',(0.577350269189625,-0.577350269189626,0.577350269189626)) ;
#97447=DIRECTION('ref_axis',(1.27903606950626E-14,0.707106781186554,0.707106781186541)) ;
#97448=DIRECTION('center_axis',(0.577350269189636,-0.577350269189592,0.57735026918965)) ;
#97449=DIRECTION('ref_axis',(0.707106781186558,3.40611850366138E-15,-0.707106781186537)) ;
#97450=DIRECTION('center_axis',(0.,0.,-1.)) ;
#97451=DIRECTION('ref_axis',(-1.,0.,0.)) ;
#97452=DIRECTION('center_axis',(0.,0.,1.)) ;
#97453=DIRECTION('ref_axis',(-1.,1.57209315010398E-14,0.)) ;
#97454=DIRECTION('center_axis',(0.,0.,-1.)) ;
#97455=DIRECTION('ref_axis',(-1.,0.,0.)) ;
#97456=DIRECTION('center_axis',(0.,1.,0.)) ;
#97457=DIRECTION('ref_axis',(1.,0.,0.)) ;
#97458=DIRECTION('center_axis',(0.,-1.,7.76229792195976E-15)) ;
#97459=DIRECTION('ref_axis',(3.46944695195364E-14,7.76229792195976E-15,
1.)) ;
#97460=DIRECTION('center_axis',(-3.46944695195361E-14,3.46944695195361E-14,
1.)) ;
#97461=DIRECTION('ref_axis',(-7.17464813734306E-43,1.,-3.46944695195361E-14)) ;
#97462=DIRECTION('center_axis',(0.577350269189625,-0.577350269189626,-0.577350269189626)) ;
#97463=DIRECTION('ref_axis',(5.20172641667636E-15,0.70710678118655,-0.707106781186545)) ;
#97464=DIRECTION('center_axis',(0.577350269189625,-0.577350269189626,-0.577350269189626)) ;
#97465=DIRECTION('ref_axis',(5.11416588733871E-15,0.70710678118655,-0.707106781186545)) ;
#97466=DIRECTION('center_axis',(0.577350269189624,-0.577350269189625,-0.577350269189629)) ;
#97467=DIRECTION('ref_axis',(4.29556475679742E-15,0.707106781186552,-0.707106781186543)) ;
#97468=DIRECTION('center_axis',(0.,0.,-1.)) ;
#97469=DIRECTION('ref_axis',(-1.,0.,0.)) ;
#97470=DIRECTION('center_axis',(0.,0.,1.)) ;
#97471=DIRECTION('ref_axis',(1.,0.,0.)) ;
#97472=DIRECTION('center_axis',(0.,1.,1.95511867169518E-16)) ;
#97473=DIRECTION('ref_axis',(0.,-1.95511867169518E-16,1.)) ;
#97474=DIRECTION('center_axis',(-7.65717784317885E-15,-1.,-7.84883952026447E-15)) ;
#97475=DIRECTION('ref_axis',(-8.90241127119925E-32,7.84883952026447E-15,
-1.)) ;
#97476=DIRECTION('center_axis',(0.,1.,0.)) ;
#97477=DIRECTION('ref_axis',(1.,0.,0.)) ;
#97478=DIRECTION('center_axis',(-1.28749007982652E-15,-1.,1.47915175691198E-15)) ;
#97479=DIRECTION('ref_axis',(3.46944695195364E-14,1.47915175691194E-15,
1.)) ;
#97480=DIRECTION('center_axis',(0.,1.,0.)) ;
#97481=DIRECTION('ref_axis',(1.,0.,0.)) ;
#97482=DIRECTION('center_axis',(-0.577350269189619,-0.577350269189621,-0.577350269189638)) ;
#97483=DIRECTION('ref_axis',(1.66660234080318E-14,-0.707106781186566,0.707106781186529)) ;
#97484=DIRECTION('center_axis',(0.,0.,1.)) ;
#97485=DIRECTION('ref_axis',(-1.,-3.52365706057788E-15,0.)) ;
#97486=DIRECTION('center_axis',(0.,1.,-1.95511867169518E-16)) ;
#97487=DIRECTION('ref_axis',(0.,1.95511867169518E-16,1.)) ;
#97488=DIRECTION('center_axis',(0.,-1.,3.06658683336682E-15)) ;
#97489=DIRECTION('ref_axis',(0.,-3.06658683336682E-15,-1.)) ;
#97490=DIRECTION('center_axis',(0.,0.,-1.)) ;
#97491=DIRECTION('ref_axis',(-1.,0.,0.)) ;
#97492=DIRECTION('center_axis',(-3.4694469519536E-14,-3.46944695195361E-14,
1.)) ;
#97493=DIRECTION('ref_axis',(-8.96831017167883E-43,-1.,-3.46944695195361E-14)) ;
#97494=DIRECTION('center_axis',(0.577350269189625,0.577350269189626,0.577350269189627)) ;
#97495=DIRECTION('ref_axis',(5.35231302451417E-15,-0.707106781186551,0.707106781186544)) ;
#97496=DIRECTION('center_axis',(0.577350269189625,0.577350269189626,0.577350269189627)) ;
#97497=DIRECTION('ref_axis',(5.35231302451417E-15,-0.707106781186551,0.707106781186544)) ;
#97498=DIRECTION('center_axis',(0.,1.,0.)) ;
#97499=DIRECTION('ref_axis',(1.,0.,0.)) ;
#97500=DIRECTION('center_axis',(-0.577350269189609,-0.577350269189646,0.577350269189623)) ;
#97501=DIRECTION('ref_axis',(8.91337114590872E-15,0.707106781186529,0.707106781186566)) ;
#97502=DIRECTION('center_axis',(0.,0.,-1.)) ;
#97503=DIRECTION('ref_axis',(-1.,0.,0.)) ;
#97504=DIRECTION('center_axis',(0.,0.,1.)) ;
#97505=DIRECTION('ref_axis',(-1.,1.0842021724855E-15,0.)) ;
#97506=DIRECTION('center_axis',(0.,0.,-1.)) ;
#97507=DIRECTION('ref_axis',(-1.,0.,0.)) ;
#97508=DIRECTION('center_axis',(-0.577350269189625,-0.577350269189626,0.577350269189627)) ;
#97509=DIRECTION('ref_axis',(5.35231302451417E-15,-0.707106781186551,-0.707106781186544)) ;
#97510=DIRECTION('center_axis',(0.577350269189625,0.577350269189626,-0.577350269189627)) ;
#97511=DIRECTION('ref_axis',(-6.40836823623517E-14,-0.707106781186516,-0.707106781186579)) ;
#97512=DIRECTION('center_axis',(0.577350269189625,0.577350269189625,-0.577350269189628)) ;
#97513=DIRECTION('ref_axis',(-0.707106781186552,5.19478420936363E-15,-0.707106781186543)) ;
#97514=DIRECTION('center_axis',(-0.577350269189625,-0.577350269189625,0.577350269189628)) ;
#97515=DIRECTION('ref_axis',(-0.707106781186566,3.31891725521342E-14,-0.707106781186529)) ;
#97516=DIRECTION('center_axis',(-0.577350269189652,-0.577350269189606,0.57735026918962)) ;
#97517=DIRECTION('ref_axis',(0.707106781186528,-3.96520952299298E-16,0.707106781186567)) ;
#97518=DIRECTION('center_axis',(0.,0.,-1.)) ;
#97519=DIRECTION('ref_axis',(-1.,0.,0.)) ;
#97520=DIRECTION('center_axis',(0.,0.,1.)) ;
#97521=DIRECTION('ref_axis',(-1.,-8.67361737988404E-15,0.)) ;
#97522=DIRECTION('center_axis',(0.,0.,-1.)) ;
#97523=DIRECTION('ref_axis',(-1.,0.,0.)) ;
#97524=DIRECTION('center_axis',(2.08166817117218E-16,1.,0.)) ;
#97525=DIRECTION('ref_axis',(1.,0.,0.)) ;
#97526=DIRECTION('center_axis',(-1.,0.,-1.66745659064321E-14)) ;
#97527=DIRECTION('ref_axis',(1.66745659064321E-14,2.60208521396523E-14,
-1.)) ;
#97528=DIRECTION('center_axis',(-3.46944695195361E-14,-3.4694469519536E-14,
1.)) ;
#97529=DIRECTION('ref_axis',(-1.,-1.68611237719883E-42,-3.46944695195361E-14)) ;
#97530=DIRECTION('center_axis',(-0.577350269189625,-0.577350269189625,-0.577350269189628)) ;
#97531=DIRECTION('ref_axis',(-0.707106781186552,5.19478420936363E-15,0.707106781186543)) ;
#97532=DIRECTION('center_axis',(-0.577350269189625,-0.577350269189625,-0.577350269189628)) ;
#97533=DIRECTION('ref_axis',(-0.707106781186552,5.1349792556416E-15,0.707106781186543)) ;
#97534=DIRECTION('center_axis',(-0.577350269189626,-0.577350269189626,-0.577350269189626)) ;
#97535=DIRECTION('ref_axis',(0.707106781186547,-0.707106781186548,6.36902276417946E-16)) ;
#97536=DIRECTION('center_axis',(0.,0.,-1.)) ;
#97537=DIRECTION('ref_axis',(-1.,0.,0.)) ;
#97538=DIRECTION('center_axis',(0.,0.,1.)) ;
#97539=DIRECTION('ref_axis',(1.,0.,0.)) ;
#97540=DIRECTION('center_axis',(-1.,0.,9.8563833862319E-18)) ;
#97541=DIRECTION('ref_axis',(9.8563833862319E-18,0.,1.)) ;
#97542=DIRECTION('center_axis',(-1.,8.87690528722497E-15,-8.87690528722518E-15)) ;
#97543=DIRECTION('ref_axis',(-8.87690528722518E-15,4.48415508583942E-43,
1.)) ;
#97544=DIRECTION('center_axis',(2.08166817117218E-16,1.,0.)) ;
#97545=DIRECTION('ref_axis',(1.,0.,0.)) ;
#97546=DIRECTION('center_axis',(-1.,8.53809210832325E-15,8.53809210832346E-15)) ;
#97547=DIRECTION('ref_axis',(-8.53809210832339E-15,8.67361737988409E-15,
-1.)) ;
#97548=DIRECTION('center_axis',(2.08166817117218E-16,1.,0.)) ;
#97549=DIRECTION('ref_axis',(1.,0.,0.)) ;
#97550=DIRECTION('center_axis',(-0.577350269189622,0.577350269189621,-0.577350269189634)) ;
#97551=DIRECTION('ref_axis',(0.707106781186563,1.66970714627838E-14,-0.707106781186532)) ;
#97552=DIRECTION('center_axis',(0.,0.,1.)) ;
#97553=DIRECTION('ref_axis',(-1.,0.,0.)) ;
#97554=DIRECTION('center_axis',(-1.,0.,-9.8563833862319E-18)) ;
#97555=DIRECTION('ref_axis',(-9.8563833862319E-18,0.,1.)) ;
#97556=DIRECTION('center_axis',(-1.,0.,-1.34163173959798E-15)) ;
#97557=DIRECTION('ref_axis',(-1.34163173959798E-15,0.,1.)) ;
#97558=DIRECTION('center_axis',(0.,0.,-1.)) ;
#97559=DIRECTION('ref_axis',(-1.,0.,0.)) ;
#97560=DIRECTION('center_axis',(-3.46944695195361E-14,3.4694469519536E-14,
1.)) ;
#97561=DIRECTION('ref_axis',(1.,-1.68611237719883E-42,3.46944695195361E-14)) ;
#97562=DIRECTION('center_axis',(0.577350269189625,-0.577350269189625,0.577350269189628)) ;
#97563=DIRECTION('ref_axis',(0.707106781186552,5.19478420936363E-15,-0.707106781186543)) ;
#97564=DIRECTION('center_axis',(0.577350269189625,-0.577350269189625,0.577350269189628)) ;
#97565=DIRECTION('ref_axis',(0.707106781186552,5.1349792556416E-15,-0.707106781186543)) ;
#97566=DIRECTION('center_axis',(2.08166817117218E-16,1.,0.)) ;
#97567=DIRECTION('ref_axis',(1.,0.,0.)) ;
#97568=DIRECTION('center_axis',(-0.577350269189646,0.577350269189609,0.577350269189623)) ;
#97569=DIRECTION('ref_axis',(-0.707106781186529,8.66006384940495E-15,-0.707106781186566)) ;
#97570=DIRECTION('center_axis',(0.,0.,-1.)) ;
#97571=DIRECTION('ref_axis',(-1.,0.,0.)) ;
#97572=DIRECTION('center_axis',(0.,0.,1.)) ;
#97573=DIRECTION('ref_axis',(-1.,0.,0.)) ;
#97574=DIRECTION('center_axis',(0.,0.,-1.)) ;
#97575=DIRECTION('ref_axis',(-1.,0.,0.)) ;
#97576=DIRECTION('center_axis',(-0.577350269189625,0.577350269189625,0.577350269189628)) ;
#97577=DIRECTION('ref_axis',(0.707106781186552,5.1349792556416E-15,0.707106781186543)) ;
#97578=DIRECTION('center_axis',(0.577350269189625,-0.577350269189625,-0.577350269189628)) ;
#97579=DIRECTION('ref_axis',(0.707106781186559,1.92955635991398E-14,0.707106781186536)) ;
#97580=DIRECTION('center_axis',(-0.577350269189625,0.577350269189626,-0.577350269189626)) ;
#97581=DIRECTION('ref_axis',(5.20172641667636E-15,0.70710678118655,0.707106781186545)) ;
#97582=DIRECTION('center_axis',(0.577350269189625,-0.577350269189626,0.577350269189626)) ;
#97583=DIRECTION('ref_axis',(1.27903606950626E-14,0.707106781186554,0.707106781186541)) ;
#97584=DIRECTION('center_axis',(0.577350269189636,-0.577350269189592,0.57735026918965)) ;
#97585=DIRECTION('ref_axis',(0.707106781186558,3.40611850366138E-15,-0.707106781186537)) ;
#97586=DIRECTION('center_axis',(0.,0.,-1.)) ;
#97587=DIRECTION('ref_axis',(-1.,0.,0.)) ;
#97588=DIRECTION('center_axis',(0.,0.,1.)) ;
#97589=DIRECTION('ref_axis',(-1.,1.57209315010398E-14,0.)) ;
#97590=DIRECTION('center_axis',(0.,0.,-1.)) ;
#97591=DIRECTION('ref_axis',(-1.,0.,0.)) ;
#97592=DIRECTION('center_axis',(0.,1.,0.)) ;
#97593=DIRECTION('ref_axis',(1.,0.,0.)) ;
#97594=DIRECTION('center_axis',(0.,-1.,7.76229792195976E-15)) ;
#97595=DIRECTION('ref_axis',(3.46944695195364E-14,7.76229792195976E-15,
1.)) ;
#97596=DIRECTION('center_axis',(-3.46944695195361E-14,3.46944695195361E-14,
1.)) ;
#97597=DIRECTION('ref_axis',(-7.17464813734306E-43,1.,-3.46944695195361E-14)) ;
#97598=DIRECTION('center_axis',(0.577350269189625,-0.577350269189626,-0.577350269189626)) ;
#97599=DIRECTION('ref_axis',(5.20172641667636E-15,0.70710678118655,-0.707106781186545)) ;
#97600=DIRECTION('center_axis',(0.577350269189625,-0.577350269189626,-0.577350269189626)) ;
#97601=DIRECTION('ref_axis',(5.11416588733871E-15,0.70710678118655,-0.707106781186545)) ;
#97602=DIRECTION('center_axis',(0.577350269189624,-0.577350269189625,-0.577350269189629)) ;
#97603=DIRECTION('ref_axis',(4.29556475679742E-15,0.707106781186552,-0.707106781186543)) ;
#97604=DIRECTION('center_axis',(0.,0.,-1.)) ;
#97605=DIRECTION('ref_axis',(-1.,0.,0.)) ;
#97606=DIRECTION('center_axis',(0.,0.,1.)) ;
#97607=DIRECTION('ref_axis',(1.,0.,0.)) ;
#97608=DIRECTION('center_axis',(0.,1.,1.95511867169518E-16)) ;
#97609=DIRECTION('ref_axis',(0.,-1.95511867169518E-16,1.)) ;
#97610=DIRECTION('center_axis',(-7.65717784317885E-15,-1.,-7.84883952026447E-15)) ;
#97611=DIRECTION('ref_axis',(-8.90241127119925E-32,7.84883952026447E-15,
-1.)) ;
#97612=DIRECTION('center_axis',(0.,1.,0.)) ;
#97613=DIRECTION('ref_axis',(1.,0.,0.)) ;
#97614=DIRECTION('center_axis',(-1.28749007982652E-15,-1.,1.47915175691198E-15)) ;
#97615=DIRECTION('ref_axis',(3.46944695195364E-14,1.47915175691194E-15,
1.)) ;
#97616=DIRECTION('center_axis',(0.,1.,0.)) ;
#97617=DIRECTION('ref_axis',(1.,0.,0.)) ;
#97618=DIRECTION('center_axis',(-0.577350269189619,-0.577350269189621,-0.577350269189638)) ;
#97619=DIRECTION('ref_axis',(1.66660234080318E-14,-0.707106781186566,0.707106781186529)) ;
#97620=DIRECTION('center_axis',(0.,0.,1.)) ;
#97621=DIRECTION('ref_axis',(-1.,-3.52365706057788E-15,0.)) ;
#97622=DIRECTION('center_axis',(0.,1.,-1.95511867169518E-16)) ;
#97623=DIRECTION('ref_axis',(0.,1.95511867169518E-16,1.)) ;
#97624=DIRECTION('center_axis',(0.,-1.,3.06658683336682E-15)) ;
#97625=DIRECTION('ref_axis',(0.,-3.06658683336682E-15,-1.)) ;
#97626=DIRECTION('center_axis',(0.,0.,-1.)) ;
#97627=DIRECTION('ref_axis',(-1.,0.,0.)) ;
#97628=DIRECTION('center_axis',(-3.4694469519536E-14,-3.46944695195361E-14,
1.)) ;
#97629=DIRECTION('ref_axis',(-8.96831017167883E-43,-1.,-3.46944695195361E-14)) ;
#97630=DIRECTION('center_axis',(0.577350269189625,0.577350269189626,0.577350269189627)) ;
#97631=DIRECTION('ref_axis',(5.35231302451417E-15,-0.707106781186551,0.707106781186544)) ;
#97632=DIRECTION('center_axis',(0.577350269189625,0.577350269189626,0.577350269189627)) ;
#97633=DIRECTION('ref_axis',(5.35231302451417E-15,-0.707106781186551,0.707106781186544)) ;
#97634=DIRECTION('center_axis',(0.,1.,0.)) ;
#97635=DIRECTION('ref_axis',(1.,0.,0.)) ;
#97636=DIRECTION('center_axis',(-0.577350269189609,-0.577350269189646,0.577350269189623)) ;
#97637=DIRECTION('ref_axis',(8.91337114590872E-15,0.707106781186529,0.707106781186566)) ;
#97638=DIRECTION('center_axis',(0.,0.,-1.)) ;
#97639=DIRECTION('ref_axis',(-1.,0.,0.)) ;
#97640=DIRECTION('center_axis',(0.,0.,1.)) ;
#97641=DIRECTION('ref_axis',(-1.,1.0842021724855E-15,0.)) ;
#97642=DIRECTION('center_axis',(0.,0.,-1.)) ;
#97643=DIRECTION('ref_axis',(-1.,0.,0.)) ;
#97644=DIRECTION('center_axis',(-0.577350269189625,-0.577350269189626,0.577350269189627)) ;
#97645=DIRECTION('ref_axis',(5.35231302451417E-15,-0.707106781186551,-0.707106781186544)) ;
#97646=DIRECTION('center_axis',(0.577350269189625,0.577350269189626,-0.577350269189627)) ;
#97647=DIRECTION('ref_axis',(-6.40836823623517E-14,-0.707106781186516,-0.707106781186579)) ;
#97648=DIRECTION('center_axis',(0.577350269189625,0.577350269189625,-0.577350269189628)) ;
#97649=DIRECTION('ref_axis',(-0.707106781186552,5.19478420936363E-15,-0.707106781186543)) ;
#97650=DIRECTION('center_axis',(-0.577350269189625,-0.577350269189625,0.577350269189628)) ;
#97651=DIRECTION('ref_axis',(-0.707106781186566,3.31891725521342E-14,-0.707106781186529)) ;
#97652=DIRECTION('center_axis',(-0.577350269189652,-0.577350269189606,0.57735026918962)) ;
#97653=DIRECTION('ref_axis',(0.707106781186528,-3.96520952299298E-16,0.707106781186567)) ;
#97654=DIRECTION('center_axis',(0.,0.,-1.)) ;
#97655=DIRECTION('ref_axis',(-1.,0.,0.)) ;
#97656=DIRECTION('center_axis',(0.,0.,1.)) ;
#97657=DIRECTION('ref_axis',(-1.,-8.67361737988404E-15,0.)) ;
#97658=DIRECTION('center_axis',(0.,0.,-1.)) ;
#97659=DIRECTION('ref_axis',(-1.,0.,0.)) ;
#97660=DIRECTION('center_axis',(2.08166817117218E-16,1.,0.)) ;
#97661=DIRECTION('ref_axis',(1.,0.,0.)) ;
#97662=DIRECTION('center_axis',(-1.,0.,-1.66745659064321E-14)) ;
#97663=DIRECTION('ref_axis',(1.66745659064321E-14,2.60208521396523E-14,
-1.)) ;
#97664=DIRECTION('center_axis',(-3.46944695195361E-14,-3.4694469519536E-14,
1.)) ;
#97665=DIRECTION('ref_axis',(-1.,-1.68611237719883E-42,-3.46944695195361E-14)) ;
#97666=DIRECTION('center_axis',(-0.577350269189625,-0.577350269189625,-0.577350269189628)) ;
#97667=DIRECTION('ref_axis',(-0.707106781186552,5.19478420936363E-15,0.707106781186543)) ;
#97668=DIRECTION('center_axis',(-0.577350269189625,-0.577350269189625,-0.577350269189628)) ;
#97669=DIRECTION('ref_axis',(-0.707106781186552,5.1349792556416E-15,0.707106781186543)) ;
#97670=DIRECTION('center_axis',(-0.577350269189626,-0.577350269189626,-0.577350269189626)) ;
#97671=DIRECTION('ref_axis',(0.707106781186547,-0.707106781186548,6.36902276417946E-16)) ;
#97672=DIRECTION('center_axis',(0.,0.,-1.)) ;
#97673=DIRECTION('ref_axis',(-1.,0.,0.)) ;
#97674=DIRECTION('center_axis',(0.,0.,1.)) ;
#97675=DIRECTION('ref_axis',(1.,0.,0.)) ;
#97676=DIRECTION('center_axis',(-1.,0.,9.8563833862319E-18)) ;
#97677=DIRECTION('ref_axis',(9.8563833862319E-18,0.,1.)) ;
#97678=DIRECTION('center_axis',(-1.,8.87690528722497E-15,-8.87690528722518E-15)) ;
#97679=DIRECTION('ref_axis',(-8.87690528722518E-15,4.48415508583942E-43,
1.)) ;
#97680=DIRECTION('center_axis',(2.08166817117218E-16,1.,0.)) ;
#97681=DIRECTION('ref_axis',(1.,0.,0.)) ;
#97682=DIRECTION('center_axis',(-1.,8.53809210832325E-15,8.53809210832346E-15)) ;
#97683=DIRECTION('ref_axis',(-8.53809210832339E-15,8.67361737988409E-15,
-1.)) ;
#97684=DIRECTION('center_axis',(2.08166817117218E-16,1.,0.)) ;
#97685=DIRECTION('ref_axis',(1.,0.,0.)) ;
#97686=DIRECTION('center_axis',(-0.577350269189622,0.577350269189621,-0.577350269189634)) ;
#97687=DIRECTION('ref_axis',(0.707106781186563,1.66970714627838E-14,-0.707106781186532)) ;
#97688=DIRECTION('center_axis',(0.,0.,1.)) ;
#97689=DIRECTION('ref_axis',(-1.,0.,0.)) ;
#97690=DIRECTION('center_axis',(-1.,0.,-9.8563833862319E-18)) ;
#97691=DIRECTION('ref_axis',(-9.8563833862319E-18,0.,1.)) ;
#97692=DIRECTION('center_axis',(-1.,0.,-1.34163173959798E-15)) ;
#97693=DIRECTION('ref_axis',(-1.34163173959798E-15,0.,1.)) ;
#97694=DIRECTION('center_axis',(0.,0.,-1.)) ;
#97695=DIRECTION('ref_axis',(-1.,0.,0.)) ;
#97696=DIRECTION('center_axis',(-3.46944695195361E-14,3.4694469519536E-14,
1.)) ;
#97697=DIRECTION('ref_axis',(1.,-1.68611237719883E-42,3.46944695195361E-14)) ;
#97698=DIRECTION('center_axis',(0.577350269189625,-0.577350269189625,0.577350269189628)) ;
#97699=DIRECTION('ref_axis',(0.707106781186552,5.19478420936363E-15,-0.707106781186543)) ;
#97700=DIRECTION('center_axis',(0.577350269189625,-0.577350269189625,0.577350269189628)) ;
#97701=DIRECTION('ref_axis',(0.707106781186552,5.1349792556416E-15,-0.707106781186543)) ;
#97702=DIRECTION('center_axis',(2.08166817117218E-16,1.,0.)) ;
#97703=DIRECTION('ref_axis',(1.,0.,0.)) ;
#97704=DIRECTION('center_axis',(-0.577350269189646,0.577350269189609,0.577350269189623)) ;
#97705=DIRECTION('ref_axis',(-0.707106781186529,8.66006384940495E-15,-0.707106781186566)) ;
#97706=DIRECTION('center_axis',(0.,0.,-1.)) ;
#97707=DIRECTION('ref_axis',(-1.,0.,0.)) ;
#97708=DIRECTION('center_axis',(0.,0.,1.)) ;
#97709=DIRECTION('ref_axis',(-1.,0.,0.)) ;
#97710=DIRECTION('center_axis',(0.,0.,-1.)) ;
#97711=DIRECTION('ref_axis',(-1.,0.,0.)) ;
#97712=DIRECTION('center_axis',(-0.577350269189625,0.577350269189625,0.577350269189628)) ;
#97713=DIRECTION('ref_axis',(0.707106781186552,5.1349792556416E-15,0.707106781186543)) ;
#97714=DIRECTION('center_axis',(0.577350269189625,-0.577350269189625,-0.577350269189628)) ;
#97715=DIRECTION('ref_axis',(0.707106781186559,1.92955635991398E-14,0.707106781186536)) ;
#97716=DIRECTION('center_axis',(-0.577350269189625,0.577350269189626,-0.577350269189626)) ;
#97717=DIRECTION('ref_axis',(5.20172641667636E-15,0.70710678118655,0.707106781186545)) ;
#97718=DIRECTION('center_axis',(0.577350269189625,-0.577350269189626,0.577350269189626)) ;
#97719=DIRECTION('ref_axis',(1.27903606950626E-14,0.707106781186554,0.707106781186541)) ;
#97720=DIRECTION('center_axis',(0.577350269189636,-0.577350269189592,0.57735026918965)) ;
#97721=DIRECTION('ref_axis',(0.707106781186558,3.40611850366138E-15,-0.707106781186537)) ;
#97722=DIRECTION('center_axis',(0.,0.,-1.)) ;
#97723=DIRECTION('ref_axis',(-1.,0.,0.)) ;
#97724=DIRECTION('center_axis',(0.,0.,1.)) ;
#97725=DIRECTION('ref_axis',(-1.,1.57209315010398E-14,0.)) ;
#97726=DIRECTION('center_axis',(0.,0.,-1.)) ;
#97727=DIRECTION('ref_axis',(-1.,0.,0.)) ;
#97728=DIRECTION('center_axis',(0.,1.,0.)) ;
#97729=DIRECTION('ref_axis',(1.,0.,0.)) ;
#97730=DIRECTION('center_axis',(0.,-1.,7.76229792195976E-15)) ;
#97731=DIRECTION('ref_axis',(3.46944695195364E-14,7.76229792195976E-15,
1.)) ;
#97732=DIRECTION('center_axis',(-3.46944695195361E-14,3.46944695195361E-14,
1.)) ;
#97733=DIRECTION('ref_axis',(-7.17464813734306E-43,1.,-3.46944695195361E-14)) ;
#97734=DIRECTION('center_axis',(0.577350269189625,-0.577350269189626,-0.577350269189626)) ;
#97735=DIRECTION('ref_axis',(5.20172641667636E-15,0.70710678118655,-0.707106781186545)) ;
#97736=DIRECTION('center_axis',(0.577350269189625,-0.577350269189626,-0.577350269189626)) ;
#97737=DIRECTION('ref_axis',(5.11416588733871E-15,0.70710678118655,-0.707106781186545)) ;
#97738=DIRECTION('center_axis',(0.577350269189624,-0.577350269189625,-0.577350269189629)) ;
#97739=DIRECTION('ref_axis',(4.29556475679742E-15,0.707106781186552,-0.707106781186543)) ;
#97740=DIRECTION('center_axis',(0.,0.,-1.)) ;
#97741=DIRECTION('ref_axis',(-1.,0.,0.)) ;
#97742=DIRECTION('center_axis',(0.,0.,1.)) ;
#97743=DIRECTION('ref_axis',(1.,0.,0.)) ;
#97744=DIRECTION('center_axis',(0.,1.,1.95511867169518E-16)) ;
#97745=DIRECTION('ref_axis',(0.,-1.95511867169518E-16,1.)) ;
#97746=DIRECTION('center_axis',(-7.65717784317885E-15,-1.,-7.84883952026447E-15)) ;
#97747=DIRECTION('ref_axis',(-8.90241127119925E-32,7.84883952026447E-15,
-1.)) ;
#97748=DIRECTION('center_axis',(0.,1.,0.)) ;
#97749=DIRECTION('ref_axis',(1.,0.,0.)) ;
#97750=DIRECTION('center_axis',(-1.28749007982652E-15,-1.,1.47915175691198E-15)) ;
#97751=DIRECTION('ref_axis',(3.46944695195364E-14,1.47915175691194E-15,
1.)) ;
#97752=DIRECTION('center_axis',(0.,1.,0.)) ;
#97753=DIRECTION('ref_axis',(1.,0.,0.)) ;
#97754=DIRECTION('center_axis',(-0.577350269189619,-0.577350269189621,-0.577350269189638)) ;
#97755=DIRECTION('ref_axis',(1.66660234080318E-14,-0.707106781186566,0.707106781186529)) ;
#97756=DIRECTION('center_axis',(0.,0.,1.)) ;
#97757=DIRECTION('ref_axis',(-1.,-3.52365706057788E-15,0.)) ;
#97758=DIRECTION('center_axis',(0.,1.,-1.95511867169518E-16)) ;
#97759=DIRECTION('ref_axis',(0.,1.95511867169518E-16,1.)) ;
#97760=DIRECTION('center_axis',(0.,-1.,3.06658683336682E-15)) ;
#97761=DIRECTION('ref_axis',(0.,-3.06658683336682E-15,-1.)) ;
#97762=DIRECTION('center_axis',(0.,0.,-1.)) ;
#97763=DIRECTION('ref_axis',(-1.,0.,0.)) ;
#97764=DIRECTION('center_axis',(-3.4694469519536E-14,-3.46944695195361E-14,
1.)) ;
#97765=DIRECTION('ref_axis',(-8.96831017167883E-43,-1.,-3.46944695195361E-14)) ;
#97766=DIRECTION('center_axis',(0.577350269189625,0.577350269189626,0.577350269189627)) ;
#97767=DIRECTION('ref_axis',(5.35231302451417E-15,-0.707106781186551,0.707106781186544)) ;
#97768=DIRECTION('center_axis',(0.577350269189625,0.577350269189626,0.577350269189627)) ;
#97769=DIRECTION('ref_axis',(5.35231302451417E-15,-0.707106781186551,0.707106781186544)) ;
#97770=DIRECTION('center_axis',(0.,1.,0.)) ;
#97771=DIRECTION('ref_axis',(1.,0.,0.)) ;
#97772=DIRECTION('center_axis',(-0.577350269189609,-0.577350269189646,0.577350269189623)) ;
#97773=DIRECTION('ref_axis',(8.91337114590872E-15,0.707106781186529,0.707106781186566)) ;
#97774=DIRECTION('center_axis',(0.,0.,-1.)) ;
#97775=DIRECTION('ref_axis',(-1.,0.,0.)) ;
#97776=DIRECTION('center_axis',(0.,0.,1.)) ;
#97777=DIRECTION('ref_axis',(-1.,1.0842021724855E-15,0.)) ;
#97778=DIRECTION('center_axis',(0.,0.,-1.)) ;
#97779=DIRECTION('ref_axis',(-1.,0.,0.)) ;
#97780=DIRECTION('center_axis',(-0.577350269189625,-0.577350269189626,0.577350269189627)) ;
#97781=DIRECTION('ref_axis',(5.35231302451417E-15,-0.707106781186551,-0.707106781186544)) ;
#97782=DIRECTION('center_axis',(0.577350269189625,0.577350269189626,-0.577350269189627)) ;
#97783=DIRECTION('ref_axis',(-6.40836823623517E-14,-0.707106781186516,-0.707106781186579)) ;
#97784=DIRECTION('center_axis',(0.577350269189625,0.577350269189625,-0.577350269189628)) ;
#97785=DIRECTION('ref_axis',(-0.707106781186552,5.19478420936363E-15,-0.707106781186543)) ;
#97786=DIRECTION('center_axis',(-0.577350269189625,-0.577350269189625,0.577350269189628)) ;
#97787=DIRECTION('ref_axis',(-0.707106781186562,2.56048320762387E-14,-0.707106781186533)) ;
#97788=DIRECTION('center_axis',(-0.577350269189542,-0.577350269189661,0.577350269189675)) ;
#97789=DIRECTION('ref_axis',(3.44881489367205E-15,-0.707106781186558,-0.707106781186537)) ;
#97790=DIRECTION('center_axis',(0.,0.,-1.)) ;
#97791=DIRECTION('ref_axis',(-1.,0.,0.)) ;
#97792=DIRECTION('center_axis',(0.,0.,1.)) ;
#97793=DIRECTION('ref_axis',(-1.,-8.67361737988404E-15,0.)) ;
#97794=DIRECTION('center_axis',(0.,0.,-1.)) ;
#97795=DIRECTION('ref_axis',(-1.,0.,0.)) ;
#97796=DIRECTION('center_axis',(2.08166817117218E-16,1.,0.)) ;
#97797=DIRECTION('ref_axis',(1.,0.,0.)) ;
#97798=DIRECTION('center_axis',(-1.,0.,9.05601424228639E-14)) ;
#97799=DIRECTION('ref_axis',(-9.05601424228639E-14,0.,-1.)) ;
#97800=DIRECTION('center_axis',(6.93889390390722E-14,6.93889390390721E-14,
1.)) ;
#97801=DIRECTION('ref_axis',(-1.,-6.3534872372487E-42,6.93889390390722E-14)) ;
#97802=DIRECTION('center_axis',(-0.577350269189625,-0.577350269189625,-0.577350269189628)) ;
#97803=DIRECTION('ref_axis',(-0.707106781186552,5.19478420936363E-15,0.707106781186543)) ;
#97804=DIRECTION('center_axis',(-0.577350269189625,-0.577350269189625,-0.577350269189628)) ;
#97805=DIRECTION('ref_axis',(-0.707106781186552,5.1349792556416E-15,0.707106781186543)) ;
#97806=DIRECTION('center_axis',(-0.577350269189609,-0.577350269189608,-0.57735026918966)) ;
#97807=DIRECTION('ref_axis',(-0.707106781186576,-5.08171669240118E-15,0.707106781186519)) ;
#97808=DIRECTION('center_axis',(0.,0.,-1.)) ;
#97809=DIRECTION('ref_axis',(-1.,0.,0.)) ;
#97810=DIRECTION('center_axis',(0.,0.,1.)) ;
#97811=DIRECTION('ref_axis',(1.,0.,0.)) ;
#97812=DIRECTION('center_axis',(-1.,0.,9.8563833862319E-18)) ;
#97813=DIRECTION('ref_axis',(9.8563833862319E-18,0.,1.)) ;
#97814=DIRECTION('center_axis',(-1.,1.31459513413869E-14,-1.31459513413873E-14)) ;
#97815=DIRECTION('ref_axis',(-1.31459513413873E-14,1.17484863248993E-41,
1.)) ;
#97816=DIRECTION('center_axis',(2.08166817117218E-16,1.,0.)) ;
#97817=DIRECTION('ref_axis',(1.,0.,0.)) ;
#97818=DIRECTION('center_axis',(-1.,-1.77538105744504E-14,-1.77538105744508E-14)) ;
#97819=DIRECTION('ref_axis',(1.77538105744506E-14,8.67361737988379E-15,
-1.)) ;
#97820=DIRECTION('center_axis',(2.08166817117218E-16,1.,0.)) ;
#97821=DIRECTION('ref_axis',(1.,0.,0.)) ;
#97822=DIRECTION('center_axis',(-0.577350269189595,0.577350269189594,-0.577350269189688)) ;
#97823=DIRECTION('ref_axis',(0.707106781186627,4.55186387217293E-14,-0.707106781186468)) ;
#97824=DIRECTION('center_axis',(-9.81307786677359E-14,0.,1.)) ;
#97825=DIRECTION('ref_axis',(-1.,0.,-9.81307786677359E-14)) ;
#97826=DIRECTION('center_axis',(-1.,0.,-9.8563833862319E-18)) ;
#97827=DIRECTION('ref_axis',(-9.8563833862319E-18,0.,1.)) ;
#97828=DIRECTION('center_axis',(-1.,0.,8.71102322353262E-14)) ;
#97829=DIRECTION('ref_axis',(8.71102322353262E-14,0.,1.)) ;
#97830=DIRECTION('center_axis',(0.,0.,-1.)) ;
#97831=DIRECTION('ref_axis',(-1.,0.,0.)) ;
#97832=DIRECTION('center_axis',(6.93889390390722E-14,-6.93889390390721E-14,
1.)) ;
#97833=DIRECTION('ref_axis',(1.,-6.3534872372487E-42,-6.93889390390722E-14)) ;
#97834=DIRECTION('center_axis',(0.577350269189625,-0.577350269189625,0.577350269189628)) ;
#97835=DIRECTION('ref_axis',(0.707106781186552,5.19478420936363E-15,-0.707106781186543)) ;
#97836=DIRECTION('center_axis',(0.577350269189625,-0.577350269189625,0.577350269189628)) ;
#97837=DIRECTION('ref_axis',(0.707106781186552,5.1349792556416E-15,-0.707106781186543)) ;
#97838=DIRECTION('center_axis',(2.08166817117218E-16,1.,0.)) ;
#97839=DIRECTION('ref_axis',(1.,0.,0.)) ;
#97840=DIRECTION('center_axis',(-0.577350269189538,0.577350269189662,0.577350269189676)) ;
#97841=DIRECTION('ref_axis',(1.74300544639431E-14,0.707106781186565,-0.70710678118653)) ;
#97842=DIRECTION('center_axis',(0.,0.,-1.)) ;
#97843=DIRECTION('ref_axis',(-1.,0.,0.)) ;
#97844=DIRECTION('center_axis',(0.,0.,1.)) ;
#97845=DIRECTION('ref_axis',(-1.,0.,0.)) ;
#97846=DIRECTION('center_axis',(0.,0.,-1.)) ;
#97847=DIRECTION('ref_axis',(-1.,0.,0.)) ;
#97848=DIRECTION('center_axis',(-0.577350269189625,0.577350269189625,0.577350269189628)) ;
#97849=DIRECTION('ref_axis',(0.707106781186552,5.1349792556416E-15,0.707106781186543)) ;
#97850=DIRECTION('center_axis',(0.577350269189625,-0.577350269189625,-0.577350269189628)) ;
#97851=DIRECTION('ref_axis',(0.707106781186562,2.5899563042358E-14,0.707106781186533)) ;
#97852=DIRECTION('center_axis',(-0.577350269189625,0.577350269189626,-0.577350269189626)) ;
#97853=DIRECTION('ref_axis',(5.20172641667636E-15,0.70710678118655,0.707106781186545)) ;
#97854=DIRECTION('center_axis',(0.577350269189625,-0.577350269189626,0.577350269189626)) ;
#97855=DIRECTION('ref_axis',(4.10196750502305E-14,0.707106781186568,0.707106781186527)) ;
#97856=DIRECTION('center_axis',(0.577350269189612,-0.57735026918964,0.577350269189626)) ;
#97857=DIRECTION('ref_axis',(-8.27428663398926E-15,-0.707106781186543,-0.707106781186552)) ;
#97858=DIRECTION('center_axis',(0.,0.,-1.)) ;
#97859=DIRECTION('ref_axis',(-1.,0.,0.)) ;
#97860=DIRECTION('center_axis',(0.,0.,1.)) ;
#97861=DIRECTION('ref_axis',(-1.,1.35525271560688E-14,0.)) ;
#97862=DIRECTION('center_axis',(0.,0.,-1.)) ;
#97863=DIRECTION('ref_axis',(-1.,0.,0.)) ;
#97864=DIRECTION('center_axis',(0.,1.,0.)) ;
#97865=DIRECTION('ref_axis',(1.,0.,0.)) ;
#97866=DIRECTION('center_axis',(0.,-1.,1.13080389480401E-14)) ;
#97867=DIRECTION('ref_axis',(1.12757025938489E-13,1.13080389480401E-14,
1.)) ;
#97868=DIRECTION('center_axis',(0.,0.,1.)) ;
#97869=DIRECTION('ref_axis',(-1.,0.,0.)) ;
#97870=DIRECTION('center_axis',(0.577350269189625,-0.577350269189626,-0.577350269189626)) ;
#97871=DIRECTION('ref_axis',(5.20172641667636E-15,0.70710678118655,-0.707106781186545)) ;
#97872=DIRECTION('center_axis',(0.577350269189625,-0.577350269189626,-0.577350269189626)) ;
#97873=DIRECTION('ref_axis',(5.11416588733871E-15,0.70710678118655,-0.707106781186545)) ;
#97874=DIRECTION('center_axis',(0.577350269189618,-0.577350269189619,-0.57735026918964)) ;
#97875=DIRECTION('ref_axis',(1.15945863464918E-15,0.707106781186561,-0.707106781186534)) ;
#97876=DIRECTION('center_axis',(0.,0.,-1.)) ;
#97877=DIRECTION('ref_axis',(-1.,0.,0.)) ;
#97878=DIRECTION('center_axis',(0.,0.,1.)) ;
#97879=DIRECTION('ref_axis',(1.,0.,0.)) ;
#97880=DIRECTION('center_axis',(0.,1.,1.95511867169518E-16)) ;
#97881=DIRECTION('ref_axis',(0.,-1.95511867169518E-16,1.)) ;
#97882=DIRECTION('center_axis',(4.26226979058352E-14,-1.,4.24310362287508E-14)) ;
#97883=DIRECTION('ref_axis',(1.,4.26226979058352E-14,4.69939452995971E-41)) ;
#97884=DIRECTION('center_axis',(0.,1.,0.)) ;
#97885=DIRECTION('ref_axis',(1.,0.,0.)) ;
#97886=DIRECTION('center_axis',(-1.00288700954911E-14,-1.,1.02205317725767E-14)) ;
#97887=DIRECTION('ref_axis',(3.46944695195352E-14,1.02205317725764E-14,
1.)) ;
#97888=DIRECTION('center_axis',(0.,1.,0.)) ;
#97889=DIRECTION('ref_axis',(1.,0.,0.)) ;
#97890=DIRECTION('center_axis',(-0.577350269189659,-0.57735026918966,-0.577350269189558)) ;
#97891=DIRECTION('ref_axis',(-0.707106781186543,0.707106781186552,-1.03102727271032E-14)) ;
#97892=DIRECTION('center_axis',(0.,9.8130778667736E-14,1.)) ;
#97893=DIRECTION('ref_axis',(-8.67361737988403E-15,1.,-9.8130778667736E-14)) ;
#97894=DIRECTION('center_axis',(0.,1.,-1.95511867169518E-16)) ;
#97895=DIRECTION('ref_axis',(0.,1.95511867169518E-16,1.)) ;
#97896=DIRECTION('center_axis',(0.,-1.,9.83224403448236E-14)) ;
#97897=DIRECTION('ref_axis',(0.,-9.83224403448236E-14,-1.)) ;
#97898=DIRECTION('center_axis',(0.,0.,-1.)) ;
#97899=DIRECTION('ref_axis',(-1.,0.,0.)) ;
#97900=DIRECTION('center_axis',(0.,0.,1.)) ;
#97901=DIRECTION('ref_axis',(1.,0.,0.)) ;
#97902=DIRECTION('center_axis',(0.577350269189625,0.577350269189626,0.577350269189627)) ;
#97903=DIRECTION('ref_axis',(5.35231302451417E-15,-0.707106781186551,0.707106781186544)) ;
#97904=DIRECTION('center_axis',(0.577350269189625,0.577350269189626,0.577350269189627)) ;
#97905=DIRECTION('ref_axis',(5.35231302451417E-15,-0.707106781186551,0.707106781186544)) ;
#97906=DIRECTION('center_axis',(0.,1.,0.)) ;
#97907=DIRECTION('ref_axis',(1.,0.,0.)) ;
#97908=DIRECTION('center_axis',(-0.57735026918964,-0.577350269189583,0.577350269189654)) ;
#97909=DIRECTION('ref_axis',(-0.707106781186567,2.1970613508967E-14,-0.707106781186528)) ;
#97910=DIRECTION('center_axis',(0.,0.,-1.)) ;
#97911=DIRECTION('ref_axis',(-1.,0.,0.)) ;
#97912=DIRECTION('center_axis',(0.,0.,1.)) ;
#97913=DIRECTION('ref_axis',(-1.,1.0842021724855E-15,0.)) ;
#97914=DIRECTION('center_axis',(0.,0.,-1.)) ;
#97915=DIRECTION('ref_axis',(-1.,0.,0.)) ;
#97916=DIRECTION('center_axis',(-0.577350269189625,-0.577350269189626,0.577350269189627)) ;
#97917=DIRECTION('ref_axis',(5.35231302451417E-15,-0.707106781186551,-0.707106781186544)) ;
#97918=DIRECTION('center_axis',(0.577350269189625,0.577350269189626,-0.577350269189627)) ;
#97919=DIRECTION('ref_axis',(4.8009187113684E-14,-0.707106781186572,-0.707106781186523)) ;
#97920=DIRECTION('center_axis',(0.,0.,1.)) ;
#97921=DIRECTION('ref_axis',(1.,0.,0.)) ;
#97922=DIRECTION('center_axis',(0.,-1.,0.)) ;
#97923=DIRECTION('ref_axis',(0.,0.,-1.)) ;
#97924=DIRECTION('center_axis',(9.85638338623186E-18,1.,0.)) ;
#97925=DIRECTION('ref_axis',(-1.,9.85638338623186E-18,0.)) ;
#97926=DIRECTION('center_axis',(0.,-1.,0.)) ;
#97927=DIRECTION('ref_axis',(0.,0.,-1.)) ;
#97928=DIRECTION('center_axis',(0.,1.,0.)) ;
#97929=DIRECTION('ref_axis',(1.,0.,0.)) ;
#97930=DIRECTION('center_axis',(-1.,-7.66646708341686E-16,0.)) ;
#97931=DIRECTION('ref_axis',(7.66646708341686E-16,-1.,0.)) ;
#97932=DIRECTION('center_axis',(1.,-9.85638338623186E-18,0.)) ;
#97933=DIRECTION('ref_axis',(9.85638338623186E-18,1.,0.)) ;
#97934=DIRECTION('center_axis',(-1.,0.,0.)) ;
#97935=DIRECTION('ref_axis',(0.,0.,1.)) ;
#97936=DIRECTION('center_axis',(0.,1.,0.)) ;
#97937=DIRECTION('ref_axis',(1.,0.,0.)) ;
#97938=DIRECTION('center_axis',(0.,1.,0.)) ;
#97939=DIRECTION('ref_axis',(0.,0.,1.)) ;
#97940=DIRECTION('center_axis',(-9.85638338623186E-18,-1.,0.)) ;
#97941=DIRECTION('ref_axis',(1.,-9.85638338623186E-18,0.)) ;
#97942=DIRECTION('center_axis',(0.,1.,0.)) ;
#97943=DIRECTION('ref_axis',(0.,0.,1.)) ;
#97944=DIRECTION('center_axis',(0.,0.,1.)) ;
#97945=DIRECTION('ref_axis',(1.,0.,0.)) ;
#97946=DIRECTION('center_axis',(0.,0.,1.)) ;
#97947=DIRECTION('ref_axis',(1.,0.,0.)) ;
#97948=DIRECTION('center_axis',(0.,-1.,0.)) ;
#97949=DIRECTION('ref_axis',(0.,0.,-1.)) ;
#97950=DIRECTION('center_axis',(-9.85638338623186E-18,-1.,0.)) ;
#97951=DIRECTION('ref_axis',(1.,-9.85638338623186E-18,0.)) ;
#97952=DIRECTION('center_axis',(0.,-1.,0.)) ;
#97953=DIRECTION('ref_axis',(0.,0.,-1.)) ;
#97954=DIRECTION('center_axis',(0.,1.,0.)) ;
#97955=DIRECTION('ref_axis',(1.,0.,0.)) ;
#97956=DIRECTION('center_axis',(1.,-3.06658683336674E-15,0.)) ;
#97957=DIRECTION('ref_axis',(3.06658683336674E-15,1.,0.)) ;
#97958=DIRECTION('center_axis',(1.,-9.85638338623186E-18,0.)) ;
#97959=DIRECTION('ref_axis',(9.85638338623186E-18,1.,0.)) ;
#97960=DIRECTION('center_axis',(1.,0.,0.)) ;
#97961=DIRECTION('ref_axis',(0.,0.,-1.)) ;
#97962=DIRECTION('center_axis',(0.,1.,0.)) ;
#97963=DIRECTION('ref_axis',(1.,0.,0.)) ;
#97964=DIRECTION('center_axis',(0.,1.,0.)) ;
#97965=DIRECTION('ref_axis',(0.,0.,1.)) ;
#97966=DIRECTION('center_axis',(-9.85638338623186E-18,-1.,0.)) ;
#97967=DIRECTION('ref_axis',(1.,-9.85638338623186E-18,0.)) ;
#97968=DIRECTION('center_axis',(0.,1.,0.)) ;
#97969=DIRECTION('ref_axis',(0.,0.,1.)) ;
#97970=DIRECTION('center_axis',(0.,0.,1.)) ;
#97971=DIRECTION('ref_axis',(1.,0.,0.)) ;
#97972=DIRECTION('center_axis',(-1.,-1.95511867169517E-16,0.)) ;
#97973=DIRECTION('ref_axis',(1.95511867169517E-16,-1.,0.)) ;
#97974=DIRECTION('center_axis',(1.,0.,0.)) ;
#97975=DIRECTION('ref_axis',(0.,0.,-1.)) ;
#97976=DIRECTION('center_axis',(0.,1.,0.)) ;
#97977=DIRECTION('ref_axis',(1.,0.,0.)) ;
#97978=DIRECTION('center_axis',(7.66646708341686E-16,-1.,0.)) ;
#97979=DIRECTION('ref_axis',(1.,7.66646708341686E-16,0.)) ;
#97980=DIRECTION('center_axis',(-1.95511867169517E-16,1.,0.)) ;
#97981=DIRECTION('ref_axis',(-1.,-1.95511867169517E-16,0.)) ;
#97982=DIRECTION('center_axis',(0.,-1.,0.)) ;
#97983=DIRECTION('ref_axis',(0.,0.,-1.)) ;
#97984=DIRECTION('center_axis',(0.,1.,0.)) ;
#97985=DIRECTION('ref_axis',(1.,0.,0.)) ;
#97986=DIRECTION('center_axis',(-1.,0.,0.)) ;
#97987=DIRECTION('ref_axis',(0.,0.,1.)) ;
#97988=DIRECTION('center_axis',(1.,-1.06642836637918E-16,0.)) ;
#97989=DIRECTION('ref_axis',(1.06642836637918E-16,1.,0.)) ;
#97990=DIRECTION('center_axis',(1.,1.95511867169517E-16,0.)) ;
#97991=DIRECTION('ref_axis',(-1.95511867169517E-16,1.,0.)) ;
#97992=DIRECTION('center_axis',(1.,0.,0.)) ;
#97993=DIRECTION('ref_axis',(0.,0.,-1.)) ;
#97994=DIRECTION('center_axis',(0.,1.,0.)) ;
#97995=DIRECTION('ref_axis',(1.,0.,0.)) ;
#97996=DIRECTION('center_axis',(2.29994012502506E-15,-1.,0.)) ;
#97997=DIRECTION('ref_axis',(1.,2.29994012502506E-15,0.)) ;
#97998=DIRECTION('center_axis',(-1.95511867169517E-16,1.,0.)) ;
#97999=DIRECTION('ref_axis',(-1.,-1.95511867169517E-16,0.)) ;
#98000=DIRECTION('center_axis',(0.,-1.,0.)) ;
#98001=DIRECTION('ref_axis',(0.,0.,-1.)) ;
#98002=DIRECTION('center_axis',(-1.,1.06642836637918E-16,0.)) ;
#98003=DIRECTION('ref_axis',(-1.06642836637918E-16,-1.,0.)) ;
#98004=DIRECTION('center_axis',(1.,0.,0.)) ;
#98005=DIRECTION('ref_axis',(0.,0.,-1.)) ;
#98006=DIRECTION('center_axis',(0.,1.,0.)) ;
#98007=DIRECTION('ref_axis',(1.,0.,0.)) ;
#98008=DIRECTION('center_axis',(0.,0.,1.)) ;
#98009=DIRECTION('ref_axis',(1.,0.,0.)) ;
#98010=DIRECTION('center_axis',(0.,-1.,0.)) ;
#98011=DIRECTION('ref_axis',(0.,0.,-1.)) ;
#98012=DIRECTION('center_axis',(9.85638338623186E-18,1.,0.)) ;
#98013=DIRECTION('ref_axis',(-1.,9.85638338623186E-18,0.)) ;
#98014=DIRECTION('center_axis',(0.,-1.,0.)) ;
#98015=DIRECTION('ref_axis',(0.,0.,-1.)) ;
#98016=DIRECTION('center_axis',(0.,1.,0.)) ;
#98017=DIRECTION('ref_axis',(1.,0.,0.)) ;
#98018=DIRECTION('center_axis',(-1.,-1.14997006251252E-14,0.)) ;
#98019=DIRECTION('ref_axis',(1.14997006251252E-14,-1.,0.)) ;
#98020=DIRECTION('center_axis',(1.,-9.85638338623186E-18,0.)) ;
#98021=DIRECTION('ref_axis',(9.85638338623186E-18,1.,0.)) ;
#98022=DIRECTION('center_axis',(-1.,0.,0.)) ;
#98023=DIRECTION('ref_axis',(0.,0.,1.)) ;
#98024=DIRECTION('center_axis',(0.,1.,0.)) ;
#98025=DIRECTION('ref_axis',(1.,0.,0.)) ;
#98026=DIRECTION('center_axis',(0.,1.,0.)) ;
#98027=DIRECTION('ref_axis',(0.,0.,1.)) ;
#98028=DIRECTION('center_axis',(-9.85638338623186E-18,-1.,0.)) ;
#98029=DIRECTION('ref_axis',(1.,-9.85638338623186E-18,0.)) ;
#98030=DIRECTION('center_axis',(0.,1.,0.)) ;
#98031=DIRECTION('ref_axis',(0.,0.,1.)) ;
#98032=DIRECTION('center_axis',(0.,0.,1.)) ;
#98033=DIRECTION('ref_axis',(1.,0.,0.)) ;
#98034=DIRECTION('center_axis',(0.,0.,1.)) ;
#98035=DIRECTION('ref_axis',(1.,0.,0.)) ;
#98036=DIRECTION('center_axis',(0.,-1.,0.)) ;
#98037=DIRECTION('ref_axis',(0.,0.,-1.)) ;
#98038=DIRECTION('center_axis',(-9.85638338623186E-18,-1.,0.)) ;
#98039=DIRECTION('ref_axis',(1.,-9.85638338623186E-18,0.)) ;
#98040=DIRECTION('center_axis',(0.,-1.,0.)) ;
#98041=DIRECTION('ref_axis',(0.,0.,-1.)) ;
#98042=DIRECTION('center_axis',(0.,1.,0.)) ;
#98043=DIRECTION('ref_axis',(1.,0.,0.)) ;
#98044=DIRECTION('center_axis',(1.,3.83323354170843E-15,0.)) ;
#98045=DIRECTION('ref_axis',(-3.83323354170843E-15,1.,0.)) ;
#98046=DIRECTION('center_axis',(1.,-9.85638338623186E-18,0.)) ;
#98047=DIRECTION('ref_axis',(9.85638338623186E-18,1.,0.)) ;
#98048=DIRECTION('center_axis',(1.,0.,0.)) ;
#98049=DIRECTION('ref_axis',(0.,0.,-1.)) ;
#98050=DIRECTION('center_axis',(0.,1.,0.)) ;
#98051=DIRECTION('ref_axis',(1.,0.,0.)) ;
#98052=DIRECTION('center_axis',(0.,1.,0.)) ;
#98053=DIRECTION('ref_axis',(0.,0.,1.)) ;
#98054=DIRECTION('center_axis',(-9.85638338623186E-18,-1.,0.)) ;
#98055=DIRECTION('ref_axis',(1.,-9.85638338623186E-18,0.)) ;
#98056=DIRECTION('center_axis',(0.,1.,0.)) ;
#98057=DIRECTION('ref_axis',(0.,0.,1.)) ;
#98058=DIRECTION('center_axis',(0.,0.,1.)) ;
#98059=DIRECTION('ref_axis',(1.,0.,0.)) ;
#98060=DIRECTION('center_axis',(-1.,-1.95511867169517E-16,0.)) ;
#98061=DIRECTION('ref_axis',(1.95511867169517E-16,-1.,0.)) ;
#98062=DIRECTION('center_axis',(1.,0.,0.)) ;
#98063=DIRECTION('ref_axis',(0.,0.,-1.)) ;
#98064=DIRECTION('center_axis',(0.,1.,0.)) ;
#98065=DIRECTION('ref_axis',(1.,0.,0.)) ;
#98066=DIRECTION('center_axis',(4.59988025005012E-15,-1.,0.)) ;
#98067=DIRECTION('ref_axis',(1.,4.59988025005012E-15,0.)) ;
#98068=DIRECTION('center_axis',(-1.95511867169517E-16,1.,0.)) ;
#98069=DIRECTION('ref_axis',(-1.,-1.95511867169517E-16,0.)) ;
#98070=DIRECTION('center_axis',(0.,-1.,0.)) ;
#98071=DIRECTION('ref_axis',(0.,0.,-1.)) ;
#98072=DIRECTION('center_axis',(0.,1.,0.)) ;
#98073=DIRECTION('ref_axis',(1.,0.,0.)) ;
#98074=DIRECTION('center_axis',(-1.,0.,0.)) ;
#98075=DIRECTION('ref_axis',(0.,0.,1.)) ;
#98076=DIRECTION('center_axis',(1.,-1.06642836637918E-16,0.)) ;
#98077=DIRECTION('ref_axis',(1.06642836637918E-16,1.,0.)) ;
#98078=DIRECTION('center_axis',(1.,1.95511867169517E-16,0.)) ;
#98079=DIRECTION('ref_axis',(-1.95511867169517E-16,1.,0.)) ;
#98080=DIRECTION('center_axis',(1.,0.,0.)) ;
#98081=DIRECTION('ref_axis',(0.,0.,-1.)) ;
#98082=DIRECTION('center_axis',(0.,1.,0.)) ;
#98083=DIRECTION('ref_axis',(1.,0.,0.)) ;
#98084=DIRECTION('center_axis',(-1.53329341668337E-15,-1.,0.)) ;
#98085=DIRECTION('ref_axis',(1.,-1.53329341668337E-15,0.)) ;
#98086=DIRECTION('center_axis',(-1.95511867169517E-16,1.,0.)) ;
#98087=DIRECTION('ref_axis',(-1.,-1.95511867169517E-16,0.)) ;
#98088=DIRECTION('center_axis',(0.,-1.,0.)) ;
#98089=DIRECTION('ref_axis',(0.,0.,-1.)) ;
#98090=DIRECTION('center_axis',(-1.,1.06642836637918E-16,0.)) ;
#98091=DIRECTION('ref_axis',(-1.06642836637918E-16,-1.,0.)) ;
#98092=DIRECTION('center_axis',(1.,0.,0.)) ;
#98093=DIRECTION('ref_axis',(0.,0.,-1.)) ;
#98094=DIRECTION('center_axis',(0.,1.,0.)) ;
#98095=DIRECTION('ref_axis',(1.,0.,0.)) ;
#98096=DIRECTION('center_axis',(0.,0.,1.)) ;
#98097=DIRECTION('ref_axis',(1.,0.,0.)) ;
#98098=DIRECTION('center_axis',(0.,-1.,0.)) ;
#98099=DIRECTION('ref_axis',(0.,0.,-1.)) ;
#98100=DIRECTION('center_axis',(9.85638338623186E-18,1.,0.)) ;
#98101=DIRECTION('ref_axis',(-1.,9.85638338623186E-18,0.)) ;
#98102=DIRECTION('center_axis',(0.,-1.,0.)) ;
#98103=DIRECTION('ref_axis',(0.,0.,-1.)) ;
#98104=DIRECTION('center_axis',(0.,1.,0.)) ;
#98105=DIRECTION('ref_axis',(1.,0.,0.)) ;
#98106=DIRECTION('center_axis',(-1.,-2.29994012502506E-15,0.)) ;
#98107=DIRECTION('ref_axis',(2.29994012502506E-15,-1.,0.)) ;
#98108=DIRECTION('center_axis',(1.,-9.85638338623186E-18,0.)) ;
#98109=DIRECTION('ref_axis',(9.85638338623186E-18,1.,0.)) ;
#98110=DIRECTION('center_axis',(-1.,0.,0.)) ;
#98111=DIRECTION('ref_axis',(0.,0.,1.)) ;
#98112=DIRECTION('center_axis',(0.,1.,0.)) ;
#98113=DIRECTION('ref_axis',(1.,0.,0.)) ;
#98114=DIRECTION('center_axis',(0.,1.,0.)) ;
#98115=DIRECTION('ref_axis',(0.,0.,1.)) ;
#98116=DIRECTION('center_axis',(-9.85638338623186E-18,-1.,0.)) ;
#98117=DIRECTION('ref_axis',(1.,-9.85638338623186E-18,0.)) ;
#98118=DIRECTION('center_axis',(0.,1.,0.)) ;
#98119=DIRECTION('ref_axis',(0.,0.,1.)) ;
#98120=DIRECTION('center_axis',(0.,0.,1.)) ;
#98121=DIRECTION('ref_axis',(1.,0.,0.)) ;
#98122=DIRECTION('center_axis',(0.,0.,1.)) ;
#98123=DIRECTION('ref_axis',(1.,0.,0.)) ;
#98124=DIRECTION('center_axis',(0.,-1.,0.)) ;
#98125=DIRECTION('ref_axis',(0.,0.,-1.)) ;
#98126=DIRECTION('center_axis',(-9.85638338623186E-18,-1.,0.)) ;
#98127=DIRECTION('ref_axis',(1.,-9.85638338623186E-18,0.)) ;
#98128=DIRECTION('center_axis',(0.,-1.,0.)) ;
#98129=DIRECTION('ref_axis',(0.,0.,-1.)) ;
#98130=DIRECTION('center_axis',(0.,1.,0.)) ;
#98131=DIRECTION('ref_axis',(1.,0.,0.)) ;
#98132=DIRECTION('center_axis',(1.,-7.66646708341686E-15,0.)) ;
#98133=DIRECTION('ref_axis',(7.66646708341686E-15,1.,0.)) ;
#98134=DIRECTION('center_axis',(1.,-9.85638338623186E-18,0.)) ;
#98135=DIRECTION('ref_axis',(9.85638338623186E-18,1.,0.)) ;
#98136=DIRECTION('center_axis',(1.,0.,0.)) ;
#98137=DIRECTION('ref_axis',(0.,0.,-1.)) ;
#98138=DIRECTION('center_axis',(0.,1.,0.)) ;
#98139=DIRECTION('ref_axis',(1.,0.,0.)) ;
#98140=DIRECTION('center_axis',(0.,1.,0.)) ;
#98141=DIRECTION('ref_axis',(0.,0.,1.)) ;
#98142=DIRECTION('center_axis',(-9.85638338623186E-18,-1.,0.)) ;
#98143=DIRECTION('ref_axis',(1.,-9.85638338623186E-18,0.)) ;
#98144=DIRECTION('center_axis',(0.,1.,0.)) ;
#98145=DIRECTION('ref_axis',(0.,0.,1.)) ;
#98146=DIRECTION('center_axis',(0.,0.,1.)) ;
#98147=DIRECTION('ref_axis',(1.,0.,0.)) ;
#98148=DIRECTION('center_axis',(-1.,-1.95511867169517E-16,0.)) ;
#98149=DIRECTION('ref_axis',(1.95511867169517E-16,-1.,0.)) ;
#98150=DIRECTION('center_axis',(1.,0.,0.)) ;
#98151=DIRECTION('ref_axis',(0.,0.,-1.)) ;
#98152=DIRECTION('center_axis',(0.,1.,0.)) ;
#98153=DIRECTION('ref_axis',(1.,0.,0.)) ;
#98154=DIRECTION('center_axis',(9.9664072084418E-15,-1.,0.)) ;
#98155=DIRECTION('ref_axis',(1.,9.9664072084418E-15,0.)) ;
#98156=DIRECTION('center_axis',(-1.95511867169517E-16,1.,0.)) ;
#98157=DIRECTION('ref_axis',(-1.,-1.95511867169517E-16,0.)) ;
#98158=DIRECTION('center_axis',(0.,-1.,0.)) ;
#98159=DIRECTION('ref_axis',(0.,0.,-1.)) ;
#98160=DIRECTION('center_axis',(0.,1.,0.)) ;
#98161=DIRECTION('ref_axis',(1.,0.,0.)) ;
#98162=DIRECTION('center_axis',(-1.,0.,0.)) ;
#98163=DIRECTION('ref_axis',(0.,0.,1.)) ;
#98164=DIRECTION('center_axis',(1.,-1.06642836637918E-16,0.)) ;
#98165=DIRECTION('ref_axis',(1.06642836637918E-16,1.,0.)) ;
#98166=DIRECTION('center_axis',(1.,1.95511867169517E-16,0.)) ;
#98167=DIRECTION('ref_axis',(-1.95511867169517E-16,1.,0.)) ;
#98168=DIRECTION('center_axis',(1.,0.,0.)) ;
#98169=DIRECTION('ref_axis',(0.,0.,-1.)) ;
#98170=DIRECTION('center_axis',(0.,1.,0.)) ;
#98171=DIRECTION('ref_axis',(1.,0.,0.)) ;
#98172=DIRECTION('center_axis',(6.89982037507517E-15,-1.,0.)) ;
#98173=DIRECTION('ref_axis',(1.,6.89982037507517E-15,0.)) ;
#98174=DIRECTION('center_axis',(-1.95511867169517E-16,1.,0.)) ;
#98175=DIRECTION('ref_axis',(-1.,-1.95511867169517E-16,0.)) ;
#98176=DIRECTION('center_axis',(0.,-1.,0.)) ;
#98177=DIRECTION('ref_axis',(0.,0.,-1.)) ;
#98178=DIRECTION('center_axis',(-1.,1.06642836637918E-16,0.)) ;
#98179=DIRECTION('ref_axis',(-1.06642836637918E-16,-1.,0.)) ;
#98180=DIRECTION('center_axis',(1.,0.,0.)) ;
#98181=DIRECTION('ref_axis',(0.,0.,-1.)) ;
#98182=DIRECTION('center_axis',(0.,1.,0.)) ;
#98183=DIRECTION('ref_axis',(1.,0.,0.)) ;
#98184=DIRECTION('center_axis',(0.,0.,1.)) ;
#98185=DIRECTION('ref_axis',(1.,0.,0.)) ;
#98186=DIRECTION('center_axis',(0.,-1.,0.)) ;
#98187=DIRECTION('ref_axis',(0.,0.,-1.)) ;
#98188=DIRECTION('center_axis',(9.85638338623186E-18,1.,0.)) ;
#98189=DIRECTION('ref_axis',(-1.,9.85638338623186E-18,0.)) ;
#98190=DIRECTION('center_axis',(0.,-1.,0.)) ;
#98191=DIRECTION('ref_axis',(0.,0.,-1.)) ;
#98192=DIRECTION('center_axis',(0.,1.,0.)) ;
#98193=DIRECTION('ref_axis',(1.,0.,0.)) ;
#98194=DIRECTION('center_axis',(-1.,0.,0.)) ;
#98195=DIRECTION('ref_axis',(0.,0.,1.)) ;
#98196=DIRECTION('center_axis',(1.,-9.85638338623186E-18,0.)) ;
#98197=DIRECTION('ref_axis',(9.85638338623186E-18,1.,0.)) ;
#98198=DIRECTION('center_axis',(-1.,0.,0.)) ;
#98199=DIRECTION('ref_axis',(0.,0.,1.)) ;
#98200=DIRECTION('center_axis',(0.,1.,0.)) ;
#98201=DIRECTION('ref_axis',(1.,0.,0.)) ;
#98202=DIRECTION('center_axis',(0.,1.,0.)) ;
#98203=DIRECTION('ref_axis',(0.,0.,1.)) ;
#98204=DIRECTION('center_axis',(-9.85638338623186E-18,-1.,0.)) ;
#98205=DIRECTION('ref_axis',(1.,-9.85638338623186E-18,0.)) ;
#98206=DIRECTION('center_axis',(0.,1.,0.)) ;
#98207=DIRECTION('ref_axis',(0.,0.,1.)) ;
#98208=DIRECTION('center_axis',(0.,0.,1.)) ;
#98209=DIRECTION('ref_axis',(1.,0.,0.)) ;
#98210=DIRECTION('center_axis',(0.,0.,1.)) ;
#98211=DIRECTION('ref_axis',(1.,0.,0.)) ;
#98212=DIRECTION('center_axis',(0.,-1.,0.)) ;
#98213=DIRECTION('ref_axis',(0.,0.,-1.)) ;
#98214=DIRECTION('center_axis',(-9.85638338623186E-18,-1.,0.)) ;
#98215=DIRECTION('ref_axis',(1.,-9.85638338623186E-18,0.)) ;
#98216=DIRECTION('center_axis',(0.,-1.,0.)) ;
#98217=DIRECTION('ref_axis',(0.,0.,-1.)) ;
#98218=DIRECTION('center_axis',(0.,1.,0.)) ;
#98219=DIRECTION('ref_axis',(1.,0.,0.)) ;
#98220=DIRECTION('center_axis',(1.,-9.19976050010023E-15,0.)) ;
#98221=DIRECTION('ref_axis',(9.19976050010023E-15,1.,0.)) ;
#98222=DIRECTION('center_axis',(1.,-9.85638338623186E-18,0.)) ;
#98223=DIRECTION('ref_axis',(9.85638338623186E-18,1.,0.)) ;
#98224=DIRECTION('center_axis',(1.,0.,0.)) ;
#98225=DIRECTION('ref_axis',(0.,0.,-1.)) ;
#98226=DIRECTION('center_axis',(0.,1.,0.)) ;
#98227=DIRECTION('ref_axis',(1.,0.,0.)) ;
#98228=DIRECTION('center_axis',(0.,1.,0.)) ;
#98229=DIRECTION('ref_axis',(0.,0.,1.)) ;
#98230=DIRECTION('center_axis',(-9.85638338623186E-18,-1.,0.)) ;
#98231=DIRECTION('ref_axis',(1.,-9.85638338623186E-18,0.)) ;
#98232=DIRECTION('center_axis',(0.,1.,0.)) ;
#98233=DIRECTION('ref_axis',(0.,0.,1.)) ;
#98234=DIRECTION('center_axis',(0.,0.,1.)) ;
#98235=DIRECTION('ref_axis',(1.,0.,0.)) ;
#98236=DIRECTION('center_axis',(-1.,-1.95511867169517E-16,0.)) ;
#98237=DIRECTION('ref_axis',(1.95511867169517E-16,-1.,0.)) ;
#98238=DIRECTION('center_axis',(1.,0.,0.)) ;
#98239=DIRECTION('ref_axis',(0.,0.,-1.)) ;
#98240=DIRECTION('center_axis',(0.,1.,0.)) ;
#98241=DIRECTION('ref_axis',(1.,0.,0.)) ;
#98242=DIRECTION('center_axis',(-1.53329341668337E-15,-1.,0.)) ;
#98243=DIRECTION('ref_axis',(1.,-1.53329341668337E-15,0.)) ;
#98244=DIRECTION('center_axis',(-1.95511867169517E-16,1.,0.)) ;
#98245=DIRECTION('ref_axis',(-1.,-1.95511867169517E-16,0.)) ;
#98246=DIRECTION('center_axis',(0.,-1.,0.)) ;
#98247=DIRECTION('ref_axis',(0.,0.,-1.)) ;
#98248=DIRECTION('center_axis',(0.,1.,0.)) ;
#98249=DIRECTION('ref_axis',(1.,0.,0.)) ;
#98250=DIRECTION('center_axis',(-1.,0.,0.)) ;
#98251=DIRECTION('ref_axis',(0.,0.,1.)) ;
#98252=DIRECTION('center_axis',(1.,-1.06642836637918E-16,0.)) ;
#98253=DIRECTION('ref_axis',(1.06642836637918E-16,1.,0.)) ;
#98254=DIRECTION('center_axis',(1.,1.95511867169517E-16,0.)) ;
#98255=DIRECTION('ref_axis',(-1.95511867169517E-16,1.,0.)) ;
#98256=DIRECTION('center_axis',(1.,0.,0.)) ;
#98257=DIRECTION('ref_axis',(0.,0.,-1.)) ;
#98258=DIRECTION('center_axis',(0.,1.,0.)) ;
#98259=DIRECTION('ref_axis',(1.,0.,0.)) ;
#98260=DIRECTION('center_axis',(-3.06658683336674E-15,-1.,0.)) ;
#98261=DIRECTION('ref_axis',(1.,-3.06658683336674E-15,0.)) ;
#98262=DIRECTION('center_axis',(-1.95511867169517E-16,1.,0.)) ;
#98263=DIRECTION('ref_axis',(-1.,-1.95511867169517E-16,0.)) ;
#98264=DIRECTION('center_axis',(0.,-1.,0.)) ;
#98265=DIRECTION('ref_axis',(0.,0.,-1.)) ;
#98266=DIRECTION('center_axis',(-1.,1.06642836637918E-16,0.)) ;
#98267=DIRECTION('ref_axis',(-1.06642836637918E-16,-1.,0.)) ;
#98268=DIRECTION('center_axis',(1.,0.,0.)) ;
#98269=DIRECTION('ref_axis',(0.,0.,-1.)) ;
#98270=DIRECTION('center_axis',(0.,1.,0.)) ;
#98271=DIRECTION('ref_axis',(1.,0.,0.)) ;
#98272=DIRECTION('center_axis',(0.,0.,1.)) ;
#98273=DIRECTION('ref_axis',(1.,0.,0.)) ;
#98274=DIRECTION('center_axis',(0.,-1.,0.)) ;
#98275=DIRECTION('ref_axis',(0.,0.,-1.)) ;
#98276=DIRECTION('center_axis',(9.85638338623186E-18,1.,0.)) ;
#98277=DIRECTION('ref_axis',(-1.,9.85638338623186E-18,0.)) ;
#98278=DIRECTION('center_axis',(0.,-1.,0.)) ;
#98279=DIRECTION('ref_axis',(0.,0.,-1.)) ;
#98280=DIRECTION('center_axis',(0.,1.,0.)) ;
#98281=DIRECTION('ref_axis',(1.,0.,0.)) ;
#98282=DIRECTION('center_axis',(-1.,4.59988025005012E-15,0.)) ;
#98283=DIRECTION('ref_axis',(-4.59988025005012E-15,-1.,0.)) ;
#98284=DIRECTION('center_axis',(1.,-9.85638338623186E-18,0.)) ;
#98285=DIRECTION('ref_axis',(9.85638338623186E-18,1.,0.)) ;
#98286=DIRECTION('center_axis',(-1.,0.,0.)) ;
#98287=DIRECTION('ref_axis',(0.,0.,1.)) ;
#98288=DIRECTION('center_axis',(0.,1.,0.)) ;
#98289=DIRECTION('ref_axis',(1.,0.,0.)) ;
#98290=DIRECTION('center_axis',(0.,1.,0.)) ;
#98291=DIRECTION('ref_axis',(0.,0.,1.)) ;
#98292=DIRECTION('center_axis',(-9.85638338623186E-18,-1.,0.)) ;
#98293=DIRECTION('ref_axis',(1.,-9.85638338623186E-18,0.)) ;
#98294=DIRECTION('center_axis',(0.,1.,0.)) ;
#98295=DIRECTION('ref_axis',(0.,0.,1.)) ;
#98296=DIRECTION('center_axis',(0.,0.,1.)) ;
#98297=DIRECTION('ref_axis',(1.,0.,0.)) ;
#98298=DIRECTION('center_axis',(0.,0.,1.)) ;
#98299=DIRECTION('ref_axis',(1.,0.,0.)) ;
#98300=DIRECTION('center_axis',(0.,-1.,0.)) ;
#98301=DIRECTION('ref_axis',(0.,0.,-1.)) ;
#98302=DIRECTION('center_axis',(-9.85638338623186E-18,-1.,0.)) ;
#98303=DIRECTION('ref_axis',(1.,-9.85638338623186E-18,0.)) ;
#98304=DIRECTION('center_axis',(0.,-1.,0.)) ;
#98305=DIRECTION('ref_axis',(0.,0.,-1.)) ;
#98306=DIRECTION('center_axis',(0.,1.,0.)) ;
#98307=DIRECTION('ref_axis',(1.,0.,0.)) ;
#98308=DIRECTION('center_axis',(1.,-6.13317366673349E-15,0.)) ;
#98309=DIRECTION('ref_axis',(6.13317366673349E-15,1.,0.)) ;
#98310=DIRECTION('center_axis',(1.,-9.85638338623186E-18,0.)) ;
#98311=DIRECTION('ref_axis',(9.85638338623186E-18,1.,0.)) ;
#98312=DIRECTION('center_axis',(1.,0.,0.)) ;
#98313=DIRECTION('ref_axis',(0.,0.,-1.)) ;
#98314=DIRECTION('center_axis',(0.,1.,0.)) ;
#98315=DIRECTION('ref_axis',(1.,0.,0.)) ;
#98316=DIRECTION('center_axis',(0.,1.,0.)) ;
#98317=DIRECTION('ref_axis',(0.,0.,1.)) ;
#98318=DIRECTION('center_axis',(-9.85638338623186E-18,-1.,0.)) ;
#98319=DIRECTION('ref_axis',(1.,-9.85638338623186E-18,0.)) ;
#98320=DIRECTION('center_axis',(0.,1.,0.)) ;
#98321=DIRECTION('ref_axis',(0.,0.,1.)) ;
#98322=DIRECTION('center_axis',(0.,0.,1.)) ;
#98323=DIRECTION('ref_axis',(1.,0.,0.)) ;
#98324=DIRECTION('center_axis',(-1.,-1.95511867169517E-16,0.)) ;
#98325=DIRECTION('ref_axis',(1.95511867169517E-16,-1.,0.)) ;
#98326=DIRECTION('center_axis',(1.,0.,0.)) ;
#98327=DIRECTION('ref_axis',(0.,0.,-1.)) ;
#98328=DIRECTION('center_axis',(0.,1.,0.)) ;
#98329=DIRECTION('ref_axis',(1.,0.,0.)) ;
#98330=DIRECTION('center_axis',(1.22663473334668E-14,-1.,0.)) ;
#98331=DIRECTION('ref_axis',(1.,1.22663473334668E-14,0.)) ;
#98332=DIRECTION('center_axis',(-1.95511867169517E-16,1.,0.)) ;
#98333=DIRECTION('ref_axis',(-1.,-1.95511867169517E-16,0.)) ;
#98334=DIRECTION('center_axis',(0.,-1.,0.)) ;
#98335=DIRECTION('ref_axis',(0.,0.,-1.)) ;
#98336=DIRECTION('center_axis',(0.,1.,0.)) ;
#98337=DIRECTION('ref_axis',(1.,0.,0.)) ;
#98338=DIRECTION('center_axis',(-1.,0.,0.)) ;
#98339=DIRECTION('ref_axis',(0.,0.,1.)) ;
#98340=DIRECTION('center_axis',(1.,-1.06642836637918E-16,0.)) ;
#98341=DIRECTION('ref_axis',(1.06642836637918E-16,1.,0.)) ;
#98342=DIRECTION('center_axis',(1.,1.95511867169517E-16,0.)) ;
#98343=DIRECTION('ref_axis',(-1.95511867169517E-16,1.,0.)) ;
#98344=DIRECTION('center_axis',(1.,0.,0.)) ;
#98345=DIRECTION('ref_axis',(0.,0.,-1.)) ;
#98346=DIRECTION('center_axis',(0.,1.,0.)) ;
#98347=DIRECTION('ref_axis',(1.,0.,0.)) ;
#98348=DIRECTION('center_axis',(-8.43311379175855E-15,-1.,0.)) ;
#98349=DIRECTION('ref_axis',(1.,-8.43311379175855E-15,0.)) ;
#98350=DIRECTION('center_axis',(-1.95511867169517E-16,1.,0.)) ;
#98351=DIRECTION('ref_axis',(-1.,-1.95511867169517E-16,0.)) ;
#98352=DIRECTION('center_axis',(0.,-1.,0.)) ;
#98353=DIRECTION('ref_axis',(0.,0.,-1.)) ;
#98354=DIRECTION('center_axis',(-1.,1.06642836637918E-16,0.)) ;
#98355=DIRECTION('ref_axis',(-1.06642836637918E-16,-1.,0.)) ;
#98356=DIRECTION('center_axis',(1.,0.,0.)) ;
#98357=DIRECTION('ref_axis',(0.,0.,-1.)) ;
#98358=DIRECTION('center_axis',(0.,1.,0.)) ;
#98359=DIRECTION('ref_axis',(1.,0.,0.)) ;
#98360=DIRECTION('center_axis',(0.,0.,1.)) ;
#98361=DIRECTION('ref_axis',(1.,0.,0.)) ;
#98362=DIRECTION('center_axis',(0.,-1.,0.)) ;
#98363=DIRECTION('ref_axis',(0.,0.,-1.)) ;
#98364=DIRECTION('center_axis',(9.85638338623186E-18,1.,0.)) ;
#98365=DIRECTION('ref_axis',(-1.,9.85638338623186E-18,0.)) ;
#98366=DIRECTION('center_axis',(0.,-1.,0.)) ;
#98367=DIRECTION('ref_axis',(0.,0.,-1.)) ;
#98368=DIRECTION('center_axis',(0.,1.,0.)) ;
#98369=DIRECTION('ref_axis',(1.,0.,0.)) ;
#98370=DIRECTION('center_axis',(-1.,4.59988025005012E-15,0.)) ;
#98371=DIRECTION('ref_axis',(-4.59988025005012E-15,-1.,0.)) ;
#98372=DIRECTION('center_axis',(1.,-9.85638338623186E-18,0.)) ;
#98373=DIRECTION('ref_axis',(9.85638338623186E-18,1.,0.)) ;
#98374=DIRECTION('center_axis',(-1.,0.,0.)) ;
#98375=DIRECTION('ref_axis',(0.,0.,1.)) ;
#98376=DIRECTION('center_axis',(0.,1.,0.)) ;
#98377=DIRECTION('ref_axis',(1.,0.,0.)) ;
#98378=DIRECTION('center_axis',(0.,1.,0.)) ;
#98379=DIRECTION('ref_axis',(0.,0.,1.)) ;
#98380=DIRECTION('center_axis',(-9.85638338623186E-18,-1.,0.)) ;
#98381=DIRECTION('ref_axis',(1.,-9.85638338623186E-18,0.)) ;
#98382=DIRECTION('center_axis',(0.,1.,0.)) ;
#98383=DIRECTION('ref_axis',(0.,0.,1.)) ;
#98384=DIRECTION('center_axis',(0.,0.,1.)) ;
#98385=DIRECTION('ref_axis',(1.,0.,0.)) ;
#98386=DIRECTION('center_axis',(0.,0.,1.)) ;
#98387=DIRECTION('ref_axis',(1.,0.,0.)) ;
#98388=DIRECTION('center_axis',(0.,-1.,0.)) ;
#98389=DIRECTION('ref_axis',(0.,0.,-1.)) ;
#98390=DIRECTION('center_axis',(-9.85638338623186E-18,-1.,0.)) ;
#98391=DIRECTION('ref_axis',(1.,-9.85638338623186E-18,0.)) ;
#98392=DIRECTION('center_axis',(0.,-1.,0.)) ;
#98393=DIRECTION('ref_axis',(0.,0.,-1.)) ;
#98394=DIRECTION('center_axis',(0.,1.,0.)) ;
#98395=DIRECTION('ref_axis',(1.,0.,0.)) ;
#98396=DIRECTION('center_axis',(1.,-6.13317366673349E-15,0.)) ;
#98397=DIRECTION('ref_axis',(6.13317366673349E-15,1.,0.)) ;
#98398=DIRECTION('center_axis',(1.,-9.85638338623186E-18,0.)) ;
#98399=DIRECTION('ref_axis',(9.85638338623186E-18,1.,0.)) ;
#98400=DIRECTION('center_axis',(1.,0.,0.)) ;
#98401=DIRECTION('ref_axis',(0.,0.,-1.)) ;
#98402=DIRECTION('center_axis',(0.,1.,0.)) ;
#98403=DIRECTION('ref_axis',(1.,0.,0.)) ;
#98404=DIRECTION('center_axis',(0.,1.,0.)) ;
#98405=DIRECTION('ref_axis',(0.,0.,1.)) ;
#98406=DIRECTION('center_axis',(-9.85638338623186E-18,-1.,0.)) ;
#98407=DIRECTION('ref_axis',(1.,-9.85638338623186E-18,0.)) ;
#98408=DIRECTION('center_axis',(0.,1.,0.)) ;
#98409=DIRECTION('ref_axis',(0.,0.,1.)) ;
#98410=DIRECTION('center_axis',(0.,0.,1.)) ;
#98411=DIRECTION('ref_axis',(1.,0.,0.)) ;
#98412=DIRECTION('center_axis',(-1.,-1.95511867169517E-16,0.)) ;
#98413=DIRECTION('ref_axis',(1.95511867169517E-16,-1.,0.)) ;
#98414=DIRECTION('center_axis',(1.,0.,0.)) ;
#98415=DIRECTION('ref_axis',(0.,0.,-1.)) ;
#98416=DIRECTION('center_axis',(0.,1.,0.)) ;
#98417=DIRECTION('ref_axis',(1.,0.,0.)) ;
#98418=DIRECTION('center_axis',(1.22663473334668E-14,-1.,0.)) ;
#98419=DIRECTION('ref_axis',(1.,1.22663473334668E-14,0.)) ;
#98420=DIRECTION('center_axis',(-1.95511867169517E-16,1.,0.)) ;
#98421=DIRECTION('ref_axis',(-1.,-1.95511867169517E-16,0.)) ;
#98422=DIRECTION('center_axis',(0.,-1.,0.)) ;
#98423=DIRECTION('ref_axis',(0.,0.,-1.)) ;
#98424=DIRECTION('center_axis',(0.,1.,0.)) ;
#98425=DIRECTION('ref_axis',(1.,0.,0.)) ;
#98426=DIRECTION('center_axis',(-1.,0.,0.)) ;
#98427=DIRECTION('ref_axis',(0.,0.,1.)) ;
#98428=DIRECTION('center_axis',(1.,-1.06642836637918E-16,0.)) ;
#98429=DIRECTION('ref_axis',(1.06642836637918E-16,1.,0.)) ;
#98430=DIRECTION('center_axis',(1.,1.95511867169517E-16,0.)) ;
#98431=DIRECTION('ref_axis',(-1.95511867169517E-16,1.,0.)) ;
#98432=DIRECTION('center_axis',(1.,0.,0.)) ;
#98433=DIRECTION('ref_axis',(0.,0.,-1.)) ;
#98434=DIRECTION('center_axis',(0.,1.,0.)) ;
#98435=DIRECTION('ref_axis',(1.,0.,0.)) ;
#98436=DIRECTION('center_axis',(-8.43311379175855E-15,-1.,0.)) ;
#98437=DIRECTION('ref_axis',(1.,-8.43311379175855E-15,0.)) ;
#98438=DIRECTION('center_axis',(-1.95511867169517E-16,1.,0.)) ;
#98439=DIRECTION('ref_axis',(-1.,-1.95511867169517E-16,0.)) ;
#98440=DIRECTION('center_axis',(0.,-1.,0.)) ;
#98441=DIRECTION('ref_axis',(0.,0.,-1.)) ;
#98442=DIRECTION('center_axis',(-1.,1.06642836637918E-16,0.)) ;
#98443=DIRECTION('ref_axis',(-1.06642836637918E-16,-1.,0.)) ;
#98444=DIRECTION('center_axis',(1.,0.,0.)) ;
#98445=DIRECTION('ref_axis',(0.,0.,-1.)) ;
#98446=DIRECTION('center_axis',(0.,1.,0.)) ;
#98447=DIRECTION('ref_axis',(1.,0.,0.)) ;
#98448=DIRECTION('center_axis',(0.,0.,1.)) ;
#98449=DIRECTION('ref_axis',(1.,0.,0.)) ;
#98450=DIRECTION('center_axis',(0.,-1.,0.)) ;
#98451=DIRECTION('ref_axis',(0.,0.,-1.)) ;
#98452=DIRECTION('center_axis',(9.85638338623186E-18,1.,0.)) ;
#98453=DIRECTION('ref_axis',(-1.,9.85638338623186E-18,0.)) ;
#98454=DIRECTION('center_axis',(0.,-1.,0.)) ;
#98455=DIRECTION('ref_axis',(0.,0.,-1.)) ;
#98456=DIRECTION('center_axis',(0.,1.,0.)) ;
#98457=DIRECTION('ref_axis',(1.,0.,0.)) ;
#98458=DIRECTION('center_axis',(-1.,4.59988025005012E-15,0.)) ;
#98459=DIRECTION('ref_axis',(-4.59988025005012E-15,-1.,0.)) ;
#98460=DIRECTION('center_axis',(1.,-9.85638338623186E-18,0.)) ;
#98461=DIRECTION('ref_axis',(9.85638338623186E-18,1.,0.)) ;
#98462=DIRECTION('center_axis',(-1.,0.,0.)) ;
#98463=DIRECTION('ref_axis',(0.,0.,1.)) ;
#98464=DIRECTION('center_axis',(0.,1.,0.)) ;
#98465=DIRECTION('ref_axis',(1.,0.,0.)) ;
#98466=DIRECTION('center_axis',(0.,1.,0.)) ;
#98467=DIRECTION('ref_axis',(0.,0.,1.)) ;
#98468=DIRECTION('center_axis',(-9.85638338623186E-18,-1.,0.)) ;
#98469=DIRECTION('ref_axis',(1.,-9.85638338623186E-18,0.)) ;
#98470=DIRECTION('center_axis',(0.,1.,0.)) ;
#98471=DIRECTION('ref_axis',(0.,0.,1.)) ;
#98472=DIRECTION('center_axis',(0.,0.,1.)) ;
#98473=DIRECTION('ref_axis',(1.,0.,0.)) ;
#98474=DIRECTION('center_axis',(0.,0.,1.)) ;
#98475=DIRECTION('ref_axis',(1.,0.,0.)) ;
#98476=DIRECTION('center_axis',(0.,-1.,0.)) ;
#98477=DIRECTION('ref_axis',(0.,0.,-1.)) ;
#98478=DIRECTION('center_axis',(-9.85638338623186E-18,-1.,0.)) ;
#98479=DIRECTION('ref_axis',(1.,-9.85638338623186E-18,0.)) ;
#98480=DIRECTION('center_axis',(0.,-1.,0.)) ;
#98481=DIRECTION('ref_axis',(0.,0.,-1.)) ;
#98482=DIRECTION('center_axis',(0.,1.,0.)) ;
#98483=DIRECTION('ref_axis',(1.,0.,0.)) ;
#98484=DIRECTION('center_axis',(1.,-6.13317366673349E-15,0.)) ;
#98485=DIRECTION('ref_axis',(6.13317366673349E-15,1.,0.)) ;
#98486=DIRECTION('center_axis',(1.,-9.85638338623186E-18,0.)) ;
#98487=DIRECTION('ref_axis',(9.85638338623186E-18,1.,0.)) ;
#98488=DIRECTION('center_axis',(1.,0.,0.)) ;
#98489=DIRECTION('ref_axis',(0.,0.,-1.)) ;
#98490=DIRECTION('center_axis',(0.,1.,0.)) ;
#98491=DIRECTION('ref_axis',(1.,0.,0.)) ;
#98492=DIRECTION('center_axis',(0.,1.,0.)) ;
#98493=DIRECTION('ref_axis',(0.,0.,1.)) ;
#98494=DIRECTION('center_axis',(-9.85638338623186E-18,-1.,0.)) ;
#98495=DIRECTION('ref_axis',(1.,-9.85638338623186E-18,0.)) ;
#98496=DIRECTION('center_axis',(0.,1.,0.)) ;
#98497=DIRECTION('ref_axis',(0.,0.,1.)) ;
#98498=DIRECTION('center_axis',(0.,0.,1.)) ;
#98499=DIRECTION('ref_axis',(1.,0.,0.)) ;
#98500=DIRECTION('center_axis',(-1.,-1.95511867169517E-16,0.)) ;
#98501=DIRECTION('ref_axis',(1.95511867169517E-16,-1.,0.)) ;
#98502=DIRECTION('center_axis',(1.,0.,0.)) ;
#98503=DIRECTION('ref_axis',(0.,0.,-1.)) ;
#98504=DIRECTION('center_axis',(0.,1.,0.)) ;
#98505=DIRECTION('ref_axis',(1.,0.,0.)) ;
#98506=DIRECTION('center_axis',(1.22663473334668E-14,-1.,0.)) ;
#98507=DIRECTION('ref_axis',(1.,1.22663473334668E-14,0.)) ;
#98508=DIRECTION('center_axis',(-1.95511867169517E-16,1.,0.)) ;
#98509=DIRECTION('ref_axis',(-1.,-1.95511867169517E-16,0.)) ;
#98510=DIRECTION('center_axis',(0.,-1.,0.)) ;
#98511=DIRECTION('ref_axis',(0.,0.,-1.)) ;
#98512=DIRECTION('center_axis',(0.,1.,0.)) ;
#98513=DIRECTION('ref_axis',(1.,0.,0.)) ;
#98514=DIRECTION('center_axis',(-1.,0.,0.)) ;
#98515=DIRECTION('ref_axis',(0.,0.,1.)) ;
#98516=DIRECTION('center_axis',(1.,-1.06642836637918E-16,0.)) ;
#98517=DIRECTION('ref_axis',(1.06642836637918E-16,1.,0.)) ;
#98518=DIRECTION('center_axis',(1.,1.95511867169517E-16,0.)) ;
#98519=DIRECTION('ref_axis',(-1.95511867169517E-16,1.,0.)) ;
#98520=DIRECTION('center_axis',(1.,0.,0.)) ;
#98521=DIRECTION('ref_axis',(0.,0.,-1.)) ;
#98522=DIRECTION('center_axis',(0.,1.,0.)) ;
#98523=DIRECTION('ref_axis',(1.,0.,0.)) ;
#98524=DIRECTION('center_axis',(-8.43311379175855E-15,-1.,0.)) ;
#98525=DIRECTION('ref_axis',(1.,-8.43311379175855E-15,0.)) ;
#98526=DIRECTION('center_axis',(-1.95511867169517E-16,1.,0.)) ;
#98527=DIRECTION('ref_axis',(-1.,-1.95511867169517E-16,0.)) ;
#98528=DIRECTION('center_axis',(0.,-1.,0.)) ;
#98529=DIRECTION('ref_axis',(0.,0.,-1.)) ;
#98530=DIRECTION('center_axis',(-1.,1.06642836637918E-16,0.)) ;
#98531=DIRECTION('ref_axis',(-1.06642836637918E-16,-1.,0.)) ;
#98532=DIRECTION('center_axis',(1.,0.,0.)) ;
#98533=DIRECTION('ref_axis',(0.,0.,-1.)) ;
#98534=DIRECTION('center_axis',(0.,1.,0.)) ;
#98535=DIRECTION('ref_axis',(1.,0.,0.)) ;
#98536=DIRECTION('center_axis',(0.,0.,1.)) ;
#98537=DIRECTION('ref_axis',(1.,0.,0.)) ;
#98538=DIRECTION('center_axis',(0.,-1.,0.)) ;
#98539=DIRECTION('ref_axis',(0.,0.,-1.)) ;
#98540=DIRECTION('center_axis',(9.85638338623186E-18,1.,0.)) ;
#98541=DIRECTION('ref_axis',(-1.,9.85638338623186E-18,0.)) ;
#98542=DIRECTION('center_axis',(0.,-1.,0.)) ;
#98543=DIRECTION('ref_axis',(0.,0.,-1.)) ;
#98544=DIRECTION('center_axis',(0.,1.,0.)) ;
#98545=DIRECTION('ref_axis',(1.,0.,0.)) ;
#98546=DIRECTION('center_axis',(-1.,4.59988025005012E-15,0.)) ;
#98547=DIRECTION('ref_axis',(-4.59988025005012E-15,-1.,0.)) ;
#98548=DIRECTION('center_axis',(1.,-9.85638338623186E-18,0.)) ;
#98549=DIRECTION('ref_axis',(9.85638338623186E-18,1.,0.)) ;
#98550=DIRECTION('center_axis',(-1.,0.,0.)) ;
#98551=DIRECTION('ref_axis',(0.,0.,1.)) ;
#98552=DIRECTION('center_axis',(0.,1.,0.)) ;
#98553=DIRECTION('ref_axis',(1.,0.,0.)) ;
#98554=DIRECTION('center_axis',(0.,1.,0.)) ;
#98555=DIRECTION('ref_axis',(0.,0.,1.)) ;
#98556=DIRECTION('center_axis',(-9.85638338623186E-18,-1.,0.)) ;
#98557=DIRECTION('ref_axis',(1.,-9.85638338623186E-18,0.)) ;
#98558=DIRECTION('center_axis',(0.,1.,0.)) ;
#98559=DIRECTION('ref_axis',(0.,0.,1.)) ;
#98560=DIRECTION('center_axis',(0.,0.,1.)) ;
#98561=DIRECTION('ref_axis',(1.,0.,0.)) ;
#98562=DIRECTION('center_axis',(0.,0.,1.)) ;
#98563=DIRECTION('ref_axis',(1.,0.,0.)) ;
#98564=DIRECTION('center_axis',(0.,-1.,0.)) ;
#98565=DIRECTION('ref_axis',(0.,0.,-1.)) ;
#98566=DIRECTION('center_axis',(-9.85638338623186E-18,-1.,0.)) ;
#98567=DIRECTION('ref_axis',(1.,-9.85638338623186E-18,0.)) ;
#98568=DIRECTION('center_axis',(0.,-1.,0.)) ;
#98569=DIRECTION('ref_axis',(0.,0.,-1.)) ;
#98570=DIRECTION('center_axis',(0.,1.,0.)) ;
#98571=DIRECTION('ref_axis',(1.,0.,0.)) ;
#98572=DIRECTION('center_axis',(1.,-6.13317366673349E-15,0.)) ;
#98573=DIRECTION('ref_axis',(6.13317366673349E-15,1.,0.)) ;
#98574=DIRECTION('center_axis',(1.,-9.85638338623186E-18,0.)) ;
#98575=DIRECTION('ref_axis',(9.85638338623186E-18,1.,0.)) ;
#98576=DIRECTION('center_axis',(1.,0.,0.)) ;
#98577=DIRECTION('ref_axis',(0.,0.,-1.)) ;
#98578=DIRECTION('center_axis',(0.,1.,0.)) ;
#98579=DIRECTION('ref_axis',(1.,0.,0.)) ;
#98580=DIRECTION('center_axis',(0.,1.,0.)) ;
#98581=DIRECTION('ref_axis',(0.,0.,1.)) ;
#98582=DIRECTION('center_axis',(-9.85638338623186E-18,-1.,0.)) ;
#98583=DIRECTION('ref_axis',(1.,-9.85638338623186E-18,0.)) ;
#98584=DIRECTION('center_axis',(0.,1.,0.)) ;
#98585=DIRECTION('ref_axis',(0.,0.,1.)) ;
#98586=DIRECTION('center_axis',(0.,0.,1.)) ;
#98587=DIRECTION('ref_axis',(1.,0.,0.)) ;
#98588=DIRECTION('center_axis',(-1.,-1.95511867169517E-16,0.)) ;
#98589=DIRECTION('ref_axis',(1.95511867169517E-16,-1.,0.)) ;
#98590=DIRECTION('center_axis',(1.,0.,0.)) ;
#98591=DIRECTION('ref_axis',(0.,0.,-1.)) ;
#98592=DIRECTION('center_axis',(0.,1.,0.)) ;
#98593=DIRECTION('ref_axis',(1.,0.,0.)) ;
#98594=DIRECTION('center_axis',(1.22663473334668E-14,-1.,0.)) ;
#98595=DIRECTION('ref_axis',(1.,1.22663473334668E-14,0.)) ;
#98596=DIRECTION('center_axis',(-1.95511867169517E-16,1.,0.)) ;
#98597=DIRECTION('ref_axis',(-1.,-1.95511867169517E-16,0.)) ;
#98598=DIRECTION('center_axis',(0.,-1.,0.)) ;
#98599=DIRECTION('ref_axis',(0.,0.,-1.)) ;
#98600=DIRECTION('center_axis',(0.,1.,0.)) ;
#98601=DIRECTION('ref_axis',(1.,0.,0.)) ;
#98602=DIRECTION('center_axis',(-1.,0.,0.)) ;
#98603=DIRECTION('ref_axis',(0.,0.,1.)) ;
#98604=DIRECTION('center_axis',(1.,-1.06642836637918E-16,0.)) ;
#98605=DIRECTION('ref_axis',(1.06642836637918E-16,1.,0.)) ;
#98606=DIRECTION('center_axis',(1.,1.95511867169517E-16,0.)) ;
#98607=DIRECTION('ref_axis',(-1.95511867169517E-16,1.,0.)) ;
#98608=DIRECTION('center_axis',(1.,0.,0.)) ;
#98609=DIRECTION('ref_axis',(0.,0.,-1.)) ;
#98610=DIRECTION('center_axis',(0.,1.,0.)) ;
#98611=DIRECTION('ref_axis',(1.,0.,0.)) ;
#98612=DIRECTION('center_axis',(-8.43311379175855E-15,-1.,0.)) ;
#98613=DIRECTION('ref_axis',(1.,-8.43311379175855E-15,0.)) ;
#98614=DIRECTION('center_axis',(-1.95511867169517E-16,1.,0.)) ;
#98615=DIRECTION('ref_axis',(-1.,-1.95511867169517E-16,0.)) ;
#98616=DIRECTION('center_axis',(0.,-1.,0.)) ;
#98617=DIRECTION('ref_axis',(0.,0.,-1.)) ;
#98618=DIRECTION('center_axis',(-1.,1.06642836637918E-16,0.)) ;
#98619=DIRECTION('ref_axis',(-1.06642836637918E-16,-1.,0.)) ;
#98620=DIRECTION('center_axis',(1.,0.,0.)) ;
#98621=DIRECTION('ref_axis',(0.,0.,-1.)) ;
#98622=DIRECTION('center_axis',(0.,1.,0.)) ;
#98623=DIRECTION('ref_axis',(1.,0.,0.)) ;
#98624=DIRECTION('center_axis',(0.,0.,1.)) ;
#98625=DIRECTION('ref_axis',(1.,0.,0.)) ;
#98626=DIRECTION('center_axis',(0.,-1.,0.)) ;
#98627=DIRECTION('ref_axis',(0.,0.,-1.)) ;
#98628=DIRECTION('center_axis',(9.85638338623186E-18,1.,0.)) ;
#98629=DIRECTION('ref_axis',(-1.,9.85638338623186E-18,0.)) ;
#98630=DIRECTION('center_axis',(0.,-1.,0.)) ;
#98631=DIRECTION('ref_axis',(0.,0.,-1.)) ;
#98632=DIRECTION('center_axis',(0.,1.,0.)) ;
#98633=DIRECTION('ref_axis',(1.,0.,0.)) ;
#98634=DIRECTION('center_axis',(-1.,1.83995210002007E-14,0.)) ;
#98635=DIRECTION('ref_axis',(-1.83995210002007E-14,-1.,0.)) ;
#98636=DIRECTION('center_axis',(1.,-9.85638338623186E-18,0.)) ;
#98637=DIRECTION('ref_axis',(9.85638338623186E-18,1.,0.)) ;
#98638=DIRECTION('center_axis',(-1.,0.,0.)) ;
#98639=DIRECTION('ref_axis',(0.,0.,1.)) ;
#98640=DIRECTION('center_axis',(0.,1.,0.)) ;
#98641=DIRECTION('ref_axis',(1.,0.,0.)) ;
#98642=DIRECTION('center_axis',(0.,1.,0.)) ;
#98643=DIRECTION('ref_axis',(0.,0.,1.)) ;
#98644=DIRECTION('center_axis',(-9.85638338623186E-18,-1.,0.)) ;
#98645=DIRECTION('ref_axis',(1.,-9.85638338623186E-18,0.)) ;
#98646=DIRECTION('center_axis',(0.,1.,0.)) ;
#98647=DIRECTION('ref_axis',(0.,0.,1.)) ;
#98648=DIRECTION('center_axis',(0.,0.,1.)) ;
#98649=DIRECTION('ref_axis',(1.,0.,0.)) ;
#98650=DIRECTION('center_axis',(0.,0.,1.)) ;
#98651=DIRECTION('ref_axis',(1.,0.,0.)) ;
#98652=DIRECTION('center_axis',(0.,-1.,0.)) ;
#98653=DIRECTION('ref_axis',(0.,0.,-1.)) ;
#98654=DIRECTION('center_axis',(-9.85638338623186E-18,-1.,0.)) ;
#98655=DIRECTION('ref_axis',(1.,-9.85638338623186E-18,0.)) ;
#98656=DIRECTION('center_axis',(0.,-1.,0.)) ;
#98657=DIRECTION('ref_axis',(0.,0.,-1.)) ;
#98658=DIRECTION('center_axis',(0.,1.,0.)) ;
#98659=DIRECTION('ref_axis',(1.,0.,0.)) ;
#98660=DIRECTION('center_axis',(1.,2.22327545419092E-14,0.)) ;
#98661=DIRECTION('ref_axis',(-2.22327545419092E-14,1.,0.)) ;
#98662=DIRECTION('center_axis',(1.,-9.85638338623186E-18,0.)) ;
#98663=DIRECTION('ref_axis',(9.85638338623186E-18,1.,0.)) ;
#98664=DIRECTION('center_axis',(1.,0.,0.)) ;
#98665=DIRECTION('ref_axis',(0.,0.,-1.)) ;
#98666=DIRECTION('center_axis',(0.,1.,0.)) ;
#98667=DIRECTION('ref_axis',(1.,0.,0.)) ;
#98668=DIRECTION('center_axis',(0.,1.,0.)) ;
#98669=DIRECTION('ref_axis',(0.,0.,1.)) ;
#98670=DIRECTION('center_axis',(-9.85638338623186E-18,-1.,0.)) ;
#98671=DIRECTION('ref_axis',(1.,-9.85638338623186E-18,0.)) ;
#98672=DIRECTION('center_axis',(0.,1.,0.)) ;
#98673=DIRECTION('ref_axis',(0.,0.,1.)) ;
#98674=DIRECTION('center_axis',(0.,0.,1.)) ;
#98675=DIRECTION('ref_axis',(1.,0.,0.)) ;
#98676=DIRECTION('center_axis',(-1.,-1.95511867169517E-16,0.)) ;
#98677=DIRECTION('ref_axis',(1.95511867169517E-16,-1.,0.)) ;
#98678=DIRECTION('center_axis',(1.,0.,0.)) ;
#98679=DIRECTION('ref_axis',(0.,0.,-1.)) ;
#98680=DIRECTION('center_axis',(0.,1.,0.)) ;
#98681=DIRECTION('ref_axis',(1.,0.,0.)) ;
#98682=DIRECTION('center_axis',(-1.83995210002007E-14,-1.,0.)) ;
#98683=DIRECTION('ref_axis',(1.,-1.83995210002007E-14,0.)) ;
#98684=DIRECTION('center_axis',(-1.95511867169517E-16,1.,0.)) ;
#98685=DIRECTION('ref_axis',(-1.,-1.95511867169517E-16,0.)) ;
#98686=DIRECTION('center_axis',(0.,-1.,0.)) ;
#98687=DIRECTION('ref_axis',(0.,0.,-1.)) ;
#98688=DIRECTION('center_axis',(0.,1.,0.)) ;
#98689=DIRECTION('ref_axis',(1.,0.,0.)) ;
#98690=DIRECTION('center_axis',(-1.,0.,0.)) ;
#98691=DIRECTION('ref_axis',(0.,0.,1.)) ;
#98692=DIRECTION('center_axis',(1.,-1.06642836637918E-16,0.)) ;
#98693=DIRECTION('ref_axis',(1.06642836637918E-16,1.,0.)) ;
#98694=DIRECTION('center_axis',(1.,1.95511867169517E-16,0.)) ;
#98695=DIRECTION('ref_axis',(-1.95511867169517E-16,1.,0.)) ;
#98696=DIRECTION('center_axis',(1.,0.,0.)) ;
#98697=DIRECTION('ref_axis',(0.,0.,-1.)) ;
#98698=DIRECTION('center_axis',(0.,1.,0.)) ;
#98699=DIRECTION('ref_axis',(1.,0.,0.)) ;
#98700=DIRECTION('center_axis',(2.68326347919587E-14,-1.,0.)) ;
#98701=DIRECTION('ref_axis',(1.,2.68326347919587E-14,0.)) ;
#98702=DIRECTION('center_axis',(-1.95511867169517E-16,1.,0.)) ;
#98703=DIRECTION('ref_axis',(-1.,-1.95511867169517E-16,0.)) ;
#98704=DIRECTION('center_axis',(0.,-1.,0.)) ;
#98705=DIRECTION('ref_axis',(0.,0.,-1.)) ;
#98706=DIRECTION('center_axis',(-1.,1.06642836637918E-16,0.)) ;
#98707=DIRECTION('ref_axis',(-1.06642836637918E-16,-1.,0.)) ;
#98708=DIRECTION('center_axis',(1.,0.,0.)) ;
#98709=DIRECTION('ref_axis',(0.,0.,-1.)) ;
#98710=DIRECTION('center_axis',(0.,1.,0.)) ;
#98711=DIRECTION('ref_axis',(1.,0.,0.)) ;
#113858=CARTESIAN_POINT('',(0.,0.,0.)) ;
#113859=CARTESIAN_POINT('Origin',(2.3,0.,-34.29)) ;
#113860=CARTESIAN_POINT('',(2.4,-1.10218211923262E-16,-33.39)) ;
#113861=CARTESIAN_POINT('Origin',(2.4,0.,-34.29)) ;
#113862=CARTESIAN_POINT('',(2.3,-1.22464679914735E-16,-33.29)) ;
#113863=CARTESIAN_POINT('Origin',(2.3,-1.10218211923262E-16,-33.39)) ;
#113864=CARTESIAN_POINT('',(2.3,1.22464679914735E-16,-35.29)) ;
#113865=CARTESIAN_POINT('Origin',(2.3,0.,-34.29)) ;
#113866=CARTESIAN_POINT('Origin',(2.3,0.,-34.29)) ;
#113867=CARTESIAN_POINT('Origin',(1.5,0.,-34.29)) ;
#113868=CARTESIAN_POINT('',(1.4,-1.34711147906208E-16,-35.39)) ;
#113869=CARTESIAN_POINT('Origin',(1.4,0.,-34.29)) ;
#113870=CARTESIAN_POINT('',(1.5,-1.22464679914735E-16,-35.29)) ;
#113871=CARTESIAN_POINT('Origin',(1.5,-1.34711147906209E-16,-35.39)) ;
#113872=CARTESIAN_POINT('Origin',(1.5,0.,-34.29)) ;
#113873=CARTESIAN_POINT('Origin',(1.5,3.15,-33.0314213562373)) ;
#113874=CARTESIAN_POINT('',(1.5,3.07928932188135,-32.9607106781187)) ;
#113875=CARTESIAN_POINT('',(1.5,3.25,-33.0314213562373)) ;
#113876=CARTESIAN_POINT('Origin',(1.5,3.15,-33.0314213562373)) ;
#113877=CARTESIAN_POINT('',(1.4,3.15,-33.0314213562373)) ;
#113878=CARTESIAN_POINT('Origin',(1.5,3.15,-33.0314213562373)) ;
#113879=CARTESIAN_POINT('Origin',(1.5,3.15,-33.0314213562373)) ;
#113880=CARTESIAN_POINT('Origin',(0.500000000000001,-4.56640444411537E-17,
-34.69)) ;
#113881=CARTESIAN_POINT('',(0.600000000000001,0.4,-34.69)) ;
#113882=CARTESIAN_POINT('',(0.59561299721608,0.370705721320401,-34.6607057213204)) ;
#113883=CARTESIAN_POINT('Origin',(0.500000000014529,0.399999999998192,-34.6899999999979)) ;
#113884=CARTESIAN_POINT('',(0.500000000000001,0.4,-34.79)) ;
#113885=CARTESIAN_POINT('Origin',(0.500000000000001,0.4,-34.69)) ;
#113886=CARTESIAN_POINT('',(0.500000000000001,-1.9,-34.79)) ;
#113887=CARTESIAN_POINT('',(0.500000000000001,0.5,-34.79)) ;
#113888=CARTESIAN_POINT('',(0.600000000000001,-1.9,-34.69)) ;
#113889=CARTESIAN_POINT('Origin',(0.500000000000001,-1.9,-34.69)) ;
#113890=CARTESIAN_POINT('',(0.600000000000001,-0.3,-34.69)) ;
#113891=CARTESIAN_POINT('',(0.600000000000001,-2.39800009914437E-17,-34.69)) ;
#113892=CARTESIAN_POINT('',(0.600000000000001,0.299999999999999,-34.69)) ;
#113893=CARTESIAN_POINT('',(0.600000000000001,-2.39800009914437E-17,-34.69)) ;
#113894=CARTESIAN_POINT('Ctrl Pts',(0.600000000000001,0.300000000000003,
-34.69)) ;
#113895=CARTESIAN_POINT('Ctrl Pts',(0.600000000000001,0.312243016306297,
-34.69)) ;
#113896=CARTESIAN_POINT('Ctrl Pts',(0.60006974742297,0.324350425899703,
-34.6877515285214)) ;
#113897=CARTESIAN_POINT('Ctrl Pts',(0.599517124288205,0.34619696929781,
-34.6793954490601)) ;
#113898=CARTESIAN_POINT('Ctrl Pts',(0.598927484301131,0.355857825373572,
-34.6736750447227)) ;
#113899=CARTESIAN_POINT('Ctrl Pts',(0.596766673872563,0.366539012308038,
-34.6647023851096)) ;
#113900=CARTESIAN_POINT('Ctrl Pts',(0.59623562910414,0.368676603883175,
-34.6627379168092)) ;
#113901=CARTESIAN_POINT('Ctrl Pts',(0.59561299721608,0.370705721320409,
-34.6607057213204)) ;
#113902=CARTESIAN_POINT('Origin',(2.3,0.,-30.48)) ;
#113903=CARTESIAN_POINT('',(2.4,-1.10218211923262E-16,-29.58)) ;
#113904=CARTESIAN_POINT('Origin',(2.4,0.,-30.48)) ;
#113905=CARTESIAN_POINT('',(2.3,-1.22464679914735E-16,-29.48)) ;
#113906=CARTESIAN_POINT('Origin',(2.3,-1.10218211923262E-16,-29.58)) ;
#113907=CARTESIAN_POINT('',(2.3,1.22464679914735E-16,-31.48)) ;
#113908=CARTESIAN_POINT('Origin',(2.3,0.,-30.48)) ;
#113909=CARTESIAN_POINT('Origin',(2.3,0.,-30.48)) ;
#113910=CARTESIAN_POINT('Origin',(1.5,0.,-30.48)) ;
#113911=CARTESIAN_POINT('',(1.4,-1.34711147906209E-16,-31.58)) ;
#113912=CARTESIAN_POINT('Origin',(1.4,0.,-30.48)) ;
#113913=CARTESIAN_POINT('',(1.5,-1.22464679914735E-16,-31.48)) ;
#113914=CARTESIAN_POINT('Origin',(1.5,-1.34711147906209E-16,-31.58)) ;
#113915=CARTESIAN_POINT('Origin',(1.5,0.,-30.48)) ;
#113916=CARTESIAN_POINT('Origin',(1.5,3.15,-29.2214213562373)) ;
#113917=CARTESIAN_POINT('',(1.5,3.07928932188135,-29.1507106781187)) ;
#113918=CARTESIAN_POINT('',(1.5,3.25,-29.2214213562373)) ;
#113919=CARTESIAN_POINT('Origin',(1.5,3.15,-29.2214213562373)) ;
#113920=CARTESIAN_POINT('',(1.4,3.15,-29.2214213562373)) ;
#113921=CARTESIAN_POINT('Origin',(1.5,3.15,-29.2214213562373)) ;
#113922=CARTESIAN_POINT('Origin',(1.5,3.15,-29.2214213562373)) ;
#113923=CARTESIAN_POINT('Origin',(0.500000000000001,-4.56640444411542E-17,
-30.88)) ;
#113924=CARTESIAN_POINT('',(0.600000000000001,0.4,-30.88)) ;
#113925=CARTESIAN_POINT('',(0.595612997216081,0.370705721320403,-30.8507057213204)) ;
#113926=CARTESIAN_POINT('Origin',(0.500000000043895,0.399999999994469,-30.8799999999944)) ;
#113927=CARTESIAN_POINT('',(0.500000000000001,0.4,-30.98)) ;
#113928=CARTESIAN_POINT('Origin',(0.500000000000001,0.4,-30.88)) ;
#113929=CARTESIAN_POINT('',(0.500000000000001,-1.9,-30.98)) ;
#113930=CARTESIAN_POINT('',(0.500000000000001,0.5,-30.98)) ;
#113931=CARTESIAN_POINT('',(0.600000000000001,-1.9,-30.88)) ;
#113932=CARTESIAN_POINT('Origin',(0.500000000000001,-1.9,-30.88)) ;
#113933=CARTESIAN_POINT('',(0.600000000000001,-0.3,-30.88)) ;
#113934=CARTESIAN_POINT('',(0.600000000000001,-2.39800009914441E-17,-30.88)) ;
#113935=CARTESIAN_POINT('',(0.600000000000001,0.299999999999999,-30.88)) ;
#113936=CARTESIAN_POINT('',(0.600000000000001,-2.39800009914441E-17,-30.88)) ;
#113937=CARTESIAN_POINT('Ctrl Pts',(0.600000000000001,0.300000000000003,
-30.88)) ;
#113938=CARTESIAN_POINT('Ctrl Pts',(0.600000000000001,0.312243016306059,
-30.88)) ;
#113939=CARTESIAN_POINT('Ctrl Pts',(0.600069747422976,0.324350425899479,
-30.8777515285215)) ;
#113940=CARTESIAN_POINT('Ctrl Pts',(0.59951712428821,0.346196969297596,
-30.8693954490601)) ;
#113941=CARTESIAN_POINT('Ctrl Pts',(0.598927484301166,0.355857825373397,
-30.8636750447228)) ;
#113942=CARTESIAN_POINT('Ctrl Pts',(0.596766673872565,0.36653901230802,
-30.8547023851096)) ;
#113943=CARTESIAN_POINT('Ctrl Pts',(0.596235629104145,0.368676603883157,
-30.8527379168092)) ;
#113944=CARTESIAN_POINT('Ctrl Pts',(0.595612997216081,0.370705721320405,
-30.8507057213204)) ;
#113945=CARTESIAN_POINT('Origin',(2.3,0.,-26.67)) ;
#113946=CARTESIAN_POINT('',(2.4,-1.10218211923262E-16,-25.77)) ;
#113947=CARTESIAN_POINT('Origin',(2.4,0.,-26.67)) ;
#113948=CARTESIAN_POINT('',(2.3,-1.22464679914735E-16,-25.67)) ;
#113949=CARTESIAN_POINT('Origin',(2.3,-1.10218211923262E-16,-25.77)) ;
#113950=CARTESIAN_POINT('',(2.3,1.22464679914735E-16,-27.67)) ;
#113951=CARTESIAN_POINT('Origin',(2.3,0.,-26.67)) ;
#113952=CARTESIAN_POINT('Origin',(2.3,0.,-26.67)) ;
#113953=CARTESIAN_POINT('Origin',(1.5,0.,-26.67)) ;
#113954=CARTESIAN_POINT('',(1.4,-1.34711147906209E-16,-27.77)) ;
#113955=CARTESIAN_POINT('Origin',(1.4,0.,-26.67)) ;
#113956=CARTESIAN_POINT('',(1.5,-1.22464679914735E-16,-27.67)) ;
#113957=CARTESIAN_POINT('Origin',(1.5,-1.34711147906209E-16,-27.77)) ;
#113958=CARTESIAN_POINT('Origin',(1.5,0.,-26.67)) ;
#113959=CARTESIAN_POINT('Origin',(1.5,3.15,-25.4114213562373)) ;
#113960=CARTESIAN_POINT('',(1.5,3.07928932188135,-25.3407106781187)) ;
#113961=CARTESIAN_POINT('',(1.5,3.25,-25.4114213562373)) ;
#113962=CARTESIAN_POINT('Origin',(1.5,3.15,-25.4114213562373)) ;
#113963=CARTESIAN_POINT('',(1.4,3.15,-25.4114213562373)) ;
#113964=CARTESIAN_POINT('Origin',(1.5,3.15,-25.4114213562373)) ;
#113965=CARTESIAN_POINT('Origin',(1.5,3.15,-25.4114213562373)) ;
#113966=CARTESIAN_POINT('Origin',(0.500000000000001,-4.56640444411542E-17,
-27.07)) ;
#113967=CARTESIAN_POINT('',(0.600000000000001,0.4,-27.07)) ;
#113968=CARTESIAN_POINT('',(0.595612997216081,0.370705721320403,-27.0407057213204)) ;
#113969=CARTESIAN_POINT('Origin',(0.500000000043127,0.39999999999434,-27.0699999999943)) ;
#113970=CARTESIAN_POINT('',(0.500000000000001,0.4,-27.17)) ;
#113971=CARTESIAN_POINT('Origin',(0.500000000000001,0.4,-27.07)) ;
#113972=CARTESIAN_POINT('',(0.500000000000001,-1.9,-27.17)) ;
#113973=CARTESIAN_POINT('',(0.500000000000001,0.5,-27.17)) ;
#113974=CARTESIAN_POINT('',(0.600000000000001,-1.9,-27.07)) ;
#113975=CARTESIAN_POINT('Origin',(0.500000000000001,-1.9,-27.07)) ;
#113976=CARTESIAN_POINT('',(0.600000000000001,-0.3,-27.07)) ;
#113977=CARTESIAN_POINT('',(0.600000000000001,-2.39800009914441E-17,-27.07)) ;
#113978=CARTESIAN_POINT('',(0.600000000000001,0.299999999999999,-27.07)) ;
#113979=CARTESIAN_POINT('',(0.600000000000001,-2.39800009914441E-17,-27.07)) ;
#113980=CARTESIAN_POINT('Ctrl Pts',(0.600000000000001,0.300000000000003,
-27.07)) ;
#113981=CARTESIAN_POINT('Ctrl Pts',(0.600000000000001,0.312243016306037,
-27.07)) ;
#113982=CARTESIAN_POINT('Ctrl Pts',(0.600069747422976,0.324350425899459,
-27.0677515285215)) ;
#113983=CARTESIAN_POINT('Ctrl Pts',(0.59951712428821,0.346196969297585,
-27.0593954490602)) ;
#113984=CARTESIAN_POINT('Ctrl Pts',(0.598927484301167,0.355857825373385,
-27.0536750447229)) ;
#113985=CARTESIAN_POINT('Ctrl Pts',(0.596766673872565,0.366539012308015,
-27.0447023851096)) ;
#113986=CARTESIAN_POINT('Ctrl Pts',(0.596235629104144,0.368676603883154,
-27.0427379168092)) ;
#113987=CARTESIAN_POINT('Ctrl Pts',(0.59561299721608,0.370705721320403,
-27.0407057213204)) ;
#113988=CARTESIAN_POINT('Origin',(2.3,0.,-22.86)) ;
#113989=CARTESIAN_POINT('',(2.4,-1.10218211923262E-16,-21.96)) ;
#113990=CARTESIAN_POINT('Origin',(2.4,0.,-22.86)) ;
#113991=CARTESIAN_POINT('',(2.3,-1.22464679914735E-16,-21.86)) ;
#113992=CARTESIAN_POINT('Origin',(2.3,-1.10218211923262E-16,-21.96)) ;
#113993=CARTESIAN_POINT('',(2.3,1.22464679914735E-16,-23.86)) ;
#113994=CARTESIAN_POINT('Origin',(2.3,0.,-22.86)) ;
#113995=CARTESIAN_POINT('Origin',(2.3,0.,-22.86)) ;
#113996=CARTESIAN_POINT('Origin',(1.5,0.,-22.86)) ;
#113997=CARTESIAN_POINT('',(1.4,-1.34711147906209E-16,-23.96)) ;
#113998=CARTESIAN_POINT('Origin',(1.4,0.,-22.86)) ;
#113999=CARTESIAN_POINT('',(1.5,-1.22464679914735E-16,-23.86)) ;
#114000=CARTESIAN_POINT('Origin',(1.5,-1.34711147906209E-16,-23.96)) ;
#114001=CARTESIAN_POINT('Origin',(1.5,0.,-22.86)) ;
#114002=CARTESIAN_POINT('Origin',(1.5,3.15,-21.6014213562373)) ;
#114003=CARTESIAN_POINT('',(1.5,3.07928932188135,-21.5307106781187)) ;
#114004=CARTESIAN_POINT('',(1.5,3.25,-21.6014213562373)) ;
#114005=CARTESIAN_POINT('Origin',(1.5,3.15,-21.6014213562373)) ;
#114006=CARTESIAN_POINT('',(1.4,3.15,-21.6014213562373)) ;
#114007=CARTESIAN_POINT('Origin',(1.5,3.15,-21.6014213562373)) ;
#114008=CARTESIAN_POINT('Origin',(1.5,3.15,-21.6014213562373)) ;
#114009=CARTESIAN_POINT('Origin',(0.500000000000001,-4.56640444411542E-17,
-23.26)) ;
#114010=CARTESIAN_POINT('',(0.600000000000001,0.4,-23.26)) ;
#114011=CARTESIAN_POINT('',(0.595612997216081,0.370705721320403,-23.2307057213204)) ;
#114012=CARTESIAN_POINT('Origin',(0.50000000005309,0.399999999992667,-23.2599999999926)) ;
#114013=CARTESIAN_POINT('',(0.500000000000001,0.4,-23.36)) ;
#114014=CARTESIAN_POINT('Origin',(0.500000000000001,0.4,-23.26)) ;
#114015=CARTESIAN_POINT('',(0.500000000000001,-1.9,-23.36)) ;
#114016=CARTESIAN_POINT('',(0.500000000000001,0.5,-23.36)) ;
#114017=CARTESIAN_POINT('',(0.600000000000001,-1.9,-23.26)) ;
#114018=CARTESIAN_POINT('Origin',(0.500000000000001,-1.9,-23.26)) ;
#114019=CARTESIAN_POINT('',(0.600000000000001,-0.3,-23.26)) ;
#114020=CARTESIAN_POINT('',(0.600000000000001,-2.39800009914441E-17,-23.26)) ;
#114021=CARTESIAN_POINT('',(0.600000000000001,0.299999999999999,-23.26)) ;
#114022=CARTESIAN_POINT('',(0.600000000000001,-2.39800009914441E-17,-23.26)) ;
#114023=CARTESIAN_POINT('Ctrl Pts',(0.600000000000001,0.300000000000003,
-23.26)) ;
#114024=CARTESIAN_POINT('Ctrl Pts',(0.600000000000001,0.312243016306061,
-23.26)) ;
#114025=CARTESIAN_POINT('Ctrl Pts',(0.600069747422976,0.324350425899477,
-23.2577515285215)) ;
#114026=CARTESIAN_POINT('Ctrl Pts',(0.599517124288211,0.346196969297576,
-23.2493954490602)) ;
#114027=CARTESIAN_POINT('Ctrl Pts',(0.598927484301166,0.35585782537339,
-23.2436750447229)) ;
#114028=CARTESIAN_POINT('Ctrl Pts',(0.596766673872565,0.36653901230802,
-23.2347023851096)) ;
#114029=CARTESIAN_POINT('Ctrl Pts',(0.596235629104145,0.368676603883157,
-23.2327379168092)) ;
#114030=CARTESIAN_POINT('Ctrl Pts',(0.595612997216081,0.370705721320404,
-23.2307057213204)) ;
#114031=CARTESIAN_POINT('Origin',(2.3,0.,-19.05)) ;
#114032=CARTESIAN_POINT('',(2.4,-1.10218211923262E-16,-18.15)) ;
#114033=CARTESIAN_POINT('Origin',(2.4,0.,-19.05)) ;
#114034=CARTESIAN_POINT('',(2.3,-1.22464679914735E-16,-18.05)) ;
#114035=CARTESIAN_POINT('Origin',(2.3,-1.10218211923262E-16,-18.15)) ;
#114036=CARTESIAN_POINT('',(2.3,1.22464679914735E-16,-20.05)) ;
#114037=CARTESIAN_POINT('Origin',(2.3,0.,-19.05)) ;
#114038=CARTESIAN_POINT('Origin',(2.3,0.,-19.05)) ;
#114039=CARTESIAN_POINT('Origin',(1.5,0.,-19.05)) ;
#114040=CARTESIAN_POINT('',(1.4,-1.34711147906209E-16,-20.15)) ;
#114041=CARTESIAN_POINT('Origin',(1.4,0.,-19.05)) ;
#114042=CARTESIAN_POINT('',(1.5,-1.22464679914735E-16,-20.05)) ;
#114043=CARTESIAN_POINT('Origin',(1.5,-1.34711147906209E-16,-20.15)) ;
#114044=CARTESIAN_POINT('Origin',(1.5,0.,-19.05)) ;
#114045=CARTESIAN_POINT('Origin',(1.5,3.15,-17.7914213562373)) ;
#114046=CARTESIAN_POINT('',(1.5,3.07928932188135,-17.7207106781187)) ;
#114047=CARTESIAN_POINT('',(1.5,3.25,-17.7914213562373)) ;
#114048=CARTESIAN_POINT('Origin',(1.5,3.15,-17.7914213562373)) ;
#114049=CARTESIAN_POINT('',(1.4,3.15,-17.7914213562373)) ;
#114050=CARTESIAN_POINT('Origin',(1.5,3.15,-17.7914213562373)) ;
#114051=CARTESIAN_POINT('Origin',(1.5,3.15,-17.7914213562373)) ;
#114052=CARTESIAN_POINT('Origin',(0.500000000000001,-4.56640444411542E-17,
-19.45)) ;
#114053=CARTESIAN_POINT('',(0.600000000000001,0.4,-19.45)) ;
#114054=CARTESIAN_POINT('',(0.595612997216081,0.370705721320403,-19.4207057213204)) ;
#114055=CARTESIAN_POINT('Origin',(0.500000000041676,0.399999999994165,-19.4499999999941)) ;
#114056=CARTESIAN_POINT('',(0.500000000000001,0.4,-19.55)) ;
#114057=CARTESIAN_POINT('Origin',(0.500000000000001,0.4,-19.45)) ;
#114058=CARTESIAN_POINT('',(0.500000000000001,-1.9,-19.55)) ;
#114059=CARTESIAN_POINT('',(0.500000000000001,0.5,-19.55)) ;
#114060=CARTESIAN_POINT('',(0.600000000000001,-1.9,-19.45)) ;
#114061=CARTESIAN_POINT('Origin',(0.500000000000001,-1.9,-19.45)) ;
#114062=CARTESIAN_POINT('',(0.600000000000001,-0.3,-19.45)) ;
#114063=CARTESIAN_POINT('',(0.600000000000001,-2.39800009914441E-17,-19.45)) ;
#114064=CARTESIAN_POINT('',(0.600000000000001,0.299999999999999,-19.45)) ;
#114065=CARTESIAN_POINT('',(0.600000000000001,-2.39800009914441E-17,-19.45)) ;
#114066=CARTESIAN_POINT('Ctrl Pts',(0.600000000000001,0.300000000000003,
-19.45)) ;
#114067=CARTESIAN_POINT('Ctrl Pts',(0.600000000000001,0.312243016306433,
-19.45)) ;
#114068=CARTESIAN_POINT('Ctrl Pts',(0.600069747422966,0.324350425899823,
-19.4477515285214)) ;
#114069=CARTESIAN_POINT('Ctrl Pts',(0.599517124288202,0.346196969297921,
-19.43939544906)) ;
#114070=CARTESIAN_POINT('Ctrl Pts',(0.598927484301112,0.355857825373661,
-19.4336750447226)) ;
#114071=CARTESIAN_POINT('Ctrl Pts',(0.596766673872561,0.366539012308041,
-19.4247023851096)) ;
#114072=CARTESIAN_POINT('Ctrl Pts',(0.596235629104139,0.368676603883175,
-19.4227379168092)) ;
#114073=CARTESIAN_POINT('Ctrl Pts',(0.595612997216081,0.370705721320404,
-19.4207057213204)) ;
#114074=CARTESIAN_POINT('Origin',(2.3,0.,-15.24)) ;
#114075=CARTESIAN_POINT('',(2.4,-1.10218211923262E-16,-14.34)) ;
#114076=CARTESIAN_POINT('Origin',(2.4,0.,-15.24)) ;
#114077=CARTESIAN_POINT('',(2.3,-1.22464679914735E-16,-14.24)) ;
#114078=CARTESIAN_POINT('Origin',(2.3,-1.10218211923262E-16,-14.34)) ;
#114079=CARTESIAN_POINT('',(2.3,1.22464679914735E-16,-16.24)) ;
#114080=CARTESIAN_POINT('Origin',(2.3,0.,-15.24)) ;
#114081=CARTESIAN_POINT('Origin',(2.3,0.,-15.24)) ;
#114082=CARTESIAN_POINT('Origin',(1.5,0.,-15.24)) ;
#114083=CARTESIAN_POINT('',(1.4,-1.34711147906209E-16,-16.34)) ;
#114084=CARTESIAN_POINT('Origin',(1.4,0.,-15.24)) ;
#114085=CARTESIAN_POINT('',(1.5,-1.22464679914735E-16,-16.24)) ;
#114086=CARTESIAN_POINT('Origin',(1.5,-1.34711147906209E-16,-16.34)) ;
#114087=CARTESIAN_POINT('Origin',(1.5,0.,-15.24)) ;
#114088=CARTESIAN_POINT('Origin',(1.5,3.15,-13.9814213562373)) ;
#114089=CARTESIAN_POINT('',(1.5,3.07928932188135,-13.9107106781187)) ;
#114090=CARTESIAN_POINT('',(1.5,3.25,-13.9814213562373)) ;
#114091=CARTESIAN_POINT('Origin',(1.5,3.15,-13.9814213562373)) ;
#114092=CARTESIAN_POINT('',(1.4,3.15,-13.9814213562373)) ;
#114093=CARTESIAN_POINT('Origin',(1.5,3.15,-13.9814213562373)) ;
#114094=CARTESIAN_POINT('Origin',(1.5,3.15,-13.9814213562373)) ;
#114095=CARTESIAN_POINT('Origin',(0.500000000000001,-4.56640444411542E-17,
-15.64)) ;
#114096=CARTESIAN_POINT('',(0.600000000000001,0.4,-15.64)) ;
#114097=CARTESIAN_POINT('',(0.595612997216081,0.370705721320403,-15.6107057213204)) ;
#114098=CARTESIAN_POINT('Origin',(0.499999999962138,0.400000000005185,-15.6400000000051)) ;
#114099=CARTESIAN_POINT('',(0.500000000000001,0.4,-15.74)) ;
#114100=CARTESIAN_POINT('Origin',(0.500000000000001,0.4,-15.64)) ;
#114101=CARTESIAN_POINT('',(0.500000000000001,-1.9,-15.74)) ;
#114102=CARTESIAN_POINT('',(0.500000000000001,0.5,-15.74)) ;
#114103=CARTESIAN_POINT('',(0.600000000000001,-1.9,-15.64)) ;
#114104=CARTESIAN_POINT('Origin',(0.500000000000001,-1.9,-15.64)) ;
#114105=CARTESIAN_POINT('',(0.600000000000001,-0.3,-15.64)) ;
#114106=CARTESIAN_POINT('',(0.600000000000001,-2.39800009914441E-17,-15.64)) ;
#114107=CARTESIAN_POINT('',(0.600000000000001,0.299999999999999,-15.64)) ;
#114108=CARTESIAN_POINT('',(0.600000000000001,-2.39800009914441E-17,-15.64)) ;
#114109=CARTESIAN_POINT('Ctrl Pts',(0.600000000000001,0.300000000000003,
-15.64)) ;
#114110=CARTESIAN_POINT('Ctrl Pts',(0.600000000000001,0.312243016306305,
-15.64)) ;
#114111=CARTESIAN_POINT('Ctrl Pts',(0.60006974742297,0.324350425899701,
-15.6377515285214)) ;
#114112=CARTESIAN_POINT('Ctrl Pts',(0.599517124288205,0.346196969297796,
-15.6293954490601)) ;
#114113=CARTESIAN_POINT('Ctrl Pts',(0.59892748430113,0.355857825373563,
-15.6236750447227)) ;
#114114=CARTESIAN_POINT('Ctrl Pts',(0.596766673872562,0.366539012308031,
-15.6147023851096)) ;
#114115=CARTESIAN_POINT('Ctrl Pts',(0.596235629104141,0.368676603883168,
-15.6127379168092)) ;
#114116=CARTESIAN_POINT('Ctrl Pts',(0.59561299721608,0.370705721320404,
-15.6107057213204)) ;
#114117=CARTESIAN_POINT('Origin',(2.3,0.,-11.43)) ;
#114118=CARTESIAN_POINT('',(2.4,-1.10218211923262E-16,-10.53)) ;
#114119=CARTESIAN_POINT('Origin',(2.4,0.,-11.43)) ;
#114120=CARTESIAN_POINT('',(2.3,-1.22464679914735E-16,-10.43)) ;
#114121=CARTESIAN_POINT('Origin',(2.3,-1.10218211923262E-16,-10.53)) ;
#114122=CARTESIAN_POINT('',(2.3,1.22464679914735E-16,-12.43)) ;
#114123=CARTESIAN_POINT('Origin',(2.3,0.,-11.43)) ;
#114124=CARTESIAN_POINT('Origin',(2.3,0.,-11.43)) ;
#114125=CARTESIAN_POINT('Origin',(1.5,0.,-11.43)) ;
#114126=CARTESIAN_POINT('',(1.4,-1.34711147906209E-16,-12.53)) ;
#114127=CARTESIAN_POINT('Origin',(1.4,0.,-11.43)) ;
#114128=CARTESIAN_POINT('',(1.5,-1.22464679914735E-16,-12.43)) ;
#114129=CARTESIAN_POINT('Origin',(1.5,-1.34711147906209E-16,-12.53)) ;
#114130=CARTESIAN_POINT('Origin',(1.5,0.,-11.43)) ;
#114131=CARTESIAN_POINT('Origin',(1.5,3.15,-10.1714213562373)) ;
#114132=CARTESIAN_POINT('',(1.5,3.07928932188135,-10.1007106781187)) ;
#114133=CARTESIAN_POINT('',(1.5,3.25,-10.1714213562373)) ;
#114134=CARTESIAN_POINT('Origin',(1.5,3.15,-10.1714213562373)) ;
#114135=CARTESIAN_POINT('',(1.4,3.15,-10.1714213562373)) ;
#114136=CARTESIAN_POINT('Origin',(1.5,3.15,-10.1714213562373)) ;
#114137=CARTESIAN_POINT('Origin',(1.5,3.15,-10.1714213562373)) ;
#114138=CARTESIAN_POINT('Origin',(0.500000000000001,-4.56640444411542E-17,
-11.83)) ;
#114139=CARTESIAN_POINT('',(0.600000000000001,0.4,-11.83)) ;
#114140=CARTESIAN_POINT('',(0.59561299721608,0.370705721320402,-11.8007057213204)) ;
#114141=CARTESIAN_POINT('Origin',(0.500000000002749,0.399999999999878,-11.8299999999996)) ;
#114142=CARTESIAN_POINT('',(0.500000000000001,0.4,-11.93)) ;
#114143=CARTESIAN_POINT('Origin',(0.500000000000001,0.4,-11.83)) ;
#114144=CARTESIAN_POINT('',(0.500000000000001,-1.9,-11.93)) ;
#114145=CARTESIAN_POINT('',(0.500000000000001,0.5,-11.93)) ;
#114146=CARTESIAN_POINT('',(0.600000000000001,-1.9,-11.83)) ;
#114147=CARTESIAN_POINT('Origin',(0.500000000000001,-1.9,-11.83)) ;
#114148=CARTESIAN_POINT('',(0.600000000000001,-0.3,-11.83)) ;
#114149=CARTESIAN_POINT('',(0.600000000000001,-2.39800009914441E-17,-11.83)) ;
#114150=CARTESIAN_POINT('',(0.600000000000001,0.299999999999999,-11.83)) ;
#114151=CARTESIAN_POINT('',(0.600000000000001,-2.39800009914441E-17,-11.83)) ;
#114152=CARTESIAN_POINT('Ctrl Pts',(0.600000000000001,0.300000000000003,
-11.83)) ;
#114153=CARTESIAN_POINT('Ctrl Pts',(0.600000000000001,0.312243016306181,
-11.83)) ;
#114154=CARTESIAN_POINT('Ctrl Pts',(0.600069747422973,0.324350425899585,
-11.8277515285214)) ;
#114155=CARTESIAN_POINT('Ctrl Pts',(0.599517124288208,0.346196969297684,
-11.8193954490601)) ;
#114156=CARTESIAN_POINT('Ctrl Pts',(0.598927484301148,0.355857825373472,
-11.8136750447228)) ;
#114157=CARTESIAN_POINT('Ctrl Pts',(0.596766673872564,0.366539012308024,
-11.8047023851096)) ;
#114158=CARTESIAN_POINT('Ctrl Pts',(0.596235629104143,0.368676603883159,
-11.8027379168092)) ;
#114159=CARTESIAN_POINT('Ctrl Pts',(0.595612997216081,0.370705721320402,
-11.8007057213204)) ;
#114160=CARTESIAN_POINT('Origin',(2.3,0.,-7.62)) ;
#114161=CARTESIAN_POINT('',(2.4,-1.10218211923262E-16,-6.72)) ;
#114162=CARTESIAN_POINT('Origin',(2.4,0.,-7.62)) ;
#114163=CARTESIAN_POINT('',(2.3,-1.22464679914735E-16,-6.62)) ;
#114164=CARTESIAN_POINT('Origin',(2.3,-1.10218211923262E-16,-6.72)) ;
#114165=CARTESIAN_POINT('',(2.3,1.22464679914735E-16,-8.62)) ;
#114166=CARTESIAN_POINT('Origin',(2.3,0.,-7.62)) ;
#114167=CARTESIAN_POINT('Origin',(2.3,0.,-7.62)) ;
#114168=CARTESIAN_POINT('Origin',(1.5,0.,-7.62)) ;
#114169=CARTESIAN_POINT('',(1.4,-1.34711147906209E-16,-8.72)) ;
#114170=CARTESIAN_POINT('Origin',(1.4,0.,-7.62)) ;
#114171=CARTESIAN_POINT('',(1.5,-1.22464679914735E-16,-8.62)) ;
#114172=CARTESIAN_POINT('Origin',(1.5,-1.34711147906209E-16,-8.72)) ;
#114173=CARTESIAN_POINT('Origin',(1.5,0.,-7.62)) ;
#114174=CARTESIAN_POINT('Origin',(1.5,3.15,-6.36142135623731)) ;
#114175=CARTESIAN_POINT('',(1.5,3.07928932188135,-6.29071067811866)) ;
#114176=CARTESIAN_POINT('',(1.5,3.25,-6.36142135623731)) ;
#114177=CARTESIAN_POINT('Origin',(1.5,3.15,-6.36142135623731)) ;
#114178=CARTESIAN_POINT('',(1.4,3.15,-6.36142135623731)) ;
#114179=CARTESIAN_POINT('Origin',(1.5,3.15,-6.36142135623731)) ;
#114180=CARTESIAN_POINT('Origin',(1.5,3.15,-6.36142135623731)) ;
#114181=CARTESIAN_POINT('Origin',(0.500000000000001,-4.56640444411542E-17,
-8.02)) ;
#114182=CARTESIAN_POINT('',(0.600000000000001,0.4,-8.02)) ;
#114183=CARTESIAN_POINT('',(0.59561299721608,0.370705721320402,-7.9907057213204)) ;
#114184=CARTESIAN_POINT('Origin',(0.499999999996157,0.400000000000788,-8.02000000000056)) ;
#114185=CARTESIAN_POINT('',(0.500000000000001,0.4,-8.12)) ;
#114186=CARTESIAN_POINT('Origin',(0.500000000000001,0.4,-8.02)) ;
#114187=CARTESIAN_POINT('',(0.500000000000001,-1.9,-8.12)) ;
#114188=CARTESIAN_POINT('',(0.500000000000001,0.5,-8.12)) ;
#114189=CARTESIAN_POINT('',(0.600000000000001,-1.9,-8.02)) ;
#114190=CARTESIAN_POINT('Origin',(0.500000000000001,-1.9,-8.02)) ;
#114191=CARTESIAN_POINT('',(0.600000000000001,-0.3,-8.02)) ;
#114192=CARTESIAN_POINT('',(0.600000000000001,-2.39800009914441E-17,-8.02)) ;
#114193=CARTESIAN_POINT('',(0.600000000000001,0.299999999999999,-8.02)) ;
#114194=CARTESIAN_POINT('',(0.600000000000001,-2.39800009914441E-17,-8.02)) ;
#114195=CARTESIAN_POINT('Ctrl Pts',(0.600000000000001,0.300000000000003,
-8.02)) ;
#114196=CARTESIAN_POINT('Ctrl Pts',(0.600000000000001,0.312243016306057,
-8.02)) ;
#114197=CARTESIAN_POINT('Ctrl Pts',(0.600069747422976,0.32435042589947,
-8.01775152852148)) ;
#114198=CARTESIAN_POINT('Ctrl Pts',(0.599517124288211,0.346196969297575,
-8.00939544906016)) ;
#114199=CARTESIAN_POINT('Ctrl Pts',(0.598927484301167,0.355857825373384,
-8.00367504472285)) ;
#114200=CARTESIAN_POINT('Ctrl Pts',(0.596766673872565,0.366539012308017,
-7.99470238510958)) ;
#114201=CARTESIAN_POINT('Ctrl Pts',(0.596235629104145,0.368676603883154,
-7.9927379168092)) ;
#114202=CARTESIAN_POINT('Ctrl Pts',(0.59561299721608,0.370705721320404,
-7.9907057213204)) ;
#114203=CARTESIAN_POINT('Origin',(2.3,0.,-3.81)) ;
#114204=CARTESIAN_POINT('',(2.4,-1.10218211923262E-16,-2.91)) ;
#114205=CARTESIAN_POINT('Origin',(2.4,0.,-3.81)) ;
#114206=CARTESIAN_POINT('',(2.3,-1.22464679914735E-16,-2.81)) ;
#114207=CARTESIAN_POINT('Origin',(2.3,-1.10218211923262E-16,-2.91)) ;
#114208=CARTESIAN_POINT('',(2.3,1.22464679914735E-16,-4.81)) ;
#114209=CARTESIAN_POINT('Origin',(2.3,0.,-3.81)) ;
#114210=CARTESIAN_POINT('Origin',(2.3,0.,-3.81)) ;
#114211=CARTESIAN_POINT('Origin',(7.9,3.15,-5.06857864376269)) ;
#114212=CARTESIAN_POINT('',(8.,3.35,-5.06857864376269)) ;
#114213=CARTESIAN_POINT('',(8.,3.00857864376269,-5.21)) ;
#114214=CARTESIAN_POINT('Origin',(8.,3.15,-5.06857864376269)) ;
#114215=CARTESIAN_POINT('',(7.9,3.25,-5.06857864376269)) ;
#114216=CARTESIAN_POINT('Origin',(7.9,3.35,-5.06857864376269)) ;
#114217=CARTESIAN_POINT('',(7.9,3.07928932188135,-5.13928932188135)) ;
#114218=CARTESIAN_POINT('Origin',(7.9,3.15,-5.06857864376269)) ;
#114219=CARTESIAN_POINT('Origin',(7.9,3.00857864376269,-5.21)) ;
#114220=CARTESIAN_POINT('Origin',(7.9,3.15,-8.87857864376269)) ;
#114221=CARTESIAN_POINT('',(8.,3.35,-8.87857864376269)) ;
#114222=CARTESIAN_POINT('',(8.,3.00857864376269,-9.02)) ;
#114223=CARTESIAN_POINT('Origin',(8.,3.15,-8.87857864376269)) ;
#114224=CARTESIAN_POINT('',(7.9,3.25,-8.87857864376269)) ;
#114225=CARTESIAN_POINT('Origin',(7.9,3.35,-8.87857864376269)) ;
#114226=CARTESIAN_POINT('',(7.9,3.07928932188135,-8.94928932188134)) ;
#114227=CARTESIAN_POINT('Origin',(7.9,3.15,-8.87857864376269)) ;
#114228=CARTESIAN_POINT('Origin',(7.9,3.00857864376269,-9.02)) ;
#114229=CARTESIAN_POINT('Origin',(7.9,3.15,-12.6885786437627)) ;
#114230=CARTESIAN_POINT('',(8.,3.35,-12.6885786437627)) ;
#114231=CARTESIAN_POINT('',(8.,3.00857864376269,-12.83)) ;
#114232=CARTESIAN_POINT('Origin',(8.,3.15,-12.6885786437627)) ;
#114233=CARTESIAN_POINT('',(7.9,3.25,-12.6885786437627)) ;
#114234=CARTESIAN_POINT('Origin',(7.9,3.35,-12.6885786437627)) ;
#114235=CARTESIAN_POINT('',(7.9,3.07928932188135,-12.7592893218813)) ;
#114236=CARTESIAN_POINT('Origin',(7.9,3.15,-12.6885786437627)) ;
#114237=CARTESIAN_POINT('Origin',(7.9,3.00857864376269,-12.83)) ;
#114238=CARTESIAN_POINT('Origin',(7.9,3.15,-16.4985786437627)) ;
#114239=CARTESIAN_POINT('',(8.,3.35,-16.4985786437627)) ;
#114240=CARTESIAN_POINT('',(8.,3.00857864376269,-16.64)) ;
#114241=CARTESIAN_POINT('Origin',(8.,3.15,-16.4985786437627)) ;
#114242=CARTESIAN_POINT('',(7.9,3.25,-16.4985786437627)) ;
#114243=CARTESIAN_POINT('Origin',(7.9,3.35,-16.4985786437627)) ;
#114244=CARTESIAN_POINT('',(7.9,3.07928932188135,-16.5692893218813)) ;
#114245=CARTESIAN_POINT('Origin',(7.9,3.15,-16.4985786437627)) ;
#114246=CARTESIAN_POINT('Origin',(7.9,3.00857864376269,-16.64)) ;
#114247=CARTESIAN_POINT('Origin',(7.9,3.15,-20.3085786437627)) ;
#114248=CARTESIAN_POINT('',(8.,3.35,-20.3085786437627)) ;
#114249=CARTESIAN_POINT('',(8.,3.00857864376269,-20.45)) ;
#114250=CARTESIAN_POINT('Origin',(8.,3.15,-20.3085786437627)) ;
#114251=CARTESIAN_POINT('',(7.9,3.25,-20.3085786437627)) ;
#114252=CARTESIAN_POINT('Origin',(7.9,3.35,-20.3085786437627)) ;
#114253=CARTESIAN_POINT('',(7.9,3.07928932188135,-20.3792893218813)) ;
#114254=CARTESIAN_POINT('Origin',(7.9,3.15,-20.3085786437627)) ;
#114255=CARTESIAN_POINT('Origin',(7.9,3.00857864376269,-20.45)) ;
#114256=CARTESIAN_POINT('Origin',(7.9,3.15,-24.1185786437627)) ;
#114257=CARTESIAN_POINT('',(8.,3.35,-24.1185786437627)) ;
#114258=CARTESIAN_POINT('',(8.,3.00857864376269,-24.26)) ;
#114259=CARTESIAN_POINT('Origin',(8.,3.15,-24.1185786437627)) ;
#114260=CARTESIAN_POINT('',(7.9,3.25,-24.1185786437627)) ;
#114261=CARTESIAN_POINT('Origin',(7.9,3.35,-24.1185786437627)) ;
#114262=CARTESIAN_POINT('',(7.9,3.07928932188135,-24.1892893218813)) ;
#114263=CARTESIAN_POINT('Origin',(7.9,3.15,-24.1185786437627)) ;
#114264=CARTESIAN_POINT('Origin',(7.9,3.00857864376269,-24.26)) ;
#114265=CARTESIAN_POINT('Origin',(7.9,3.15,-27.9285786437627)) ;
#114266=CARTESIAN_POINT('',(8.,3.35,-27.9285786437627)) ;
#114267=CARTESIAN_POINT('',(8.,3.00857864376269,-28.07)) ;
#114268=CARTESIAN_POINT('Origin',(8.,3.15,-27.9285786437627)) ;
#114269=CARTESIAN_POINT('',(7.9,3.25,-27.9285786437627)) ;
#114270=CARTESIAN_POINT('Origin',(7.9,3.35,-27.9285786437627)) ;
#114271=CARTESIAN_POINT('',(7.9,3.07928932188135,-27.9992893218813)) ;
#114272=CARTESIAN_POINT('Origin',(7.9,3.15,-27.9285786437627)) ;
#114273=CARTESIAN_POINT('Origin',(7.9,3.00857864376269,-28.07)) ;
#114274=CARTESIAN_POINT('Origin',(7.9,3.15,-31.7385786437627)) ;
#114275=CARTESIAN_POINT('',(8.,3.35,-31.7385786437627)) ;
#114276=CARTESIAN_POINT('',(8.,3.00857864376269,-31.88)) ;
#114277=CARTESIAN_POINT('Origin',(8.,3.15,-31.7385786437627)) ;
#114278=CARTESIAN_POINT('',(7.9,3.25,-31.7385786437627)) ;
#114279=CARTESIAN_POINT('Origin',(7.9,3.35,-31.7385786437627)) ;
#114280=CARTESIAN_POINT('',(7.9,3.07928932188135,-31.8092893218813)) ;
#114281=CARTESIAN_POINT('Origin',(7.9,3.15,-31.7385786437627)) ;
#114282=CARTESIAN_POINT('Origin',(7.9,3.00857864376269,-31.88)) ;
#114283=CARTESIAN_POINT('Origin',(7.9,3.15,-35.5485786437627)) ;
#114284=CARTESIAN_POINT('',(8.,3.35,-35.5485786437627)) ;
#114285=CARTESIAN_POINT('',(8.,3.00857864376269,-35.69)) ;
#114286=CARTESIAN_POINT('Origin',(8.,3.15,-35.5485786437627)) ;
#114287=CARTESIAN_POINT('',(7.9,3.25,-35.5485786437627)) ;
#114288=CARTESIAN_POINT('Origin',(7.9,3.35,-35.5485786437627)) ;
#114289=CARTESIAN_POINT('',(7.9,3.07928932188135,-35.6192893218813)) ;
#114290=CARTESIAN_POINT('Origin',(7.9,3.15,-35.5485786437627)) ;
#114291=CARTESIAN_POINT('Origin',(7.9,3.00857864376269,-35.69)) ;
#114292=CARTESIAN_POINT('Origin',(1.5,0.,-3.81)) ;
#114293=CARTESIAN_POINT('',(1.4,-1.34711147906209E-16,-4.91)) ;
#114294=CARTESIAN_POINT('Origin',(1.4,0.,-3.81)) ;
#114295=CARTESIAN_POINT('',(1.5,-1.22464679914735E-16,-4.81)) ;
#114296=CARTESIAN_POINT('Origin',(1.5,-1.34711147906209E-16,-4.91)) ;
#114297=CARTESIAN_POINT('Origin',(1.5,0.,-3.81)) ;
#114298=CARTESIAN_POINT('Origin',(1.5,3.15,-2.55142135623731)) ;
#114299=CARTESIAN_POINT('',(1.5,3.07928932188135,-2.48071067811865)) ;
#114300=CARTESIAN_POINT('',(1.5,3.25,-2.55142135623731)) ;
#114301=CARTESIAN_POINT('Origin',(1.5,3.15,-2.55142135623731)) ;
#114302=CARTESIAN_POINT('',(1.4,3.15,-2.55142135623731)) ;
#114303=CARTESIAN_POINT('Origin',(1.5,3.15,-2.55142135623731)) ;
#114304=CARTESIAN_POINT('Origin',(1.5,3.15,-2.55142135623731)) ;
#114305=CARTESIAN_POINT('Origin',(0.500000000000001,-4.56640444411539E-17,
-4.21)) ;
#114306=CARTESIAN_POINT('',(0.600000000000001,0.4,-4.21)) ;
#114307=CARTESIAN_POINT('',(0.595612997216081,0.370705721320403,-4.1807057213204)) ;
#114308=CARTESIAN_POINT('Origin',(0.499999999992608,0.400000000001211,-4.21000000000122)) ;
#114309=CARTESIAN_POINT('',(0.500000000000001,0.4,-4.31)) ;
#114310=CARTESIAN_POINT('Origin',(0.500000000000001,0.4,-4.21)) ;
#114311=CARTESIAN_POINT('',(0.500000000000001,-1.9,-4.31)) ;
#114312=CARTESIAN_POINT('',(0.500000000000001,0.5,-4.31)) ;
#114313=CARTESIAN_POINT('',(0.600000000000001,-1.9,-4.21)) ;
#114314=CARTESIAN_POINT('Origin',(0.500000000000001,-1.9,-4.21)) ;
#114315=CARTESIAN_POINT('',(0.600000000000001,-0.3,-4.21)) ;
#114316=CARTESIAN_POINT('',(0.600000000000001,-2.39800009914439E-17,-4.21)) ;
#114317=CARTESIAN_POINT('',(0.600000000000001,0.299999999999999,-4.21)) ;
#114318=CARTESIAN_POINT('',(0.600000000000001,-2.39800009914439E-17,-4.21)) ;
#114319=CARTESIAN_POINT('Ctrl Pts',(0.600000000000001,0.300000000000003,
-4.21)) ;
#114320=CARTESIAN_POINT('Ctrl Pts',(0.600000000000001,0.312243016306119,
-4.21)) ;
#114321=CARTESIAN_POINT('Ctrl Pts',(0.600069747422974,0.324350425899533,
-4.20775152852146)) ;
#114322=CARTESIAN_POINT('Ctrl Pts',(0.599517124288209,0.346196969297642,
-4.19939544906013)) ;
#114323=CARTESIAN_POINT('Ctrl Pts',(0.598927484301157,0.355857825373437,
-4.19367504472281)) ;
#114324=CARTESIAN_POINT('Ctrl Pts',(0.596766673872564,0.366539012308024,
-4.18470238510957)) ;
#114325=CARTESIAN_POINT('Ctrl Pts',(0.596235629104143,0.36867660388316,
-4.18273791680919)) ;
#114326=CARTESIAN_POINT('Ctrl Pts',(0.595612997216081,0.370705721320404,
-4.1807057213204)) ;
#114327=CARTESIAN_POINT('Origin',(2.4,0.,-34.29)) ;
#114328=CARTESIAN_POINT('',(2.4,-1.22464679914735E-16,-35.29)) ;
#114329=CARTESIAN_POINT('Origin',(2.4,0.,-30.48)) ;
#114330=CARTESIAN_POINT('',(2.4,-1.22464679914735E-16,-31.48)) ;
#114331=CARTESIAN_POINT('Origin',(2.4,0.,-26.67)) ;
#114332=CARTESIAN_POINT('',(2.4,-1.22464679914735E-16,-27.67)) ;
#114333=CARTESIAN_POINT('Origin',(2.4,0.,-22.86)) ;
#114334=CARTESIAN_POINT('',(2.4,-1.22464679914735E-16,-23.86)) ;
#114335=CARTESIAN_POINT('Origin',(2.4,0.,-19.05)) ;
#114336=CARTESIAN_POINT('',(2.4,-1.22464679914735E-16,-20.05)) ;
#114337=CARTESIAN_POINT('Origin',(2.4,0.,-15.24)) ;
#114338=CARTESIAN_POINT('',(2.4,-1.22464679914735E-16,-16.24)) ;
#114339=CARTESIAN_POINT('Origin',(2.4,0.,-11.43)) ;
#114340=CARTESIAN_POINT('',(2.4,-1.22464679914735E-16,-12.43)) ;
#114341=CARTESIAN_POINT('Origin',(2.4,0.,-7.62)) ;
#114342=CARTESIAN_POINT('',(2.4,-1.22464679914735E-16,-8.62)) ;
#114343=CARTESIAN_POINT('Origin',(2.4,0.,-3.81)) ;
#114344=CARTESIAN_POINT('',(2.4,-1.22464679914735E-16,-4.81)) ;
#114345=CARTESIAN_POINT('Origin',(1.4,3.15,-5.06857864376269)) ;
#114346=CARTESIAN_POINT('',(1.5,3.25,-5.06857864376269)) ;
#114347=CARTESIAN_POINT('',(1.5,3.07928932188135,-5.13928932188135)) ;
#114348=CARTESIAN_POINT('Origin',(1.5,3.15,-5.06857864376269)) ;
#114349=CARTESIAN_POINT('',(1.4,3.07928932188135,-5.13928932188135)) ;
#114350=CARTESIAN_POINT('',(1.4,3.25,-5.06857864376269)) ;
#114351=CARTESIAN_POINT('Origin',(1.4,3.15,-8.87857864376269)) ;
#114352=CARTESIAN_POINT('',(1.5,3.25,-8.87857864376269)) ;
#114353=CARTESIAN_POINT('',(1.5,3.07928932188135,-8.94928932188134)) ;
#114354=CARTESIAN_POINT('Origin',(1.5,3.15,-8.87857864376269)) ;
#114355=CARTESIAN_POINT('',(1.4,3.07928932188135,-8.94928932188134)) ;
#114356=CARTESIAN_POINT('',(1.4,3.25,-8.87857864376269)) ;
#114357=CARTESIAN_POINT('Origin',(1.4,3.15,-12.6885786437627)) ;
#114358=CARTESIAN_POINT('',(1.5,3.25,-12.6885786437627)) ;
#114359=CARTESIAN_POINT('',(1.5,3.07928932188135,-12.7592893218813)) ;
#114360=CARTESIAN_POINT('Origin',(1.5,3.15,-12.6885786437627)) ;
#114361=CARTESIAN_POINT('',(1.4,3.07928932188135,-12.7592893218813)) ;
#114362=CARTESIAN_POINT('',(1.4,3.25,-12.6885786437627)) ;
#114363=CARTESIAN_POINT('Origin',(1.4,3.15,-16.4985786437627)) ;
#114364=CARTESIAN_POINT('',(1.5,3.25,-16.4985786437627)) ;
#114365=CARTESIAN_POINT('',(1.5,3.07928932188135,-16.5692893218813)) ;
#114366=CARTESIAN_POINT('Origin',(1.5,3.15,-16.4985786437627)) ;
#114367=CARTESIAN_POINT('',(1.4,3.07928932188135,-16.5692893218813)) ;
#114368=CARTESIAN_POINT('',(1.4,3.25,-16.4985786437627)) ;
#114369=CARTESIAN_POINT('Origin',(1.4,3.15,-20.3085786437627)) ;
#114370=CARTESIAN_POINT('',(1.5,3.25,-20.3085786437627)) ;
#114371=CARTESIAN_POINT('',(1.5,3.07928932188135,-20.3792893218813)) ;
#114372=CARTESIAN_POINT('Origin',(1.5,3.15,-20.3085786437627)) ;
#114373=CARTESIAN_POINT('',(1.4,3.07928932188135,-20.3792893218813)) ;
#114374=CARTESIAN_POINT('',(1.4,3.25,-20.3085786437627)) ;
#114375=CARTESIAN_POINT('Origin',(1.4,3.15,-24.1185786437627)) ;
#114376=CARTESIAN_POINT('',(1.5,3.25,-24.1185786437627)) ;
#114377=CARTESIAN_POINT('',(1.5,3.07928932188135,-24.1892893218813)) ;
#114378=CARTESIAN_POINT('Origin',(1.5,3.15,-24.1185786437627)) ;
#114379=CARTESIAN_POINT('',(1.4,3.07928932188135,-24.1892893218813)) ;
#114380=CARTESIAN_POINT('',(1.4,3.25,-24.1185786437627)) ;
#114381=CARTESIAN_POINT('Origin',(1.4,3.15,-27.9285786437627)) ;
#114382=CARTESIAN_POINT('',(1.5,3.25,-27.9285786437627)) ;
#114383=CARTESIAN_POINT('',(1.5,3.07928932188135,-27.9992893218813)) ;
#114384=CARTESIAN_POINT('Origin',(1.5,3.15,-27.9285786437627)) ;
#114385=CARTESIAN_POINT('',(1.4,3.07928932188135,-27.9992893218813)) ;
#114386=CARTESIAN_POINT('',(1.4,3.25,-27.9285786437627)) ;
#114387=CARTESIAN_POINT('Origin',(1.4,3.15,-31.7385786437627)) ;
#114388=CARTESIAN_POINT('',(1.5,3.25,-31.7385786437627)) ;
#114389=CARTESIAN_POINT('',(1.5,3.07928932188135,-31.8092893218813)) ;
#114390=CARTESIAN_POINT('Origin',(1.5,3.15,-31.7385786437627)) ;
#114391=CARTESIAN_POINT('',(1.4,3.07928932188135,-31.8092893218813)) ;
#114392=CARTESIAN_POINT('',(1.4,3.25,-31.7385786437627)) ;
#114393=CARTESIAN_POINT('Origin',(1.4,3.15,-35.5485786437627)) ;
#114394=CARTESIAN_POINT('',(1.5,3.25,-35.5485786437627)) ;
#114395=CARTESIAN_POINT('',(1.5,3.07928932188135,-35.6192893218813)) ;
#114396=CARTESIAN_POINT('Origin',(1.5,3.15,-35.5485786437627)) ;
#114397=CARTESIAN_POINT('',(1.4,3.07928932188135,-35.6192893218813)) ;
#114398=CARTESIAN_POINT('',(1.4,3.25,-35.5485786437627)) ;
#114399=CARTESIAN_POINT('Origin',(2.3,0.,0.)) ;
#114400=CARTESIAN_POINT('',(2.4,-1.10218211923262E-16,0.9)) ;
#114401=CARTESIAN_POINT('Origin',(2.4,0.,0.)) ;
#114402=CARTESIAN_POINT('',(2.3,-1.22464679914735E-16,1.)) ;
#114403=CARTESIAN_POINT('Origin',(2.3,-1.10218211923262E-16,0.9)) ;
#114404=CARTESIAN_POINT('',(2.3,1.22464679914735E-16,-1.)) ;
#114405=CARTESIAN_POINT('Origin',(2.3,0.,0.)) ;
#114406=CARTESIAN_POINT('Origin',(2.3,0.,0.)) ;
#114407=CARTESIAN_POINT('Origin',(7.9,3.15,-1.25857864376269)) ;
#114408=CARTESIAN_POINT('',(8.,3.35,-1.25857864376269)) ;
#114409=CARTESIAN_POINT('',(8.,3.00857864376269,-1.4)) ;
#114410=CARTESIAN_POINT('Origin',(8.,3.15,-1.25857864376269)) ;
#114411=CARTESIAN_POINT('',(7.9,3.25,-1.25857864376269)) ;
#114412=CARTESIAN_POINT('Origin',(7.9,3.35,-1.25857864376269)) ;
#114413=CARTESIAN_POINT('',(7.9,3.07928932188135,-1.32928932188135)) ;
#114414=CARTESIAN_POINT('Origin',(7.9,3.15,-1.25857864376269)) ;
#114415=CARTESIAN_POINT('Origin',(7.9,3.00857864376269,-1.4)) ;
#114416=CARTESIAN_POINT('Origin',(1.5,0.,0.)) ;
#114417=CARTESIAN_POINT('',(1.4,-1.34711147906209E-16,-1.1)) ;
#114418=CARTESIAN_POINT('Origin',(1.4,0.,0.)) ;
#114419=CARTESIAN_POINT('',(1.5,-1.22464679914735E-16,-1.)) ;
#114420=CARTESIAN_POINT('Origin',(1.5,-1.34711147906209E-16,-1.1)) ;
#114421=CARTESIAN_POINT('Origin',(1.5,0.,0.)) ;
#114422=CARTESIAN_POINT('Origin',(1.5,3.15,1.25857864376269)) ;
#114423=CARTESIAN_POINT('',(1.5,3.07928932188135,1.32928932188135)) ;
#114424=CARTESIAN_POINT('',(1.5,3.25,1.25857864376269)) ;
#114425=CARTESIAN_POINT('Origin',(1.5,3.15,1.25857864376269)) ;
#114426=CARTESIAN_POINT('',(1.4,3.15,1.25857864376269)) ;
#114427=CARTESIAN_POINT('Origin',(1.5,3.15,1.25857864376269)) ;
#114428=CARTESIAN_POINT('Origin',(1.5,3.15,1.25857864376269)) ;
#114429=CARTESIAN_POINT('Origin',(0.500000000000001,-4.5664044441154E-17,
-0.4)) ;
#114430=CARTESIAN_POINT('',(0.600000000000001,0.4,-0.4)) ;
#114431=CARTESIAN_POINT('',(0.595612997216081,0.370705721320403,-0.370705721320403)) ;
#114432=CARTESIAN_POINT('Origin',(0.499999999989667,0.400000000001553,-0.400000000001553)) ;
#114433=CARTESIAN_POINT('',(0.500000000000001,0.4,-0.5)) ;
#114434=CARTESIAN_POINT('Origin',(0.500000000000001,0.4,-0.4)) ;
#114435=CARTESIAN_POINT('',(0.500000000000001,-1.9,-0.5)) ;
#114436=CARTESIAN_POINT('',(0.500000000000001,0.5,-0.5)) ;
#114437=CARTESIAN_POINT('',(0.600000000000001,-1.9,-0.4)) ;
#114438=CARTESIAN_POINT('Origin',(0.500000000000001,-1.9,-0.4)) ;
#114439=CARTESIAN_POINT('',(0.600000000000001,-0.3,-0.4)) ;
#114440=CARTESIAN_POINT('',(0.600000000000001,-2.3980000991444E-17,-0.4)) ;
#114441=CARTESIAN_POINT('',(0.600000000000001,0.299999999999999,-0.4)) ;
#114442=CARTESIAN_POINT('',(0.600000000000001,-2.3980000991444E-17,-0.4)) ;
#114443=CARTESIAN_POINT('Ctrl Pts',(0.600000000000001,0.300000000000003,
-0.4)) ;
#114444=CARTESIAN_POINT('Ctrl Pts',(0.600000000000001,0.312243016306053,
-0.4)) ;
#114445=CARTESIAN_POINT('Ctrl Pts',(0.600069747422976,0.324350425899471,
-0.397751528521482)) ;
#114446=CARTESIAN_POINT('Ctrl Pts',(0.599517124288211,0.34619696929758,
-0.389395449060154)) ;
#114447=CARTESIAN_POINT('Ctrl Pts',(0.598927484301167,0.355857825373388,
-0.383675044722851)) ;
#114448=CARTESIAN_POINT('Ctrl Pts',(0.596766673872565,0.36653901230802,
-0.374702385109574)) ;
#114449=CARTESIAN_POINT('Ctrl Pts',(0.596235629104145,0.368676603883155,
-0.372737916809195)) ;
#114450=CARTESIAN_POINT('Ctrl Pts',(0.595612997216081,0.370705721320403,
-0.370705721320403)) ;
#114451=CARTESIAN_POINT('Origin',(2.4,0.,0.)) ;
#114452=CARTESIAN_POINT('',(2.4,-1.22464679914735E-16,-1.)) ;
#114453=CARTESIAN_POINT('Origin',(1.4,3.15,-1.25857864376269)) ;
#114454=CARTESIAN_POINT('',(1.5,3.25,-1.25857864376269)) ;
#114455=CARTESIAN_POINT('',(1.5,3.07928932188135,-1.32928932188135)) ;
#114456=CARTESIAN_POINT('Origin',(1.5,3.15,-1.25857864376269)) ;
#114457=CARTESIAN_POINT('',(1.4,3.07928932188135,-1.32928932188135)) ;
#114458=CARTESIAN_POINT('',(1.4,3.25,-1.25857864376269)) ;
#114459=CARTESIAN_POINT('Origin',(0.600000000000001,2.80617032878603E-17,
-34.29)) ;
#114460=CARTESIAN_POINT('',(0.600000000000001,-1.9,-33.89)) ;
#114461=CARTESIAN_POINT('',(0.600000000000001,-0.3,-33.89)) ;
#114462=CARTESIAN_POINT('',(0.600000000000001,-2.39800009914436E-17,-33.89)) ;
#114463=CARTESIAN_POINT('',(0.6,-0.4,-33.99)) ;
#114464=CARTESIAN_POINT('Origin',(0.6,-0.3,-33.99)) ;
#114465=CARTESIAN_POINT('',(0.6,-0.4,-34.59)) ;
#114466=CARTESIAN_POINT('',(0.6,-0.4,-33.89)) ;
#114467=CARTESIAN_POINT('Origin',(0.6,-0.3,-34.59)) ;
#114468=CARTESIAN_POINT('',(0.600000000000001,-2.1,-34.89)) ;
#114469=CARTESIAN_POINT('Origin',(0.600000000000001,-1.9,-34.89)) ;
#114470=CARTESIAN_POINT('',(0.600000000000001,-2.1,-35.565)) ;
#114471=CARTESIAN_POINT('',(0.600000000000001,-2.1,-34.29)) ;
#114472=CARTESIAN_POINT('',(0.600000000000001,-2.9,-35.565)) ;
#114473=CARTESIAN_POINT('',(0.600000000000001,-3.69904270612699E-17,-35.565)) ;
#114474=CARTESIAN_POINT('',(0.600000000000001,-2.9,-33.015)) ;
#114475=CARTESIAN_POINT('',(0.600000000000001,-2.9,-34.29)) ;
#114476=CARTESIAN_POINT('',(0.600000000000001,-2.1,-33.015)) ;
#114477=CARTESIAN_POINT('',(0.600000000000001,1.58165963986121E-16,-33.015)) ;
#114478=CARTESIAN_POINT('',(0.600000000000001,-2.1,-33.69)) ;
#114479=CARTESIAN_POINT('',(0.600000000000001,-2.1,-34.29)) ;
#114480=CARTESIAN_POINT('Origin',(0.600000000000001,-1.9,-33.69)) ;
#114481=CARTESIAN_POINT('Origin',(0.600000000000001,2.80617032878603E-17,
-30.48)) ;
#114482=CARTESIAN_POINT('',(0.600000000000001,-1.9,-30.08)) ;
#114483=CARTESIAN_POINT('',(0.600000000000001,-0.3,-30.08)) ;
#114484=CARTESIAN_POINT('',(0.600000000000001,-2.39800009914441E-17,-30.08)) ;
#114485=CARTESIAN_POINT('',(0.6,-0.4,-30.18)) ;
#114486=CARTESIAN_POINT('Origin',(0.6,-0.3,-30.18)) ;
#114487=CARTESIAN_POINT('',(0.6,-0.4,-30.78)) ;
#114488=CARTESIAN_POINT('',(0.6,-0.4,-30.08)) ;
#114489=CARTESIAN_POINT('Origin',(0.6,-0.3,-30.78)) ;
#114490=CARTESIAN_POINT('',(0.600000000000001,-2.1,-31.08)) ;
#114491=CARTESIAN_POINT('Origin',(0.600000000000001,-1.9,-31.08)) ;
#114492=CARTESIAN_POINT('',(0.600000000000001,-2.1,-31.755)) ;
#114493=CARTESIAN_POINT('',(0.600000000000001,-2.1,-30.48)) ;
#114494=CARTESIAN_POINT('',(0.600000000000001,-2.9,-31.755)) ;
#114495=CARTESIAN_POINT('',(0.600000000000001,-3.69904270612699E-17,-31.755)) ;
#114496=CARTESIAN_POINT('',(0.600000000000001,-2.9,-29.205)) ;
#114497=CARTESIAN_POINT('',(0.600000000000001,-2.9,-30.48)) ;
#114498=CARTESIAN_POINT('',(0.600000000000001,-2.1,-29.205)) ;
#114499=CARTESIAN_POINT('',(0.600000000000001,1.58165963986121E-16,-29.205)) ;
#114500=CARTESIAN_POINT('',(0.600000000000001,-2.1,-29.88)) ;
#114501=CARTESIAN_POINT('',(0.600000000000001,-2.1,-30.48)) ;
#114502=CARTESIAN_POINT('Origin',(0.600000000000001,-1.9,-29.88)) ;
#114503=CARTESIAN_POINT('Origin',(0.600000000000001,2.80617032878603E-17,
-26.67)) ;
#114504=CARTESIAN_POINT('',(0.600000000000001,-1.9,-26.27)) ;
#114505=CARTESIAN_POINT('',(0.600000000000001,-0.3,-26.27)) ;
#114506=CARTESIAN_POINT('',(0.600000000000001,-2.39800009914441E-17,-26.27)) ;
#114507=CARTESIAN_POINT('',(0.6,-0.4,-26.37)) ;
#114508=CARTESIAN_POINT('Origin',(0.6,-0.3,-26.37)) ;
#114509=CARTESIAN_POINT('',(0.6,-0.4,-26.97)) ;
#114510=CARTESIAN_POINT('',(0.6,-0.4,-26.27)) ;
#114511=CARTESIAN_POINT('Origin',(0.6,-0.3,-26.97)) ;
#114512=CARTESIAN_POINT('',(0.600000000000001,-2.1,-27.27)) ;
#114513=CARTESIAN_POINT('Origin',(0.600000000000001,-1.9,-27.27)) ;
#114514=CARTESIAN_POINT('',(0.600000000000001,-2.1,-27.945)) ;
#114515=CARTESIAN_POINT('',(0.600000000000001,-2.1,-26.67)) ;
#114516=CARTESIAN_POINT('',(0.600000000000001,-2.9,-27.945)) ;
#114517=CARTESIAN_POINT('',(0.600000000000001,-3.69904270612701E-17,-27.945)) ;
#114518=CARTESIAN_POINT('',(0.600000000000001,-2.9,-25.395)) ;
#114519=CARTESIAN_POINT('',(0.600000000000001,-2.9,-26.67)) ;
#114520=CARTESIAN_POINT('',(0.600000000000001,-2.1,-25.395)) ;
#114521=CARTESIAN_POINT('',(0.600000000000001,1.58165963986121E-16,-25.395)) ;
#114522=CARTESIAN_POINT('',(0.600000000000001,-2.1,-26.07)) ;
#114523=CARTESIAN_POINT('',(0.600000000000001,-2.1,-26.67)) ;
#114524=CARTESIAN_POINT('Origin',(0.600000000000001,-1.9,-26.07)) ;
#114525=CARTESIAN_POINT('Origin',(0.600000000000001,2.80617032878603E-17,
-22.86)) ;
#114526=CARTESIAN_POINT('',(0.600000000000001,-1.9,-22.46)) ;
#114527=CARTESIAN_POINT('',(0.600000000000001,-0.3,-22.46)) ;
#114528=CARTESIAN_POINT('',(0.600000000000001,-2.39800009914441E-17,-22.46)) ;
#114529=CARTESIAN_POINT('',(0.6,-0.4,-22.56)) ;
#114530=CARTESIAN_POINT('Origin',(0.6,-0.3,-22.56)) ;
#114531=CARTESIAN_POINT('',(0.6,-0.4,-23.16)) ;
#114532=CARTESIAN_POINT('',(0.6,-0.4,-22.46)) ;
#114533=CARTESIAN_POINT('Origin',(0.6,-0.3,-23.16)) ;
#114534=CARTESIAN_POINT('',(0.600000000000001,-2.1,-23.46)) ;
#114535=CARTESIAN_POINT('Origin',(0.600000000000001,-1.9,-23.46)) ;
#114536=CARTESIAN_POINT('',(0.600000000000001,-2.1,-24.135)) ;
#114537=CARTESIAN_POINT('',(0.600000000000001,-2.1,-22.86)) ;
#114538=CARTESIAN_POINT('',(0.600000000000001,-2.9,-24.135)) ;
#114539=CARTESIAN_POINT('',(0.600000000000001,-3.69904270612701E-17,-24.135)) ;
#114540=CARTESIAN_POINT('',(0.600000000000001,-2.9,-21.585)) ;
#114541=CARTESIAN_POINT('',(0.600000000000001,-2.9,-22.86)) ;
#114542=CARTESIAN_POINT('',(0.600000000000001,-2.1,-21.585)) ;
#114543=CARTESIAN_POINT('',(0.600000000000001,1.58165963986121E-16,-21.585)) ;
#114544=CARTESIAN_POINT('',(0.600000000000001,-2.1,-22.26)) ;
#114545=CARTESIAN_POINT('',(0.600000000000001,-2.1,-22.86)) ;
#114546=CARTESIAN_POINT('Origin',(0.600000000000001,-1.9,-22.26)) ;
#114547=CARTESIAN_POINT('Origin',(0.600000000000001,2.80617032878603E-17,
-19.05)) ;
#114548=CARTESIAN_POINT('',(0.600000000000001,-1.9,-18.65)) ;
#114549=CARTESIAN_POINT('',(0.600000000000001,-0.3,-18.65)) ;
#114550=CARTESIAN_POINT('',(0.600000000000001,-2.39800009914441E-17,-18.65)) ;
#114551=CARTESIAN_POINT('',(0.6,-0.4,-18.75)) ;
#114552=CARTESIAN_POINT('Origin',(0.6,-0.3,-18.75)) ;
#114553=CARTESIAN_POINT('',(0.6,-0.4,-19.35)) ;
#114554=CARTESIAN_POINT('',(0.6,-0.4,-18.65)) ;
#114555=CARTESIAN_POINT('Origin',(0.6,-0.3,-19.35)) ;
#114556=CARTESIAN_POINT('',(0.600000000000001,-2.1,-19.65)) ;
#114557=CARTESIAN_POINT('Origin',(0.600000000000001,-1.9,-19.65)) ;
#114558=CARTESIAN_POINT('',(0.600000000000001,-2.1,-20.325)) ;
#114559=CARTESIAN_POINT('',(0.600000000000001,-2.1,-19.05)) ;
#114560=CARTESIAN_POINT('',(0.600000000000001,-2.9,-20.325)) ;
#114561=CARTESIAN_POINT('',(0.600000000000001,-3.69904270612701E-17,-20.325)) ;
#114562=CARTESIAN_POINT('',(0.600000000000001,-2.9,-17.775)) ;
#114563=CARTESIAN_POINT('',(0.600000000000001,-2.9,-19.05)) ;
#114564=CARTESIAN_POINT('',(0.600000000000001,-2.1,-17.775)) ;
#114565=CARTESIAN_POINT('',(0.600000000000001,1.58165963986121E-16,-17.775)) ;
#114566=CARTESIAN_POINT('',(0.600000000000001,-2.1,-18.45)) ;
#114567=CARTESIAN_POINT('',(0.600000000000001,-2.1,-19.05)) ;
#114568=CARTESIAN_POINT('Origin',(0.600000000000001,-1.9,-18.45)) ;
#114569=CARTESIAN_POINT('Origin',(0.600000000000001,2.80617032878603E-17,
-15.24)) ;
#114570=CARTESIAN_POINT('',(0.600000000000001,-1.9,-14.84)) ;
#114571=CARTESIAN_POINT('',(0.600000000000001,-0.3,-14.84)) ;
#114572=CARTESIAN_POINT('',(0.600000000000001,-2.39800009914441E-17,-14.84)) ;
#114573=CARTESIAN_POINT('',(0.6,-0.4,-14.94)) ;
#114574=CARTESIAN_POINT('Origin',(0.6,-0.3,-14.94)) ;
#114575=CARTESIAN_POINT('',(0.6,-0.4,-15.54)) ;
#114576=CARTESIAN_POINT('',(0.6,-0.4,-14.84)) ;
#114577=CARTESIAN_POINT('Origin',(0.6,-0.3,-15.54)) ;
#114578=CARTESIAN_POINT('',(0.600000000000001,-2.1,-15.84)) ;
#114579=CARTESIAN_POINT('Origin',(0.600000000000001,-1.9,-15.84)) ;
#114580=CARTESIAN_POINT('',(0.600000000000001,-2.1,-16.515)) ;
#114581=CARTESIAN_POINT('',(0.600000000000001,-2.1,-15.24)) ;
#114582=CARTESIAN_POINT('',(0.600000000000001,-2.9,-16.515)) ;
#114583=CARTESIAN_POINT('',(0.600000000000001,-3.69904270612701E-17,-16.515)) ;
#114584=CARTESIAN_POINT('',(0.600000000000001,-2.9,-13.965)) ;
#114585=CARTESIAN_POINT('',(0.600000000000001,-2.9,-15.24)) ;
#114586=CARTESIAN_POINT('',(0.600000000000001,-2.1,-13.965)) ;
#114587=CARTESIAN_POINT('',(0.600000000000001,1.58165963986121E-16,-13.965)) ;
#114588=CARTESIAN_POINT('',(0.600000000000001,-2.1,-14.64)) ;
#114589=CARTESIAN_POINT('',(0.600000000000001,-2.1,-15.24)) ;
#114590=CARTESIAN_POINT('Origin',(0.600000000000001,-1.9,-14.64)) ;
#114591=CARTESIAN_POINT('Origin',(0.600000000000001,2.80617032878603E-17,
-11.43)) ;
#114592=CARTESIAN_POINT('',(0.600000000000001,-1.9,-11.03)) ;
#114593=CARTESIAN_POINT('',(0.600000000000001,-0.3,-11.03)) ;
#114594=CARTESIAN_POINT('',(0.600000000000001,-2.39800009914441E-17,-11.03)) ;
#114595=CARTESIAN_POINT('',(0.6,-0.4,-11.13)) ;
#114596=CARTESIAN_POINT('Origin',(0.6,-0.3,-11.13)) ;
#114597=CARTESIAN_POINT('',(0.6,-0.4,-11.73)) ;
#114598=CARTESIAN_POINT('',(0.6,-0.4,-11.03)) ;
#114599=CARTESIAN_POINT('Origin',(0.6,-0.3,-11.73)) ;
#114600=CARTESIAN_POINT('',(0.600000000000001,-2.1,-12.03)) ;
#114601=CARTESIAN_POINT('Origin',(0.600000000000001,-1.9,-12.03)) ;
#114602=CARTESIAN_POINT('',(0.600000000000001,-2.1,-12.705)) ;
#114603=CARTESIAN_POINT('',(0.600000000000001,-2.1,-11.43)) ;
#114604=CARTESIAN_POINT('',(0.600000000000001,-2.9,-12.705)) ;
#114605=CARTESIAN_POINT('',(0.600000000000001,-3.69904270612701E-17,-12.705)) ;
#114606=CARTESIAN_POINT('',(0.600000000000001,-2.9,-10.155)) ;
#114607=CARTESIAN_POINT('',(0.600000000000001,-2.9,-11.43)) ;
#114608=CARTESIAN_POINT('',(0.600000000000001,-2.1,-10.155)) ;
#114609=CARTESIAN_POINT('',(0.600000000000001,1.58165963986121E-16,-10.155)) ;
#114610=CARTESIAN_POINT('',(0.600000000000001,-2.1,-10.83)) ;
#114611=CARTESIAN_POINT('',(0.600000000000001,-2.1,-11.43)) ;
#114612=CARTESIAN_POINT('Origin',(0.600000000000001,-1.9,-10.83)) ;
#114613=CARTESIAN_POINT('Origin',(0.600000000000001,2.80617032878603E-17,
-7.62)) ;
#114614=CARTESIAN_POINT('',(0.600000000000001,-1.9,-7.22)) ;
#114615=CARTESIAN_POINT('',(0.600000000000001,-0.3,-7.22)) ;
#114616=CARTESIAN_POINT('',(0.600000000000001,-2.39800009914439E-17,-7.22)) ;
#114617=CARTESIAN_POINT('',(0.6,-0.4,-7.32)) ;
#114618=CARTESIAN_POINT('Origin',(0.6,-0.3,-7.32)) ;
#114619=CARTESIAN_POINT('',(0.6,-0.4,-7.92)) ;
#114620=CARTESIAN_POINT('',(0.6,-0.4,-7.22)) ;
#114621=CARTESIAN_POINT('Origin',(0.6,-0.3,-7.92)) ;
#114622=CARTESIAN_POINT('',(0.600000000000001,-2.1,-8.22)) ;
#114623=CARTESIAN_POINT('Origin',(0.600000000000001,-1.9,-8.22)) ;
#114624=CARTESIAN_POINT('',(0.600000000000001,-2.1,-8.895)) ;
#114625=CARTESIAN_POINT('',(0.600000000000001,-2.1,-7.62)) ;
#114626=CARTESIAN_POINT('',(0.600000000000001,-2.9,-8.895)) ;
#114627=CARTESIAN_POINT('',(0.600000000000001,-3.69904270612701E-17,-8.895)) ;
#114628=CARTESIAN_POINT('',(0.600000000000001,-2.9,-6.345)) ;
#114629=CARTESIAN_POINT('',(0.600000000000001,-2.9,-7.62)) ;
#114630=CARTESIAN_POINT('',(0.600000000000001,-2.1,-6.345)) ;
#114631=CARTESIAN_POINT('',(0.600000000000001,1.58165963986121E-16,-6.345)) ;
#114632=CARTESIAN_POINT('',(0.600000000000001,-2.1,-7.02)) ;
#114633=CARTESIAN_POINT('',(0.600000000000001,-2.1,-7.62)) ;
#114634=CARTESIAN_POINT('Origin',(0.600000000000001,-1.9,-7.02)) ;
#114635=CARTESIAN_POINT('Origin',(0.600000000000001,2.80617032878603E-17,
-3.81)) ;
#114636=CARTESIAN_POINT('',(0.600000000000001,-1.9,-3.41)) ;
#114637=CARTESIAN_POINT('',(0.600000000000001,-0.3,-3.41)) ;
#114638=CARTESIAN_POINT('',(0.600000000000001,-2.3980000991444E-17,-3.41)) ;
#114639=CARTESIAN_POINT('',(0.6,-0.4,-3.51)) ;
#114640=CARTESIAN_POINT('Origin',(0.6,-0.3,-3.51)) ;
#114641=CARTESIAN_POINT('',(0.6,-0.4,-4.11)) ;
#114642=CARTESIAN_POINT('',(0.6,-0.4,-3.41)) ;
#114643=CARTESIAN_POINT('Origin',(0.6,-0.3,-4.11)) ;
#114644=CARTESIAN_POINT('',(0.600000000000001,-2.1,-4.41)) ;
#114645=CARTESIAN_POINT('Origin',(0.600000000000001,-1.9,-4.41)) ;
#114646=CARTESIAN_POINT('',(0.600000000000001,-2.1,-5.085)) ;
#114647=CARTESIAN_POINT('',(0.600000000000001,-2.1,-3.81)) ;
#114648=CARTESIAN_POINT('',(0.600000000000001,-2.9,-5.085)) ;
#114649=CARTESIAN_POINT('',(0.600000000000001,-3.699042706127E-17,-5.085)) ;
#114650=CARTESIAN_POINT('',(0.600000000000001,-2.9,-2.535)) ;
#114651=CARTESIAN_POINT('',(0.600000000000001,-2.9,-3.81)) ;
#114652=CARTESIAN_POINT('',(0.600000000000001,-2.1,-2.535)) ;
#114653=CARTESIAN_POINT('',(0.600000000000001,1.58165963986121E-16,-2.535)) ;
#114654=CARTESIAN_POINT('',(0.600000000000001,-2.1,-3.21)) ;
#114655=CARTESIAN_POINT('',(0.600000000000001,-2.1,-3.81)) ;
#114656=CARTESIAN_POINT('Origin',(0.600000000000001,-1.9,-3.21)) ;
#114657=CARTESIAN_POINT('Origin',(-0.999999999999999,1.25,-35.665)) ;
#114658=CARTESIAN_POINT('',(-1.1,-1.9,-35.665)) ;
#114659=CARTESIAN_POINT('',(-0.899999999999999,-2.1,-35.665)) ;
#114660=CARTESIAN_POINT('Origin',(-0.899999999999999,-1.9,-35.665)) ;
#114661=CARTESIAN_POINT('',(-1.1,-2.9,-35.665)) ;
#114662=CARTESIAN_POINT('',(-1.1,-2.9,-35.665)) ;
#114663=CARTESIAN_POINT('',(0.500000000000001,-2.9,-35.665)) ;
#114664=CARTESIAN_POINT('',(0.600000000000001,-2.9,-35.665)) ;
#114665=CARTESIAN_POINT('',(0.500000000000001,-2.1,-35.665)) ;
#114666=CARTESIAN_POINT('',(0.5,1.25,-35.665)) ;
#114667=CARTESIAN_POINT('',(-0.999999999999999,-2.1,-35.665)) ;
#114668=CARTESIAN_POINT('Origin',(-0.999999999999999,1.25,-32.915)) ;
#114669=CARTESIAN_POINT('',(-0.899999999999999,-2.1,-32.915)) ;
#114670=CARTESIAN_POINT('',(-1.1,-1.9,-32.915)) ;
#114671=CARTESIAN_POINT('Origin',(-0.899999999999999,-1.9,-32.915)) ;
#114672=CARTESIAN_POINT('',(0.500000000000001,-2.1,-32.915)) ;
#114673=CARTESIAN_POINT('',(0.600000000000001,-2.1,-32.915)) ;
#114674=CARTESIAN_POINT('',(0.500000000000001,-2.9,-32.915)) ;
#114675=CARTESIAN_POINT('',(0.5,1.25,-32.915)) ;
#114676=CARTESIAN_POINT('',(-1.1,-2.9,-32.915)) ;
#114677=CARTESIAN_POINT('',(-1.1,-2.9,-32.915)) ;
#114678=CARTESIAN_POINT('',(-1.1,1.25,-32.915)) ;
#114679=CARTESIAN_POINT('Origin',(-0.999999999999999,1.25,-31.855)) ;
#114680=CARTESIAN_POINT('',(-1.1,-1.9,-31.855)) ;
#114681=CARTESIAN_POINT('',(-0.899999999999999,-2.1,-31.855)) ;
#114682=CARTESIAN_POINT('Origin',(-0.899999999999999,-1.9,-31.855)) ;
#114683=CARTESIAN_POINT('',(-1.1,-2.9,-31.855)) ;
#114684=CARTESIAN_POINT('',(-1.1,-2.9,-31.855)) ;
#114685=CARTESIAN_POINT('',(0.500000000000001,-2.9,-31.855)) ;
#114686=CARTESIAN_POINT('',(0.600000000000001,-2.9,-31.855)) ;
#114687=CARTESIAN_POINT('',(0.500000000000001,-2.1,-31.855)) ;
#114688=CARTESIAN_POINT('',(0.5,1.25,-31.855)) ;
#114689=CARTESIAN_POINT('',(-0.999999999999999,-2.1,-31.855)) ;
#114690=CARTESIAN_POINT('Origin',(-0.999999999999999,1.25,-29.105)) ;
#114691=CARTESIAN_POINT('',(-0.899999999999999,-2.1,-29.105)) ;
#114692=CARTESIAN_POINT('',(-1.1,-1.9,-29.105)) ;
#114693=CARTESIAN_POINT('Origin',(-0.899999999999999,-1.9,-29.105)) ;
#114694=CARTESIAN_POINT('',(0.500000000000001,-2.1,-29.105)) ;
#114695=CARTESIAN_POINT('',(0.600000000000001,-2.1,-29.105)) ;
#114696=CARTESIAN_POINT('',(0.500000000000001,-2.9,-29.105)) ;
#114697=CARTESIAN_POINT('',(0.5,1.25,-29.105)) ;
#114698=CARTESIAN_POINT('',(-1.1,-2.9,-29.105)) ;
#114699=CARTESIAN_POINT('',(-1.1,-2.9,-29.105)) ;
#114700=CARTESIAN_POINT('',(-1.1,1.25,-29.105)) ;
#114701=CARTESIAN_POINT('Origin',(-0.999999999999999,1.25,-28.045)) ;
#114702=CARTESIAN_POINT('',(-1.1,-1.9,-28.045)) ;
#114703=CARTESIAN_POINT('',(-0.899999999999999,-2.1,-28.045)) ;
#114704=CARTESIAN_POINT('Origin',(-0.899999999999999,-1.9,-28.045)) ;
#114705=CARTESIAN_POINT('',(-1.1,-2.9,-28.045)) ;
#114706=CARTESIAN_POINT('',(-1.1,-2.9,-28.045)) ;
#114707=CARTESIAN_POINT('',(0.500000000000001,-2.9,-28.045)) ;
#114708=CARTESIAN_POINT('',(0.600000000000001,-2.9,-28.045)) ;
#114709=CARTESIAN_POINT('',(0.500000000000001,-2.1,-28.045)) ;
#114710=CARTESIAN_POINT('',(0.5,1.25,-28.045)) ;
#114711=CARTESIAN_POINT('',(-0.999999999999999,-2.1,-28.045)) ;
#114712=CARTESIAN_POINT('Origin',(-0.999999999999999,1.25,-25.295)) ;
#114713=CARTESIAN_POINT('',(-0.899999999999999,-2.1,-25.295)) ;
#114714=CARTESIAN_POINT('',(-1.1,-1.9,-25.295)) ;
#114715=CARTESIAN_POINT('Origin',(-0.899999999999999,-1.9,-25.295)) ;
#114716=CARTESIAN_POINT('',(0.500000000000001,-2.1,-25.295)) ;
#114717=CARTESIAN_POINT('',(0.600000000000001,-2.1,-25.295)) ;
#114718=CARTESIAN_POINT('',(0.500000000000001,-2.9,-25.295)) ;
#114719=CARTESIAN_POINT('',(0.5,1.25,-25.295)) ;
#114720=CARTESIAN_POINT('',(-1.1,-2.9,-25.295)) ;
#114721=CARTESIAN_POINT('',(-1.1,-2.9,-25.295)) ;
#114722=CARTESIAN_POINT('',(-1.1,1.25,-25.295)) ;
#114723=CARTESIAN_POINT('Origin',(-0.999999999999999,1.25,-24.235)) ;
#114724=CARTESIAN_POINT('',(-1.1,-1.9,-24.235)) ;
#114725=CARTESIAN_POINT('',(-0.899999999999999,-2.1,-24.235)) ;
#114726=CARTESIAN_POINT('Origin',(-0.899999999999999,-1.9,-24.235)) ;
#114727=CARTESIAN_POINT('',(-1.1,-2.9,-24.235)) ;
#114728=CARTESIAN_POINT('',(-1.1,-2.9,-24.235)) ;
#114729=CARTESIAN_POINT('',(0.500000000000001,-2.9,-24.235)) ;
#114730=CARTESIAN_POINT('',(0.600000000000001,-2.9,-24.235)) ;
#114731=CARTESIAN_POINT('',(0.500000000000001,-2.1,-24.235)) ;
#114732=CARTESIAN_POINT('',(0.5,1.25,-24.235)) ;
#114733=CARTESIAN_POINT('',(-0.999999999999999,-2.1,-24.235)) ;
#114734=CARTESIAN_POINT('Origin',(-0.999999999999999,1.25,-21.485)) ;
#114735=CARTESIAN_POINT('',(-0.899999999999999,-2.1,-21.485)) ;
#114736=CARTESIAN_POINT('',(-1.1,-1.9,-21.485)) ;
#114737=CARTESIAN_POINT('Origin',(-0.899999999999999,-1.9,-21.485)) ;
#114738=CARTESIAN_POINT('',(0.500000000000001,-2.1,-21.485)) ;
#114739=CARTESIAN_POINT('',(0.600000000000001,-2.1,-21.485)) ;
#114740=CARTESIAN_POINT('',(0.500000000000001,-2.9,-21.485)) ;
#114741=CARTESIAN_POINT('',(0.5,1.25,-21.485)) ;
#114742=CARTESIAN_POINT('',(-1.1,-2.9,-21.485)) ;
#114743=CARTESIAN_POINT('',(-1.1,-2.9,-21.485)) ;
#114744=CARTESIAN_POINT('',(-1.1,1.25,-21.485)) ;
#114745=CARTESIAN_POINT('Origin',(-0.999999999999999,1.25,-20.425)) ;
#114746=CARTESIAN_POINT('',(-1.1,-1.9,-20.425)) ;
#114747=CARTESIAN_POINT('',(-0.899999999999999,-2.1,-20.425)) ;
#114748=CARTESIAN_POINT('Origin',(-0.899999999999999,-1.9,-20.425)) ;
#114749=CARTESIAN_POINT('',(-1.1,-2.9,-20.425)) ;
#114750=CARTESIAN_POINT('',(-1.1,-2.9,-20.425)) ;
#114751=CARTESIAN_POINT('',(0.500000000000001,-2.9,-20.425)) ;
#114752=CARTESIAN_POINT('',(0.600000000000001,-2.9,-20.425)) ;
#114753=CARTESIAN_POINT('',(0.500000000000001,-2.1,-20.425)) ;
#114754=CARTESIAN_POINT('',(0.5,1.25,-20.425)) ;
#114755=CARTESIAN_POINT('',(-0.999999999999999,-2.1,-20.425)) ;
#114756=CARTESIAN_POINT('Origin',(-0.999999999999999,1.25,-17.675)) ;
#114757=CARTESIAN_POINT('',(-0.899999999999999,-2.1,-17.675)) ;
#114758=CARTESIAN_POINT('',(-1.1,-1.9,-17.675)) ;
#114759=CARTESIAN_POINT('Origin',(-0.899999999999999,-1.9,-17.675)) ;
#114760=CARTESIAN_POINT('',(0.500000000000001,-2.1,-17.675)) ;
#114761=CARTESIAN_POINT('',(0.600000000000001,-2.1,-17.675)) ;
#114762=CARTESIAN_POINT('',(0.500000000000001,-2.9,-17.675)) ;
#114763=CARTESIAN_POINT('',(0.5,1.25,-17.675)) ;
#114764=CARTESIAN_POINT('',(-1.1,-2.9,-17.675)) ;
#114765=CARTESIAN_POINT('',(-1.1,-2.9,-17.675)) ;
#114766=CARTESIAN_POINT('',(-1.1,1.25,-17.675)) ;
#114767=CARTESIAN_POINT('Origin',(-0.999999999999999,1.25,-16.615)) ;
#114768=CARTESIAN_POINT('',(-1.1,-1.9,-16.615)) ;
#114769=CARTESIAN_POINT('',(-0.899999999999999,-2.1,-16.615)) ;
#114770=CARTESIAN_POINT('Origin',(-0.899999999999999,-1.9,-16.615)) ;
#114771=CARTESIAN_POINT('',(-1.1,-2.9,-16.615)) ;
#114772=CARTESIAN_POINT('',(-1.1,-2.9,-16.615)) ;
#114773=CARTESIAN_POINT('',(0.500000000000001,-2.9,-16.615)) ;
#114774=CARTESIAN_POINT('',(0.600000000000001,-2.9,-16.615)) ;
#114775=CARTESIAN_POINT('',(0.500000000000001,-2.1,-16.615)) ;
#114776=CARTESIAN_POINT('',(0.5,1.25,-16.615)) ;
#114777=CARTESIAN_POINT('',(-0.999999999999999,-2.1,-16.615)) ;
#114778=CARTESIAN_POINT('Origin',(-0.999999999999999,1.25,-13.865)) ;
#114779=CARTESIAN_POINT('',(-0.899999999999999,-2.1,-13.865)) ;
#114780=CARTESIAN_POINT('',(-1.1,-1.9,-13.865)) ;
#114781=CARTESIAN_POINT('Origin',(-0.899999999999999,-1.9,-13.865)) ;
#114782=CARTESIAN_POINT('',(0.500000000000001,-2.1,-13.865)) ;
#114783=CARTESIAN_POINT('',(0.600000000000001,-2.1,-13.865)) ;
#114784=CARTESIAN_POINT('',(0.500000000000001,-2.9,-13.865)) ;
#114785=CARTESIAN_POINT('',(0.5,1.25,-13.865)) ;
#114786=CARTESIAN_POINT('',(-1.1,-2.9,-13.865)) ;
#114787=CARTESIAN_POINT('',(-1.1,-2.9,-13.865)) ;
#114788=CARTESIAN_POINT('',(-1.1,1.25,-13.865)) ;
#114789=CARTESIAN_POINT('Origin',(-0.999999999999999,1.25,-12.805)) ;
#114790=CARTESIAN_POINT('',(-1.1,-1.9,-12.805)) ;
#114791=CARTESIAN_POINT('',(-0.899999999999999,-2.1,-12.805)) ;
#114792=CARTESIAN_POINT('Origin',(-0.899999999999999,-1.9,-12.805)) ;
#114793=CARTESIAN_POINT('',(-1.1,-2.9,-12.805)) ;
#114794=CARTESIAN_POINT('',(-1.1,-2.9,-12.805)) ;
#114795=CARTESIAN_POINT('',(0.500000000000001,-2.9,-12.805)) ;
#114796=CARTESIAN_POINT('',(0.600000000000001,-2.9,-12.805)) ;
#114797=CARTESIAN_POINT('',(0.500000000000001,-2.1,-12.805)) ;
#114798=CARTESIAN_POINT('',(0.5,1.25,-12.805)) ;
#114799=CARTESIAN_POINT('',(-0.999999999999999,-2.1,-12.805)) ;
#114800=CARTESIAN_POINT('Origin',(-0.999999999999999,1.25,-10.055)) ;
#114801=CARTESIAN_POINT('',(-0.899999999999999,-2.1,-10.055)) ;
#114802=CARTESIAN_POINT('',(-1.1,-1.9,-10.055)) ;
#114803=CARTESIAN_POINT('Origin',(-0.899999999999999,-1.9,-10.055)) ;
#114804=CARTESIAN_POINT('',(0.500000000000001,-2.1,-10.055)) ;
#114805=CARTESIAN_POINT('',(0.600000000000001,-2.1,-10.055)) ;
#114806=CARTESIAN_POINT('',(0.500000000000001,-2.9,-10.055)) ;
#114807=CARTESIAN_POINT('',(0.5,1.25,-10.055)) ;
#114808=CARTESIAN_POINT('',(-1.1,-2.9,-10.055)) ;
#114809=CARTESIAN_POINT('',(-1.1,-2.9,-10.055)) ;
#114810=CARTESIAN_POINT('',(-1.1,1.25,-10.055)) ;
#114811=CARTESIAN_POINT('Origin',(-0.999999999999999,1.25,-8.995)) ;
#114812=CARTESIAN_POINT('',(-1.1,-1.9,-8.995)) ;
#114813=CARTESIAN_POINT('',(-0.899999999999999,-2.1,-8.995)) ;
#114814=CARTESIAN_POINT('Origin',(-0.899999999999999,-1.9,-8.995)) ;
#114815=CARTESIAN_POINT('',(-1.1,-2.9,-8.995)) ;
#114816=CARTESIAN_POINT('',(-1.1,-2.9,-8.995)) ;
#114817=CARTESIAN_POINT('',(0.500000000000001,-2.9,-8.995)) ;
#114818=CARTESIAN_POINT('',(0.600000000000001,-2.9,-8.995)) ;
#114819=CARTESIAN_POINT('',(0.500000000000001,-2.1,-8.995)) ;
#114820=CARTESIAN_POINT('',(0.5,1.25,-8.995)) ;
#114821=CARTESIAN_POINT('',(-0.999999999999999,-2.1,-8.995)) ;
#114822=CARTESIAN_POINT('Origin',(-0.999999999999999,1.25,-6.245)) ;
#114823=CARTESIAN_POINT('',(-0.899999999999999,-2.1,-6.245)) ;
#114824=CARTESIAN_POINT('',(-1.1,-1.9,-6.245)) ;
#114825=CARTESIAN_POINT('Origin',(-0.899999999999999,-1.9,-6.245)) ;
#114826=CARTESIAN_POINT('',(0.500000000000001,-2.1,-6.245)) ;
#114827=CARTESIAN_POINT('',(0.600000000000001,-2.1,-6.245)) ;
#114828=CARTESIAN_POINT('',(0.500000000000001,-2.9,-6.245)) ;
#114829=CARTESIAN_POINT('',(0.5,1.25,-6.245)) ;
#114830=CARTESIAN_POINT('',(-1.1,-2.9,-6.245)) ;
#114831=CARTESIAN_POINT('',(-1.1,-2.9,-6.245)) ;
#114832=CARTESIAN_POINT('',(-1.1,1.25,-6.245)) ;
#114833=CARTESIAN_POINT('Origin',(-0.999999999999999,1.25,-5.185)) ;
#114834=CARTESIAN_POINT('',(-1.1,-1.9,-5.185)) ;
#114835=CARTESIAN_POINT('',(-0.899999999999999,-2.1,-5.185)) ;
#114836=CARTESIAN_POINT('Origin',(-0.899999999999999,-1.9,-5.185)) ;
#114837=CARTESIAN_POINT('',(-1.1,-2.9,-5.185)) ;
#114838=CARTESIAN_POINT('',(-1.1,-2.9,-5.185)) ;
#114839=CARTESIAN_POINT('',(0.500000000000001,-2.9,-5.185)) ;
#114840=CARTESIAN_POINT('',(0.600000000000001,-2.9,-5.185)) ;
#114841=CARTESIAN_POINT('',(0.500000000000001,-2.1,-5.185)) ;
#114842=CARTESIAN_POINT('',(0.5,1.25,-5.185)) ;
#114843=CARTESIAN_POINT('',(-0.999999999999999,-2.1,-5.185)) ;
#114844=CARTESIAN_POINT('Origin',(-0.999999999999999,1.25,-2.435)) ;
#114845=CARTESIAN_POINT('',(-0.899999999999999,-2.1,-2.435)) ;
#114846=CARTESIAN_POINT('',(-1.1,-1.9,-2.435)) ;
#114847=CARTESIAN_POINT('Origin',(-0.899999999999999,-1.9,-2.435)) ;
#114848=CARTESIAN_POINT('',(0.500000000000001,-2.1,-2.435)) ;
#114849=CARTESIAN_POINT('',(0.600000000000001,-2.1,-2.435)) ;
#114850=CARTESIAN_POINT('',(0.500000000000001,-2.9,-2.435)) ;
#114851=CARTESIAN_POINT('',(0.5,1.25,-2.435)) ;
#114852=CARTESIAN_POINT('',(-1.1,-2.9,-2.435)) ;
#114853=CARTESIAN_POINT('',(-1.1,-2.9,-2.435)) ;
#114854=CARTESIAN_POINT('',(-1.1,1.25,-2.435)) ;
#114855=CARTESIAN_POINT('Origin',(-1.1,-2.9,-36.89)) ;
#114856=CARTESIAN_POINT('',(-1.2,-2.9,-2.335)) ;
#114857=CARTESIAN_POINT('',(-1.2,-2.9,-1.475)) ;
#114858=CARTESIAN_POINT('',(-1.2,-2.9,-36.89)) ;
#114859=CARTESIAN_POINT('',(-1.1,-3.,-2.335)) ;
#114860=CARTESIAN_POINT('Origin',(-1.1,-2.9,-2.335)) ;
#114861=CARTESIAN_POINT('',(-1.1,-3.,-1.475)) ;
#114862=CARTESIAN_POINT('',(-1.1,-3.,-36.89)) ;
#114863=CARTESIAN_POINT('Origin',(-1.1,-2.9,-1.475)) ;
#114864=CARTESIAN_POINT('Origin',(-1.1,-2.9,-36.89)) ;
#114865=CARTESIAN_POINT('',(-1.2,-2.9,-6.145)) ;
#114866=CARTESIAN_POINT('',(-1.2,-2.9,-5.285)) ;
#114867=CARTESIAN_POINT('',(-1.2,-2.9,-36.89)) ;
#114868=CARTESIAN_POINT('',(-1.1,-3.,-6.145)) ;
#114869=CARTESIAN_POINT('Origin',(-1.1,-2.9,-6.145)) ;
#114870=CARTESIAN_POINT('',(-1.1,-3.,-5.285)) ;
#114871=CARTESIAN_POINT('',(-1.1,-3.,-36.89)) ;
#114872=CARTESIAN_POINT('Origin',(-1.1,-2.9,-5.285)) ;
#114873=CARTESIAN_POINT('Origin',(-1.1,-2.9,-36.89)) ;
#114874=CARTESIAN_POINT('',(-1.2,-2.9,-9.955)) ;
#114875=CARTESIAN_POINT('',(-1.2,-2.9,-9.095)) ;
#114876=CARTESIAN_POINT('',(-1.2,-2.9,-36.89)) ;
#114877=CARTESIAN_POINT('',(-1.1,-3.,-9.955)) ;
#114878=CARTESIAN_POINT('Origin',(-1.1,-2.9,-9.955)) ;
#114879=CARTESIAN_POINT('',(-1.1,-3.,-9.095)) ;
#114880=CARTESIAN_POINT('',(-1.1,-3.,-36.89)) ;
#114881=CARTESIAN_POINT('Origin',(-1.1,-2.9,-9.095)) ;
#114882=CARTESIAN_POINT('Origin',(-1.1,-2.9,-36.89)) ;
#114883=CARTESIAN_POINT('',(-1.2,-2.9,-13.765)) ;
#114884=CARTESIAN_POINT('',(-1.2,-2.9,-12.905)) ;
#114885=CARTESIAN_POINT('',(-1.2,-2.9,-36.89)) ;
#114886=CARTESIAN_POINT('',(-1.1,-3.,-13.765)) ;
#114887=CARTESIAN_POINT('Origin',(-1.1,-2.9,-13.765)) ;
#114888=CARTESIAN_POINT('',(-1.1,-3.,-12.905)) ;
#114889=CARTESIAN_POINT('',(-1.1,-3.,-36.89)) ;
#114890=CARTESIAN_POINT('Origin',(-1.1,-2.9,-12.905)) ;
#114891=CARTESIAN_POINT('Origin',(-1.1,-2.9,-36.89)) ;
#114892=CARTESIAN_POINT('',(-1.2,-2.9,-17.575)) ;
#114893=CARTESIAN_POINT('',(-1.2,-2.9,-16.715)) ;
#114894=CARTESIAN_POINT('',(-1.2,-2.9,-36.89)) ;
#114895=CARTESIAN_POINT('',(-1.1,-3.,-17.575)) ;
#114896=CARTESIAN_POINT('Origin',(-1.1,-2.9,-17.575)) ;
#114897=CARTESIAN_POINT('',(-1.1,-3.,-16.715)) ;
#114898=CARTESIAN_POINT('',(-1.1,-3.,-36.89)) ;
#114899=CARTESIAN_POINT('Origin',(-1.1,-2.9,-16.715)) ;
#114900=CARTESIAN_POINT('Origin',(-1.1,-2.9,-36.89)) ;
#114901=CARTESIAN_POINT('',(-1.2,-2.9,-21.385)) ;
#114902=CARTESIAN_POINT('',(-1.2,-2.9,-20.525)) ;
#114903=CARTESIAN_POINT('',(-1.2,-2.9,-36.89)) ;
#114904=CARTESIAN_POINT('',(-1.1,-3.,-21.385)) ;
#114905=CARTESIAN_POINT('Origin',(-1.1,-2.9,-21.385)) ;
#114906=CARTESIAN_POINT('',(-1.1,-3.,-20.525)) ;
#114907=CARTESIAN_POINT('',(-1.1,-3.,-36.89)) ;
#114908=CARTESIAN_POINT('Origin',(-1.1,-2.9,-20.525)) ;
#114909=CARTESIAN_POINT('Origin',(-1.1,-2.9,-36.89)) ;
#114910=CARTESIAN_POINT('',(-1.2,-2.9,-25.195)) ;
#114911=CARTESIAN_POINT('',(-1.2,-2.9,-24.335)) ;
#114912=CARTESIAN_POINT('',(-1.2,-2.9,-36.89)) ;
#114913=CARTESIAN_POINT('',(-1.1,-3.,-25.195)) ;
#114914=CARTESIAN_POINT('Origin',(-1.1,-2.9,-25.195)) ;
#114915=CARTESIAN_POINT('',(-1.1,-3.,-24.335)) ;
#114916=CARTESIAN_POINT('',(-1.1,-3.,-36.89)) ;
#114917=CARTESIAN_POINT('Origin',(-1.1,-2.9,-24.335)) ;
#114918=CARTESIAN_POINT('Origin',(-1.1,-2.9,-36.89)) ;
#114919=CARTESIAN_POINT('',(-1.2,-2.9,-29.005)) ;
#114920=CARTESIAN_POINT('',(-1.2,-2.9,-28.145)) ;
#114921=CARTESIAN_POINT('',(-1.2,-2.9,-36.89)) ;
#114922=CARTESIAN_POINT('',(-1.1,-3.,-29.005)) ;
#114923=CARTESIAN_POINT('Origin',(-1.1,-2.9,-29.005)) ;
#114924=CARTESIAN_POINT('',(-1.1,-3.,-28.145)) ;
#114925=CARTESIAN_POINT('',(-1.1,-3.,-36.89)) ;
#114926=CARTESIAN_POINT('Origin',(-1.1,-2.9,-28.145)) ;
#114927=CARTESIAN_POINT('Origin',(-1.1,-2.9,-36.89)) ;
#114928=CARTESIAN_POINT('',(-1.2,-2.9,-32.815)) ;
#114929=CARTESIAN_POINT('',(-1.2,-2.9,-31.955)) ;
#114930=CARTESIAN_POINT('',(-1.2,-2.9,-36.89)) ;
#114931=CARTESIAN_POINT('',(-1.1,-3.,-32.815)) ;
#114932=CARTESIAN_POINT('Origin',(-1.1,-2.9,-32.815)) ;
#114933=CARTESIAN_POINT('',(-1.1,-3.,-31.955)) ;
#114934=CARTESIAN_POINT('',(-1.1,-3.,-36.89)) ;
#114935=CARTESIAN_POINT('Origin',(-1.1,-2.9,-31.955)) ;
#114936=CARTESIAN_POINT('Origin',(0.600000000000001,2.80617032878603E-17,
0.)) ;
#114937=CARTESIAN_POINT('',(0.600000000000001,-1.9,0.4)) ;
#114938=CARTESIAN_POINT('',(0.600000000000001,-0.3,0.4)) ;
#114939=CARTESIAN_POINT('',(0.600000000000001,-2.3980000991444E-17,0.4)) ;
#114940=CARTESIAN_POINT('',(0.6,-0.4,0.3)) ;
#114941=CARTESIAN_POINT('Origin',(0.6,-0.3,0.3)) ;
#114942=CARTESIAN_POINT('',(0.6,-0.4,-0.3)) ;
#114943=CARTESIAN_POINT('',(0.6,-0.4,0.4)) ;
#114944=CARTESIAN_POINT('Origin',(0.6,-0.3,-0.3)) ;
#114945=CARTESIAN_POINT('',(0.600000000000001,-2.1,-0.6)) ;
#114946=CARTESIAN_POINT('Origin',(0.600000000000001,-1.9,-0.6)) ;
#114947=CARTESIAN_POINT('',(0.600000000000001,-2.1,-1.275)) ;
#114948=CARTESIAN_POINT('',(0.600000000000001,-2.1,0.)) ;
#114949=CARTESIAN_POINT('',(0.600000000000001,-2.9,-1.275)) ;
#114950=CARTESIAN_POINT('',(0.600000000000001,-3.699042706127E-17,-1.275)) ;
#114951=CARTESIAN_POINT('',(0.600000000000001,-2.9,1.275)) ;
#114952=CARTESIAN_POINT('',(0.600000000000001,-2.9,0.)) ;
#114953=CARTESIAN_POINT('',(0.600000000000001,-2.1,1.275)) ;
#114954=CARTESIAN_POINT('',(0.600000000000001,1.58165963986121E-16,1.275)) ;
#114955=CARTESIAN_POINT('',(0.600000000000001,-2.1,0.6)) ;
#114956=CARTESIAN_POINT('',(0.600000000000001,-2.1,0.)) ;
#114957=CARTESIAN_POINT('Origin',(0.600000000000001,-1.9,0.6)) ;
#114958=CARTESIAN_POINT('Origin',(-0.999999999999999,1.25,-1.375)) ;
#114959=CARTESIAN_POINT('',(-1.1,-1.9,-1.375)) ;
#114960=CARTESIAN_POINT('',(-0.899999999999999,-2.1,-1.375)) ;
#114961=CARTESIAN_POINT('Origin',(-0.899999999999999,-1.9,-1.375)) ;
#114962=CARTESIAN_POINT('',(-1.1,-2.9,-1.375)) ;
#114963=CARTESIAN_POINT('',(-1.1,-2.9,-1.375)) ;
#114964=CARTESIAN_POINT('',(0.500000000000001,-2.9,-1.375)) ;
#114965=CARTESIAN_POINT('',(0.600000000000001,-2.9,-1.375)) ;
#114966=CARTESIAN_POINT('',(0.500000000000001,-2.1,-1.375)) ;
#114967=CARTESIAN_POINT('',(0.5,1.25,-1.375)) ;
#114968=CARTESIAN_POINT('',(-0.999999999999999,-2.1,-1.375)) ;
#114969=CARTESIAN_POINT('Origin',(-0.999999999999999,1.25,1.375)) ;
#114970=CARTESIAN_POINT('',(-0.899999999999999,-2.1,1.375)) ;
#114971=CARTESIAN_POINT('',(-1.1,-1.9,1.375)) ;
#114972=CARTESIAN_POINT('Origin',(-0.899999999999999,-1.9,1.375)) ;
#114973=CARTESIAN_POINT('',(0.500000000000001,-2.1,1.375)) ;
#114974=CARTESIAN_POINT('',(0.600000000000001,-2.1,1.375)) ;
#114975=CARTESIAN_POINT('',(0.500000000000001,-2.9,1.375)) ;
#114976=CARTESIAN_POINT('',(0.5,1.25,1.375)) ;
#114977=CARTESIAN_POINT('',(-1.1,-2.9,1.375)) ;
#114978=CARTESIAN_POINT('',(-1.1,-2.9,1.375)) ;
#114979=CARTESIAN_POINT('',(-1.1,1.25,1.375)) ;
#114980=CARTESIAN_POINT('Origin',(-1.1,-2.9,-36.89)) ;
#114981=CARTESIAN_POINT('',(-1.2,-2.9,1.475)) ;
#114982=CARTESIAN_POINT('',(-1.2,-2.9,2.5)) ;
#114983=CARTESIAN_POINT('',(-1.2,-2.9,-36.89)) ;
#114984=CARTESIAN_POINT('',(-1.1,-3.,1.475)) ;
#114985=CARTESIAN_POINT('Origin',(-1.1,-2.9,1.475)) ;
#114986=CARTESIAN_POINT('',(-1.1,-3.,2.5)) ;
#114987=CARTESIAN_POINT('',(-1.1,-3.,-36.89)) ;
#114988=CARTESIAN_POINT('Origin',(-1.1,-2.9,2.5)) ;
#114989=CARTESIAN_POINT('Origin',(7.9,-2.9,-36.89)) ;
#114990=CARTESIAN_POINT('',(7.9,-3.,-36.79)) ;
#114991=CARTESIAN_POINT('',(7.9,-3.,2.5)) ;
#114992=CARTESIAN_POINT('',(7.9,-3.,-36.89)) ;
#114993=CARTESIAN_POINT('',(8.,-2.9,-36.79)) ;
#114994=CARTESIAN_POINT('Origin',(7.9,-2.9,-36.79)) ;
#114995=CARTESIAN_POINT('',(8.,-2.9,2.5)) ;
#114996=CARTESIAN_POINT('',(8.,-2.9,-36.89)) ;
#114997=CARTESIAN_POINT('Origin',(7.9,-2.9,2.5)) ;
#114998=CARTESIAN_POINT('Origin',(-1.1,-3.,-36.89)) ;
#114999=CARTESIAN_POINT('',(0.500000000000001,-3.,-35.765)) ;
#115000=CARTESIAN_POINT('',(0.700000000000002,-3.,-35.565)) ;
#115001=CARTESIAN_POINT('Origin',(0.500000000000001,-3.,-35.565)) ;
#115002=CARTESIAN_POINT('',(-1.1,-3.,-35.765)) ;
#115003=CARTESIAN_POINT('',(-1.1,-3.,-35.765)) ;
#115004=CARTESIAN_POINT('',(-1.1,-3.,-36.79)) ;
#115005=CARTESIAN_POINT('',(-1.1,-3.,-36.89)) ;
#115006=CARTESIAN_POINT('',(7.9,-3.,-36.79)) ;
#115007=CARTESIAN_POINT('',(-1.1,-3.,2.5)) ;
#115008=CARTESIAN_POINT('',(0.500000000000001,-3.,1.475)) ;
#115009=CARTESIAN_POINT('',(0.600000000000001,-3.,1.475)) ;
#115010=CARTESIAN_POINT('',(0.700000000000002,-3.,1.275)) ;
#115011=CARTESIAN_POINT('Origin',(0.500000000000001,-3.,1.275)) ;
#115012=CARTESIAN_POINT('',(0.700000000000002,-3.,-1.275)) ;
#115013=CARTESIAN_POINT('',(0.700000000000002,-3.,-36.89)) ;
#115014=CARTESIAN_POINT('',(0.500000000000001,-3.,-1.475)) ;
#115015=CARTESIAN_POINT('Origin',(0.500000000000001,-3.,-1.275)) ;
#115016=CARTESIAN_POINT('',(-1.1,-3.,-1.475)) ;
#115017=CARTESIAN_POINT('',(0.500000000000001,-3.,-2.335)) ;
#115018=CARTESIAN_POINT('',(0.600000000000001,-3.,-2.335)) ;
#115019=CARTESIAN_POINT('',(0.700000000000002,-3.,-2.535)) ;
#115020=CARTESIAN_POINT('Origin',(0.500000000000001,-3.,-2.535)) ;
#115021=CARTESIAN_POINT('',(0.700000000000002,-3.,-5.085)) ;
#115022=CARTESIAN_POINT('',(0.700000000000002,-3.,-36.89)) ;
#115023=CARTESIAN_POINT('',(0.500000000000001,-3.,-5.285)) ;
#115024=CARTESIAN_POINT('Origin',(0.500000000000001,-3.,-5.085)) ;
#115025=CARTESIAN_POINT('',(-1.1,-3.,-5.285)) ;
#115026=CARTESIAN_POINT('',(0.500000000000001,-3.,-6.145)) ;
#115027=CARTESIAN_POINT('',(0.600000000000001,-3.,-6.145)) ;
#115028=CARTESIAN_POINT('',(0.700000000000002,-3.,-6.345)) ;
#115029=CARTESIAN_POINT('Origin',(0.500000000000001,-3.,-6.345)) ;
#115030=CARTESIAN_POINT('',(0.700000000000002,-3.,-8.895)) ;
#115031=CARTESIAN_POINT('',(0.700000000000002,-3.,-36.89)) ;
#115032=CARTESIAN_POINT('',(0.500000000000001,-3.,-9.095)) ;
#115033=CARTESIAN_POINT('Origin',(0.500000000000001,-3.,-8.895)) ;
#115034=CARTESIAN_POINT('',(-1.1,-3.,-9.095)) ;
#115035=CARTESIAN_POINT('',(0.500000000000001,-3.,-9.955)) ;
#115036=CARTESIAN_POINT('',(0.600000000000001,-3.,-9.955)) ;
#115037=CARTESIAN_POINT('',(0.700000000000002,-3.,-10.155)) ;
#115038=CARTESIAN_POINT('Origin',(0.500000000000001,-3.,-10.155)) ;
#115039=CARTESIAN_POINT('',(0.700000000000002,-3.,-12.705)) ;
#115040=CARTESIAN_POINT('',(0.700000000000002,-3.,-36.89)) ;
#115041=CARTESIAN_POINT('',(0.500000000000001,-3.,-12.905)) ;
#115042=CARTESIAN_POINT('Origin',(0.500000000000001,-3.,-12.705)) ;
#115043=CARTESIAN_POINT('',(-1.1,-3.,-12.905)) ;
#115044=CARTESIAN_POINT('',(0.500000000000001,-3.,-13.765)) ;
#115045=CARTESIAN_POINT('',(0.600000000000001,-3.,-13.765)) ;
#115046=CARTESIAN_POINT('',(0.700000000000002,-3.,-13.965)) ;
#115047=CARTESIAN_POINT('Origin',(0.500000000000001,-3.,-13.965)) ;
#115048=CARTESIAN_POINT('',(0.700000000000002,-3.,-16.515)) ;
#115049=CARTESIAN_POINT('',(0.700000000000002,-3.,-36.89)) ;
#115050=CARTESIAN_POINT('',(0.500000000000001,-3.,-16.715)) ;
#115051=CARTESIAN_POINT('Origin',(0.500000000000001,-3.,-16.515)) ;
#115052=CARTESIAN_POINT('',(-1.1,-3.,-16.715)) ;
#115053=CARTESIAN_POINT('',(0.500000000000001,-3.,-17.575)) ;
#115054=CARTESIAN_POINT('',(0.600000000000001,-3.,-17.575)) ;
#115055=CARTESIAN_POINT('',(0.700000000000002,-3.,-17.775)) ;
#115056=CARTESIAN_POINT('Origin',(0.500000000000001,-3.,-17.775)) ;
#115057=CARTESIAN_POINT('',(0.700000000000002,-3.,-20.325)) ;
#115058=CARTESIAN_POINT('',(0.700000000000002,-3.,-36.89)) ;
#115059=CARTESIAN_POINT('',(0.500000000000001,-3.,-20.525)) ;
#115060=CARTESIAN_POINT('Origin',(0.500000000000001,-3.,-20.325)) ;
#115061=CARTESIAN_POINT('',(-1.1,-3.,-20.525)) ;
#115062=CARTESIAN_POINT('',(0.500000000000001,-3.,-21.385)) ;
#115063=CARTESIAN_POINT('',(0.600000000000001,-3.,-21.385)) ;
#115064=CARTESIAN_POINT('',(0.700000000000002,-3.,-21.585)) ;
#115065=CARTESIAN_POINT('Origin',(0.500000000000001,-3.,-21.585)) ;
#115066=CARTESIAN_POINT('',(0.700000000000002,-3.,-24.135)) ;
#115067=CARTESIAN_POINT('',(0.700000000000002,-3.,-36.89)) ;
#115068=CARTESIAN_POINT('',(0.500000000000001,-3.,-24.335)) ;
#115069=CARTESIAN_POINT('Origin',(0.500000000000001,-3.,-24.135)) ;
#115070=CARTESIAN_POINT('',(-1.1,-3.,-24.335)) ;
#115071=CARTESIAN_POINT('',(0.500000000000001,-3.,-25.195)) ;
#115072=CARTESIAN_POINT('',(0.600000000000001,-3.,-25.195)) ;
#115073=CARTESIAN_POINT('',(0.700000000000002,-3.,-25.395)) ;
#115074=CARTESIAN_POINT('Origin',(0.500000000000001,-3.,-25.395)) ;
#115075=CARTESIAN_POINT('',(0.700000000000002,-3.,-27.945)) ;
#115076=CARTESIAN_POINT('',(0.700000000000002,-3.,-36.89)) ;
#115077=CARTESIAN_POINT('',(0.500000000000001,-3.,-28.145)) ;
#115078=CARTESIAN_POINT('Origin',(0.500000000000001,-3.,-27.945)) ;
#115079=CARTESIAN_POINT('',(-1.1,-3.,-28.145)) ;
#115080=CARTESIAN_POINT('',(0.500000000000001,-3.,-29.005)) ;
#115081=CARTESIAN_POINT('',(0.600000000000001,-3.,-29.005)) ;
#115082=CARTESIAN_POINT('',(0.700000000000002,-3.,-29.205)) ;
#115083=CARTESIAN_POINT('Origin',(0.500000000000001,-3.,-29.205)) ;
#115084=CARTESIAN_POINT('',(0.700000000000002,-3.,-31.755)) ;
#115085=CARTESIAN_POINT('',(0.700000000000002,-3.,-36.89)) ;
#115086=CARTESIAN_POINT('',(0.500000000000001,-3.,-31.955)) ;
#115087=CARTESIAN_POINT('Origin',(0.500000000000001,-3.,-31.755)) ;
#115088=CARTESIAN_POINT('',(-1.1,-3.,-31.955)) ;
#115089=CARTESIAN_POINT('',(0.500000000000001,-3.,-32.815)) ;
#115090=CARTESIAN_POINT('',(0.600000000000001,-3.,-32.815)) ;
#115091=CARTESIAN_POINT('',(0.700000000000002,-3.,-33.015)) ;
#115092=CARTESIAN_POINT('Origin',(0.500000000000001,-3.,-33.015)) ;
#115093=CARTESIAN_POINT('',(0.700000000000002,-3.,-36.89)) ;
#115094=CARTESIAN_POINT('Origin',(-1.1,-2.9,-36.89)) ;
#115095=CARTESIAN_POINT('',(-1.2,-2.9,-35.765)) ;
#115096=CARTESIAN_POINT('Origin',(-1.1,-2.9,-35.765)) ;
#115097=CARTESIAN_POINT('',(-1.2,-2.9,-36.79)) ;
#115098=CARTESIAN_POINT('',(-1.2,-2.9,-36.89)) ;
#115099=CARTESIAN_POINT('Origin',(-1.1,-2.9,-36.79)) ;
#115100=CARTESIAN_POINT('Origin',(-1.2,4.15,-36.89)) ;
#115101=CARTESIAN_POINT('',(-1.2,1.15,-32.815)) ;
#115102=CARTESIAN_POINT('',(-1.2,1.35,-33.015)) ;
#115103=CARTESIAN_POINT('Origin',(-1.2,1.15,-33.015)) ;
#115104=CARTESIAN_POINT('',(-1.2,-2.9,-32.815)) ;
#115105=CARTESIAN_POINT('',(-1.2,1.15,-31.955)) ;
#115106=CARTESIAN_POINT('',(-1.2,1.25,-31.955)) ;
#115107=CARTESIAN_POINT('',(-1.2,1.35,-31.755)) ;
#115108=CARTESIAN_POINT('Origin',(-1.2,1.15,-31.755)) ;
#115109=CARTESIAN_POINT('',(-1.2,1.35,-29.205)) ;
#115110=CARTESIAN_POINT('',(-1.2,1.35,-29.105)) ;
#115111=CARTESIAN_POINT('',(-1.2,1.15,-29.005)) ;
#115112=CARTESIAN_POINT('Origin',(-1.2,1.15,-29.205)) ;
#115113=CARTESIAN_POINT('',(-1.2,-2.9,-29.005)) ;
#115114=CARTESIAN_POINT('',(-1.2,1.15,-28.145)) ;
#115115=CARTESIAN_POINT('',(-1.2,1.25,-28.145)) ;
#115116=CARTESIAN_POINT('',(-1.2,1.35,-27.945)) ;
#115117=CARTESIAN_POINT('Origin',(-1.2,1.15,-27.945)) ;
#115118=CARTESIAN_POINT('',(-1.2,1.35,-25.395)) ;
#115119=CARTESIAN_POINT('',(-1.2,1.35,-25.295)) ;
#115120=CARTESIAN_POINT('',(-1.2,1.15,-25.195)) ;
#115121=CARTESIAN_POINT('Origin',(-1.2,1.15,-25.395)) ;
#115122=CARTESIAN_POINT('',(-1.2,-2.9,-25.195)) ;
#115123=CARTESIAN_POINT('',(-1.2,1.15,-24.335)) ;
#115124=CARTESIAN_POINT('',(-1.2,1.25,-24.335)) ;
#115125=CARTESIAN_POINT('',(-1.2,1.35,-24.135)) ;
#115126=CARTESIAN_POINT('Origin',(-1.2,1.15,-24.135)) ;
#115127=CARTESIAN_POINT('',(-1.2,1.35,-21.585)) ;
#115128=CARTESIAN_POINT('',(-1.2,1.35,-21.485)) ;
#115129=CARTESIAN_POINT('',(-1.2,1.15,-21.385)) ;
#115130=CARTESIAN_POINT('Origin',(-1.2,1.15,-21.585)) ;
#115131=CARTESIAN_POINT('',(-1.2,-2.9,-21.385)) ;
#115132=CARTESIAN_POINT('',(-1.2,1.15,-20.525)) ;
#115133=CARTESIAN_POINT('',(-1.2,1.25,-20.525)) ;
#115134=CARTESIAN_POINT('',(-1.2,1.35,-20.325)) ;
#115135=CARTESIAN_POINT('Origin',(-1.2,1.15,-20.325)) ;
#115136=CARTESIAN_POINT('',(-1.2,1.35,-17.775)) ;
#115137=CARTESIAN_POINT('',(-1.2,1.35,-17.675)) ;
#115138=CARTESIAN_POINT('',(-1.2,1.15,-17.575)) ;
#115139=CARTESIAN_POINT('Origin',(-1.2,1.15,-17.775)) ;
#115140=CARTESIAN_POINT('',(-1.2,-2.9,-17.575)) ;
#115141=CARTESIAN_POINT('',(-1.2,1.15,-16.715)) ;
#115142=CARTESIAN_POINT('',(-1.2,1.25,-16.715)) ;
#115143=CARTESIAN_POINT('',(-1.2,1.35,-16.515)) ;
#115144=CARTESIAN_POINT('Origin',(-1.2,1.15,-16.515)) ;
#115145=CARTESIAN_POINT('',(-1.2,1.35,-13.965)) ;
#115146=CARTESIAN_POINT('',(-1.2,1.35,-13.865)) ;
#115147=CARTESIAN_POINT('',(-1.2,1.15,-13.765)) ;
#115148=CARTESIAN_POINT('Origin',(-1.2,1.15,-13.965)) ;
#115149=CARTESIAN_POINT('',(-1.2,-2.9,-13.765)) ;
#115150=CARTESIAN_POINT('',(-1.2,1.15,-12.905)) ;
#115151=CARTESIAN_POINT('',(-1.2,1.25,-12.905)) ;
#115152=CARTESIAN_POINT('',(-1.2,1.35,-12.705)) ;
#115153=CARTESIAN_POINT('Origin',(-1.2,1.15,-12.705)) ;
#115154=CARTESIAN_POINT('',(-1.2,1.35,-10.155)) ;
#115155=CARTESIAN_POINT('',(-1.2,1.35,-10.055)) ;
#115156=CARTESIAN_POINT('',(-1.2,1.15,-9.955)) ;
#115157=CARTESIAN_POINT('Origin',(-1.2,1.15,-10.155)) ;
#115158=CARTESIAN_POINT('',(-1.2,-2.9,-9.955)) ;
#115159=CARTESIAN_POINT('',(-1.2,1.15,-9.095)) ;
#115160=CARTESIAN_POINT('',(-1.2,1.25,-9.095)) ;
#115161=CARTESIAN_POINT('',(-1.2,1.35,-8.895)) ;
#115162=CARTESIAN_POINT('Origin',(-1.2,1.15,-8.895)) ;
#115163=CARTESIAN_POINT('',(-1.2,1.35,-6.345)) ;
#115164=CARTESIAN_POINT('',(-1.2,1.35,-6.245)) ;
#115165=CARTESIAN_POINT('',(-1.2,1.15,-6.145)) ;
#115166=CARTESIAN_POINT('Origin',(-1.2,1.15,-6.345)) ;
#115167=CARTESIAN_POINT('',(-1.2,-2.9,-6.145)) ;
#115168=CARTESIAN_POINT('',(-1.2,1.15,-5.285)) ;
#115169=CARTESIAN_POINT('',(-1.2,1.25,-5.285)) ;
#115170=CARTESIAN_POINT('',(-1.2,1.35,-5.085)) ;
#115171=CARTESIAN_POINT('Origin',(-1.2,1.15,-5.085)) ;
#115172=CARTESIAN_POINT('',(-1.2,1.35,-2.535)) ;
#115173=CARTESIAN_POINT('',(-1.2,1.35,-2.435)) ;
#115174=CARTESIAN_POINT('',(-1.2,1.15,-2.335)) ;
#115175=CARTESIAN_POINT('Origin',(-1.2,1.15,-2.535)) ;
#115176=CARTESIAN_POINT('',(-1.2,-2.9,-2.335)) ;
#115177=CARTESIAN_POINT('',(-1.2,1.15,-1.475)) ;
#115178=CARTESIAN_POINT('',(-1.2,1.25,-1.475)) ;
#115179=CARTESIAN_POINT('',(-1.2,1.35,-1.275)) ;
#115180=CARTESIAN_POINT('Origin',(-1.2,1.15,-1.275)) ;
#115181=CARTESIAN_POINT('',(-1.2,1.35,1.275)) ;
#115182=CARTESIAN_POINT('',(-1.2,1.35,1.37499999999999)) ;
#115183=CARTESIAN_POINT('',(-1.2,1.15,1.475)) ;
#115184=CARTESIAN_POINT('Origin',(-1.2,1.15,1.275)) ;
#115185=CARTESIAN_POINT('',(-1.2,-2.9,1.475)) ;
#115186=CARTESIAN_POINT('',(-1.2,4.15,2.5)) ;
#115187=CARTESIAN_POINT('',(-1.2,4.15,2.5)) ;
#115188=CARTESIAN_POINT('',(-1.2,4.15,-36.79)) ;
#115189=CARTESIAN_POINT('',(-1.2,4.15,-36.89)) ;
#115190=CARTESIAN_POINT('',(-1.2,-2.9,-36.79)) ;
#115191=CARTESIAN_POINT('',(-1.2,1.15,-35.765)) ;
#115192=CARTESIAN_POINT('',(-1.2,1.25,-35.765)) ;
#115193=CARTESIAN_POINT('',(-1.2,1.35,-35.565)) ;
#115194=CARTESIAN_POINT('Origin',(-1.2,1.15,-35.565)) ;
#115195=CARTESIAN_POINT('',(-1.2,1.35,-32.915)) ;
#115196=CARTESIAN_POINT('Origin',(-1.1,4.15,-36.89)) ;
#115197=CARTESIAN_POINT('',(-1.1,4.25,-36.79)) ;
#115198=CARTESIAN_POINT('',(-1.1,4.25,2.5)) ;
#115199=CARTESIAN_POINT('',(-1.1,4.25,-36.89)) ;
#115200=CARTESIAN_POINT('Origin',(-1.1,4.15,-36.79)) ;
#115201=CARTESIAN_POINT('Origin',(-1.1,4.15,2.5)) ;
#115202=CARTESIAN_POINT('Origin',(-1.1,4.25,-36.89)) ;
#115203=CARTESIAN_POINT('',(4.35,4.25,-36.79)) ;
#115204=CARTESIAN_POINT('',(4.35,4.25,2.5)) ;
#115205=CARTESIAN_POINT('',(4.35,4.25,-36.89)) ;
#115206=CARTESIAN_POINT('',(-1.1,4.25,-36.79)) ;
#115207=CARTESIAN_POINT('',(-1.1,4.25,2.5)) ;
#115208=CARTESIAN_POINT('Origin',(4.35,4.35,-36.89)) ;
#115209=CARTESIAN_POINT('',(4.45,4.35,-36.79)) ;
#115210=CARTESIAN_POINT('',(4.45,4.35,2.5)) ;
#115211=CARTESIAN_POINT('',(4.45,4.35,-36.89)) ;
#115212=CARTESIAN_POINT('Origin',(4.35,4.35,-36.79)) ;
#115213=CARTESIAN_POINT('Origin',(4.35,4.35,2.5)) ;
#115214=CARTESIAN_POINT('Origin',(4.45,4.55,-36.89)) ;
#115215=CARTESIAN_POINT('',(4.45,4.55,-36.79)) ;
#115216=CARTESIAN_POINT('',(4.45,4.55,2.5)) ;
#115217=CARTESIAN_POINT('',(4.45,4.55,-36.89)) ;
#115218=CARTESIAN_POINT('',(4.45,4.35,-36.79)) ;
#115219=CARTESIAN_POINT('',(4.45,4.55,2.5)) ;
#115220=CARTESIAN_POINT('Origin',(4.55,4.55,-36.89)) ;
#115221=CARTESIAN_POINT('',(4.55,4.65,-36.79)) ;
#115222=CARTESIAN_POINT('',(4.55,4.65,2.5)) ;
#115223=CARTESIAN_POINT('',(4.55,4.65,-36.89)) ;
#115224=CARTESIAN_POINT('Origin',(4.55,4.55,-36.79)) ;
#115225=CARTESIAN_POINT('Origin',(4.55,4.55,2.5)) ;
#115226=CARTESIAN_POINT('Origin',(4.75,4.65,-36.89)) ;
#115227=CARTESIAN_POINT('',(4.75,4.65,-36.79)) ;
#115228=CARTESIAN_POINT('',(4.75,4.65,2.5)) ;
#115229=CARTESIAN_POINT('',(4.75,4.65,-36.89)) ;
#115230=CARTESIAN_POINT('',(4.55,4.65,-36.79)) ;
#115231=CARTESIAN_POINT('',(4.75,4.65,2.5)) ;
#115232=CARTESIAN_POINT('Origin',(4.75,4.55,-36.89)) ;
#115233=CARTESIAN_POINT('',(4.85,4.55,-36.79)) ;
#115234=CARTESIAN_POINT('',(4.85,4.55,2.5)) ;
#115235=CARTESIAN_POINT('',(4.85,4.55,-36.89)) ;
#115236=CARTESIAN_POINT('Origin',(4.75,4.55,-36.79)) ;
#115237=CARTESIAN_POINT('Origin',(4.75,4.55,2.5)) ;
#115238=CARTESIAN_POINT('Origin',(4.85,4.35,-36.89)) ;
#115239=CARTESIAN_POINT('',(4.85,4.35,-36.79)) ;
#115240=CARTESIAN_POINT('',(4.85,4.35,2.5)) ;
#115241=CARTESIAN_POINT('',(4.85,4.35,-36.89)) ;
#115242=CARTESIAN_POINT('',(4.85,4.55,-36.79)) ;
#115243=CARTESIAN_POINT('',(4.85,4.35,2.5)) ;
#115244=CARTESIAN_POINT('Origin',(4.95,4.35,-36.89)) ;
#115245=CARTESIAN_POINT('',(4.95,4.25,-36.79)) ;
#115246=CARTESIAN_POINT('',(4.95,4.25,2.5)) ;
#115247=CARTESIAN_POINT('',(4.95,4.25,-36.89)) ;
#115248=CARTESIAN_POINT('Origin',(4.95,4.35,-36.79)) ;
#115249=CARTESIAN_POINT('Origin',(4.95,4.35,2.5)) ;
#115250=CARTESIAN_POINT('Origin',(4.95,4.25,-36.89)) ;
#115251=CARTESIAN_POINT('',(7.9,4.25,-36.79)) ;
#115252=CARTESIAN_POINT('',(7.9,4.25,2.5)) ;
#115253=CARTESIAN_POINT('',(7.9,4.25,-36.89)) ;
#115254=CARTESIAN_POINT('',(4.95,4.25,-36.79)) ;
#115255=CARTESIAN_POINT('',(4.95,4.25,2.5)) ;
#115256=CARTESIAN_POINT('Origin',(7.9,4.15,-36.89)) ;
#115257=CARTESIAN_POINT('',(8.,4.15,-36.79)) ;
#115258=CARTESIAN_POINT('',(8.,4.15,2.5)) ;
#115259=CARTESIAN_POINT('',(8.,4.15,-36.89)) ;
#115260=CARTESIAN_POINT('Origin',(7.9,4.15,-36.79)) ;
#115261=CARTESIAN_POINT('Origin',(7.9,4.15,2.5)) ;
#115262=CARTESIAN_POINT('Origin',(8.,4.15,-36.89)) ;
#115263=CARTESIAN_POINT('',(8.,4.15,-36.79)) ;
#115264=CARTESIAN_POINT('',(8.,4.15,2.5)) ;
#115265=CARTESIAN_POINT('',(8.,1.9,-32.54)) ;
#115266=CARTESIAN_POINT('',(8.,2.1,-32.74)) ;
#115267=CARTESIAN_POINT('Origin',(8.,1.9,-32.74)) ;
#115268=CARTESIAN_POINT('',(8.,2.1,-33.69)) ;
#115269=CARTESIAN_POINT('',(8.,2.1,-33.69)) ;
#115270=CARTESIAN_POINT('',(8.,2.4,-33.69)) ;
#115271=CARTESIAN_POINT('',(8.,2.4,-33.69)) ;
#115272=CARTESIAN_POINT('',(8.,2.4,-33.5814213562373)) ;
#115273=CARTESIAN_POINT('',(8.,2.4,-33.5814213562373)) ;
#115274=CARTESIAN_POINT('',(8.,2.45857864376269,-33.44)) ;
#115275=CARTESIAN_POINT('Origin',(8.,2.6,-33.5814213562373)) ;
#115276=CARTESIAN_POINT('',(8.,3.00857864376269,-32.89)) ;
#115277=CARTESIAN_POINT('',(8.,3.00857864376269,-32.89)) ;
#115278=CARTESIAN_POINT('',(8.,3.35,-33.0314213562373)) ;
#115279=CARTESIAN_POINT('Origin',(8.,3.15,-33.0314213562373)) ;
#115280=CARTESIAN_POINT('',(8.,3.35,-35.5485786437627)) ;
#115281=CARTESIAN_POINT('',(8.,2.45857864376269,-35.14)) ;
#115282=CARTESIAN_POINT('',(8.,2.45857864376269,-35.14)) ;
#115283=CARTESIAN_POINT('',(8.,2.4,-34.9985786437627)) ;
#115284=CARTESIAN_POINT('Origin',(8.,2.6,-34.9985786437627)) ;
#115285=CARTESIAN_POINT('',(8.,2.4,-34.89)) ;
#115286=CARTESIAN_POINT('',(8.,2.4,-34.89)) ;
#115287=CARTESIAN_POINT('',(8.,2.1,-34.89)) ;
#115288=CARTESIAN_POINT('',(8.,2.1,-34.89)) ;
#115289=CARTESIAN_POINT('',(8.,2.1,-35.84)) ;
#115290=CARTESIAN_POINT('',(8.,2.1,-35.84)) ;
#115291=CARTESIAN_POINT('',(8.,1.9,-36.04)) ;
#115292=CARTESIAN_POINT('Origin',(8.,1.9,-35.84)) ;
#115293=CARTESIAN_POINT('',(8.,-2.15,-36.04)) ;
#115294=CARTESIAN_POINT('',(8.,-2.15,-36.04)) ;
#115295=CARTESIAN_POINT('',(8.,-2.35,-35.84)) ;
#115296=CARTESIAN_POINT('Origin',(8.,-2.15,-35.84)) ;
#115297=CARTESIAN_POINT('',(8.,-2.35,-35.1931195934094)) ;
#115298=CARTESIAN_POINT('',(8.,-2.35,-35.1931195934094)) ;
#115299=CARTESIAN_POINT('',(8.,-2.32153024911032,-35.0902732340176)) ;
#115300=CARTESIAN_POINT('Origin',(8.,-2.15,-35.1931195934094)) ;
#115301=CARTESIAN_POINT('',(8.,-2.32153024911033,-33.4897267659824)) ;
#115302=CARTESIAN_POINT('Origin',(8.,-3.65625,-34.29)) ;
#115303=CARTESIAN_POINT('',(8.,-2.35,-33.3868804065906)) ;
#115304=CARTESIAN_POINT('Origin',(8.,-2.15,-33.3868804065906)) ;
#115305=CARTESIAN_POINT('',(8.,-2.35,-32.74)) ;
#115306=CARTESIAN_POINT('',(8.,-2.35,-32.74)) ;
#115307=CARTESIAN_POINT('',(8.,-2.15,-32.54)) ;
#115308=CARTESIAN_POINT('Origin',(8.,-2.15,-32.74)) ;
#115309=CARTESIAN_POINT('',(8.,1.9,-32.54)) ;
#115310=CARTESIAN_POINT('',(8.,1.9,-28.73)) ;
#115311=CARTESIAN_POINT('',(8.,2.1,-28.93)) ;
#115312=CARTESIAN_POINT('Origin',(8.,1.9,-28.93)) ;
#115313=CARTESIAN_POINT('',(8.,2.1,-29.88)) ;
#115314=CARTESIAN_POINT('',(8.,2.1,-29.88)) ;
#115315=CARTESIAN_POINT('',(8.,2.4,-29.88)) ;
#115316=CARTESIAN_POINT('',(8.,2.4,-29.88)) ;
#115317=CARTESIAN_POINT('',(8.,2.4,-29.7714213562373)) ;
#115318=CARTESIAN_POINT('',(8.,2.4,-29.7714213562373)) ;
#115319=CARTESIAN_POINT('',(8.,2.45857864376269,-29.63)) ;
#115320=CARTESIAN_POINT('Origin',(8.,2.6,-29.7714213562373)) ;
#115321=CARTESIAN_POINT('',(8.,3.00857864376269,-29.08)) ;
#115322=CARTESIAN_POINT('',(8.,3.00857864376269,-29.08)) ;
#115323=CARTESIAN_POINT('',(8.,3.35,-29.2214213562373)) ;
#115324=CARTESIAN_POINT('Origin',(8.,3.15,-29.2214213562373)) ;
#115325=CARTESIAN_POINT('',(8.,3.35,-31.7385786437627)) ;
#115326=CARTESIAN_POINT('',(8.,2.45857864376269,-31.33)) ;
#115327=CARTESIAN_POINT('',(8.,2.45857864376269,-31.33)) ;
#115328=CARTESIAN_POINT('',(8.,2.4,-31.1885786437627)) ;
#115329=CARTESIAN_POINT('Origin',(8.,2.6,-31.1885786437627)) ;
#115330=CARTESIAN_POINT('',(8.,2.4,-31.08)) ;
#115331=CARTESIAN_POINT('',(8.,2.4,-31.08)) ;
#115332=CARTESIAN_POINT('',(8.,2.1,-31.08)) ;
#115333=CARTESIAN_POINT('',(8.,2.1,-31.08)) ;
#115334=CARTESIAN_POINT('',(8.,2.1,-32.03)) ;
#115335=CARTESIAN_POINT('',(8.,2.1,-32.03)) ;
#115336=CARTESIAN_POINT('',(8.,1.9,-32.23)) ;
#115337=CARTESIAN_POINT('Origin',(8.,1.9,-32.03)) ;
#115338=CARTESIAN_POINT('',(8.,-2.15,-32.23)) ;
#115339=CARTESIAN_POINT('',(8.,-2.15,-32.23)) ;
#115340=CARTESIAN_POINT('',(8.,-2.35,-32.03)) ;
#115341=CARTESIAN_POINT('Origin',(8.,-2.15,-32.03)) ;
#115342=CARTESIAN_POINT('',(8.,-2.35,-31.3831195934094)) ;
#115343=CARTESIAN_POINT('',(8.,-2.35,-31.3831195934094)) ;
#115344=CARTESIAN_POINT('',(8.,-2.32153024911032,-31.2802732340176)) ;
#115345=CARTESIAN_POINT('Origin',(8.,-2.15,-31.3831195934094)) ;
#115346=CARTESIAN_POINT('',(8.,-2.32153024911032,-29.6797267659824)) ;
#115347=CARTESIAN_POINT('Origin',(8.,-3.65625,-30.48)) ;
#115348=CARTESIAN_POINT('',(8.,-2.35,-29.5768804065906)) ;
#115349=CARTESIAN_POINT('Origin',(8.,-2.15,-29.5768804065906)) ;
#115350=CARTESIAN_POINT('',(8.,-2.35,-28.93)) ;
#115351=CARTESIAN_POINT('',(8.,-2.35,-28.93)) ;
#115352=CARTESIAN_POINT('',(8.,-2.15,-28.73)) ;
#115353=CARTESIAN_POINT('Origin',(8.,-2.15,-28.93)) ;
#115354=CARTESIAN_POINT('',(8.,1.9,-28.73)) ;
#115355=CARTESIAN_POINT('',(8.,1.9,-24.92)) ;
#115356=CARTESIAN_POINT('',(8.,2.1,-25.12)) ;
#115357=CARTESIAN_POINT('Origin',(8.,1.9,-25.12)) ;
#115358=CARTESIAN_POINT('',(8.,2.1,-26.07)) ;
#115359=CARTESIAN_POINT('',(8.,2.1,-26.07)) ;
#115360=CARTESIAN_POINT('',(8.,2.4,-26.07)) ;
#115361=CARTESIAN_POINT('',(8.,2.4,-26.07)) ;
#115362=CARTESIAN_POINT('',(8.,2.4,-25.9614213562373)) ;
#115363=CARTESIAN_POINT('',(8.,2.4,-25.9614213562373)) ;
#115364=CARTESIAN_POINT('',(8.,2.45857864376269,-25.82)) ;
#115365=CARTESIAN_POINT('Origin',(8.,2.6,-25.9614213562373)) ;
#115366=CARTESIAN_POINT('',(8.,3.00857864376269,-25.27)) ;
#115367=CARTESIAN_POINT('',(8.,3.00857864376269,-25.27)) ;
#115368=CARTESIAN_POINT('',(8.,3.35,-25.4114213562373)) ;
#115369=CARTESIAN_POINT('Origin',(8.,3.15,-25.4114213562373)) ;
#115370=CARTESIAN_POINT('',(8.,3.35,-27.9285786437627)) ;
#115371=CARTESIAN_POINT('',(8.,2.45857864376269,-27.52)) ;
#115372=CARTESIAN_POINT('',(8.,2.45857864376269,-27.52)) ;
#115373=CARTESIAN_POINT('',(8.,2.4,-27.3785786437627)) ;
#115374=CARTESIAN_POINT('Origin',(8.,2.6,-27.3785786437627)) ;
#115375=CARTESIAN_POINT('',(8.,2.4,-27.27)) ;
#115376=CARTESIAN_POINT('',(8.,2.4,-27.27)) ;
#115377=CARTESIAN_POINT('',(8.,2.1,-27.27)) ;
#115378=CARTESIAN_POINT('',(8.,2.1,-27.27)) ;
#115379=CARTESIAN_POINT('',(8.,2.1,-28.22)) ;
#115380=CARTESIAN_POINT('',(8.,2.1,-28.22)) ;
#115381=CARTESIAN_POINT('',(8.,1.9,-28.42)) ;
#115382=CARTESIAN_POINT('Origin',(8.,1.9,-28.22)) ;
#115383=CARTESIAN_POINT('',(8.,-2.15,-28.42)) ;
#115384=CARTESIAN_POINT('',(8.,-2.15,-28.42)) ;
#115385=CARTESIAN_POINT('',(8.,-2.35,-28.22)) ;
#115386=CARTESIAN_POINT('Origin',(8.,-2.15,-28.22)) ;
#115387=CARTESIAN_POINT('',(8.,-2.35,-27.5731195934094)) ;
#115388=CARTESIAN_POINT('',(8.,-2.35,-27.5731195934094)) ;
#115389=CARTESIAN_POINT('',(8.,-2.32153024911032,-27.4702732340176)) ;
#115390=CARTESIAN_POINT('Origin',(8.,-2.15,-27.5731195934094)) ;
#115391=CARTESIAN_POINT('',(8.,-2.32153024911032,-25.8697267659824)) ;
#115392=CARTESIAN_POINT('Origin',(8.,-3.65625,-26.67)) ;
#115393=CARTESIAN_POINT('',(8.,-2.35,-25.7668804065906)) ;
#115394=CARTESIAN_POINT('Origin',(8.,-2.15,-25.7668804065906)) ;
#115395=CARTESIAN_POINT('',(8.,-2.35,-25.12)) ;
#115396=CARTESIAN_POINT('',(8.,-2.35,-25.12)) ;
#115397=CARTESIAN_POINT('',(8.,-2.15,-24.92)) ;
#115398=CARTESIAN_POINT('Origin',(8.,-2.15,-25.12)) ;
#115399=CARTESIAN_POINT('',(8.,1.9,-24.92)) ;
#115400=CARTESIAN_POINT('',(8.,1.9,-21.11)) ;
#115401=CARTESIAN_POINT('',(8.,2.1,-21.31)) ;
#115402=CARTESIAN_POINT('Origin',(8.,1.9,-21.31)) ;
#115403=CARTESIAN_POINT('',(8.,2.1,-22.26)) ;
#115404=CARTESIAN_POINT('',(8.,2.1,-22.26)) ;
#115405=CARTESIAN_POINT('',(8.,2.4,-22.26)) ;
#115406=CARTESIAN_POINT('',(8.,2.4,-22.26)) ;
#115407=CARTESIAN_POINT('',(8.,2.4,-22.1514213562373)) ;
#115408=CARTESIAN_POINT('',(8.,2.4,-22.1514213562373)) ;
#115409=CARTESIAN_POINT('',(8.,2.45857864376269,-22.01)) ;
#115410=CARTESIAN_POINT('Origin',(8.,2.6,-22.1514213562373)) ;
#115411=CARTESIAN_POINT('',(8.,3.00857864376269,-21.46)) ;
#115412=CARTESIAN_POINT('',(8.,3.00857864376269,-21.46)) ;
#115413=CARTESIAN_POINT('',(8.,3.35,-21.6014213562373)) ;
#115414=CARTESIAN_POINT('Origin',(8.,3.15,-21.6014213562373)) ;
#115415=CARTESIAN_POINT('',(8.,3.35,-24.1185786437627)) ;
#115416=CARTESIAN_POINT('',(8.,2.45857864376269,-23.71)) ;
#115417=CARTESIAN_POINT('',(8.,2.45857864376269,-23.71)) ;
#115418=CARTESIAN_POINT('',(8.,2.4,-23.5685786437627)) ;
#115419=CARTESIAN_POINT('Origin',(8.,2.6,-23.5685786437627)) ;
#115420=CARTESIAN_POINT('',(8.,2.4,-23.46)) ;
#115421=CARTESIAN_POINT('',(8.,2.4,-23.46)) ;
#115422=CARTESIAN_POINT('',(8.,2.1,-23.46)) ;
#115423=CARTESIAN_POINT('',(8.,2.1,-23.46)) ;
#115424=CARTESIAN_POINT('',(8.,2.1,-24.41)) ;
#115425=CARTESIAN_POINT('',(8.,2.1,-24.41)) ;
#115426=CARTESIAN_POINT('',(8.,1.9,-24.61)) ;
#115427=CARTESIAN_POINT('Origin',(8.,1.9,-24.41)) ;
#115428=CARTESIAN_POINT('',(8.,-2.15,-24.61)) ;
#115429=CARTESIAN_POINT('',(8.,-2.15,-24.61)) ;
#115430=CARTESIAN_POINT('',(8.,-2.35,-24.41)) ;
#115431=CARTESIAN_POINT('Origin',(8.,-2.15,-24.41)) ;
#115432=CARTESIAN_POINT('',(8.,-2.35,-23.7631195934094)) ;
#115433=CARTESIAN_POINT('',(8.,-2.35,-23.7631195934094)) ;
#115434=CARTESIAN_POINT('',(8.,-2.32153024911032,-23.6602732340176)) ;
#115435=CARTESIAN_POINT('Origin',(8.,-2.15,-23.7631195934094)) ;
#115436=CARTESIAN_POINT('',(8.,-2.32153024911032,-22.0597267659824)) ;
#115437=CARTESIAN_POINT('Origin',(8.,-3.65625,-22.86)) ;
#115438=CARTESIAN_POINT('',(8.,-2.35,-21.9568804065906)) ;
#115439=CARTESIAN_POINT('Origin',(8.,-2.15,-21.9568804065906)) ;
#115440=CARTESIAN_POINT('',(8.,-2.35,-21.31)) ;
#115441=CARTESIAN_POINT('',(8.,-2.35,-21.31)) ;
#115442=CARTESIAN_POINT('',(8.,-2.15,-21.11)) ;
#115443=CARTESIAN_POINT('Origin',(8.,-2.15,-21.31)) ;
#115444=CARTESIAN_POINT('',(8.,1.9,-21.11)) ;
#115445=CARTESIAN_POINT('',(8.,1.9,-17.3)) ;
#115446=CARTESIAN_POINT('',(8.,2.1,-17.5)) ;
#115447=CARTESIAN_POINT('Origin',(8.,1.9,-17.5)) ;
#115448=CARTESIAN_POINT('',(8.,2.1,-18.45)) ;
#115449=CARTESIAN_POINT('',(8.,2.1,-18.45)) ;
#115450=CARTESIAN_POINT('',(8.,2.4,-18.45)) ;
#115451=CARTESIAN_POINT('',(8.,2.4,-18.45)) ;
#115452=CARTESIAN_POINT('',(8.,2.4,-18.3414213562373)) ;
#115453=CARTESIAN_POINT('',(8.,2.4,-18.3414213562373)) ;
#115454=CARTESIAN_POINT('',(8.,2.45857864376269,-18.2)) ;
#115455=CARTESIAN_POINT('Origin',(8.,2.6,-18.3414213562373)) ;
#115456=CARTESIAN_POINT('',(8.,3.00857864376269,-17.65)) ;
#115457=CARTESIAN_POINT('',(8.,3.00857864376269,-17.65)) ;
#115458=CARTESIAN_POINT('',(8.,3.35,-17.7914213562373)) ;
#115459=CARTESIAN_POINT('Origin',(8.,3.15,-17.7914213562373)) ;
#115460=CARTESIAN_POINT('',(8.,3.35,-20.3085786437627)) ;
#115461=CARTESIAN_POINT('',(8.,2.45857864376269,-19.9)) ;
#115462=CARTESIAN_POINT('',(8.,2.45857864376269,-19.9)) ;
#115463=CARTESIAN_POINT('',(8.,2.4,-19.7585786437627)) ;
#115464=CARTESIAN_POINT('Origin',(8.,2.6,-19.7585786437627)) ;
#115465=CARTESIAN_POINT('',(8.,2.4,-19.65)) ;
#115466=CARTESIAN_POINT('',(8.,2.4,-19.65)) ;
#115467=CARTESIAN_POINT('',(8.,2.1,-19.65)) ;
#115468=CARTESIAN_POINT('',(8.,2.1,-19.65)) ;
#115469=CARTESIAN_POINT('',(8.,2.1,-20.6)) ;
#115470=CARTESIAN_POINT('',(8.,2.1,-20.6)) ;
#115471=CARTESIAN_POINT('',(8.,1.9,-20.8)) ;
#115472=CARTESIAN_POINT('Origin',(8.,1.9,-20.6)) ;
#115473=CARTESIAN_POINT('',(8.,-2.15,-20.8)) ;
#115474=CARTESIAN_POINT('',(8.,-2.15,-20.8)) ;
#115475=CARTESIAN_POINT('',(8.,-2.35,-20.6)) ;
#115476=CARTESIAN_POINT('Origin',(8.,-2.15,-20.6)) ;
#115477=CARTESIAN_POINT('',(8.,-2.35,-19.9531195934094)) ;
#115478=CARTESIAN_POINT('',(8.,-2.35,-19.9531195934094)) ;
#115479=CARTESIAN_POINT('',(8.,-2.32153024911032,-19.8502732340176)) ;
#115480=CARTESIAN_POINT('Origin',(8.,-2.15,-19.9531195934094)) ;
#115481=CARTESIAN_POINT('',(8.,-2.32153024911032,-18.2497267659824)) ;
#115482=CARTESIAN_POINT('Origin',(8.,-3.65625,-19.05)) ;
#115483=CARTESIAN_POINT('',(8.,-2.35,-18.1468804065906)) ;
#115484=CARTESIAN_POINT('Origin',(8.,-2.15,-18.1468804065906)) ;
#115485=CARTESIAN_POINT('',(8.,-2.35,-17.5)) ;
#115486=CARTESIAN_POINT('',(8.,-2.35,-17.5)) ;
#115487=CARTESIAN_POINT('',(8.,-2.15,-17.3)) ;
#115488=CARTESIAN_POINT('Origin',(8.,-2.15,-17.5)) ;
#115489=CARTESIAN_POINT('',(8.,1.9,-17.3)) ;
#115490=CARTESIAN_POINT('',(8.,1.9,-13.49)) ;
#115491=CARTESIAN_POINT('',(8.,2.1,-13.69)) ;
#115492=CARTESIAN_POINT('Origin',(8.,1.9,-13.69)) ;
#115493=CARTESIAN_POINT('',(8.,2.1,-14.64)) ;
#115494=CARTESIAN_POINT('',(8.,2.1,-14.64)) ;
#115495=CARTESIAN_POINT('',(8.,2.4,-14.64)) ;
#115496=CARTESIAN_POINT('',(8.,2.4,-14.64)) ;
#115497=CARTESIAN_POINT('',(8.,2.4,-14.5314213562373)) ;
#115498=CARTESIAN_POINT('',(8.,2.4,-14.5314213562373)) ;
#115499=CARTESIAN_POINT('',(8.,2.45857864376269,-14.39)) ;
#115500=CARTESIAN_POINT('Origin',(8.,2.6,-14.5314213562373)) ;
#115501=CARTESIAN_POINT('',(8.,3.00857864376269,-13.84)) ;
#115502=CARTESIAN_POINT('',(8.,3.00857864376269,-13.84)) ;
#115503=CARTESIAN_POINT('',(8.,3.35,-13.9814213562373)) ;
#115504=CARTESIAN_POINT('Origin',(8.,3.15,-13.9814213562373)) ;
#115505=CARTESIAN_POINT('',(8.,3.35,-16.4985786437627)) ;
#115506=CARTESIAN_POINT('',(8.,2.45857864376269,-16.09)) ;
#115507=CARTESIAN_POINT('',(8.,2.45857864376269,-16.09)) ;
#115508=CARTESIAN_POINT('',(8.,2.4,-15.9485786437627)) ;
#115509=CARTESIAN_POINT('Origin',(8.,2.6,-15.9485786437627)) ;
#115510=CARTESIAN_POINT('',(8.,2.4,-15.84)) ;
#115511=CARTESIAN_POINT('',(8.,2.4,-15.84)) ;
#115512=CARTESIAN_POINT('',(8.,2.1,-15.84)) ;
#115513=CARTESIAN_POINT('',(8.,2.1,-15.84)) ;
#115514=CARTESIAN_POINT('',(8.,2.1,-16.79)) ;
#115515=CARTESIAN_POINT('',(8.,2.1,-16.79)) ;
#115516=CARTESIAN_POINT('',(8.,1.9,-16.99)) ;
#115517=CARTESIAN_POINT('Origin',(8.,1.9,-16.79)) ;
#115518=CARTESIAN_POINT('',(8.,-2.15,-16.99)) ;
#115519=CARTESIAN_POINT('',(8.,-2.15,-16.99)) ;
#115520=CARTESIAN_POINT('',(8.,-2.35,-16.79)) ;
#115521=CARTESIAN_POINT('Origin',(8.,-2.15,-16.79)) ;
#115522=CARTESIAN_POINT('',(8.,-2.35,-16.1431195934094)) ;
#115523=CARTESIAN_POINT('',(8.,-2.35,-16.1431195934094)) ;
#115524=CARTESIAN_POINT('',(8.,-2.32153024911032,-16.0402732340176)) ;
#115525=CARTESIAN_POINT('Origin',(8.,-2.15,-16.1431195934094)) ;
#115526=CARTESIAN_POINT('',(8.,-2.32153024911032,-14.4397267659824)) ;
#115527=CARTESIAN_POINT('Origin',(8.,-3.65625,-15.24)) ;
#115528=CARTESIAN_POINT('',(8.,-2.35,-14.3368804065906)) ;
#115529=CARTESIAN_POINT('Origin',(8.,-2.15,-14.3368804065906)) ;
#115530=CARTESIAN_POINT('',(8.,-2.35,-13.69)) ;
#115531=CARTESIAN_POINT('',(8.,-2.35,-13.69)) ;
#115532=CARTESIAN_POINT('',(8.,-2.15,-13.49)) ;
#115533=CARTESIAN_POINT('Origin',(8.,-2.15,-13.69)) ;
#115534=CARTESIAN_POINT('',(8.,1.9,-13.49)) ;
#115535=CARTESIAN_POINT('',(8.,1.9,-9.68)) ;
#115536=CARTESIAN_POINT('',(8.,2.1,-9.88)) ;
#115537=CARTESIAN_POINT('Origin',(8.,1.9,-9.88)) ;
#115538=CARTESIAN_POINT('',(8.,2.1,-10.83)) ;
#115539=CARTESIAN_POINT('',(8.,2.1,-10.83)) ;
#115540=CARTESIAN_POINT('',(8.,2.4,-10.83)) ;
#115541=CARTESIAN_POINT('',(8.,2.4,-10.83)) ;
#115542=CARTESIAN_POINT('',(8.,2.4,-10.7214213562373)) ;
#115543=CARTESIAN_POINT('',(8.,2.4,-10.7214213562373)) ;
#115544=CARTESIAN_POINT('',(8.,2.45857864376269,-10.58)) ;
#115545=CARTESIAN_POINT('Origin',(8.,2.6,-10.7214213562373)) ;
#115546=CARTESIAN_POINT('',(8.,3.00857864376269,-10.03)) ;
#115547=CARTESIAN_POINT('',(8.,3.00857864376269,-10.03)) ;
#115548=CARTESIAN_POINT('',(8.,3.35,-10.1714213562373)) ;
#115549=CARTESIAN_POINT('Origin',(8.,3.15,-10.1714213562373)) ;
#115550=CARTESIAN_POINT('',(8.,3.35,-12.6885786437627)) ;
#115551=CARTESIAN_POINT('',(8.,2.45857864376269,-12.28)) ;
#115552=CARTESIAN_POINT('',(8.,2.45857864376269,-12.28)) ;
#115553=CARTESIAN_POINT('',(8.,2.4,-12.1385786437627)) ;
#115554=CARTESIAN_POINT('Origin',(8.,2.6,-12.1385786437627)) ;
#115555=CARTESIAN_POINT('',(8.,2.4,-12.03)) ;
#115556=CARTESIAN_POINT('',(8.,2.4,-12.03)) ;
#115557=CARTESIAN_POINT('',(8.,2.1,-12.03)) ;
#115558=CARTESIAN_POINT('',(8.,2.1,-12.03)) ;
#115559=CARTESIAN_POINT('',(8.,2.1,-12.98)) ;
#115560=CARTESIAN_POINT('',(8.,2.1,-12.98)) ;
#115561=CARTESIAN_POINT('',(8.,1.9,-13.18)) ;
#115562=CARTESIAN_POINT('Origin',(8.,1.9,-12.98)) ;
#115563=CARTESIAN_POINT('',(8.,-2.15,-13.18)) ;
#115564=CARTESIAN_POINT('',(8.,-2.15,-13.18)) ;
#115565=CARTESIAN_POINT('',(8.,-2.35,-12.98)) ;
#115566=CARTESIAN_POINT('Origin',(8.,-2.15,-12.98)) ;
#115567=CARTESIAN_POINT('',(8.,-2.35,-12.3331195934094)) ;
#115568=CARTESIAN_POINT('',(8.,-2.35,-12.3331195934094)) ;
#115569=CARTESIAN_POINT('',(8.,-2.32153024911032,-12.2302732340176)) ;
#115570=CARTESIAN_POINT('Origin',(8.,-2.15,-12.3331195934094)) ;
#115571=CARTESIAN_POINT('',(8.,-2.32153024911032,-10.6297267659824)) ;
#115572=CARTESIAN_POINT('Origin',(8.,-3.65625,-11.43)) ;
#115573=CARTESIAN_POINT('',(8.,-2.35,-10.5268804065906)) ;
#115574=CARTESIAN_POINT('Origin',(8.,-2.15,-10.5268804065906)) ;
#115575=CARTESIAN_POINT('',(8.,-2.35,-9.88)) ;
#115576=CARTESIAN_POINT('',(8.,-2.35,-9.88)) ;
#115577=CARTESIAN_POINT('',(8.,-2.15,-9.68)) ;
#115578=CARTESIAN_POINT('Origin',(8.,-2.15,-9.88)) ;
#115579=CARTESIAN_POINT('',(8.,1.9,-9.68)) ;
#115580=CARTESIAN_POINT('',(8.,1.9,-5.87)) ;
#115581=CARTESIAN_POINT('',(8.,2.1,-6.07)) ;
#115582=CARTESIAN_POINT('Origin',(8.,1.9,-6.07)) ;
#115583=CARTESIAN_POINT('',(8.,2.1,-7.02)) ;
#115584=CARTESIAN_POINT('',(8.,2.1,-7.02)) ;
#115585=CARTESIAN_POINT('',(8.,2.4,-7.02)) ;
#115586=CARTESIAN_POINT('',(8.,2.4,-7.02)) ;
#115587=CARTESIAN_POINT('',(8.,2.4,-6.91142135623731)) ;
#115588=CARTESIAN_POINT('',(8.,2.4,-6.91142135623731)) ;
#115589=CARTESIAN_POINT('',(8.,2.45857864376269,-6.77)) ;
#115590=CARTESIAN_POINT('Origin',(8.,2.6,-6.91142135623731)) ;
#115591=CARTESIAN_POINT('',(8.,3.00857864376269,-6.22)) ;
#115592=CARTESIAN_POINT('',(8.,3.00857864376269,-6.22)) ;
#115593=CARTESIAN_POINT('',(8.,3.35,-6.36142135623731)) ;
#115594=CARTESIAN_POINT('Origin',(8.,3.15,-6.36142135623731)) ;
#115595=CARTESIAN_POINT('',(8.,3.35,-8.87857864376269)) ;
#115596=CARTESIAN_POINT('',(8.,2.45857864376269,-8.47)) ;
#115597=CARTESIAN_POINT('',(8.,2.45857864376269,-8.47)) ;
#115598=CARTESIAN_POINT('',(8.,2.4,-8.32857864376269)) ;
#115599=CARTESIAN_POINT('Origin',(8.,2.6,-8.32857864376269)) ;
#115600=CARTESIAN_POINT('',(8.,2.4,-8.22)) ;
#115601=CARTESIAN_POINT('',(8.,2.4,-8.22)) ;
#115602=CARTESIAN_POINT('',(8.,2.1,-8.22)) ;
#115603=CARTESIAN_POINT('',(8.,2.1,-8.22)) ;
#115604=CARTESIAN_POINT('',(8.,2.1,-9.17)) ;
#115605=CARTESIAN_POINT('',(8.,2.1,-9.17)) ;
#115606=CARTESIAN_POINT('',(8.,1.9,-9.37)) ;
#115607=CARTESIAN_POINT('Origin',(8.,1.9,-9.17)) ;
#115608=CARTESIAN_POINT('',(8.,-2.15,-9.37)) ;
#115609=CARTESIAN_POINT('',(8.,-2.15,-9.37)) ;
#115610=CARTESIAN_POINT('',(8.,-2.35,-9.17)) ;
#115611=CARTESIAN_POINT('Origin',(8.,-2.15,-9.17)) ;
#115612=CARTESIAN_POINT('',(8.,-2.35,-8.52311959340942)) ;
#115613=CARTESIAN_POINT('',(8.,-2.35,-8.52311959340942)) ;
#115614=CARTESIAN_POINT('',(8.,-2.32153024911032,-8.4202732340176)) ;
#115615=CARTESIAN_POINT('Origin',(8.,-2.15,-8.52311959340942)) ;
#115616=CARTESIAN_POINT('',(8.,-2.32153024911032,-6.8197267659824)) ;
#115617=CARTESIAN_POINT('Origin',(8.,-3.65625,-7.62)) ;
#115618=CARTESIAN_POINT('',(8.,-2.35,-6.71688040659058)) ;
#115619=CARTESIAN_POINT('Origin',(8.,-2.15,-6.71688040659058)) ;
#115620=CARTESIAN_POINT('',(8.,-2.35,-6.07)) ;
#115621=CARTESIAN_POINT('',(8.,-2.35,-6.07)) ;
#115622=CARTESIAN_POINT('',(8.,-2.15,-5.87)) ;
#115623=CARTESIAN_POINT('Origin',(8.,-2.15,-6.07)) ;
#115624=CARTESIAN_POINT('',(8.,1.9,-5.87)) ;
#115625=CARTESIAN_POINT('',(8.,1.9,-2.06)) ;
#115626=CARTESIAN_POINT('',(8.,2.1,-2.26)) ;
#115627=CARTESIAN_POINT('Origin',(8.,1.9,-2.26)) ;
#115628=CARTESIAN_POINT('',(8.,2.1,-3.21)) ;
#115629=CARTESIAN_POINT('',(8.,2.1,-3.21)) ;
#115630=CARTESIAN_POINT('',(8.,2.4,-3.21)) ;
#115631=CARTESIAN_POINT('',(8.,2.4,-3.21)) ;
#115632=CARTESIAN_POINT('',(8.,2.4,-3.10142135623731)) ;
#115633=CARTESIAN_POINT('',(8.,2.4,-3.10142135623731)) ;
#115634=CARTESIAN_POINT('',(8.,2.45857864376269,-2.96)) ;
#115635=CARTESIAN_POINT('Origin',(8.,2.6,-3.10142135623731)) ;
#115636=CARTESIAN_POINT('',(8.,3.00857864376269,-2.41)) ;
#115637=CARTESIAN_POINT('',(8.,3.00857864376269,-2.41)) ;
#115638=CARTESIAN_POINT('',(8.,3.35,-2.55142135623731)) ;
#115639=CARTESIAN_POINT('Origin',(8.,3.15,-2.55142135623731)) ;
#115640=CARTESIAN_POINT('',(8.,3.35,-5.06857864376269)) ;
#115641=CARTESIAN_POINT('',(8.,2.45857864376269,-4.66)) ;
#115642=CARTESIAN_POINT('',(8.,2.45857864376269,-4.66)) ;
#115643=CARTESIAN_POINT('',(8.,2.4,-4.51857864376269)) ;
#115644=CARTESIAN_POINT('Origin',(8.,2.6,-4.51857864376269)) ;
#115645=CARTESIAN_POINT('',(8.,2.4,-4.41)) ;
#115646=CARTESIAN_POINT('',(8.,2.4,-4.41)) ;
#115647=CARTESIAN_POINT('',(8.,2.1,-4.41)) ;
#115648=CARTESIAN_POINT('',(8.,2.1,-4.41)) ;
#115649=CARTESIAN_POINT('',(8.,2.1,-5.36)) ;
#115650=CARTESIAN_POINT('',(8.,2.1,-5.36)) ;
#115651=CARTESIAN_POINT('',(8.,1.9,-5.56)) ;
#115652=CARTESIAN_POINT('Origin',(8.,1.9,-5.36)) ;
#115653=CARTESIAN_POINT('',(8.,-2.15,-5.56)) ;
#115654=CARTESIAN_POINT('',(8.,-2.15,-5.56)) ;
#115655=CARTESIAN_POINT('',(8.,-2.35,-5.36)) ;
#115656=CARTESIAN_POINT('Origin',(8.,-2.15,-5.36)) ;
#115657=CARTESIAN_POINT('',(8.,-2.35,-4.71311959340942)) ;
#115658=CARTESIAN_POINT('',(8.,-2.35,-4.71311959340942)) ;
#115659=CARTESIAN_POINT('',(8.,-2.32153024911032,-4.6102732340176)) ;
#115660=CARTESIAN_POINT('Origin',(8.,-2.15,-4.71311959340942)) ;
#115661=CARTESIAN_POINT('',(8.,-2.32153024911032,-3.0097267659824)) ;
#115662=CARTESIAN_POINT('Origin',(8.,-3.65625,-3.81)) ;
#115663=CARTESIAN_POINT('',(8.,-2.35,-2.90688040659058)) ;
#115664=CARTESIAN_POINT('Origin',(8.,-2.15,-2.90688040659058)) ;
#115665=CARTESIAN_POINT('',(8.,-2.35,-2.26)) ;
#115666=CARTESIAN_POINT('',(8.,-2.35,-2.26)) ;
#115667=CARTESIAN_POINT('',(8.,-2.15,-2.06)) ;
#115668=CARTESIAN_POINT('Origin',(8.,-2.15,-2.26)) ;
#115669=CARTESIAN_POINT('',(8.,1.9,-2.06)) ;
#115670=CARTESIAN_POINT('',(8.,1.9,1.75)) ;
#115671=CARTESIAN_POINT('',(8.,2.1,1.55)) ;
#115672=CARTESIAN_POINT('Origin',(8.,1.9,1.55)) ;
#115673=CARTESIAN_POINT('',(8.,2.1,0.6)) ;
#115674=CARTESIAN_POINT('',(8.,2.1,0.600000000000003)) ;
#115675=CARTESIAN_POINT('',(8.,2.4,0.6)) ;
#115676=CARTESIAN_POINT('',(8.,2.4,0.6)) ;
#115677=CARTESIAN_POINT('',(8.,2.4,0.70857864376269)) ;
#115678=CARTESIAN_POINT('',(8.,2.4,0.70857864376269)) ;
#115679=CARTESIAN_POINT('',(8.,2.45857864376269,0.849999999999999)) ;
#115680=CARTESIAN_POINT('Origin',(8.,2.6,0.70857864376269)) ;
#115681=CARTESIAN_POINT('',(8.,3.00857864376269,1.4)) ;
#115682=CARTESIAN_POINT('',(8.,3.00857864376269,1.4)) ;
#115683=CARTESIAN_POINT('',(8.,3.35,1.25857864376269)) ;
#115684=CARTESIAN_POINT('Origin',(8.,3.15,1.25857864376269)) ;
#115685=CARTESIAN_POINT('',(8.,3.35,-1.25857864376269)) ;
#115686=CARTESIAN_POINT('',(8.,2.45857864376269,-0.850000000000001)) ;
#115687=CARTESIAN_POINT('',(8.,2.45857864376269,-0.85)) ;
#115688=CARTESIAN_POINT('',(8.,2.4,-0.70857864376269)) ;
#115689=CARTESIAN_POINT('Origin',(8.,2.6,-0.70857864376269)) ;
#115690=CARTESIAN_POINT('',(8.,2.4,-0.6)) ;
#115691=CARTESIAN_POINT('',(8.,2.4,-0.6)) ;
#115692=CARTESIAN_POINT('',(8.,2.1,-0.6)) ;
#115693=CARTESIAN_POINT('',(8.,2.1,-0.6)) ;
#115694=CARTESIAN_POINT('',(8.,2.1,-1.55)) ;
#115695=CARTESIAN_POINT('',(8.,2.1,-1.55)) ;
#115696=CARTESIAN_POINT('',(8.,1.9,-1.75)) ;
#115697=CARTESIAN_POINT('Origin',(8.,1.9,-1.55)) ;
#115698=CARTESIAN_POINT('',(8.,-2.15,-1.75)) ;
#115699=CARTESIAN_POINT('',(8.,-2.15,-1.75)) ;
#115700=CARTESIAN_POINT('',(8.,-2.35,-1.55)) ;
#115701=CARTESIAN_POINT('Origin',(8.,-2.15,-1.55)) ;
#115702=CARTESIAN_POINT('',(8.,-2.35,-0.903119593409422)) ;
#115703=CARTESIAN_POINT('',(8.,-2.35,-0.903119593409422)) ;
#115704=CARTESIAN_POINT('',(8.,-2.32153024911032,-0.800273234017602)) ;
#115705=CARTESIAN_POINT('Origin',(8.,-2.15,-0.903119593409422)) ;
#115706=CARTESIAN_POINT('',(8.,-2.32153024911032,0.800273234017602)) ;
#115707=CARTESIAN_POINT('Origin',(8.,-3.65625,0.)) ;
#115708=CARTESIAN_POINT('',(8.,-2.35,0.903119593409422)) ;
#115709=CARTESIAN_POINT('Origin',(8.,-2.15,0.903119593409422)) ;
#115710=CARTESIAN_POINT('',(8.,-2.35,1.55)) ;
#115711=CARTESIAN_POINT('',(8.,-2.35,1.55)) ;
#115712=CARTESIAN_POINT('',(8.,-2.15,1.75)) ;
#115713=CARTESIAN_POINT('Origin',(8.,-2.15,1.55)) ;
#115714=CARTESIAN_POINT('',(8.,1.9,1.75)) ;
#115715=CARTESIAN_POINT('Origin',(7.9,-2.9,-36.89)) ;
#115716=CARTESIAN_POINT('',(7.9,4.15,-36.89)) ;
#115717=CARTESIAN_POINT('',(7.9,-2.9,-36.89)) ;
#115718=CARTESIAN_POINT('',(7.9,-2.9,-36.89)) ;
#115719=CARTESIAN_POINT('',(-1.1,-2.9,-36.89)) ;
#115720=CARTESIAN_POINT('',(-1.1,-2.9,-36.89)) ;
#115721=CARTESIAN_POINT('',(-1.1,4.15,-36.89)) ;
#115722=CARTESIAN_POINT('',(-1.1,4.15,-36.89)) ;
#115723=CARTESIAN_POINT('',(4.35,4.15,-36.89)) ;
#115724=CARTESIAN_POINT('',(4.35,4.15,-36.89)) ;
#115725=CARTESIAN_POINT('',(4.55,4.35,-36.89)) ;
#115726=CARTESIAN_POINT('Origin',(4.35,4.35,-36.89)) ;
#115727=CARTESIAN_POINT('',(4.55,4.55,-36.89)) ;
#115728=CARTESIAN_POINT('',(4.55,4.55,-36.89)) ;
#115729=CARTESIAN_POINT('',(4.75,4.55,-36.89)) ;
#115730=CARTESIAN_POINT('',(4.75,4.55,-36.89)) ;
#115731=CARTESIAN_POINT('',(4.75,4.35,-36.89)) ;
#115732=CARTESIAN_POINT('',(4.75,4.35,-36.89)) ;
#115733=CARTESIAN_POINT('',(4.95,4.15,-36.89)) ;
#115734=CARTESIAN_POINT('Origin',(4.95,4.35,-36.89)) ;
#115735=CARTESIAN_POINT('',(7.9,4.15,-36.89)) ;
#115736=CARTESIAN_POINT('Origin',(7.9,-2.9,2.6)) ;
#115737=CARTESIAN_POINT('',(-1.1,4.15,2.6)) ;
#115738=CARTESIAN_POINT('',(-1.1,-2.9,2.6)) ;
#115739=CARTESIAN_POINT('',(-1.1,-2.9,2.6)) ;
#115740=CARTESIAN_POINT('',(7.9,-2.9,2.6)) ;
#115741=CARTESIAN_POINT('',(7.9,-2.9,2.6)) ;
#115742=CARTESIAN_POINT('',(7.9,4.15,2.6)) ;
#115743=CARTESIAN_POINT('',(7.9,-2.9,2.6)) ;
#115744=CARTESIAN_POINT('',(4.95,4.15,2.6)) ;
#115745=CARTESIAN_POINT('',(7.9,4.15,2.6)) ;
#115746=CARTESIAN_POINT('',(4.75,4.35,2.6)) ;
#115747=CARTESIAN_POINT('Origin',(4.95,4.35,2.6)) ;
#115748=CARTESIAN_POINT('',(4.75,4.55,2.6)) ;
#115749=CARTESIAN_POINT('',(4.74999999999997,-2.89999999999999,2.6)) ;
#115750=CARTESIAN_POINT('',(4.55,4.55,2.6)) ;
#115751=CARTESIAN_POINT('',(7.9,4.55,2.6)) ;
#115752=CARTESIAN_POINT('',(4.55,4.35,2.6)) ;
#115753=CARTESIAN_POINT('',(4.55,-2.9,2.6)) ;
#115754=CARTESIAN_POINT('',(4.35,4.15,2.6)) ;
#115755=CARTESIAN_POINT('Origin',(4.35,4.35,2.6)) ;
#115756=CARTESIAN_POINT('',(7.9,4.15,2.6)) ;
#115757=CARTESIAN_POINT('Origin',(-0.999999999999999,-1.59070596587277E-16,
0.)) ;
#115758=CARTESIAN_POINT('',(-0.999999999999999,-1.9,0.6)) ;
#115759=CARTESIAN_POINT('',(-0.999999999999999,-1.9,1.275)) ;
#115760=CARTESIAN_POINT('',(-0.999999999999999,-1.9,1.375)) ;
#115761=CARTESIAN_POINT('',(-0.999999999999999,1.15,1.275)) ;
#115762=CARTESIAN_POINT('',(-0.999999999999999,-2.89663358890161E-17,1.275)) ;
#115763=CARTESIAN_POINT('',(-0.999999999999999,1.15,-1.275)) ;
#115764=CARTESIAN_POINT('',(-0.999999999999999,1.15,0.)) ;
#115765=CARTESIAN_POINT('',(-0.999999999999999,-1.9,-1.275)) ;
#115766=CARTESIAN_POINT('',(-0.999999999999999,-2.24122726936407E-16,-1.275)) ;
#115767=CARTESIAN_POINT('',(-0.999999999999999,-1.9,-0.6)) ;
#115768=CARTESIAN_POINT('',(-0.999999999999999,-1.9,-0.5)) ;
#115769=CARTESIAN_POINT('',(-0.999999999999999,0.4,-0.6)) ;
#115770=CARTESIAN_POINT('',(-0.999999999999999,0.5,-0.6)) ;
#115771=CARTESIAN_POINT('',(-0.999999999999999,0.6,-0.4)) ;
#115772=CARTESIAN_POINT('Origin',(-0.999999999999999,0.4,-0.4)) ;
#115773=CARTESIAN_POINT('',(-0.999999999999999,0.6,0.4)) ;
#115774=CARTESIAN_POINT('',(-0.999999999999999,0.6,0.5)) ;
#115775=CARTESIAN_POINT('',(-0.999999999999999,0.4,0.6)) ;
#115776=CARTESIAN_POINT('Origin',(-0.999999999999999,0.4,0.4)) ;
#115777=CARTESIAN_POINT('',(-0.999999999999999,-2.,0.6)) ;
#115778=CARTESIAN_POINT('Origin',(0.600000000000001,-2.,-0.5)) ;
#115779=CARTESIAN_POINT('',(0.500000000000001,-2.,-0.6)) ;
#115780=CARTESIAN_POINT('',(-0.899999999999999,-2.,-0.6)) ;
#115781=CARTESIAN_POINT('',(0.600000000000001,-2.,-0.6)) ;
#115782=CARTESIAN_POINT('',(-0.899999999999999,-2.,-1.275)) ;
#115783=CARTESIAN_POINT('',(-0.899999999999999,-2.,-1.375)) ;
#115784=CARTESIAN_POINT('',(0.500000000000001,-2.,-1.275)) ;
#115785=CARTESIAN_POINT('',(0.600000000000001,-2.,-1.275)) ;
#115786=CARTESIAN_POINT('',(0.500000000000001,-2.,-0.5)) ;
#115787=CARTESIAN_POINT('Origin',(0.600000000000001,0.5,-0.5)) ;
#115788=CARTESIAN_POINT('',(-0.899999999999999,0.4,-0.5)) ;
#115789=CARTESIAN_POINT('',(-0.999999999999999,0.4,-0.5)) ;
#115790=CARTESIAN_POINT('',(-0.899999999999999,-1.9,-0.5)) ;
#115791=CARTESIAN_POINT('',(-0.899999999999999,-2.,-0.5)) ;
#115792=CARTESIAN_POINT('',(0.600000000000001,-1.9,-0.5)) ;
#115793=CARTESIAN_POINT('Origin',(0.600000000000001,0.5,0.5)) ;
#115794=CARTESIAN_POINT('',(0.500000000000001,0.5,0.4)) ;
#115795=CARTESIAN_POINT('',(-0.899999999999999,0.5,0.4)) ;
#115796=CARTESIAN_POINT('',(-0.999999999999999,0.5,0.4)) ;
#115797=CARTESIAN_POINT('',(-0.899999999999999,0.5,-0.4)) ;
#115798=CARTESIAN_POINT('',(-0.899999999999999,0.5,-0.5)) ;
#115799=CARTESIAN_POINT('',(0.500000000000001,0.5,-0.4)) ;
#115800=CARTESIAN_POINT('',(0.600000000000001,0.5,-0.4)) ;
#115801=CARTESIAN_POINT('',(0.500000000000001,0.5,0.5)) ;
#115802=CARTESIAN_POINT('Origin',(0.600000000000001,-2.,0.5)) ;
#115803=CARTESIAN_POINT('',(0.500000000000001,-1.9,0.5)) ;
#115804=CARTESIAN_POINT('',(-0.899999999999999,-1.9,0.5)) ;
#115805=CARTESIAN_POINT('',(0.600000000000001,-1.9,0.5)) ;
#115806=CARTESIAN_POINT('',(-0.899999999999999,0.4,0.5)) ;
#115807=CARTESIAN_POINT('',(-0.899999999999999,0.5,0.5)) ;
#115808=CARTESIAN_POINT('',(0.500000000000001,0.4,0.5)) ;
#115809=CARTESIAN_POINT('',(0.600000000000001,0.4,0.5)) ;
#115810=CARTESIAN_POINT('',(0.500000000000001,-2.,0.5)) ;
#115811=CARTESIAN_POINT('Origin',(0.600000000000001,-2.,1.375)) ;
#115812=CARTESIAN_POINT('',(0.500000000000001,-2.,1.275)) ;
#115813=CARTESIAN_POINT('',(-0.899999999999999,-2.,1.275)) ;
#115814=CARTESIAN_POINT('',(-0.999999999999999,-2.,1.275)) ;
#115815=CARTESIAN_POINT('',(-0.899999999999999,-2.,0.6)) ;
#115816=CARTESIAN_POINT('',(-0.899999999999999,-2.,0.5)) ;
#115817=CARTESIAN_POINT('',(0.500000000000001,-2.,0.6)) ;
#115818=CARTESIAN_POINT('',(0.600000000000001,-2.,0.6)) ;
#115819=CARTESIAN_POINT('',(0.500000000000001,-2.,1.375)) ;
#115820=CARTESIAN_POINT('Origin',(1.4,2.1,0.6)) ;
#115821=CARTESIAN_POINT('',(1.5,2.,0.6)) ;
#115822=CARTESIAN_POINT('',(7.9,2.,0.6)) ;
#115823=CARTESIAN_POINT('',(1.4,2.,0.6)) ;
#115824=CARTESIAN_POINT('',(1.5,2.1,0.5)) ;
#115825=CARTESIAN_POINT('Origin',(1.5,2.1,0.6)) ;
#115826=CARTESIAN_POINT('',(7.9,2.1,0.5)) ;
#115827=CARTESIAN_POINT('',(1.4,2.1,0.5)) ;
#115828=CARTESIAN_POINT('Origin',(7.9,2.1,0.6)) ;
#115829=CARTESIAN_POINT('Origin',(1.4,2.4,0.5)) ;
#115830=CARTESIAN_POINT('',(1.5,2.4,0.5)) ;
#115831=CARTESIAN_POINT('',(1.5,2.4,0.5)) ;
#115832=CARTESIAN_POINT('',(7.9,2.4,0.5)) ;
#115833=CARTESIAN_POINT('',(1.4,2.4,0.5)) ;
#115834=CARTESIAN_POINT('',(7.9,2.1,0.5)) ;
#115835=CARTESIAN_POINT('Origin',(1.4,2.4,0.6)) ;
#115836=CARTESIAN_POINT('',(1.5,2.5,0.6)) ;
#115837=CARTESIAN_POINT('Origin',(1.5,2.4,0.6)) ;
#115838=CARTESIAN_POINT('',(7.9,2.5,0.6)) ;
#115839=CARTESIAN_POINT('',(1.4,2.5,0.6)) ;
#115840=CARTESIAN_POINT('Origin',(7.9,2.4,0.6)) ;
#115841=CARTESIAN_POINT('Origin',(1.4,2.5,0.70857864376269)) ;
#115842=CARTESIAN_POINT('',(1.5,2.5,0.70857864376269)) ;
#115843=CARTESIAN_POINT('',(1.5,2.5,0.70857864376269)) ;
#115844=CARTESIAN_POINT('',(7.9,2.5,0.70857864376269)) ;
#115845=CARTESIAN_POINT('',(1.4,2.5,0.70857864376269)) ;
#115846=CARTESIAN_POINT('',(7.9,2.5,0.6)) ;
#115847=CARTESIAN_POINT('Origin',(1.4,2.6,0.70857864376269)) ;
#115848=CARTESIAN_POINT('',(1.5,2.52928932188135,0.779289321881344)) ;
#115849=CARTESIAN_POINT('Origin',(1.5,2.6,0.70857864376269)) ;
#115850=CARTESIAN_POINT('',(7.9,2.52928932188135,0.779289321881344)) ;
#115851=CARTESIAN_POINT('',(1.4,2.52928932188135,0.779289321881344)) ;
#115852=CARTESIAN_POINT('Origin',(7.9,2.6,0.70857864376269)) ;
#115853=CARTESIAN_POINT('Origin',(1.4,3.07928932188135,1.32928932188135)) ;
#115854=CARTESIAN_POINT('',(1.5,3.07928932188135,1.32928932188134)) ;
#115855=CARTESIAN_POINT('',(7.9,3.07928932188135,1.32928932188135)) ;
#115856=CARTESIAN_POINT('',(1.4,3.07928932188135,1.32928932188135)) ;
#115857=CARTESIAN_POINT('',(7.9,2.52928932188135,0.779289321881344)) ;
#115858=CARTESIAN_POINT('Origin',(1.4,3.15,1.25857864376269)) ;
#115859=CARTESIAN_POINT('',(7.9,3.25,1.25857864376269)) ;
#115860=CARTESIAN_POINT('',(1.4,3.25,1.25857864376269)) ;
#115861=CARTESIAN_POINT('Origin',(7.9,3.15,1.25857864376269)) ;
#115862=CARTESIAN_POINT('Origin',(1.4,3.25,-1.25857864376269)) ;
#115863=CARTESIAN_POINT('',(1.5,3.25,-1.25857864376269)) ;
#115864=CARTESIAN_POINT('',(7.9,3.25,1.25857864376269)) ;
#115865=CARTESIAN_POINT('Origin',(1.4,2.52928932188134,-0.779289321881346)) ;
#115866=CARTESIAN_POINT('',(1.5,2.52928932188134,-0.779289321881346)) ;
#115867=CARTESIAN_POINT('',(1.5,2.52928932188134,-0.779289321881346)) ;
#115868=CARTESIAN_POINT('',(7.9,2.52928932188134,-0.779289321881346)) ;
#115869=CARTESIAN_POINT('',(1.4,2.52928932188134,-0.779289321881346)) ;
#115870=CARTESIAN_POINT('',(7.9,3.07928932188135,-1.32928932188135)) ;
#115871=CARTESIAN_POINT('Origin',(1.4,2.6,-0.70857864376269)) ;
#115872=CARTESIAN_POINT('',(1.5,2.5,-0.70857864376269)) ;
#115873=CARTESIAN_POINT('Origin',(1.5,2.6,-0.70857864376269)) ;
#115874=CARTESIAN_POINT('',(7.9,2.5,-0.70857864376269)) ;
#115875=CARTESIAN_POINT('',(1.4,2.5,-0.70857864376269)) ;
#115876=CARTESIAN_POINT('Origin',(7.9,2.6,-0.70857864376269)) ;
#115877=CARTESIAN_POINT('Origin',(1.4,2.5,-0.6)) ;
#115878=CARTESIAN_POINT('',(1.5,2.5,-0.6)) ;
#115879=CARTESIAN_POINT('',(1.5,2.5,-0.6)) ;
#115880=CARTESIAN_POINT('',(7.9,2.5,-0.6)) ;
#115881=CARTESIAN_POINT('',(1.4,2.5,-0.6)) ;
#115882=CARTESIAN_POINT('',(7.9,2.5,-0.70857864376269)) ;
#115883=CARTESIAN_POINT('Origin',(1.4,2.4,-0.6)) ;
#115884=CARTESIAN_POINT('',(1.5,2.4,-0.5)) ;
#115885=CARTESIAN_POINT('Origin',(1.5,2.4,-0.6)) ;
#115886=CARTESIAN_POINT('',(7.9,2.4,-0.5)) ;
#115887=CARTESIAN_POINT('',(1.4,2.4,-0.5)) ;
#115888=CARTESIAN_POINT('Origin',(7.9,2.4,-0.6)) ;
#115889=CARTESIAN_POINT('Origin',(1.4,2.1,-0.5)) ;
#115890=CARTESIAN_POINT('',(1.5,2.1,-0.5)) ;
#115891=CARTESIAN_POINT('',(1.5,2.1,-0.5)) ;
#115892=CARTESIAN_POINT('',(7.9,2.1,-0.5)) ;
#115893=CARTESIAN_POINT('',(1.4,2.1,-0.5)) ;
#115894=CARTESIAN_POINT('',(7.9,2.4,-0.5)) ;
#115895=CARTESIAN_POINT('Origin',(1.4,2.1,-0.6)) ;
#115896=CARTESIAN_POINT('',(1.5,2.,-0.6)) ;
#115897=CARTESIAN_POINT('Origin',(1.5,2.1,-0.6)) ;
#115898=CARTESIAN_POINT('',(7.9,2.,-0.6)) ;
#115899=CARTESIAN_POINT('',(1.4,2.,-0.6)) ;
#115900=CARTESIAN_POINT('Origin',(7.9,2.1,-0.6)) ;
#115901=CARTESIAN_POINT('Origin',(1.4,2.,-0.6)) ;
#115902=CARTESIAN_POINT('',(1.5,2.,-1.55)) ;
#115903=CARTESIAN_POINT('',(1.5,2.,-1.55)) ;
#115904=CARTESIAN_POINT('',(7.9,2.,-1.55)) ;
#115905=CARTESIAN_POINT('',(1.4,2.,-1.55)) ;
#115906=CARTESIAN_POINT('',(7.9,2.,-0.6)) ;
#115907=CARTESIAN_POINT('Origin',(1.4,1.9,-1.55)) ;
#115908=CARTESIAN_POINT('',(1.5,1.9,-1.65)) ;
#115909=CARTESIAN_POINT('Origin',(1.5,1.9,-1.55)) ;
#115910=CARTESIAN_POINT('',(7.9,1.9,-1.65)) ;
#115911=CARTESIAN_POINT('',(1.4,1.9,-1.65)) ;
#115912=CARTESIAN_POINT('Origin',(7.9,1.9,-1.55)) ;
#115913=CARTESIAN_POINT('Origin',(1.4,1.9,-1.65)) ;
#115914=CARTESIAN_POINT('',(1.5,-2.15,-1.65)) ;
#115915=CARTESIAN_POINT('',(1.5,-2.15,-1.65)) ;
#115916=CARTESIAN_POINT('',(7.9,-2.15,-1.65)) ;
#115917=CARTESIAN_POINT('',(1.4,-2.15,-1.65)) ;
#115918=CARTESIAN_POINT('',(7.9,1.9,-1.65)) ;
#115919=CARTESIAN_POINT('Origin',(1.4,-2.15,-1.55)) ;
#115920=CARTESIAN_POINT('',(1.5,-2.25,-1.55)) ;
#115921=CARTESIAN_POINT('Origin',(1.5,-2.15,-1.55)) ;
#115922=CARTESIAN_POINT('',(7.9,-2.25,-1.55)) ;
#115923=CARTESIAN_POINT('',(1.4,-2.25,-1.55)) ;
#115924=CARTESIAN_POINT('Origin',(7.9,-2.15,-1.55)) ;
#115925=CARTESIAN_POINT('Origin',(1.4,-2.25,-0.903119593409422)) ;
#115926=CARTESIAN_POINT('',(1.5,-2.25,-0.903119593409422)) ;
#115927=CARTESIAN_POINT('',(1.5,-2.25,-0.903119593409423)) ;
#115928=CARTESIAN_POINT('',(7.9,-2.25,-0.903119593409422)) ;
#115929=CARTESIAN_POINT('',(1.4,-2.25,-0.903119593409422)) ;
#115930=CARTESIAN_POINT('',(7.9,-2.25,-1.55)) ;
#115931=CARTESIAN_POINT('Origin',(1.4,-2.15,-0.903119593409422)) ;
#115932=CARTESIAN_POINT('',(1.5,-2.23576512455516,-0.851696413713512)) ;
#115933=CARTESIAN_POINT('Origin',(1.5,-2.15,-0.903119593409422)) ;
#115934=CARTESIAN_POINT('',(7.9,-2.23576512455516,-0.851696413713512)) ;
#115935=CARTESIAN_POINT('',(1.4,-2.23576512455516,-0.851696413713512)) ;
#115936=CARTESIAN_POINT('Origin',(7.9,-2.15,-0.903119593409422)) ;
#115937=CARTESIAN_POINT('Origin',(1.4,-3.65625,0.)) ;
#115938=CARTESIAN_POINT('',(1.5,-2.23576512455516,0.851696413713512)) ;
#115939=CARTESIAN_POINT('Origin',(1.5,-3.65625,0.)) ;
#115940=CARTESIAN_POINT('',(7.9,-2.23576512455516,0.851696413713512)) ;
#115941=CARTESIAN_POINT('',(1.4,-2.23576512455516,0.851696413713512)) ;
#115942=CARTESIAN_POINT('Origin',(7.9,-3.65625,0.)) ;
#115943=CARTESIAN_POINT('Origin',(1.4,-2.15,0.903119593409422)) ;
#115944=CARTESIAN_POINT('',(1.5,-2.25,0.903119593409422)) ;
#115945=CARTESIAN_POINT('Origin',(1.5,-2.15,0.903119593409422)) ;
#115946=CARTESIAN_POINT('',(7.9,-2.25,0.903119593409422)) ;
#115947=CARTESIAN_POINT('',(1.4,-2.25,0.903119593409422)) ;
#115948=CARTESIAN_POINT('Origin',(7.9,-2.15,0.903119593409422)) ;
#115949=CARTESIAN_POINT('Origin',(1.4,-2.25,1.55)) ;
#115950=CARTESIAN_POINT('',(1.5,-2.25,1.55)) ;
#115951=CARTESIAN_POINT('',(1.5,-2.25,1.55)) ;
#115952=CARTESIAN_POINT('',(7.9,-2.25,1.55)) ;
#115953=CARTESIAN_POINT('',(1.4,-2.25,1.55)) ;
#115954=CARTESIAN_POINT('',(7.9,-2.25,0.903119593409422)) ;
#115955=CARTESIAN_POINT('Origin',(1.4,-2.15,1.55)) ;
#115956=CARTESIAN_POINT('',(1.5,-2.15,1.65)) ;
#115957=CARTESIAN_POINT('Origin',(1.5,-2.15,1.55)) ;
#115958=CARTESIAN_POINT('',(7.9,-2.15,1.65)) ;
#115959=CARTESIAN_POINT('',(1.4,-2.15,1.65)) ;
#115960=CARTESIAN_POINT('Origin',(7.9,-2.15,1.55)) ;
#115961=CARTESIAN_POINT('Origin',(1.4,1.9,1.65)) ;
#115962=CARTESIAN_POINT('',(1.5,1.9,1.65)) ;
#115963=CARTESIAN_POINT('',(1.5,1.9,1.65)) ;
#115964=CARTESIAN_POINT('',(7.9,1.9,1.65)) ;
#115965=CARTESIAN_POINT('',(1.4,1.9,1.65)) ;
#115966=CARTESIAN_POINT('',(7.9,-2.15,1.65)) ;
#115967=CARTESIAN_POINT('Origin',(1.4,1.9,1.55)) ;
#115968=CARTESIAN_POINT('',(1.5,2.,1.55)) ;
#115969=CARTESIAN_POINT('Origin',(1.5,1.9,1.55)) ;
#115970=CARTESIAN_POINT('',(7.9,2.,1.55)) ;
#115971=CARTESIAN_POINT('',(1.4,2.,1.55)) ;
#115972=CARTESIAN_POINT('Origin',(7.9,1.9,1.55)) ;
#115973=CARTESIAN_POINT('Origin',(1.4,2.,1.55)) ;
#115974=CARTESIAN_POINT('',(1.5,2.,0.6)) ;
#115975=CARTESIAN_POINT('',(7.9,2.,1.55)) ;
#115976=CARTESIAN_POINT('Origin',(1.4,2.1,0.6)) ;
#115977=CARTESIAN_POINT('',(1.4,2.6,0.6)) ;
#115978=CARTESIAN_POINT('',(1.4,2.4,0.4)) ;
#115979=CARTESIAN_POINT('Origin',(1.4,2.4,0.6)) ;
#115980=CARTESIAN_POINT('',(1.4,2.1,0.4)) ;
#115981=CARTESIAN_POINT('',(1.4,2.1,0.4)) ;
#115982=CARTESIAN_POINT('',(1.4,1.9,0.6)) ;
#115983=CARTESIAN_POINT('Origin',(1.4,2.1,0.6)) ;
#115984=CARTESIAN_POINT('',(1.4,1.9,1.55)) ;
#115985=CARTESIAN_POINT('',(1.4,1.9,1.55)) ;
#115986=CARTESIAN_POINT('',(1.4,-2.15,1.55)) ;
#115987=CARTESIAN_POINT('',(1.4,-2.15,1.55)) ;
#115988=CARTESIAN_POINT('',(1.4,-2.15,0.903119593409422)) ;
#115989=CARTESIAN_POINT('',(1.4,-2.15,0.903119593409422)) ;
#115990=CARTESIAN_POINT('',(1.4,-2.15,-0.903119593409422)) ;
#115991=CARTESIAN_POINT('Origin',(1.4,-3.65625,0.)) ;
#115992=CARTESIAN_POINT('',(1.4,-2.15,-1.55)) ;
#115993=CARTESIAN_POINT('',(1.4,-2.15,-1.55)) ;
#115994=CARTESIAN_POINT('',(1.4,1.9,-1.55)) ;
#115995=CARTESIAN_POINT('',(1.4,1.9,-1.55)) ;
#115996=CARTESIAN_POINT('',(1.4,1.9,-0.6)) ;
#115997=CARTESIAN_POINT('',(1.4,1.9,-0.6)) ;
#115998=CARTESIAN_POINT('',(1.4,2.1,-0.4)) ;
#115999=CARTESIAN_POINT('Origin',(1.4,2.1,-0.6)) ;
#116000=CARTESIAN_POINT('',(1.4,2.4,-0.4)) ;
#116001=CARTESIAN_POINT('',(1.4,2.4,-0.4)) ;
#116002=CARTESIAN_POINT('',(1.4,2.6,-0.6)) ;
#116003=CARTESIAN_POINT('Origin',(1.4,2.4,-0.6)) ;
#116004=CARTESIAN_POINT('',(1.4,2.6,-0.70857864376269)) ;
#116005=CARTESIAN_POINT('',(1.4,2.6,-0.70857864376269)) ;
#116006=CARTESIAN_POINT('',(1.4,3.15,-1.25857864376269)) ;
#116007=CARTESIAN_POINT('',(1.4,3.15,-1.25857864376269)) ;
#116008=CARTESIAN_POINT('',(1.4,3.15,1.25857864376269)) ;
#116009=CARTESIAN_POINT('',(1.4,2.6,0.708578643762689)) ;
#116010=CARTESIAN_POINT('',(1.4,2.6,0.708578643762689)) ;
#116011=CARTESIAN_POINT('',(1.4,2.6,0.6)) ;
#116012=CARTESIAN_POINT('Origin',(2.4,0.,0.)) ;
#116013=CARTESIAN_POINT('',(2.4,0.3,0.4)) ;
#116014=CARTESIAN_POINT('',(2.4,-0.3,0.4)) ;
#116015=CARTESIAN_POINT('',(2.4,0.,0.4)) ;
#116016=CARTESIAN_POINT('',(2.4,0.4,0.3)) ;
#116017=CARTESIAN_POINT('Origin',(2.4,0.3,0.3)) ;
#116018=CARTESIAN_POINT('',(2.4,0.4,-0.3)) ;
#116019=CARTESIAN_POINT('',(2.4,0.4,0.)) ;
#116020=CARTESIAN_POINT('',(2.4,0.3,-0.4)) ;
#116021=CARTESIAN_POINT('Origin',(2.4,0.3,-0.3)) ;
#116022=CARTESIAN_POINT('',(2.4,-0.3,-0.4)) ;
#116023=CARTESIAN_POINT('',(2.4,0.,-0.4)) ;
#116024=CARTESIAN_POINT('',(2.4,-0.4,-0.3)) ;
#116025=CARTESIAN_POINT('Origin',(2.4,-0.3,-0.3)) ;
#116026=CARTESIAN_POINT('',(2.4,-0.4,0.3)) ;
#116027=CARTESIAN_POINT('',(2.4,-0.4,0.)) ;
#116028=CARTESIAN_POINT('Origin',(2.4,-0.3,0.3)) ;
#116029=CARTESIAN_POINT('Origin',(-0.899999999999999,-2.,0.6)) ;
#116030=CARTESIAN_POINT('Origin',(-0.899999999999999,0.4,0.6)) ;
#116031=CARTESIAN_POINT('Origin',(-0.899999999999999,-1.9,0.6)) ;
#116032=CARTESIAN_POINT('Origin',(0.600000000000001,0.4,0.4)) ;
#116033=CARTESIAN_POINT('Origin',(0.500000000000001,0.4,0.4)) ;
#116034=CARTESIAN_POINT('Origin',(-0.899999999999999,0.4,0.4)) ;
#116035=CARTESIAN_POINT('Origin',(0.500000000000001,0.4,0.4)) ;
#116036=CARTESIAN_POINT('',(0.600000000000001,0.4,0.4)) ;
#116037=CARTESIAN_POINT('Origin',(0.500000000000001,0.4,0.4)) ;
#116038=CARTESIAN_POINT('Origin',(0.500000000000001,0.4,0.4)) ;
#116039=CARTESIAN_POINT('Origin',(-0.899999999999999,-1.9,0.6)) ;
#116040=CARTESIAN_POINT('Origin',(-0.899999999999999,-1.9,0.6)) ;
#116041=CARTESIAN_POINT('Origin',(-0.899999999999999,-1.9,0.6)) ;
#116042=CARTESIAN_POINT('Origin',(-0.899999999999999,0.4,0.4)) ;
#116043=CARTESIAN_POINT('Origin',(-0.899999999999999,0.6,0.4)) ;
#116044=CARTESIAN_POINT('Origin',(0.500000000000001,0.4,0.)) ;
#116045=CARTESIAN_POINT('Origin',(0.500000000000001,0.4,-0.4)) ;
#116046=CARTESIAN_POINT('',(0.600000000000001,0.4,-0.3)) ;
#116047=CARTESIAN_POINT('Ctrl Pts',(0.595612997216081,0.370705721320403,
-0.370705721320403)) ;
#116048=CARTESIAN_POINT('Ctrl Pts',(0.596180587760892,0.372558268494357,
-0.368855498832167)) ;
#116049=CARTESIAN_POINT('Ctrl Pts',(0.596672461925686,0.374355839771985,
-0.36691417986631)) ;
#116050=CARTESIAN_POINT('Ctrl Pts',(0.599015141889212,0.383869350930065,
-0.355764993656267)) ;
#116051=CARTESIAN_POINT('Ctrl Pts',(0.599609996542525,0.390224332900451,
-0.34497260265412)) ;
#116052=CARTESIAN_POINT('Ctrl Pts',(0.600050586298726,0.398117439141561,
-0.32233105320467)) ;
#116053=CARTESIAN_POINT('Ctrl Pts',(0.600000000000001,0.399999999999999,
-0.311201250633524)) ;
#116054=CARTESIAN_POINT('Ctrl Pts',(0.600000000000001,0.399999999999999,
-0.3)) ;
#116055=CARTESIAN_POINT('',(0.600000000000001,0.4,0.)) ;
#116056=CARTESIAN_POINT('Origin',(0.500000000000001,-4.5664044441154E-17,
0.4)) ;
#116057=CARTESIAN_POINT('',(0.500000000000001,0.394987437106619,0.3)) ;
#116058=CARTESIAN_POINT('Ctrl Pts',(0.500000000000001,0.394987437106619,
0.3)) ;
#116059=CARTESIAN_POINT('Ctrl Pts',(0.505940567948951,0.3955844866499,0.3)) ;
#116060=CARTESIAN_POINT('Ctrl Pts',(0.511931971019139,0.396132036079018,
0.300533699672039)) ;
#116061=CARTESIAN_POINT('Ctrl Pts',(0.517829015308548,0.396618246075354,
0.301602204226276)) ;
#116062=CARTESIAN_POINT('Ctrl Pts',(0.522982218721202,0.397043126556053,
0.30253592984289)) ;
#116063=CARTESIAN_POINT('Ctrl Pts',(0.528062648970231,0.397421319341388,
0.303877173202936)) ;
#116064=CARTESIAN_POINT('Ctrl Pts',(0.532978106724001,0.397751505046071,
0.305594256123367)) ;
#116065=CARTESIAN_POINT('Ctrl Pts',(0.538583536338965,0.398128038182999,
0.307552362150451)) ;
#116066=CARTESIAN_POINT('Ctrl Pts',(0.544059405914892,0.398447721828296,
0.310029991688954)) ;
#116067=CARTESIAN_POINT('Ctrl Pts',(0.549268572255782,0.398712331108984,
0.312979268057107)) ;
#116068=CARTESIAN_POINT('Ctrl Pts',(0.553856850427146,0.398945401221756,
0.315577015853159)) ;
#116069=CARTESIAN_POINT('Ctrl Pts',(0.558237825069326,0.399135987683843,
0.318539615020013)) ;
#116070=CARTESIAN_POINT('Ctrl Pts',(0.562333836086213,0.399290378266507,
0.32180477713583)) ;
#116071=CARTESIAN_POINT('Ctrl Pts',(0.566990328957893,0.399465895042381,
0.325516731047696)) ;
#116072=CARTESIAN_POINT('Ctrl Pts',(0.571349096493423,0.399597278936107,
0.329677193515201)) ;
#116073=CARTESIAN_POINT('Ctrl Pts',(0.575296920056712,0.399694832180837,
0.334194424020656)) ;
#116074=CARTESIAN_POINT('Ctrl Pts',(0.578744263667908,0.399780018245913,
0.338138988784921)) ;
#116075=CARTESIAN_POINT('Ctrl Pts',(0.58187831456043,0.399839626289636,
0.342354478157894)) ;
#116076=CARTESIAN_POINT('Ctrl Pts',(0.584648147334856,0.399882153365958,
0.346758182292707)) ;
#116077=CARTESIAN_POINT('Ctrl Pts',(0.587839270208173,0.399931148788079,
0.351831687495501)) ;
#116078=CARTESIAN_POINT('Ctrl Pts',(0.590595054415093,0.399958289583404,
0.357233363755549)) ;
#116079=CARTESIAN_POINT('Ctrl Pts',(0.592838618943104,0.399974357003159,
0.362838314990607)) ;
#116080=CARTESIAN_POINT('Ctrl Pts',(0.594777336851655,0.399988241245861,
0.367681687757603)) ;
#116081=CARTESIAN_POINT('Ctrl Pts',(0.596334051506189,0.399993946552814,
0.372675833772872)) ;
#116082=CARTESIAN_POINT('Ctrl Pts',(0.597488309822308,0.39999684570125,
0.377728281431604)) ;
#116083=CARTESIAN_POINT('Ctrl Pts',(0.598804024094401,0.400000150378306,
0.383487458039442)) ;
#116084=CARTESIAN_POINT('Ctrl Pts',(0.599612685195431,0.399999963509465,
0.389397156109403)) ;
#116085=CARTESIAN_POINT('Ctrl Pts',(0.599890230999721,0.399999993975383,
0.395315797738928)) ;
#116086=CARTESIAN_POINT('Ctrl Pts',(0.5999634645494,0.400000002014155,0.396877497210183)) ;
#116087=CARTESIAN_POINT('Ctrl Pts',(0.600000000000001,0.399999999999999,
0.398439778490821)) ;
#116088=CARTESIAN_POINT('Ctrl Pts',(0.600000000000001,0.399999999999999,
0.4)) ;
#116089=CARTESIAN_POINT('',(0.600000000000001,0.299999999999999,0.4)) ;
#116090=CARTESIAN_POINT('Ctrl Pts',(0.500000000000001,0.394987437106619,
0.3)) ;
#116091=CARTESIAN_POINT('Ctrl Pts',(0.500454935589698,0.395033159853734,
0.3)) ;
#116092=CARTESIAN_POINT('Ctrl Pts',(0.500909898680399,0.395078570329052,
0.300003104508874)) ;
#116093=CARTESIAN_POINT('Ctrl Pts',(0.502892456245148,0.395275075889088,
0.300030166058056)) ;
#116094=CARTESIAN_POINT('Ctrl Pts',(0.504418747482362,0.395422812032197,
0.300086014579005)) ;
#116095=CARTESIAN_POINT('Ctrl Pts',(0.508462199543372,0.395804395682036,
0.300326718943359)) ;
#116096=CARTESIAN_POINT('Ctrl Pts',(0.510974953343318,0.396031485023319,
0.300572060854946)) ;
#116097=CARTESIAN_POINT('Ctrl Pts',(0.521160739721334,0.396903453186241,
0.301957205508451)) ;
#116098=CARTESIAN_POINT('Ctrl Pts',(0.528708678528457,0.397444933153163,
0.303895782295333)) ;
#116099=CARTESIAN_POINT('Ctrl Pts',(0.54594320635814,0.398105551684111,
0.310535360548881)) ;
#116100=CARTESIAN_POINT('Ctrl Pts',(0.555229535466871,0.397987646678423,
0.315964641164077)) ;
#116101=CARTESIAN_POINT('Ctrl Pts',(0.571394604995807,0.395490482808029,
0.329224486636193)) ;
#116102=CARTESIAN_POINT('Ctrl Pts',(0.578055313702881,0.393198948698321,
0.336759254368297)) ;
#116103=CARTESIAN_POINT('Ctrl Pts',(0.58855913220255,0.385442756729278,
0.352607766016028)) ;
#116104=CARTESIAN_POINT('Ctrl Pts',(0.592167355639995,0.380240075126846,
0.360451734393248)) ;
#116105=CARTESIAN_POINT('Ctrl Pts',(0.597496615531129,0.365892753466911,
0.376074478204782)) ;
#116106=CARTESIAN_POINT('Ctrl Pts',(0.598734255154207,0.356660564300593,
0.38322725827313)) ;
#116107=CARTESIAN_POINT('Ctrl Pts',(0.600012754681692,0.335223914398488,
0.394417694134416)) ;
#116108=CARTESIAN_POINT('Ctrl Pts',(0.59999390055981,0.32265503709182,0.398338480634425)) ;
#116109=CARTESIAN_POINT('Ctrl Pts',(0.600000296204999,0.306106913582345,
0.399860373652956)) ;
#116110=CARTESIAN_POINT('Ctrl Pts',(0.600000000000001,0.303050992413431,
0.4)) ;
#116111=CARTESIAN_POINT('Ctrl Pts',(0.600000000000001,0.299999999999999,
0.4)) ;
#116112=CARTESIAN_POINT('',(0.600000000000001,-2.3980000991444E-17,0.4)) ;
#116113=CARTESIAN_POINT('Origin',(0.500000000000001,-1.9,0.4)) ;
#116114=CARTESIAN_POINT('Origin',(0.600000000000001,-1.9,0.6)) ;
#116115=CARTESIAN_POINT('Origin',(0.500000000000001,-1.9,0.6)) ;
#116116=CARTESIAN_POINT('Origin',(-0.899999999999999,-1.9,1.375)) ;
#116117=CARTESIAN_POINT('Origin',(-0.899999999999999,-1.9,1.275)) ;
#116118=CARTESIAN_POINT('Origin',(-0.899999999999999,0.6,0.5)) ;
#116119=CARTESIAN_POINT('Origin',(-0.899999999999999,0.6,-0.4)) ;
#116120=CARTESIAN_POINT('Origin',(0.600000000000001,0.4,-0.4)) ;
#116121=CARTESIAN_POINT('Origin',(0.500000000000001,0.4,-0.4)) ;
#116122=CARTESIAN_POINT('Origin',(-0.899999999999999,0.4,-0.4)) ;
#116123=CARTESIAN_POINT('Origin',(0.500000000000001,0.4,-0.4)) ;
#116124=CARTESIAN_POINT('Origin',(0.500000000000001,-1.9,0.6)) ;
#116125=CARTESIAN_POINT('Origin',(0.500000000000001,-2.1,0.6)) ;
#116126=CARTESIAN_POINT('Origin',(-0.899999999999999,-1.9,1.275)) ;
#116127=CARTESIAN_POINT('Origin',(-1.1,-1.9,1.275)) ;
#116128=CARTESIAN_POINT('Origin',(-0.899999999999999,-2.1,1.275)) ;
#116129=CARTESIAN_POINT('Origin',(-0.899999999999999,0.4,-0.4)) ;
#116130=CARTESIAN_POINT('Origin',(-0.899999999999999,0.4,-0.6)) ;
#116131=CARTESIAN_POINT('Origin',(0.500000000000001,-2.1,0.)) ;
#116132=CARTESIAN_POINT('Origin',(0.500000000000001,-2.1,1.275)) ;
#116133=CARTESIAN_POINT('Origin',(0.600000000000001,-2.1,1.275)) ;
#116134=CARTESIAN_POINT('Origin',(0.500000000000001,-2.1,1.275)) ;
#116135=CARTESIAN_POINT('Origin',(-1.1,-4.42727195005762E-17,1.275)) ;
#116136=CARTESIAN_POINT('',(-1.1,1.15,1.375)) ;
#116137=CARTESIAN_POINT('',(-1.1,1.25,1.375)) ;
#116138=CARTESIAN_POINT('Origin',(-1.1,1.15,1.275)) ;
#116139=CARTESIAN_POINT('Origin',(-0.899999999999999,0.5,-0.6)) ;
#116140=CARTESIAN_POINT('Origin',(-0.899999999999999,-1.9,-0.6)) ;
#116141=CARTESIAN_POINT('Origin',(0.600000000000001,-1.9,-0.6)) ;
#116142=CARTESIAN_POINT('Origin',(0.500000000000001,-1.9,-0.6)) ;
#116143=CARTESIAN_POINT('Origin',(-0.899999999999999,-1.9,-0.6)) ;
#116144=CARTESIAN_POINT('Origin',(0.500000000000001,-1.9,-0.6)) ;
#116145=CARTESIAN_POINT('Origin',(0.500000000000001,-2.1,-0.6)) ;
#116146=CARTESIAN_POINT('Origin',(0.500000000000001,-2.1,1.275)) ;
#116147=CARTESIAN_POINT('Origin',(0.500000000000001,-2.1,1.275)) ;
#116148=CARTESIAN_POINT('Origin',(-1.1,-2.9,1.475)) ;
#116149=CARTESIAN_POINT('Origin',(-1.1,-2.9,1.475)) ;
#116150=CARTESIAN_POINT('Origin',(-1.1,-2.9,1.475)) ;
#116151=CARTESIAN_POINT('Origin',(-1.1,1.25,1.475)) ;
#116152=CARTESIAN_POINT('Origin',(-1.1,1.15,1.475)) ;
#116153=CARTESIAN_POINT('Origin',(-1.1,1.15,1.275)) ;
#116154=CARTESIAN_POINT('',(-1.1,1.25,1.275)) ;
#116155=CARTESIAN_POINT('Origin',(-1.1,1.15,1.275)) ;
#116156=CARTESIAN_POINT('Origin',(-1.1,1.15,1.275)) ;
#116157=CARTESIAN_POINT('Origin',(-0.899999999999999,-1.9,-0.6)) ;
#116158=CARTESIAN_POINT('Origin',(-0.899999999999999,-1.9,-0.6)) ;
#116159=CARTESIAN_POINT('Origin',(0.500000000000001,-2.1,0.)) ;
#116160=CARTESIAN_POINT('Origin',(0.500000000000001,-2.1,-1.275)) ;
#116161=CARTESIAN_POINT('Origin',(0.500000000000001,1.36481920536411E-16,
1.275)) ;
#116162=CARTESIAN_POINT('Origin',(0.500000000000001,-2.9,1.275)) ;
#116163=CARTESIAN_POINT('Origin',(-0.999999999999999,-2.9,1.475)) ;
#116164=CARTESIAN_POINT('Origin',(0.500000000000001,-2.9,1.475)) ;
#116165=CARTESIAN_POINT('Origin',(-1.1,1.15,1.275)) ;
#116166=CARTESIAN_POINT('Origin',(-1.1,1.35,1.275)) ;
#116167=CARTESIAN_POINT('Origin',(-1.1,1.15,0.)) ;
#116168=CARTESIAN_POINT('',(-1.1,1.25,-1.275)) ;
#116169=CARTESIAN_POINT('',(-1.1,1.25,-1.375)) ;
#116170=CARTESIAN_POINT('Origin',(-1.1,1.15,-1.275)) ;
#116171=CARTESIAN_POINT('Origin',(-0.899999999999999,-1.9,-0.5)) ;
#116172=CARTESIAN_POINT('Origin',(-0.899999999999999,-1.9,-1.275)) ;
#116173=CARTESIAN_POINT('Origin',(-0.999999999999999,-2.1,-1.275)) ;
#116174=CARTESIAN_POINT('Origin',(0.500000000000001,-2.1,-1.275)) ;
#116175=CARTESIAN_POINT('Origin',(-0.899999999999999,-2.1,-1.275)) ;
#116176=CARTESIAN_POINT('Origin',(0.500000000000001,-2.1,-1.275)) ;
#116177=CARTESIAN_POINT('Origin',(0.500000000000001,-2.1,-1.275)) ;
#116178=CARTESIAN_POINT('Origin',(0.500000000000001,-2.9,1.275)) ;
#116179=CARTESIAN_POINT('Origin',(0.700000000000002,-2.9,1.275)) ;
#116180=CARTESIAN_POINT('Origin',(-1.1,1.35,-1.375)) ;
#116181=CARTESIAN_POINT('Origin',(-1.1,1.35,-1.275)) ;
#116182=CARTESIAN_POINT('Origin',(-1.1,1.15,-1.275)) ;
#116183=CARTESIAN_POINT('',(-1.1,1.15,-1.375)) ;
#116184=CARTESIAN_POINT('Origin',(-1.1,1.15,-1.275)) ;
#116185=CARTESIAN_POINT('Origin',(-1.1,1.15,-1.275)) ;
#116186=CARTESIAN_POINT('Origin',(-0.899999999999999,-1.9,-1.275)) ;
#116187=CARTESIAN_POINT('Origin',(-1.1,-1.9,-1.275)) ;
#116188=CARTESIAN_POINT('Origin',(0.500000000000001,-5.86744705109801E-17,
-1.275)) ;
#116189=CARTESIAN_POINT('Origin',(0.500000000000001,-2.9,-1.275)) ;
#116190=CARTESIAN_POINT('Origin',(0.700000000000002,-2.9,0.)) ;
#116191=CARTESIAN_POINT('Origin',(0.700000000000002,-2.9,-1.275)) ;
#116192=CARTESIAN_POINT('Origin',(-1.1,1.15,-1.275)) ;
#116193=CARTESIAN_POINT('Origin',(-1.1,1.15,-1.475)) ;
#116194=CARTESIAN_POINT('Origin',(-1.1,-2.39429110547967E-16,-1.275)) ;
#116195=CARTESIAN_POINT('',(-1.1,1.25,-1.375)) ;
#116196=CARTESIAN_POINT('Origin',(0.500000000000001,-2.9,-1.275)) ;
#116197=CARTESIAN_POINT('Origin',(0.500000000000001,-2.9,-1.475)) ;
#116198=CARTESIAN_POINT('Origin',(-1.1,1.25,-1.475)) ;
#116199=CARTESIAN_POINT('Origin',(-1.1,-2.9,-1.475)) ;
#116200=CARTESIAN_POINT('Origin',(-1.1,-2.9,-1.475)) ;
#116201=CARTESIAN_POINT('Origin',(-1.1,-2.9,-1.475)) ;
#116202=CARTESIAN_POINT('Origin',(-1.1,-2.9,-1.475)) ;
#116203=CARTESIAN_POINT('Origin',(4.55,4.55,-36.79)) ;
#116204=CARTESIAN_POINT('Origin',(4.55,4.55,-36.79)) ;
#116205=CARTESIAN_POINT('Origin',(4.55,4.55,-36.79)) ;
#116206=CARTESIAN_POINT('Origin',(4.55,4.55,-36.79)) ;
#116207=CARTESIAN_POINT('Origin',(4.55,4.35,-36.79)) ;
#116208=CARTESIAN_POINT('Origin',(4.75,4.55,-36.79)) ;
#116209=CARTESIAN_POINT('Origin',(4.75,4.55,-36.79)) ;
#116210=CARTESIAN_POINT('Origin',(4.35,4.35,-36.79)) ;
#116211=CARTESIAN_POINT('Origin',(4.35,4.15,-36.79)) ;
#116212=CARTESIAN_POINT('Origin',(4.75,4.55,-36.79)) ;
#116213=CARTESIAN_POINT('Origin',(4.75,4.55,-36.79)) ;
#116214=CARTESIAN_POINT('Origin',(-1.1,4.15,-36.79)) ;
#116215=CARTESIAN_POINT('Origin',(-1.1,4.15,-36.79)) ;
#116216=CARTESIAN_POINT('Origin',(4.75,4.35,-36.79)) ;
#116217=CARTESIAN_POINT('Origin',(4.75,4.35,-36.79)) ;
#116218=CARTESIAN_POINT('Origin',(-1.1,4.15,-36.79)) ;
#116219=CARTESIAN_POINT('Origin',(-1.1,4.15,-36.79)) ;
#116220=CARTESIAN_POINT('Origin',(4.95,4.35,-36.79)) ;
#116221=CARTESIAN_POINT('Origin',(4.95,4.15,-36.79)) ;
#116222=CARTESIAN_POINT('Origin',(-1.1,4.15,-36.79)) ;
#116223=CARTESIAN_POINT('Origin',(-1.1,-2.9,-36.79)) ;
#116224=CARTESIAN_POINT('Origin',(4.95,4.15,-36.79)) ;
#116225=CARTESIAN_POINT('Origin',(7.9,4.15,-36.79)) ;
#116226=CARTESIAN_POINT('Origin',(-1.1,-2.9,-36.79)) ;
#116227=CARTESIAN_POINT('Origin',(-1.1,-2.9,-36.79)) ;
#116228=CARTESIAN_POINT('Origin',(7.9,4.15,-36.79)) ;
#116229=CARTESIAN_POINT('Origin',(7.9,4.15,-36.79)) ;
#116230=CARTESIAN_POINT('Origin',(-1.1,-2.9,-36.79)) ;
#116231=CARTESIAN_POINT('Origin',(7.9,-2.9,-36.79)) ;
#116232=CARTESIAN_POINT('Origin',(7.9,4.15,-36.79)) ;
#116233=CARTESIAN_POINT('Origin',(7.9,-2.9,-36.79)) ;
#116234=CARTESIAN_POINT('Origin',(7.9,-2.9,-36.79)) ;
#116235=CARTESIAN_POINT('Origin',(4.55,4.55,2.5)) ;
#116236=CARTESIAN_POINT('Origin',(4.55,4.55,2.5)) ;
#116237=CARTESIAN_POINT('Origin',(4.55,4.55,2.5)) ;
#116238=CARTESIAN_POINT('Origin',(4.55,-2.9,2.5)) ;
#116239=CARTESIAN_POINT('Origin',(4.55,4.35,2.5)) ;
#116240=CARTESIAN_POINT('Origin',(7.9,4.55,2.5)) ;
#116241=CARTESIAN_POINT('Origin',(4.75,4.55,2.5)) ;
#116242=CARTESIAN_POINT('Origin',(4.35,4.35,2.5)) ;
#116243=CARTESIAN_POINT('Origin',(4.35,4.15,2.5)) ;
#116244=CARTESIAN_POINT('Origin',(4.75,4.55,2.5)) ;
#116245=CARTESIAN_POINT('Origin',(4.75,4.55,2.5)) ;
#116246=CARTESIAN_POINT('Origin',(7.9,4.15,2.5)) ;
#116247=CARTESIAN_POINT('Origin',(-1.1,4.15,2.5)) ;
#116248=CARTESIAN_POINT('Origin',(4.74999999999997,-2.89999999999999,2.5)) ;
#116249=CARTESIAN_POINT('Origin',(4.75,4.35,2.5)) ;
#116250=CARTESIAN_POINT('Origin',(-1.1,4.15,2.5)) ;
#116251=CARTESIAN_POINT('Origin',(-1.1,4.15,2.5)) ;
#116252=CARTESIAN_POINT('Origin',(4.95,4.35,2.5)) ;
#116253=CARTESIAN_POINT('Origin',(4.95,4.15,2.5)) ;
#116254=CARTESIAN_POINT('Origin',(-1.1,-2.9,2.5)) ;
#116255=CARTESIAN_POINT('Origin',(-1.1,-2.9,2.5)) ;
#116256=CARTESIAN_POINT('Origin',(7.9,4.15,2.5)) ;
#116257=CARTESIAN_POINT('Origin',(7.9,4.15,2.5)) ;
#116258=CARTESIAN_POINT('Origin',(-1.1,-2.9,2.5)) ;
#116259=CARTESIAN_POINT('Origin',(-1.1,-2.9,2.5)) ;
#116260=CARTESIAN_POINT('Origin',(7.9,4.15,2.5)) ;
#116261=CARTESIAN_POINT('Origin',(7.9,4.15,2.5)) ;
#116262=CARTESIAN_POINT('Origin',(7.9,-2.9,2.5)) ;
#116263=CARTESIAN_POINT('Origin',(7.9,-2.9,2.5)) ;
#116264=CARTESIAN_POINT('Origin',(7.9,-2.9,2.5)) ;
#116265=CARTESIAN_POINT('Origin',(7.9,-2.9,2.5)) ;
#116266=CARTESIAN_POINT('Origin',(7.9,-2.9,2.5)) ;
#116267=CARTESIAN_POINT('Origin',(1.5,1.9,0.6)) ;
#116268=CARTESIAN_POINT('Origin',(1.5,1.9,-1.55)) ;
#116269=CARTESIAN_POINT('Origin',(1.5,1.9,-0.6)) ;
#116270=CARTESIAN_POINT('Origin',(1.5,2.1,-0.6)) ;
#116271=CARTESIAN_POINT('Origin',(1.5,2.1,-0.4)) ;
#116272=CARTESIAN_POINT('Origin',(1.5,1.9,-1.55)) ;
#116273=CARTESIAN_POINT('Origin',(1.5,1.9,-1.55)) ;
#116274=CARTESIAN_POINT('Origin',(1.5,2.1,-0.4)) ;
#116275=CARTESIAN_POINT('Origin',(1.5,2.4,-0.4)) ;
#116276=CARTESIAN_POINT('Origin',(1.5,2.1,-1.55)) ;
#116277=CARTESIAN_POINT('Origin',(1.5,-2.15,-1.55)) ;
#116278=CARTESIAN_POINT('Origin',(1.5,2.4,-0.6)) ;
#116279=CARTESIAN_POINT('Origin',(1.5,2.6,-0.6)) ;
#116280=CARTESIAN_POINT('Origin',(1.5,-2.15,-1.55)) ;
#116281=CARTESIAN_POINT('Origin',(1.5,-2.15,-1.55)) ;
#116282=CARTESIAN_POINT('Origin',(1.5,2.6,0.6)) ;
#116283=CARTESIAN_POINT('Origin',(1.5,2.6,-0.70857864376269)) ;
#116284=CARTESIAN_POINT('Origin',(1.5,-2.15,0.6)) ;
#116285=CARTESIAN_POINT('Origin',(1.5,-2.15,-0.903119593409422)) ;
#116286=CARTESIAN_POINT('Origin',(1.5,2.6,-0.70857864376269)) ;
#116287=CARTESIAN_POINT('Origin',(1.5,2.6,-0.70857864376269)) ;
#116288=CARTESIAN_POINT('Origin',(1.5,-2.15,-0.903119593409422)) ;
#116289=CARTESIAN_POINT('Origin',(1.5,-2.15,-0.903119593409422)) ;
#116290=CARTESIAN_POINT('Origin',(1.5,1.69571067811865,0.195710678118654)) ;
#116291=CARTESIAN_POINT('Origin',(1.5,3.15,-1.25857864376269)) ;
#116292=CARTESIAN_POINT('Origin',(1.5,-3.65625,0.)) ;
#116293=CARTESIAN_POINT('Origin',(1.5,-2.15,0.903119593409423)) ;
#116294=CARTESIAN_POINT('Origin',(1.5,3.15,-1.25857864376269)) ;
#116295=CARTESIAN_POINT('Origin',(1.5,3.15,-1.25857864376269)) ;
#116296=CARTESIAN_POINT('Origin',(1.5,-2.15,0.903119593409422)) ;
#116297=CARTESIAN_POINT('Origin',(1.5,-2.15,0.903119593409422)) ;
#116298=CARTESIAN_POINT('Origin',(1.5,3.15,0.6)) ;
#116299=CARTESIAN_POINT('Origin',(1.5,-2.15,0.6)) ;
#116300=CARTESIAN_POINT('Origin',(1.5,-2.15,1.55)) ;
#116301=CARTESIAN_POINT('Origin',(1.5,-2.15,1.55)) ;
#116302=CARTESIAN_POINT('Origin',(1.5,-2.15,1.55)) ;
#116303=CARTESIAN_POINT('Origin',(1.5,2.29571067811866,0.404289321881344)) ;
#116304=CARTESIAN_POINT('Origin',(1.5,2.6,0.708578643762689)) ;
#116305=CARTESIAN_POINT('Origin',(1.5,2.1,1.55)) ;
#116306=CARTESIAN_POINT('Origin',(1.5,1.9,1.55)) ;
#116307=CARTESIAN_POINT('Origin',(1.5,2.6,0.70857864376269)) ;
#116308=CARTESIAN_POINT('Origin',(1.5,2.6,0.70857864376269)) ;
#116309=CARTESIAN_POINT('Origin',(1.5,1.9,1.55)) ;
#116310=CARTESIAN_POINT('Origin',(1.5,1.9,1.55)) ;
#116311=CARTESIAN_POINT('Origin',(1.5,2.6,0.599999999999998)) ;
#116312=CARTESIAN_POINT('Origin',(1.5,2.6,0.6)) ;
#116313=CARTESIAN_POINT('Origin',(1.5,1.9,0.6)) ;
#116314=CARTESIAN_POINT('Origin',(1.5,1.9,0.6)) ;
#116315=CARTESIAN_POINT('Origin',(1.5,2.4,0.6)) ;
#116316=CARTESIAN_POINT('Origin',(1.5,2.4,0.4)) ;
#116317=CARTESIAN_POINT('Origin',(1.5,2.1,0.6)) ;
#116318=CARTESIAN_POINT('Origin',(1.5,2.1,0.4)) ;
#116319=CARTESIAN_POINT('Origin',(1.5,2.1,0.4)) ;
#116320=CARTESIAN_POINT('Origin',(7.9,2.1,-0.6)) ;
#116321=CARTESIAN_POINT('Origin',(7.9,2.4,-0.6)) ;
#116322=CARTESIAN_POINT('Origin',(7.9,2.1,-0.6)) ;
#116323=CARTESIAN_POINT('Origin',(7.9,2.4,-0.6)) ;
#116324=CARTESIAN_POINT('Origin',(7.9,2.4,-0.6)) ;
#116325=CARTESIAN_POINT('Origin',(7.9,2.1,-0.6)) ;
#116326=CARTESIAN_POINT('Origin',(7.9,2.1,-0.6)) ;
#116327=CARTESIAN_POINT('Origin',(7.9,2.4,-0.6)) ;
#116328=CARTESIAN_POINT('Origin',(7.9,2.4,-0.70857864376269)) ;
#116329=CARTESIAN_POINT('Origin',(7.9,2.1,-0.6)) ;
#116330=CARTESIAN_POINT('Origin',(7.9,2.1,-1.55)) ;
#116331=CARTESIAN_POINT('Origin',(7.9,2.6,-0.70857864376269)) ;
#116332=CARTESIAN_POINT('Origin',(7.9,2.45857864376269,-0.85)) ;
#116333=CARTESIAN_POINT('Origin',(7.9,1.9,-1.55)) ;
#116334=CARTESIAN_POINT('Origin',(7.9,1.9,-1.75)) ;
#116335=CARTESIAN_POINT('Origin',(7.9,2.45857864376269,-0.85)) ;
#116336=CARTESIAN_POINT('Origin',(7.9,1.9,-1.75)) ;
#116337=CARTESIAN_POINT('Origin',(7.9,-2.15,-1.75)) ;
#116338=CARTESIAN_POINT('Origin',(7.9,-2.15,-1.55)) ;
#116339=CARTESIAN_POINT('Origin',(7.9,-2.35,-1.55)) ;
#116340=CARTESIAN_POINT('Origin',(7.9,3.35,-1.25857864376269)) ;
#116341=CARTESIAN_POINT('Origin',(7.9,3.35,1.25857864376269)) ;
#116342=CARTESIAN_POINT('Origin',(7.9,-2.35,-0.903119593409422)) ;
#116343=CARTESIAN_POINT('Origin',(7.9,-2.35,-0.903119593409422)) ;
#116344=CARTESIAN_POINT('Origin',(7.9,3.15,1.25857864376269)) ;
#116345=CARTESIAN_POINT('Origin',(7.9,3.00857864376269,1.4)) ;
#116346=CARTESIAN_POINT('Origin',(7.9,-2.15,-0.903119593409422)) ;
#116347=CARTESIAN_POINT('Origin',(7.9,-2.32153024911032,-0.800273234017602)) ;
#116348=CARTESIAN_POINT('Origin',(7.9,3.00857864376269,1.4)) ;
#116349=CARTESIAN_POINT('Origin',(7.9,2.45857864376269,0.849999999999999)) ;
#116350=CARTESIAN_POINT('Origin',(7.9,-3.65625,0.)) ;
#116351=CARTESIAN_POINT('Origin',(7.9,-2.32153024911032,0.800273234017602)) ;
#116352=CARTESIAN_POINT('Origin',(7.9,2.6,0.70857864376269)) ;
#116353=CARTESIAN_POINT('Origin',(7.9,2.4,0.70857864376269)) ;
#116354=CARTESIAN_POINT('Origin',(7.9,-2.15,0.903119593409422)) ;
#116355=CARTESIAN_POINT('Origin',(7.9,-2.35,0.903119593409422)) ;
#116356=CARTESIAN_POINT('Origin',(7.9,2.4,0.70857864376269)) ;
#116357=CARTESIAN_POINT('Origin',(7.9,2.4,0.600000000000001)) ;
#116358=CARTESIAN_POINT('Origin',(7.9,-2.35,1.55)) ;
#116359=CARTESIAN_POINT('Origin',(7.9,-2.35,1.55)) ;
#116360=CARTESIAN_POINT('Origin',(7.9,2.4,0.6)) ;
#116361=CARTESIAN_POINT('Origin',(7.9,2.4,0.6)) ;
#116362=CARTESIAN_POINT('Origin',(7.9,-2.15,1.55)) ;
#116363=CARTESIAN_POINT('Origin',(7.9,-2.15,1.75)) ;
#116364=CARTESIAN_POINT('Origin',(7.9,2.4,0.6)) ;
#116365=CARTESIAN_POINT('Origin',(7.9,2.1,0.6)) ;
#116366=CARTESIAN_POINT('Origin',(7.9,1.9,1.75)) ;
#116367=CARTESIAN_POINT('Origin',(7.9,1.9,1.75)) ;
#116368=CARTESIAN_POINT('Origin',(7.9,2.1,0.6)) ;
#116369=CARTESIAN_POINT('Origin',(7.9,2.1,0.6)) ;
#116370=CARTESIAN_POINT('Origin',(7.9,1.9,1.55)) ;
#116371=CARTESIAN_POINT('Origin',(7.9,2.1,1.55)) ;
#116372=CARTESIAN_POINT('Origin',(7.9,2.1,1.55)) ;
#116373=CARTESIAN_POINT('Origin',(-0.4,-0.600000000000001,0.4)) ;
#116374=CARTESIAN_POINT('',(-0.4,-0.600000000000001,0.3)) ;
#116375=CARTESIAN_POINT('',(-0.4,-0.600000000000001,-0.3)) ;
#116376=CARTESIAN_POINT('',(-0.4,-0.600000000000001,0.4)) ;
#116377=CARTESIAN_POINT('',(-0.4,-6.05857864376269,-0.3)) ;
#116378=CARTESIAN_POINT('',(-0.4,-0.600000000000001,-0.3)) ;
#116379=CARTESIAN_POINT('',(-0.4,-6.05857864376269,0.3)) ;
#116380=CARTESIAN_POINT('',(-0.4,-6.05857864376269,0.4)) ;
#116381=CARTESIAN_POINT('',(-0.4,-0.600000000000001,0.3)) ;
#116382=CARTESIAN_POINT('Origin',(-0.4,-6.1,0.4)) ;
#116383=CARTESIAN_POINT('',(-0.129289321881346,-6.37071067811866,-0.0585786437626899)) ;
#116384=CARTESIAN_POINT('',(-0.129289321881346,-6.37071067811866,0.0585786437626899)) ;
#116385=CARTESIAN_POINT('',(-0.129289321881346,-6.37071067811866,0.4)) ;
#116386=CARTESIAN_POINT('',(-0.370710678118655,-6.12928932188134,0.3)) ;
#116387=CARTESIAN_POINT('',(-0.423570226039552,-6.07642977396045,0.352859547920897)) ;
#116388=CARTESIAN_POINT('',(-0.370710678118655,-6.12928932188134,-0.3)) ;
#116389=CARTESIAN_POINT('',(-0.370710678118655,-6.12928932188134,0.4)) ;
#116390=CARTESIAN_POINT('',(-0.156903559372884,-6.34309644062712,-0.0861928812542289)) ;
#116391=CARTESIAN_POINT('Origin',(-0.1,-6.4,0.4)) ;
#116392=CARTESIAN_POINT('',(0.0585786437626908,-6.4,-0.0585786437626897)) ;
#116393=CARTESIAN_POINT('',(0.0585786437626908,-6.4,0.0585786437626898)) ;
#116394=CARTESIAN_POINT('',(0.0585786437626908,-6.4,0.4)) ;
#116395=CARTESIAN_POINT('',(-0.0585786437626908,-6.4,0.0585786437626898)) ;
#116396=CARTESIAN_POINT('',(-0.1,-6.4,0.0585786437626898)) ;
#116397=CARTESIAN_POINT('',(-0.0585786437626908,-6.4,-0.0585786437626897)) ;
#116398=CARTESIAN_POINT('',(-0.0585786437626908,-6.4,0.4)) ;
#116399=CARTESIAN_POINT('',(-0.1,-6.4,-0.0585786437626898)) ;
#116400=CARTESIAN_POINT('Origin',(0.1,-6.4,0.4)) ;
#116401=CARTESIAN_POINT('',(0.370710678118655,-6.12928932188134,-0.3)) ;
#116402=CARTESIAN_POINT('',(0.370710678118655,-6.12928932188134,0.299999999999999)) ;
#116403=CARTESIAN_POINT('',(0.370710678118655,-6.12928932188134,0.4)) ;
#116404=CARTESIAN_POINT('',(0.129289321881346,-6.37071067811866,0.0585786437626892)) ;
#116405=CARTESIAN_POINT('',(0.223570226039552,-6.27642977396045,0.152859547920897)) ;
#116406=CARTESIAN_POINT('',(0.129289321881346,-6.37071067811866,-0.05857864376269)) ;
#116407=CARTESIAN_POINT('',(0.129289321881346,-6.37071067811866,0.4)) ;
#116408=CARTESIAN_POINT('',(-0.0430964406271149,-6.54309644062712,0.113807118745771)) ;
#116409=CARTESIAN_POINT('Origin',(0.4,-6.1,0.4)) ;
#116410=CARTESIAN_POINT('',(0.4,-6.05857864376269,0.3)) ;
#116411=CARTESIAN_POINT('',(0.4,-6.05857864376269,-0.3)) ;
#116412=CARTESIAN_POINT('',(0.4,-6.05857864376269,0.4)) ;
#116413=CARTESIAN_POINT('',(0.4,-0.6,-0.3)) ;
#116414=CARTESIAN_POINT('',(0.4,-6.1,-0.3)) ;
#116415=CARTESIAN_POINT('',(0.4,-0.6,0.3)) ;
#116416=CARTESIAN_POINT('',(0.4,-0.6,0.4)) ;
#116417=CARTESIAN_POINT('',(0.4,-6.05857864376269,0.3)) ;
#116418=CARTESIAN_POINT('Origin',(0.6,-0.600000000000001,0.4)) ;
#116419=CARTESIAN_POINT('',(0.3,-6.05857864376269,0.4)) ;
#116420=CARTESIAN_POINT('',(0.3,-0.6,0.4)) ;
#116421=CARTESIAN_POINT('',(0.3,-0.6,0.4)) ;
#116422=CARTESIAN_POINT('Origin',(0.6,-0.6,0.4)) ;
#116423=CARTESIAN_POINT('',(-0.3,-0.600000000000001,0.4)) ;
#116424=CARTESIAN_POINT('Origin',(0.6,-0.600000000000001,0.4)) ;
#116425=CARTESIAN_POINT('',(-0.3,-6.05857864376269,0.4)) ;
#116426=CARTESIAN_POINT('',(-0.3,-0.600000000000001,0.4)) ;
#116427=CARTESIAN_POINT('',(0.4,-6.05857864376269,0.4)) ;
#116428=CARTESIAN_POINT('Origin',(0.6,-0.600000000000001,-0.4)) ;
#116429=CARTESIAN_POINT('',(-0.3,-6.05857864376269,-0.4)) ;
#116430=CARTESIAN_POINT('',(-0.3,-0.600000000000001,-0.4)) ;
#116431=CARTESIAN_POINT('',(-0.3,-0.600000000000001,-0.4)) ;
#116432=CARTESIAN_POINT('Origin',(0.6,-0.600000000000001,-0.4)) ;
#116433=CARTESIAN_POINT('',(0.3,-0.6,-0.4)) ;
#116434=CARTESIAN_POINT('Origin',(0.6,-0.6,-0.4)) ;
#116435=CARTESIAN_POINT('',(0.3,-6.05857864376269,-0.4)) ;
#116436=CARTESIAN_POINT('',(0.3,-0.600000000000001,-0.4)) ;
#116437=CARTESIAN_POINT('',(0.6,-6.05857864376269,-0.4)) ;
#116438=CARTESIAN_POINT('Origin',(0.6,-0.600000000000001,0.4)) ;
#116439=CARTESIAN_POINT('Origin',(0.6,-0.600000000000001,-0.3)) ;
#116440=CARTESIAN_POINT('Origin',(0.6,-0.600000000000001,0.3)) ;
#116441=CARTESIAN_POINT('Origin',(0.6,-0.6,0.4)) ;
#116442=CARTESIAN_POINT('Origin',(0.6,-0.6,-0.3)) ;
#116443=CARTESIAN_POINT('Origin',(0.6,-0.6,0.3)) ;
#116444=CARTESIAN_POINT('Origin',(7.,0.1,0.4)) ;
#116445=CARTESIAN_POINT('',(6.72928932188135,0.370710678118655,-0.3)) ;
#116446=CARTESIAN_POINT('',(6.72928932188135,0.370710678118655,0.3)) ;
#116447=CARTESIAN_POINT('',(6.72928932188135,0.370710678118655,0.4)) ;
#116448=CARTESIAN_POINT('',(6.97071067811866,0.129289321881346,0.0585786437626902)) ;
#116449=CARTESIAN_POINT('',(6.87642977396045,0.223570226039552,0.152859547920897)) ;
#116450=CARTESIAN_POINT('',(6.97071067811866,0.129289321881346,-0.0585786437626903)) ;
#116451=CARTESIAN_POINT('',(6.97071067811866,0.129289321881346,0.4)) ;
#116452=CARTESIAN_POINT('',(7.14309644062712,-0.043096440627115,0.11380711874577)) ;
#116453=CARTESIAN_POINT('Origin',(6.7,0.400000000000001,0.4)) ;
#116454=CARTESIAN_POINT('',(6.65857864376269,0.400000000000001,0.3)) ;
#116455=CARTESIAN_POINT('',(6.65857864376269,0.400000000000001,-0.3)) ;
#116456=CARTESIAN_POINT('',(6.65857864376269,0.400000000000001,0.4)) ;
#116457=CARTESIAN_POINT('',(6.7,0.400000000000001,-0.3)) ;
#116458=CARTESIAN_POINT('',(6.65857864376269,0.400000000000001,0.3)) ;
#116459=CARTESIAN_POINT('Origin',(0.6,-0.4,0.4)) ;
#116460=CARTESIAN_POINT('',(6.65857864376269,-0.400000000000001,-0.3)) ;
#116461=CARTESIAN_POINT('',(0.6,-0.4,-0.3)) ;
#116462=CARTESIAN_POINT('',(6.65857864376269,-0.400000000000001,0.3)) ;
#116463=CARTESIAN_POINT('',(6.65857864376269,-0.400000000000001,0.4)) ;
#116464=CARTESIAN_POINT('',(2.4,-0.4,0.3)) ;
#116465=CARTESIAN_POINT('Origin',(6.7,-0.400000000000001,0.4)) ;
#116466=CARTESIAN_POINT('',(6.97071067811866,-0.129289321881346,-0.0585786437626903)) ;
#116467=CARTESIAN_POINT('',(6.97071067811866,-0.129289321881346,0.0585786437626901)) ;
#116468=CARTESIAN_POINT('',(6.97071067811866,-0.129289321881346,0.4)) ;
#116469=CARTESIAN_POINT('',(6.72928932188135,-0.370710678118655,0.3)) ;
#116470=CARTESIAN_POINT('',(6.67642977396045,-0.423570226039552,0.352859547920897)) ;
#116471=CARTESIAN_POINT('',(6.72928932188135,-0.370710678118655,-0.3)) ;
#116472=CARTESIAN_POINT('',(6.72928932188135,-0.370710678118655,0.4)) ;
#116473=CARTESIAN_POINT('',(6.94309644062712,-0.156903559372885,-0.0861928812542298)) ;
#116474=CARTESIAN_POINT('Origin',(7.,-0.1,0.4)) ;
#116475=CARTESIAN_POINT('',(7.,-0.0585786437626909,0.0585786437626901)) ;
#116476=CARTESIAN_POINT('',(7.,-0.0585786437626909,-0.05857864376269)) ;
#116477=CARTESIAN_POINT('',(7.,-0.0585786437626909,0.4)) ;
#116478=CARTESIAN_POINT('',(7.,0.0585786437626909,-0.05857864376269)) ;
#116479=CARTESIAN_POINT('',(7.,-0.1,-0.05857864376269)) ;
#116480=CARTESIAN_POINT('',(7.,0.0585786437626909,0.05857864376269)) ;
#116481=CARTESIAN_POINT('',(7.,0.0585786437626909,0.4)) ;
#116482=CARTESIAN_POINT('',(7.,-0.1,0.0585786437626901)) ;
#116483=CARTESIAN_POINT('Origin',(0.6,-0.600000000000001,0.4)) ;
#116484=CARTESIAN_POINT('',(6.65857864376269,-0.300000000000001,0.4)) ;
#116485=CARTESIAN_POINT('',(6.65857864376269,0.300000000000001,0.4)) ;
#116486=CARTESIAN_POINT('',(6.65857864376269,-0.399999999999999,0.4)) ;
#116487=CARTESIAN_POINT('',(2.4,0.3,0.4)) ;
#116488=CARTESIAN_POINT('',(6.65857864376269,-0.300000000000001,0.4)) ;
#116489=CARTESIAN_POINT('Origin',(0.6,-0.600000000000001,-0.4)) ;
#116490=CARTESIAN_POINT('',(6.65857864376269,0.300000000000001,-0.4)) ;
#116491=CARTESIAN_POINT('',(0.6,0.299999999999999,-0.4)) ;
#116492=CARTESIAN_POINT('',(6.65857864376269,-0.300000000000001,-0.4)) ;
#116493=CARTESIAN_POINT('',(6.65857864376269,-0.6,-0.4)) ;
#116494=CARTESIAN_POINT('',(0.6,-0.3,-0.4)) ;
#116495=CARTESIAN_POINT('Origin',(0.4,-6.4,-0.0999999999999988)) ;
#116496=CARTESIAN_POINT('',(-0.0585786437626909,-6.37071067811866,-0.129289321881344)) ;
#116497=CARTESIAN_POINT('',(-0.3,-6.12928932188134,-0.370710678118655)) ;
#116498=CARTESIAN_POINT('',(0.113807118745769,-6.54309644062712,0.0430964406271166)) ;
#116499=CARTESIAN_POINT('',(0.3,-6.12928932188134,-0.370710678118655)) ;
#116500=CARTESIAN_POINT('',(0.4,-6.12928932188134,-0.370710678118654)) ;
#116501=CARTESIAN_POINT('',(0.058578643762691,-6.37071067811866,-0.129289321881344)) ;
#116502=CARTESIAN_POINT('',(0.152859547920897,-6.27642977396045,-0.22357022603955)) ;
#116503=CARTESIAN_POINT('',(0.4,-6.37071067811866,-0.129289321881344)) ;
#116504=CARTESIAN_POINT('Origin',(0.4,-6.1,0.4)) ;
#116505=CARTESIAN_POINT('',(0.0585786437626902,-6.37071067811866,0.129289321881344)) ;
#116506=CARTESIAN_POINT('',(0.299999999999999,-6.12928932188134,0.370710678118655)) ;
#116507=CARTESIAN_POINT('',(0.352859547920896,-6.07642977396045,0.423570226039552)) ;
#116508=CARTESIAN_POINT('',(-0.3,-6.12928932188134,0.370710678118655)) ;
#116509=CARTESIAN_POINT('',(0.4,-6.12928932188134,0.370710678118654)) ;
#116510=CARTESIAN_POINT('',(-0.058578643762691,-6.37071067811866,0.129289321881344)) ;
#116511=CARTESIAN_POINT('',(-0.086192881254231,-6.34309644062712,0.156903559372885)) ;
#116512=CARTESIAN_POINT('',(0.4,-6.37071067811866,0.129289321881344)) ;
#116513=CARTESIAN_POINT('Origin',(6.7,-0.399999999999999,-0.4)) ;
#116514=CARTESIAN_POINT('',(6.97071067811866,-0.0585786437626912,-0.129289321881345)) ;
#116515=CARTESIAN_POINT('',(6.72928932188135,-0.300000000000001,-0.370710678118655)) ;
#116516=CARTESIAN_POINT('',(6.67642977396045,-0.352859547920897,-0.423570226039551)) ;
#116517=CARTESIAN_POINT('',(6.72928932188135,0.300000000000001,-0.370710678118655)) ;
#116518=CARTESIAN_POINT('',(6.72928932188135,-0.399999999999999,-0.370710678118655)) ;
#116519=CARTESIAN_POINT('',(6.97071067811866,0.0585786437626912,-0.129289321881345)) ;
#116520=CARTESIAN_POINT('',(6.94309644062712,0.0861928812542309,-0.156903559372884)) ;
#116521=CARTESIAN_POINT('',(6.97071067811866,-0.4,-0.129289321881345)) ;
#116522=CARTESIAN_POINT('Origin',(7.,-0.399999999999999,0.0999999999999993)) ;
#116523=CARTESIAN_POINT('',(6.97071067811866,0.0585786437626911,0.129289321881345)) ;
#116524=CARTESIAN_POINT('',(6.72928932188135,0.300000000000001,0.370710678118655)) ;
#116525=CARTESIAN_POINT('',(7.14309644062712,-0.113807118745769,-0.043096440627116)) ;
#116526=CARTESIAN_POINT('',(6.72928932188135,-0.300000000000001,0.370710678118655)) ;
#116527=CARTESIAN_POINT('',(6.72928932188135,-0.399999999999999,0.370710678118655)) ;
#116528=CARTESIAN_POINT('',(6.97071067811866,-0.0585786437626911,0.129289321881345)) ;
#116529=CARTESIAN_POINT('',(6.87642977396045,-0.152859547920897,0.223570226039551)) ;
#116530=CARTESIAN_POINT('',(6.97071067811866,-0.399999999999999,0.129289321881345)) ;
#116531=CARTESIAN_POINT('Origin',(-0.11380711874577,-6.47238576250846,0.113807118745771)) ;
#116532=CARTESIAN_POINT('Origin',(0.3,-6.05857864376269,-0.3)) ;
#116533=CARTESIAN_POINT('Origin',(0.058578643762691,-6.3,-0.0585786437626897)) ;
#116534=CARTESIAN_POINT('Origin',(0.3,-6.05857864376269,0.4)) ;
#116535=CARTESIAN_POINT('Origin',(0.3,-6.05857864376269,-0.3)) ;
#116536=CARTESIAN_POINT('Origin',(0.3,-6.05857864376269,0.3)) ;
#116537=CARTESIAN_POINT('Origin',(0.0585786437626908,-6.3,-0.0585786437626897)) ;
#116538=CARTESIAN_POINT('Origin',(0.0585786437626908,-6.3,-0.0585786437626897)) ;
#116539=CARTESIAN_POINT('Origin',(0.0585786437626908,-6.3,-0.05857864376269)) ;
#116540=CARTESIAN_POINT('Origin',(0.152859547920897,-6.20571909584179,0.152859547920897)) ;
#116541=CARTESIAN_POINT('Origin',(0.3,-6.05857864376269,0.3)) ;
#116542=CARTESIAN_POINT('Origin',(0.0585786437626908,-6.3,0.0585786437626892)) ;
#116543=CARTESIAN_POINT('Origin',(0.0585786437626908,-6.3,0.4)) ;
#116544=CARTESIAN_POINT('Origin',(0.0585786437626908,-6.3,0.0585786437626898)) ;
#116545=CARTESIAN_POINT('Origin',(0.4,-6.3,-0.0585786437626897)) ;
#116546=CARTESIAN_POINT('Origin',(-0.0585786437626909,-6.3,-0.0585786437626897)) ;
#116547=CARTESIAN_POINT('Origin',(0.0585786437626908,-6.3,0.0585786437626898)) ;
#116548=CARTESIAN_POINT('Origin',(0.0585786437626902,-6.3,0.0585786437626897)) ;
#116549=CARTESIAN_POINT('Origin',(-0.0585786437626908,-6.3,-0.0585786437626897)) ;
#116550=CARTESIAN_POINT('Origin',(-0.0585786437626908,-6.3,-0.0585786437626899)) ;
#116551=CARTESIAN_POINT('Origin',(-0.0585786437626908,-6.3,-0.0585786437626897)) ;
#116552=CARTESIAN_POINT('Origin',(-0.1,-6.3,0.0585786437626898)) ;
#116553=CARTESIAN_POINT('Origin',(-0.0585786437626908,-6.3,0.0585786437626898)) ;
#116554=CARTESIAN_POINT('Origin',(-0.0585786437626908,-6.3,0.4)) ;
#116555=CARTESIAN_POINT('Origin',(-0.0585786437626908,-6.3,0.0585786437626899)) ;
#116556=CARTESIAN_POINT('Origin',(-0.0861928812542298,-6.27238576250846,
-0.0861928812542288)) ;
#116557=CARTESIAN_POINT('Origin',(-0.3,-6.05857864376269,-0.3)) ;
#116558=CARTESIAN_POINT('Origin',(-0.0585786437626909,-6.3,0.0585786437626898)) ;
#116559=CARTESIAN_POINT('Origin',(-0.058578643762691,-6.3,0.0585786437626897)) ;
#116560=CARTESIAN_POINT('Origin',(-0.3,-6.05857864376269,0.4)) ;
#116561=CARTESIAN_POINT('Origin',(-0.3,-6.05857864376269,-0.3)) ;
#116562=CARTESIAN_POINT('Origin',(-0.3,-6.05857864376269,0.3)) ;
#116563=CARTESIAN_POINT('Origin',(-0.352859547920897,-6.00571909584179,
0.352859547920897)) ;
#116564=CARTESIAN_POINT('Origin',(-0.3,-6.05857864376269,0.3)) ;
#116565=CARTESIAN_POINT('Origin',(7.07238576250846,-0.11380711874577,0.113807118745771)) ;
#116566=CARTESIAN_POINT('Origin',(6.65857864376269,0.300000000000001,-0.3)) ;
#116567=CARTESIAN_POINT('Origin',(6.9,0.0585786437626912,-0.05857864376269)) ;
#116568=CARTESIAN_POINT('Origin',(6.65857864376269,0.300000000000001,0.4)) ;
#116569=CARTESIAN_POINT('Origin',(6.65857864376269,0.300000000000001,-0.3)) ;
#116570=CARTESIAN_POINT('Origin',(6.65857864376269,0.300000000000001,0.3)) ;
#116571=CARTESIAN_POINT('Origin',(6.9,0.0585786437626909,-0.05857864376269)) ;
#116572=CARTESIAN_POINT('Origin',(6.9,0.0585786437626909,-0.05857864376269)) ;
#116573=CARTESIAN_POINT('Origin',(6.9,0.0585786437626909,-0.0585786437626903)) ;
#116574=CARTESIAN_POINT('Origin',(6.80571909584179,0.152859547920897,0.152859547920897)) ;
#116575=CARTESIAN_POINT('Origin',(6.65857864376269,0.300000000000001,0.3)) ;
#116576=CARTESIAN_POINT('Origin',(6.9,0.0585786437626909,0.0585786437626902)) ;
#116577=CARTESIAN_POINT('Origin',(6.9,0.0585786437626909,0.4)) ;
#116578=CARTESIAN_POINT('Origin',(6.9,0.0585786437626909,0.05857864376269)) ;
#116579=CARTESIAN_POINT('Origin',(6.9,-0.1,-0.05857864376269)) ;
#116580=CARTESIAN_POINT('Origin',(6.9,-0.0585786437626912,-0.05857864376269)) ;
#116581=CARTESIAN_POINT('Origin',(6.9,0.0585786437626909,0.05857864376269)) ;
#116582=CARTESIAN_POINT('Origin',(6.9,0.0585786437626911,0.05857864376269)) ;
#116583=CARTESIAN_POINT('Origin',(6.9,-0.058578643762691,-0.0585786437626901)) ;
#116584=CARTESIAN_POINT('Origin',(6.9,-0.0585786437626909,-0.0585786437626903)) ;
#116585=CARTESIAN_POINT('Origin',(6.9,-0.0585786437626909,-0.05857864376269)) ;
#116586=CARTESIAN_POINT('Origin',(6.9,-0.399999999999999,0.0585786437626901)) ;
#116587=CARTESIAN_POINT('Origin',(6.9,-0.0585786437626909,0.0585786437626901)) ;
#116588=CARTESIAN_POINT('Origin',(6.9,-0.0585786437626909,0.4)) ;
#116589=CARTESIAN_POINT('Origin',(6.9,-0.0585786437626909,0.0585786437626901)) ;
#116590=CARTESIAN_POINT('Origin',(6.87238576250846,-0.0861928812542305,
-0.0861928812542296)) ;
#116591=CARTESIAN_POINT('Origin',(6.65857864376269,-0.300000000000001,-0.3)) ;
#116592=CARTESIAN_POINT('Origin',(6.9,-0.058578643762691,0.0585786437626901)) ;
#116593=CARTESIAN_POINT('Origin',(6.9,-0.0585786437626911,0.05857864376269)) ;
#116594=CARTESIAN_POINT('Origin',(6.65857864376269,-0.300000000000001,0.4)) ;
#116595=CARTESIAN_POINT('Origin',(6.65857864376269,-0.300000000000001,-0.3)) ;
#116596=CARTESIAN_POINT('Origin',(6.65857864376269,-0.300000000000001,0.3)) ;
#116597=CARTESIAN_POINT('Origin',(6.60571909584179,-0.352859547920898,0.352859547920897)) ;
#116598=CARTESIAN_POINT('Origin',(6.65857864376269,-0.300000000000001,0.3)) ;
#116599=CARTESIAN_POINT('Origin',(0.6,-0.6,-0.3)) ;
#116600=CARTESIAN_POINT('Origin',(0.3,-0.6,-0.3)) ;
#116601=CARTESIAN_POINT('Origin',(0.3,-6.1,-0.3)) ;
#116602=CARTESIAN_POINT('Origin',(0.3,-6.05857864376269,-0.3)) ;
#116603=CARTESIAN_POINT('Origin',(0.3,-6.05857864376269,-0.3)) ;
#116604=CARTESIAN_POINT('Origin',(0.3,-6.05857864376269,-0.3)) ;
#116605=CARTESIAN_POINT('Origin',(0.4,-6.05857864376269,-0.3)) ;
#116606=CARTESIAN_POINT('Origin',(-0.3,-6.05857864376269,-0.3)) ;
#116607=CARTESIAN_POINT('Origin',(-0.3,-6.05857864376269,-0.3)) ;
#116608=CARTESIAN_POINT('Origin',(-0.3,-6.05857864376269,-0.3)) ;
#116609=CARTESIAN_POINT('Origin',(-0.3,-0.600000000000001,-0.3)) ;
#116610=CARTESIAN_POINT('Origin',(-0.3,-0.600000000000001,-0.3)) ;
#116611=CARTESIAN_POINT('Origin',(0.6,-0.600000000000001,-0.3)) ;
#116612=CARTESIAN_POINT('Origin',(0.6,-0.600000000000001,0.3)) ;
#116613=CARTESIAN_POINT('Origin',(-0.3,-0.600000000000001,0.3)) ;
#116614=CARTESIAN_POINT('Origin',(-0.3,-0.600000000000001,0.3)) ;
#116615=CARTESIAN_POINT('Origin',(-0.3,-6.05857864376269,0.3)) ;
#116616=CARTESIAN_POINT('Origin',(-0.3,-6.05857864376269,0.3)) ;
#116617=CARTESIAN_POINT('Origin',(-0.3,-6.05857864376269,0.3)) ;
#116618=CARTESIAN_POINT('Origin',(0.4,-6.05857864376269,0.3)) ;
#116619=CARTESIAN_POINT('Origin',(0.299999999999999,-6.05857864376269,0.3)) ;
#116620=CARTESIAN_POINT('Origin',(0.3,-6.05857864376269,0.3)) ;
#116621=CARTESIAN_POINT('Origin',(0.3,-6.05857864376269,0.3)) ;
#116622=CARTESIAN_POINT('Origin',(0.3,-0.600000000000001,0.3)) ;
#116623=CARTESIAN_POINT('Origin',(0.3,-0.6,0.3)) ;
#116624=CARTESIAN_POINT('Origin',(0.6,-0.6,0.3)) ;
#116625=CARTESIAN_POINT('Origin',(6.7,0.300000000000001,-0.3)) ;
#116626=CARTESIAN_POINT('Origin',(6.65857864376269,0.300000000000001,-0.3)) ;
#116627=CARTESIAN_POINT('Origin',(6.65857864376269,0.300000000000001,-0.3)) ;
#116628=CARTESIAN_POINT('Origin',(6.65857864376269,0.300000000000001,-0.3)) ;
#116629=CARTESIAN_POINT('Origin',(6.65857864376269,-0.399999999999999,-0.3)) ;
#116630=CARTESIAN_POINT('Origin',(6.65857864376269,-0.300000000000001,-0.3)) ;
#116631=CARTESIAN_POINT('Origin',(6.65857864376269,-0.300000000000001,-0.3)) ;
#116632=CARTESIAN_POINT('Origin',(6.65857864376269,-0.300000000000001,-0.3)) ;
#116633=CARTESIAN_POINT('Origin',(0.6,-0.3,-0.3)) ;
#116634=CARTESIAN_POINT('Origin',(0.6,0.299999999999999,0.3)) ;
#116635=CARTESIAN_POINT('Origin',(6.65857864376269,0.300000000000001,0.3)) ;
#116636=CARTESIAN_POINT('Origin',(6.65857864376269,0.300000000000001,0.3)) ;
#116637=CARTESIAN_POINT('Origin',(6.65857864376269,0.300000000000001,0.3)) ;
#116638=CARTESIAN_POINT('Origin',(6.65857864376269,-0.399999999999999,0.3)) ;
#116639=CARTESIAN_POINT('Origin',(6.65857864376269,-0.300000000000001,0.3)) ;
#116640=CARTESIAN_POINT('Origin',(0.6,-0.3,0.3)) ;
#116641=CARTESIAN_POINT('Origin',(6.65857864376269,-0.300000000000001,0.3)) ;
#116642=CARTESIAN_POINT('Origin',(6.65857864376269,-0.300000000000001,0.3)) ;
#116643=CARTESIAN_POINT('Origin',(-0.999999999999999,-1.59070596587277E-16,
-34.29)) ;
#116644=CARTESIAN_POINT('',(-0.999999999999999,-1.9,-33.69)) ;
#116645=CARTESIAN_POINT('',(-0.999999999999999,-1.9,-33.015)) ;
#116646=CARTESIAN_POINT('',(-0.999999999999999,-1.9,-32.915)) ;
#116647=CARTESIAN_POINT('',(-0.999999999999999,1.15,-33.015)) ;
#116648=CARTESIAN_POINT('',(-0.999999999999999,-2.89663358890162E-17,-33.015)) ;
#116649=CARTESIAN_POINT('',(-0.999999999999999,1.15,-35.565)) ;
#116650=CARTESIAN_POINT('',(-0.999999999999999,1.15,-34.29)) ;
#116651=CARTESIAN_POINT('',(-0.999999999999999,-1.9,-35.565)) ;
#116652=CARTESIAN_POINT('',(-0.999999999999999,-2.24122726936407E-16,-35.565)) ;
#116653=CARTESIAN_POINT('',(-0.999999999999999,-1.9,-34.89)) ;
#116654=CARTESIAN_POINT('',(-0.999999999999999,-1.9,-34.79)) ;
#116655=CARTESIAN_POINT('',(-0.999999999999999,0.4,-34.89)) ;
#116656=CARTESIAN_POINT('',(-0.999999999999999,0.5,-34.89)) ;
#116657=CARTESIAN_POINT('',(-0.999999999999999,0.6,-34.69)) ;
#116658=CARTESIAN_POINT('Origin',(-0.999999999999999,0.4,-34.69)) ;
#116659=CARTESIAN_POINT('',(-0.999999999999999,0.6,-33.89)) ;
#116660=CARTESIAN_POINT('',(-0.999999999999999,0.6,-33.79)) ;
#116661=CARTESIAN_POINT('',(-0.999999999999999,0.4,-33.69)) ;
#116662=CARTESIAN_POINT('Origin',(-0.999999999999999,0.4,-33.89)) ;
#116663=CARTESIAN_POINT('',(-0.999999999999999,-2.,-33.69)) ;
#116664=CARTESIAN_POINT('Origin',(-0.999999999999999,-1.59070596587277E-16,
-30.48)) ;
#116665=CARTESIAN_POINT('',(-0.999999999999999,-1.9,-29.88)) ;
#116666=CARTESIAN_POINT('',(-0.999999999999999,-1.9,-29.205)) ;
#116667=CARTESIAN_POINT('',(-0.999999999999999,-1.9,-29.105)) ;
#116668=CARTESIAN_POINT('',(-0.999999999999999,1.15,-29.205)) ;
#116669=CARTESIAN_POINT('',(-0.999999999999999,-2.89663358890162E-17,-29.205)) ;
#116670=CARTESIAN_POINT('',(-0.999999999999999,1.15,-31.755)) ;
#116671=CARTESIAN_POINT('',(-0.999999999999999,1.15,-30.48)) ;
#116672=CARTESIAN_POINT('',(-0.999999999999999,-1.9,-31.755)) ;
#116673=CARTESIAN_POINT('',(-0.999999999999999,-2.24122726936407E-16,-31.755)) ;
#116674=CARTESIAN_POINT('',(-0.999999999999999,-1.9,-31.08)) ;
#116675=CARTESIAN_POINT('',(-0.999999999999999,-1.9,-30.98)) ;
#116676=CARTESIAN_POINT('',(-0.999999999999999,0.4,-31.08)) ;
#116677=CARTESIAN_POINT('',(-0.999999999999999,0.5,-31.08)) ;
#116678=CARTESIAN_POINT('',(-0.999999999999999,0.6,-30.88)) ;
#116679=CARTESIAN_POINT('Origin',(-0.999999999999999,0.4,-30.88)) ;
#116680=CARTESIAN_POINT('',(-0.999999999999999,0.6,-30.08)) ;
#116681=CARTESIAN_POINT('',(-0.999999999999999,0.6,-29.98)) ;
#116682=CARTESIAN_POINT('',(-0.999999999999999,0.4,-29.88)) ;
#116683=CARTESIAN_POINT('Origin',(-0.999999999999999,0.4,-30.08)) ;
#116684=CARTESIAN_POINT('',(-0.999999999999999,-2.,-29.88)) ;
#116685=CARTESIAN_POINT('Origin',(-0.999999999999999,-1.59070596587277E-16,
-26.67)) ;
#116686=CARTESIAN_POINT('',(-0.999999999999999,-1.9,-26.07)) ;
#116687=CARTESIAN_POINT('',(-0.999999999999999,-1.9,-25.395)) ;
#116688=CARTESIAN_POINT('',(-0.999999999999999,-1.9,-25.295)) ;
#116689=CARTESIAN_POINT('',(-0.999999999999999,1.15,-25.395)) ;
#116690=CARTESIAN_POINT('',(-0.999999999999999,-2.89663358890162E-17,-25.395)) ;
#116691=CARTESIAN_POINT('',(-0.999999999999999,1.15,-27.945)) ;
#116692=CARTESIAN_POINT('',(-0.999999999999999,1.15,-26.67)) ;
#116693=CARTESIAN_POINT('',(-0.999999999999999,-1.9,-27.945)) ;
#116694=CARTESIAN_POINT('',(-0.999999999999999,-2.24122726936407E-16,-27.945)) ;
#116695=CARTESIAN_POINT('',(-0.999999999999999,-1.9,-27.27)) ;
#116696=CARTESIAN_POINT('',(-0.999999999999999,-1.9,-27.17)) ;
#116697=CARTESIAN_POINT('',(-0.999999999999999,0.4,-27.27)) ;
#116698=CARTESIAN_POINT('',(-0.999999999999999,0.5,-27.27)) ;
#116699=CARTESIAN_POINT('',(-0.999999999999999,0.6,-27.07)) ;
#116700=CARTESIAN_POINT('Origin',(-0.999999999999999,0.4,-27.07)) ;
#116701=CARTESIAN_POINT('',(-0.999999999999999,0.6,-26.27)) ;
#116702=CARTESIAN_POINT('',(-0.999999999999999,0.6,-26.17)) ;
#116703=CARTESIAN_POINT('',(-0.999999999999999,0.4,-26.07)) ;
#116704=CARTESIAN_POINT('Origin',(-0.999999999999999,0.4,-26.27)) ;
#116705=CARTESIAN_POINT('',(-0.999999999999999,-2.,-26.07)) ;
#116706=CARTESIAN_POINT('Origin',(-0.999999999999999,-1.59070596587277E-16,
-22.86)) ;
#116707=CARTESIAN_POINT('',(-0.999999999999999,-1.9,-22.26)) ;
#116708=CARTESIAN_POINT('',(-0.999999999999999,-1.9,-21.585)) ;
#116709=CARTESIAN_POINT('',(-0.999999999999999,-1.9,-21.485)) ;
#116710=CARTESIAN_POINT('',(-0.999999999999999,1.15,-21.585)) ;
#116711=CARTESIAN_POINT('',(-0.999999999999999,-2.89663358890162E-17,-21.585)) ;
#116712=CARTESIAN_POINT('',(-0.999999999999999,1.15,-24.135)) ;
#116713=CARTESIAN_POINT('',(-0.999999999999999,1.15,-22.86)) ;
#116714=CARTESIAN_POINT('',(-0.999999999999999,-1.9,-24.135)) ;
#116715=CARTESIAN_POINT('',(-0.999999999999999,-2.24122726936407E-16,-24.135)) ;
#116716=CARTESIAN_POINT('',(-0.999999999999999,-1.9,-23.46)) ;
#116717=CARTESIAN_POINT('',(-0.999999999999999,-1.9,-23.36)) ;
#116718=CARTESIAN_POINT('',(-0.999999999999999,0.4,-23.46)) ;
#116719=CARTESIAN_POINT('',(-0.999999999999999,0.5,-23.46)) ;
#116720=CARTESIAN_POINT('',(-0.999999999999999,0.6,-23.26)) ;
#116721=CARTESIAN_POINT('Origin',(-0.999999999999999,0.4,-23.26)) ;
#116722=CARTESIAN_POINT('',(-0.999999999999999,0.6,-22.46)) ;
#116723=CARTESIAN_POINT('',(-0.999999999999999,0.6,-22.36)) ;
#116724=CARTESIAN_POINT('',(-0.999999999999999,0.4,-22.26)) ;
#116725=CARTESIAN_POINT('Origin',(-0.999999999999999,0.4,-22.46)) ;
#116726=CARTESIAN_POINT('',(-0.999999999999999,-2.,-22.26)) ;
#116727=CARTESIAN_POINT('Origin',(-0.999999999999999,-1.59070596587277E-16,
-19.05)) ;
#116728=CARTESIAN_POINT('',(-0.999999999999999,-1.9,-18.45)) ;
#116729=CARTESIAN_POINT('',(-0.999999999999999,-1.9,-17.775)) ;
#116730=CARTESIAN_POINT('',(-0.999999999999999,-1.9,-17.675)) ;
#116731=CARTESIAN_POINT('',(-0.999999999999999,1.15,-17.775)) ;
#116732=CARTESIAN_POINT('',(-0.999999999999999,-2.89663358890162E-17,-17.775)) ;
#116733=CARTESIAN_POINT('',(-0.999999999999999,1.15,-20.325)) ;
#116734=CARTESIAN_POINT('',(-0.999999999999999,1.15,-19.05)) ;
#116735=CARTESIAN_POINT('',(-0.999999999999999,-1.9,-20.325)) ;
#116736=CARTESIAN_POINT('',(-0.999999999999999,-2.24122726936407E-16,-20.325)) ;
#116737=CARTESIAN_POINT('',(-0.999999999999999,-1.9,-19.65)) ;
#116738=CARTESIAN_POINT('',(-0.999999999999999,-1.9,-19.55)) ;
#116739=CARTESIAN_POINT('',(-0.999999999999999,0.4,-19.65)) ;
#116740=CARTESIAN_POINT('',(-0.999999999999999,0.5,-19.65)) ;
#116741=CARTESIAN_POINT('',(-0.999999999999999,0.6,-19.45)) ;
#116742=CARTESIAN_POINT('Origin',(-0.999999999999999,0.4,-19.45)) ;
#116743=CARTESIAN_POINT('',(-0.999999999999999,0.6,-18.65)) ;
#116744=CARTESIAN_POINT('',(-0.999999999999999,0.6,-18.55)) ;
#116745=CARTESIAN_POINT('',(-0.999999999999999,0.4,-18.45)) ;
#116746=CARTESIAN_POINT('Origin',(-0.999999999999999,0.4,-18.65)) ;
#116747=CARTESIAN_POINT('',(-0.999999999999999,-2.,-18.45)) ;
#116748=CARTESIAN_POINT('Origin',(-0.999999999999999,-1.59070596587277E-16,
-15.24)) ;
#116749=CARTESIAN_POINT('',(-0.999999999999999,-1.9,-14.64)) ;
#116750=CARTESIAN_POINT('',(-0.999999999999999,-1.9,-13.965)) ;
#116751=CARTESIAN_POINT('',(-0.999999999999999,-1.9,-13.865)) ;
#116752=CARTESIAN_POINT('',(-0.999999999999999,1.15,-13.965)) ;
#116753=CARTESIAN_POINT('',(-0.999999999999999,-2.8966335889016E-17,-13.965)) ;
#116754=CARTESIAN_POINT('',(-0.999999999999999,1.15,-16.515)) ;
#116755=CARTESIAN_POINT('',(-0.999999999999999,1.15,-15.24)) ;
#116756=CARTESIAN_POINT('',(-0.999999999999999,-1.9,-16.515)) ;
#116757=CARTESIAN_POINT('',(-0.999999999999999,-2.24122726936407E-16,-16.515)) ;
#116758=CARTESIAN_POINT('',(-0.999999999999999,-1.9,-15.84)) ;
#116759=CARTESIAN_POINT('',(-0.999999999999999,-1.9,-15.74)) ;
#116760=CARTESIAN_POINT('',(-0.999999999999999,0.4,-15.84)) ;
#116761=CARTESIAN_POINT('',(-0.999999999999999,0.5,-15.84)) ;
#116762=CARTESIAN_POINT('',(-0.999999999999999,0.6,-15.64)) ;
#116763=CARTESIAN_POINT('Origin',(-0.999999999999999,0.4,-15.64)) ;
#116764=CARTESIAN_POINT('',(-0.999999999999999,0.6,-14.84)) ;
#116765=CARTESIAN_POINT('',(-0.999999999999999,0.6,-14.74)) ;
#116766=CARTESIAN_POINT('',(-0.999999999999999,0.4,-14.64)) ;
#116767=CARTESIAN_POINT('Origin',(-0.999999999999999,0.4,-14.84)) ;
#116768=CARTESIAN_POINT('',(-0.999999999999999,-2.,-14.64)) ;
#116769=CARTESIAN_POINT('Origin',(-0.999999999999999,-1.59070596587277E-16,
-11.43)) ;
#116770=CARTESIAN_POINT('',(-0.999999999999999,-1.9,-10.83)) ;
#116771=CARTESIAN_POINT('',(-0.999999999999999,-1.9,-10.155)) ;
#116772=CARTESIAN_POINT('',(-0.999999999999999,-1.9,-10.055)) ;
#116773=CARTESIAN_POINT('',(-0.999999999999999,1.15,-10.155)) ;
#116774=CARTESIAN_POINT('',(-0.999999999999999,-2.8966335889016E-17,-10.155)) ;
#116775=CARTESIAN_POINT('',(-0.999999999999999,1.15,-12.705)) ;
#116776=CARTESIAN_POINT('',(-0.999999999999999,1.15,-11.43)) ;
#116777=CARTESIAN_POINT('',(-0.999999999999999,-1.9,-12.705)) ;
#116778=CARTESIAN_POINT('',(-0.999999999999999,-2.24122726936407E-16,-12.705)) ;
#116779=CARTESIAN_POINT('',(-0.999999999999999,-1.9,-12.03)) ;
#116780=CARTESIAN_POINT('',(-0.999999999999999,-1.9,-11.93)) ;
#116781=CARTESIAN_POINT('',(-0.999999999999999,0.4,-12.03)) ;
#116782=CARTESIAN_POINT('',(-0.999999999999999,0.5,-12.03)) ;
#116783=CARTESIAN_POINT('',(-0.999999999999999,0.6,-11.83)) ;
#116784=CARTESIAN_POINT('Origin',(-0.999999999999999,0.4,-11.83)) ;
#116785=CARTESIAN_POINT('',(-0.999999999999999,0.6,-11.03)) ;
#116786=CARTESIAN_POINT('',(-0.999999999999999,0.6,-10.93)) ;
#116787=CARTESIAN_POINT('',(-0.999999999999999,0.4,-10.83)) ;
#116788=CARTESIAN_POINT('Origin',(-0.999999999999999,0.4,-11.03)) ;
#116789=CARTESIAN_POINT('',(-0.999999999999999,-2.,-10.83)) ;
#116790=CARTESIAN_POINT('Origin',(-0.999999999999999,-1.59070596587277E-16,
-7.62)) ;
#116791=CARTESIAN_POINT('',(-0.999999999999999,-1.9,-7.02)) ;
#116792=CARTESIAN_POINT('',(-0.999999999999999,-1.9,-6.345)) ;
#116793=CARTESIAN_POINT('',(-0.999999999999999,-1.9,-6.245)) ;
#116794=CARTESIAN_POINT('',(-0.999999999999999,1.15,-6.345)) ;
#116795=CARTESIAN_POINT('',(-0.999999999999999,-2.89663358890161E-17,-6.345)) ;
#116796=CARTESIAN_POINT('',(-0.999999999999999,1.15,-8.895)) ;
#116797=CARTESIAN_POINT('',(-0.999999999999999,1.15,-7.62)) ;
#116798=CARTESIAN_POINT('',(-0.999999999999999,-1.9,-8.895)) ;
#116799=CARTESIAN_POINT('',(-0.999999999999999,-2.24122726936407E-16,-8.895)) ;
#116800=CARTESIAN_POINT('',(-0.999999999999999,-1.9,-8.22)) ;
#116801=CARTESIAN_POINT('',(-0.999999999999999,-1.9,-8.12)) ;
#116802=CARTESIAN_POINT('',(-0.999999999999999,0.4,-8.22)) ;
#116803=CARTESIAN_POINT('',(-0.999999999999999,0.5,-8.22)) ;
#116804=CARTESIAN_POINT('',(-0.999999999999999,0.6,-8.02)) ;
#116805=CARTESIAN_POINT('Origin',(-0.999999999999999,0.4,-8.02)) ;
#116806=CARTESIAN_POINT('',(-0.999999999999999,0.6,-7.22)) ;
#116807=CARTESIAN_POINT('',(-0.999999999999999,0.6,-7.12)) ;
#116808=CARTESIAN_POINT('',(-0.999999999999999,0.4,-7.02)) ;
#116809=CARTESIAN_POINT('Origin',(-0.999999999999999,0.4,-7.22)) ;
#116810=CARTESIAN_POINT('',(-0.999999999999999,-2.,-7.02)) ;
#116811=CARTESIAN_POINT('Origin',(-0.999999999999999,-1.59070596587277E-16,
-3.81)) ;
#116812=CARTESIAN_POINT('',(-0.999999999999999,-1.9,-3.21)) ;
#116813=CARTESIAN_POINT('',(-0.999999999999999,-1.9,-2.535)) ;
#116814=CARTESIAN_POINT('',(-0.999999999999999,-1.9,-2.435)) ;
#116815=CARTESIAN_POINT('',(-0.999999999999999,1.15,-2.535)) ;
#116816=CARTESIAN_POINT('',(-0.999999999999999,-2.89663358890161E-17,-2.535)) ;
#116817=CARTESIAN_POINT('',(-0.999999999999999,1.15,-5.085)) ;
#116818=CARTESIAN_POINT('',(-0.999999999999999,1.15,-3.81)) ;
#116819=CARTESIAN_POINT('',(-0.999999999999999,-1.9,-5.085)) ;
#116820=CARTESIAN_POINT('',(-0.999999999999999,-2.24122726936407E-16,-5.085)) ;
#116821=CARTESIAN_POINT('',(-0.999999999999999,-1.9,-4.41)) ;
#116822=CARTESIAN_POINT('',(-0.999999999999999,-1.9,-4.31)) ;
#116823=CARTESIAN_POINT('',(-0.999999999999999,0.4,-4.41)) ;
#116824=CARTESIAN_POINT('',(-0.999999999999999,0.5,-4.41)) ;
#116825=CARTESIAN_POINT('',(-0.999999999999999,0.6,-4.21)) ;
#116826=CARTESIAN_POINT('Origin',(-0.999999999999999,0.4,-4.21)) ;
#116827=CARTESIAN_POINT('',(-0.999999999999999,0.6,-3.41)) ;
#116828=CARTESIAN_POINT('',(-0.999999999999999,0.6,-3.31)) ;
#116829=CARTESIAN_POINT('',(-0.999999999999999,0.4,-3.21)) ;
#116830=CARTESIAN_POINT('Origin',(-0.999999999999999,0.4,-3.41)) ;
#116831=CARTESIAN_POINT('',(-0.999999999999999,-2.,-3.21)) ;
#116832=CARTESIAN_POINT('Origin',(0.600000000000001,-2.,-4.31)) ;
#116833=CARTESIAN_POINT('',(0.500000000000001,-2.,-4.41)) ;
#116834=CARTESIAN_POINT('',(-0.899999999999999,-2.,-4.41)) ;
#116835=CARTESIAN_POINT('',(0.600000000000001,-2.,-4.41)) ;
#116836=CARTESIAN_POINT('',(-0.899999999999999,-2.,-5.085)) ;
#116837=CARTESIAN_POINT('',(-0.899999999999999,-2.,-5.185)) ;
#116838=CARTESIAN_POINT('',(0.500000000000001,-2.,-5.085)) ;
#116839=CARTESIAN_POINT('',(0.600000000000001,-2.,-5.085)) ;
#116840=CARTESIAN_POINT('',(0.500000000000001,-2.,-4.31)) ;
#116841=CARTESIAN_POINT('Origin',(0.600000000000001,0.5,-4.31)) ;
#116842=CARTESIAN_POINT('',(-0.899999999999999,0.4,-4.31)) ;
#116843=CARTESIAN_POINT('',(-0.999999999999999,0.4,-4.31)) ;
#116844=CARTESIAN_POINT('',(-0.899999999999999,-1.9,-4.31)) ;
#116845=CARTESIAN_POINT('',(-0.899999999999999,-2.,-4.31)) ;
#116846=CARTESIAN_POINT('',(0.600000000000001,-1.9,-4.31)) ;
#116847=CARTESIAN_POINT('Origin',(0.600000000000001,0.5,-3.31)) ;
#116848=CARTESIAN_POINT('',(0.500000000000001,0.5,-3.41)) ;
#116849=CARTESIAN_POINT('',(-0.899999999999999,0.5,-3.41)) ;
#116850=CARTESIAN_POINT('',(-0.999999999999999,0.5,-3.41)) ;
#116851=CARTESIAN_POINT('',(-0.899999999999999,0.5,-4.21)) ;
#116852=CARTESIAN_POINT('',(-0.899999999999999,0.5,-4.31)) ;
#116853=CARTESIAN_POINT('',(0.500000000000001,0.5,-4.21)) ;
#116854=CARTESIAN_POINT('',(0.600000000000001,0.5,-4.21)) ;
#116855=CARTESIAN_POINT('',(0.500000000000001,0.5,-3.31)) ;
#116856=CARTESIAN_POINT('Origin',(0.600000000000001,-2.,-3.31)) ;
#116857=CARTESIAN_POINT('',(0.500000000000001,-1.9,-3.31)) ;
#116858=CARTESIAN_POINT('',(-0.899999999999999,-1.9,-3.31)) ;
#116859=CARTESIAN_POINT('',(0.600000000000001,-1.9,-3.31)) ;
#116860=CARTESIAN_POINT('',(-0.899999999999999,0.4,-3.31)) ;
#116861=CARTESIAN_POINT('',(-0.899999999999999,0.5,-3.31)) ;
#116862=CARTESIAN_POINT('',(0.500000000000001,0.4,-3.31)) ;
#116863=CARTESIAN_POINT('',(0.600000000000001,0.4,-3.31)) ;
#116864=CARTESIAN_POINT('',(0.500000000000001,-2.,-3.31)) ;
#116865=CARTESIAN_POINT('Origin',(0.600000000000001,-2.,-2.435)) ;
#116866=CARTESIAN_POINT('',(0.500000000000001,-2.,-2.535)) ;
#116867=CARTESIAN_POINT('',(-0.899999999999999,-2.,-2.535)) ;
#116868=CARTESIAN_POINT('',(-0.999999999999999,-2.,-2.535)) ;
#116869=CARTESIAN_POINT('',(-0.899999999999999,-2.,-3.21)) ;
#116870=CARTESIAN_POINT('',(-0.899999999999999,-2.,-3.31)) ;
#116871=CARTESIAN_POINT('',(0.500000000000001,-2.,-3.21)) ;
#116872=CARTESIAN_POINT('',(0.600000000000001,-2.,-3.21)) ;
#116873=CARTESIAN_POINT('',(0.500000000000001,-2.,-2.435)) ;
#116874=CARTESIAN_POINT('Origin',(0.600000000000001,-2.,-8.12)) ;
#116875=CARTESIAN_POINT('',(0.500000000000001,-2.,-8.22)) ;
#116876=CARTESIAN_POINT('',(-0.899999999999999,-2.,-8.22)) ;
#116877=CARTESIAN_POINT('',(0.600000000000001,-2.,-8.22)) ;
#116878=CARTESIAN_POINT('',(-0.899999999999999,-2.,-8.895)) ;
#116879=CARTESIAN_POINT('',(-0.899999999999999,-2.,-8.995)) ;
#116880=CARTESIAN_POINT('',(0.500000000000001,-2.,-8.895)) ;
#116881=CARTESIAN_POINT('',(0.600000000000001,-2.,-8.895)) ;
#116882=CARTESIAN_POINT('',(0.500000000000001,-2.,-8.12)) ;
#116883=CARTESIAN_POINT('Origin',(0.600000000000001,0.5,-8.12)) ;
#116884=CARTESIAN_POINT('',(-0.899999999999999,0.4,-8.12)) ;
#116885=CARTESIAN_POINT('',(-0.999999999999999,0.4,-8.12)) ;
#116886=CARTESIAN_POINT('',(-0.899999999999999,-1.9,-8.12)) ;
#116887=CARTESIAN_POINT('',(-0.899999999999999,-2.,-8.12)) ;
#116888=CARTESIAN_POINT('',(0.600000000000001,-1.9,-8.12)) ;
#116889=CARTESIAN_POINT('Origin',(0.600000000000001,0.5,-7.12)) ;
#116890=CARTESIAN_POINT('',(0.500000000000001,0.5,-7.22)) ;
#116891=CARTESIAN_POINT('',(-0.899999999999999,0.5,-7.22)) ;
#116892=CARTESIAN_POINT('',(-0.999999999999999,0.5,-7.22)) ;
#116893=CARTESIAN_POINT('',(-0.899999999999999,0.5,-8.02)) ;
#116894=CARTESIAN_POINT('',(-0.899999999999999,0.5,-8.12)) ;
#116895=CARTESIAN_POINT('',(0.500000000000001,0.5,-8.02)) ;
#116896=CARTESIAN_POINT('',(0.600000000000001,0.5,-8.02)) ;
#116897=CARTESIAN_POINT('',(0.500000000000001,0.5,-7.12)) ;
#116898=CARTESIAN_POINT('Origin',(0.600000000000001,-2.,-7.12)) ;
#116899=CARTESIAN_POINT('',(0.500000000000001,-1.9,-7.12)) ;
#116900=CARTESIAN_POINT('',(-0.899999999999999,-1.9,-7.12)) ;
#116901=CARTESIAN_POINT('',(0.600000000000001,-1.9,-7.12)) ;
#116902=CARTESIAN_POINT('',(-0.899999999999999,0.4,-7.12)) ;
#116903=CARTESIAN_POINT('',(-0.899999999999999,0.5,-7.12)) ;
#116904=CARTESIAN_POINT('',(0.500000000000001,0.4,-7.12)) ;
#116905=CARTESIAN_POINT('',(0.600000000000001,0.4,-7.12)) ;
#116906=CARTESIAN_POINT('',(0.500000000000001,-2.,-7.12)) ;
#116907=CARTESIAN_POINT('Origin',(0.600000000000001,-2.,-6.245)) ;
#116908=CARTESIAN_POINT('',(0.500000000000001,-2.,-6.345)) ;
#116909=CARTESIAN_POINT('',(-0.899999999999999,-2.,-6.345)) ;
#116910=CARTESIAN_POINT('',(-0.999999999999999,-2.,-6.345)) ;
#116911=CARTESIAN_POINT('',(-0.899999999999999,-2.,-7.02)) ;
#116912=CARTESIAN_POINT('',(-0.899999999999999,-2.,-7.12)) ;
#116913=CARTESIAN_POINT('',(0.500000000000001,-2.,-7.02)) ;
#116914=CARTESIAN_POINT('',(0.600000000000001,-2.,-7.02)) ;
#116915=CARTESIAN_POINT('',(0.500000000000001,-2.,-6.245)) ;
#116916=CARTESIAN_POINT('Origin',(0.600000000000001,-2.,-11.93)) ;
#116917=CARTESIAN_POINT('',(0.500000000000001,-2.,-12.03)) ;
#116918=CARTESIAN_POINT('',(-0.899999999999999,-2.,-12.03)) ;
#116919=CARTESIAN_POINT('',(0.600000000000001,-2.,-12.03)) ;
#116920=CARTESIAN_POINT('',(-0.899999999999999,-2.,-12.705)) ;
#116921=CARTESIAN_POINT('',(-0.899999999999999,-2.,-12.805)) ;
#116922=CARTESIAN_POINT('',(0.500000000000001,-2.,-12.705)) ;
#116923=CARTESIAN_POINT('',(0.600000000000001,-2.,-12.705)) ;
#116924=CARTESIAN_POINT('',(0.500000000000001,-2.,-11.93)) ;
#116925=CARTESIAN_POINT('Origin',(0.600000000000001,0.5,-11.93)) ;
#116926=CARTESIAN_POINT('',(-0.899999999999999,0.4,-11.93)) ;
#116927=CARTESIAN_POINT('',(-0.999999999999999,0.4,-11.93)) ;
#116928=CARTESIAN_POINT('',(-0.899999999999999,-1.9,-11.93)) ;
#116929=CARTESIAN_POINT('',(-0.899999999999999,-2.,-11.93)) ;
#116930=CARTESIAN_POINT('',(0.600000000000001,-1.9,-11.93)) ;
#116931=CARTESIAN_POINT('Origin',(0.600000000000001,0.5,-10.93)) ;
#116932=CARTESIAN_POINT('',(0.500000000000001,0.5,-11.03)) ;
#116933=CARTESIAN_POINT('',(-0.899999999999999,0.5,-11.03)) ;
#116934=CARTESIAN_POINT('',(-0.999999999999999,0.5,-11.03)) ;
#116935=CARTESIAN_POINT('',(-0.899999999999999,0.5,-11.83)) ;
#116936=CARTESIAN_POINT('',(-0.899999999999999,0.5,-11.93)) ;
#116937=CARTESIAN_POINT('',(0.500000000000001,0.5,-11.83)) ;
#116938=CARTESIAN_POINT('',(0.600000000000001,0.5,-11.83)) ;
#116939=CARTESIAN_POINT('',(0.500000000000001,0.5,-10.93)) ;
#116940=CARTESIAN_POINT('Origin',(0.600000000000001,-2.,-10.93)) ;
#116941=CARTESIAN_POINT('',(0.500000000000001,-1.9,-10.93)) ;
#116942=CARTESIAN_POINT('',(-0.899999999999999,-1.9,-10.93)) ;
#116943=CARTESIAN_POINT('',(0.600000000000001,-1.9,-10.93)) ;
#116944=CARTESIAN_POINT('',(-0.899999999999999,0.4,-10.93)) ;
#116945=CARTESIAN_POINT('',(-0.899999999999999,0.5,-10.93)) ;
#116946=CARTESIAN_POINT('',(0.500000000000001,0.4,-10.93)) ;
#116947=CARTESIAN_POINT('',(0.600000000000001,0.4,-10.93)) ;
#116948=CARTESIAN_POINT('',(0.500000000000001,-2.,-10.93)) ;
#116949=CARTESIAN_POINT('Origin',(0.600000000000001,-2.,-10.055)) ;
#116950=CARTESIAN_POINT('',(0.500000000000001,-2.,-10.155)) ;
#116951=CARTESIAN_POINT('',(-0.899999999999999,-2.,-10.155)) ;
#116952=CARTESIAN_POINT('',(-0.999999999999999,-2.,-10.155)) ;
#116953=CARTESIAN_POINT('',(-0.899999999999999,-2.,-10.83)) ;
#116954=CARTESIAN_POINT('',(-0.899999999999999,-2.,-10.93)) ;
#116955=CARTESIAN_POINT('',(0.500000000000001,-2.,-10.83)) ;
#116956=CARTESIAN_POINT('',(0.600000000000001,-2.,-10.83)) ;
#116957=CARTESIAN_POINT('',(0.500000000000001,-2.,-10.055)) ;
#116958=CARTESIAN_POINT('Origin',(0.600000000000001,-2.,-15.74)) ;
#116959=CARTESIAN_POINT('',(0.500000000000001,-2.,-15.84)) ;
#116960=CARTESIAN_POINT('',(-0.899999999999999,-2.,-15.84)) ;
#116961=CARTESIAN_POINT('',(0.600000000000001,-2.,-15.84)) ;
#116962=CARTESIAN_POINT('',(-0.899999999999999,-2.,-16.515)) ;
#116963=CARTESIAN_POINT('',(-0.899999999999999,-2.,-16.615)) ;
#116964=CARTESIAN_POINT('',(0.500000000000001,-2.,-16.515)) ;
#116965=CARTESIAN_POINT('',(0.600000000000001,-2.,-16.515)) ;
#116966=CARTESIAN_POINT('',(0.500000000000001,-2.,-15.74)) ;
#116967=CARTESIAN_POINT('Origin',(0.600000000000001,0.5,-15.74)) ;
#116968=CARTESIAN_POINT('',(-0.899999999999999,0.4,-15.74)) ;
#116969=CARTESIAN_POINT('',(-0.999999999999999,0.4,-15.74)) ;
#116970=CARTESIAN_POINT('',(-0.899999999999999,-1.9,-15.74)) ;
#116971=CARTESIAN_POINT('',(-0.899999999999999,-2.,-15.74)) ;
#116972=CARTESIAN_POINT('',(0.600000000000001,-1.9,-15.74)) ;
#116973=CARTESIAN_POINT('Origin',(0.600000000000001,0.5,-14.74)) ;
#116974=CARTESIAN_POINT('',(0.500000000000001,0.5,-14.84)) ;
#116975=CARTESIAN_POINT('',(-0.899999999999999,0.5,-14.84)) ;
#116976=CARTESIAN_POINT('',(-0.999999999999999,0.5,-14.84)) ;
#116977=CARTESIAN_POINT('',(-0.899999999999999,0.5,-15.64)) ;
#116978=CARTESIAN_POINT('',(-0.899999999999999,0.5,-15.74)) ;
#116979=CARTESIAN_POINT('',(0.500000000000001,0.5,-15.64)) ;
#116980=CARTESIAN_POINT('',(0.600000000000001,0.5,-15.64)) ;
#116981=CARTESIAN_POINT('',(0.500000000000001,0.5,-14.74)) ;
#116982=CARTESIAN_POINT('Origin',(0.600000000000001,-2.,-14.74)) ;
#116983=CARTESIAN_POINT('',(0.500000000000001,-1.9,-14.74)) ;
#116984=CARTESIAN_POINT('',(-0.899999999999999,-1.9,-14.74)) ;
#116985=CARTESIAN_POINT('',(0.600000000000001,-1.9,-14.74)) ;
#116986=CARTESIAN_POINT('',(-0.899999999999999,0.4,-14.74)) ;
#116987=CARTESIAN_POINT('',(-0.899999999999999,0.5,-14.74)) ;
#116988=CARTESIAN_POINT('',(0.500000000000001,0.4,-14.74)) ;
#116989=CARTESIAN_POINT('',(0.600000000000001,0.4,-14.74)) ;
#116990=CARTESIAN_POINT('',(0.500000000000001,-2.,-14.74)) ;
#116991=CARTESIAN_POINT('Origin',(0.600000000000001,-2.,-13.865)) ;
#116992=CARTESIAN_POINT('',(0.500000000000001,-2.,-13.965)) ;
#116993=CARTESIAN_POINT('',(-0.899999999999999,-2.,-13.965)) ;
#116994=CARTESIAN_POINT('',(-0.999999999999999,-2.,-13.965)) ;
#116995=CARTESIAN_POINT('',(-0.899999999999999,-2.,-14.64)) ;
#116996=CARTESIAN_POINT('',(-0.899999999999999,-2.,-14.74)) ;
#116997=CARTESIAN_POINT('',(0.500000000000001,-2.,-14.64)) ;
#116998=CARTESIAN_POINT('',(0.600000000000001,-2.,-14.64)) ;
#116999=CARTESIAN_POINT('',(0.500000000000001,-2.,-13.865)) ;
#117000=CARTESIAN_POINT('Origin',(0.600000000000001,-2.,-19.55)) ;
#117001=CARTESIAN_POINT('',(0.500000000000001,-2.,-19.65)) ;
#117002=CARTESIAN_POINT('',(-0.899999999999999,-2.,-19.65)) ;
#117003=CARTESIAN_POINT('',(0.600000000000001,-2.,-19.65)) ;
#117004=CARTESIAN_POINT('',(-0.899999999999999,-2.,-20.325)) ;
#117005=CARTESIAN_POINT('',(-0.899999999999999,-2.,-20.425)) ;
#117006=CARTESIAN_POINT('',(0.500000000000001,-2.,-20.325)) ;
#117007=CARTESIAN_POINT('',(0.600000000000001,-2.,-20.325)) ;
#117008=CARTESIAN_POINT('',(0.500000000000001,-2.,-19.55)) ;
#117009=CARTESIAN_POINT('Origin',(0.600000000000001,0.5,-19.55)) ;
#117010=CARTESIAN_POINT('',(-0.899999999999999,0.4,-19.55)) ;
#117011=CARTESIAN_POINT('',(-0.999999999999999,0.4,-19.55)) ;
#117012=CARTESIAN_POINT('',(-0.899999999999999,-1.9,-19.55)) ;
#117013=CARTESIAN_POINT('',(-0.899999999999999,-2.,-19.55)) ;
#117014=CARTESIAN_POINT('',(0.600000000000001,-1.9,-19.55)) ;
#117015=CARTESIAN_POINT('Origin',(0.600000000000001,0.5,-18.55)) ;
#117016=CARTESIAN_POINT('',(0.500000000000001,0.5,-18.65)) ;
#117017=CARTESIAN_POINT('',(-0.899999999999999,0.5,-18.65)) ;
#117018=CARTESIAN_POINT('',(-0.999999999999999,0.5,-18.65)) ;
#117019=CARTESIAN_POINT('',(-0.899999999999999,0.5,-19.45)) ;
#117020=CARTESIAN_POINT('',(-0.899999999999999,0.5,-19.55)) ;
#117021=CARTESIAN_POINT('',(0.500000000000001,0.5,-19.45)) ;
#117022=CARTESIAN_POINT('',(0.600000000000001,0.5,-19.45)) ;
#117023=CARTESIAN_POINT('',(0.500000000000001,0.5,-18.55)) ;
#117024=CARTESIAN_POINT('Origin',(0.600000000000001,-2.,-18.55)) ;
#117025=CARTESIAN_POINT('',(0.500000000000001,-1.9,-18.55)) ;
#117026=CARTESIAN_POINT('',(-0.899999999999999,-1.9,-18.55)) ;
#117027=CARTESIAN_POINT('',(0.600000000000001,-1.9,-18.55)) ;
#117028=CARTESIAN_POINT('',(-0.899999999999999,0.4,-18.55)) ;
#117029=CARTESIAN_POINT('',(-0.899999999999999,0.5,-18.55)) ;
#117030=CARTESIAN_POINT('',(0.500000000000001,0.4,-18.55)) ;
#117031=CARTESIAN_POINT('',(0.600000000000001,0.4,-18.55)) ;
#117032=CARTESIAN_POINT('',(0.500000000000001,-2.,-18.55)) ;
#117033=CARTESIAN_POINT('Origin',(0.600000000000001,-2.,-17.675)) ;
#117034=CARTESIAN_POINT('',(0.500000000000001,-2.,-17.775)) ;
#117035=CARTESIAN_POINT('',(-0.899999999999999,-2.,-17.775)) ;
#117036=CARTESIAN_POINT('',(-0.999999999999999,-2.,-17.775)) ;
#117037=CARTESIAN_POINT('',(-0.899999999999999,-2.,-18.45)) ;
#117038=CARTESIAN_POINT('',(-0.899999999999999,-2.,-18.55)) ;
#117039=CARTESIAN_POINT('',(0.500000000000001,-2.,-18.45)) ;
#117040=CARTESIAN_POINT('',(0.600000000000001,-2.,-18.45)) ;
#117041=CARTESIAN_POINT('',(0.500000000000001,-2.,-17.675)) ;
#117042=CARTESIAN_POINT('Origin',(0.600000000000001,-2.,-23.36)) ;
#117043=CARTESIAN_POINT('',(0.500000000000001,-2.,-23.46)) ;
#117044=CARTESIAN_POINT('',(-0.899999999999999,-2.,-23.46)) ;
#117045=CARTESIAN_POINT('',(0.600000000000001,-2.,-23.46)) ;
#117046=CARTESIAN_POINT('',(-0.899999999999999,-2.,-24.135)) ;
#117047=CARTESIAN_POINT('',(-0.899999999999999,-2.,-24.235)) ;
#117048=CARTESIAN_POINT('',(0.500000000000001,-2.,-24.135)) ;
#117049=CARTESIAN_POINT('',(0.600000000000001,-2.,-24.135)) ;
#117050=CARTESIAN_POINT('',(0.500000000000001,-2.,-23.36)) ;
#117051=CARTESIAN_POINT('Origin',(0.600000000000001,0.5,-23.36)) ;
#117052=CARTESIAN_POINT('',(-0.899999999999999,0.4,-23.36)) ;
#117053=CARTESIAN_POINT('',(-0.999999999999999,0.4,-23.36)) ;
#117054=CARTESIAN_POINT('',(-0.899999999999999,-1.9,-23.36)) ;
#117055=CARTESIAN_POINT('',(-0.899999999999999,-2.,-23.36)) ;
#117056=CARTESIAN_POINT('',(0.600000000000001,-1.9,-23.36)) ;
#117057=CARTESIAN_POINT('Origin',(0.600000000000001,0.5,-22.36)) ;
#117058=CARTESIAN_POINT('',(0.500000000000001,0.5,-22.46)) ;
#117059=CARTESIAN_POINT('',(-0.899999999999999,0.5,-22.46)) ;
#117060=CARTESIAN_POINT('',(-0.999999999999999,0.5,-22.46)) ;
#117061=CARTESIAN_POINT('',(-0.899999999999999,0.5,-23.26)) ;
#117062=CARTESIAN_POINT('',(-0.899999999999999,0.5,-23.36)) ;
#117063=CARTESIAN_POINT('',(0.500000000000001,0.5,-23.26)) ;
#117064=CARTESIAN_POINT('',(0.600000000000001,0.5,-23.26)) ;
#117065=CARTESIAN_POINT('',(0.500000000000001,0.5,-22.36)) ;
#117066=CARTESIAN_POINT('Origin',(0.600000000000001,-2.,-22.36)) ;
#117067=CARTESIAN_POINT('',(0.500000000000001,-1.9,-22.36)) ;
#117068=CARTESIAN_POINT('',(-0.899999999999999,-1.9,-22.36)) ;
#117069=CARTESIAN_POINT('',(0.600000000000001,-1.9,-22.36)) ;
#117070=CARTESIAN_POINT('',(-0.899999999999999,0.4,-22.36)) ;
#117071=CARTESIAN_POINT('',(-0.899999999999999,0.5,-22.36)) ;
#117072=CARTESIAN_POINT('',(0.500000000000001,0.4,-22.36)) ;
#117073=CARTESIAN_POINT('',(0.600000000000001,0.4,-22.36)) ;
#117074=CARTESIAN_POINT('',(0.500000000000001,-2.,-22.36)) ;
#117075=CARTESIAN_POINT('Origin',(0.600000000000001,-2.,-21.485)) ;
#117076=CARTESIAN_POINT('',(0.500000000000001,-2.,-21.585)) ;
#117077=CARTESIAN_POINT('',(-0.899999999999999,-2.,-21.585)) ;
#117078=CARTESIAN_POINT('',(-0.999999999999999,-2.,-21.585)) ;
#117079=CARTESIAN_POINT('',(-0.899999999999999,-2.,-22.26)) ;
#117080=CARTESIAN_POINT('',(-0.899999999999999,-2.,-22.36)) ;
#117081=CARTESIAN_POINT('',(0.500000000000001,-2.,-22.26)) ;
#117082=CARTESIAN_POINT('',(0.600000000000001,-2.,-22.26)) ;
#117083=CARTESIAN_POINT('',(0.500000000000001,-2.,-21.485)) ;
#117084=CARTESIAN_POINT('Origin',(0.600000000000001,-2.,-27.17)) ;
#117085=CARTESIAN_POINT('',(0.500000000000001,-2.,-27.27)) ;
#117086=CARTESIAN_POINT('',(-0.899999999999999,-2.,-27.27)) ;
#117087=CARTESIAN_POINT('',(0.600000000000001,-2.,-27.27)) ;
#117088=CARTESIAN_POINT('',(-0.899999999999999,-2.,-27.945)) ;
#117089=CARTESIAN_POINT('',(-0.899999999999999,-2.,-28.045)) ;
#117090=CARTESIAN_POINT('',(0.500000000000001,-2.,-27.945)) ;
#117091=CARTESIAN_POINT('',(0.600000000000001,-2.,-27.945)) ;
#117092=CARTESIAN_POINT('',(0.500000000000001,-2.,-27.17)) ;
#117093=CARTESIAN_POINT('Origin',(0.600000000000001,0.5,-27.17)) ;
#117094=CARTESIAN_POINT('',(-0.899999999999999,0.4,-27.17)) ;
#117095=CARTESIAN_POINT('',(-0.999999999999999,0.4,-27.17)) ;
#117096=CARTESIAN_POINT('',(-0.899999999999999,-1.9,-27.17)) ;
#117097=CARTESIAN_POINT('',(-0.899999999999999,-2.,-27.17)) ;
#117098=CARTESIAN_POINT('',(0.600000000000001,-1.9,-27.17)) ;
#117099=CARTESIAN_POINT('Origin',(0.600000000000001,0.5,-26.17)) ;
#117100=CARTESIAN_POINT('',(0.500000000000001,0.5,-26.27)) ;
#117101=CARTESIAN_POINT('',(-0.899999999999999,0.5,-26.27)) ;
#117102=CARTESIAN_POINT('',(-0.999999999999999,0.5,-26.27)) ;
#117103=CARTESIAN_POINT('',(-0.899999999999999,0.5,-27.07)) ;
#117104=CARTESIAN_POINT('',(-0.899999999999999,0.5,-27.17)) ;
#117105=CARTESIAN_POINT('',(0.500000000000001,0.5,-27.07)) ;
#117106=CARTESIAN_POINT('',(0.600000000000001,0.5,-27.07)) ;
#117107=CARTESIAN_POINT('',(0.500000000000001,0.5,-26.17)) ;
#117108=CARTESIAN_POINT('Origin',(0.600000000000001,-2.,-26.17)) ;
#117109=CARTESIAN_POINT('',(0.500000000000001,-1.9,-26.17)) ;
#117110=CARTESIAN_POINT('',(-0.899999999999999,-1.9,-26.17)) ;
#117111=CARTESIAN_POINT('',(0.600000000000001,-1.9,-26.17)) ;
#117112=CARTESIAN_POINT('',(-0.899999999999999,0.4,-26.17)) ;
#117113=CARTESIAN_POINT('',(-0.899999999999999,0.5,-26.17)) ;
#117114=CARTESIAN_POINT('',(0.500000000000001,0.4,-26.17)) ;
#117115=CARTESIAN_POINT('',(0.600000000000001,0.4,-26.17)) ;
#117116=CARTESIAN_POINT('',(0.500000000000001,-2.,-26.17)) ;
#117117=CARTESIAN_POINT('Origin',(0.600000000000001,-2.,-25.295)) ;
#117118=CARTESIAN_POINT('',(0.500000000000001,-2.,-25.395)) ;
#117119=CARTESIAN_POINT('',(-0.899999999999999,-2.,-25.395)) ;
#117120=CARTESIAN_POINT('',(-0.999999999999999,-2.,-25.395)) ;
#117121=CARTESIAN_POINT('',(-0.899999999999999,-2.,-26.07)) ;
#117122=CARTESIAN_POINT('',(-0.899999999999999,-2.,-26.17)) ;
#117123=CARTESIAN_POINT('',(0.500000000000001,-2.,-26.07)) ;
#117124=CARTESIAN_POINT('',(0.600000000000001,-2.,-26.07)) ;
#117125=CARTESIAN_POINT('',(0.500000000000001,-2.,-25.295)) ;
#117126=CARTESIAN_POINT('Origin',(0.600000000000001,-2.,-30.98)) ;
#117127=CARTESIAN_POINT('',(0.500000000000001,-2.,-31.08)) ;
#117128=CARTESIAN_POINT('',(-0.899999999999999,-2.,-31.08)) ;
#117129=CARTESIAN_POINT('',(0.600000000000001,-2.,-31.08)) ;
#117130=CARTESIAN_POINT('',(-0.899999999999999,-2.,-31.755)) ;
#117131=CARTESIAN_POINT('',(-0.899999999999999,-2.,-31.855)) ;
#117132=CARTESIAN_POINT('',(0.500000000000001,-2.,-31.755)) ;
#117133=CARTESIAN_POINT('',(0.600000000000001,-2.,-31.755)) ;
#117134=CARTESIAN_POINT('',(0.500000000000001,-2.,-30.98)) ;
#117135=CARTESIAN_POINT('Origin',(0.600000000000001,0.5,-30.98)) ;
#117136=CARTESIAN_POINT('',(-0.899999999999999,0.4,-30.98)) ;
#117137=CARTESIAN_POINT('',(-0.999999999999999,0.4,-30.98)) ;
#117138=CARTESIAN_POINT('',(-0.899999999999999,-1.9,-30.98)) ;
#117139=CARTESIAN_POINT('',(-0.899999999999999,-2.,-30.98)) ;
#117140=CARTESIAN_POINT('',(0.600000000000001,-1.9,-30.98)) ;
#117141=CARTESIAN_POINT('Origin',(0.600000000000001,0.5,-29.98)) ;
#117142=CARTESIAN_POINT('',(0.500000000000001,0.5,-30.08)) ;
#117143=CARTESIAN_POINT('',(-0.899999999999999,0.5,-30.08)) ;
#117144=CARTESIAN_POINT('',(-0.999999999999999,0.5,-30.08)) ;
#117145=CARTESIAN_POINT('',(-0.899999999999999,0.5,-30.88)) ;
#117146=CARTESIAN_POINT('',(-0.899999999999999,0.5,-30.98)) ;
#117147=CARTESIAN_POINT('',(0.500000000000001,0.5,-30.88)) ;
#117148=CARTESIAN_POINT('',(0.600000000000001,0.5,-30.88)) ;
#117149=CARTESIAN_POINT('',(0.500000000000001,0.5,-29.98)) ;
#117150=CARTESIAN_POINT('Origin',(0.600000000000001,-2.,-29.98)) ;
#117151=CARTESIAN_POINT('',(0.500000000000001,-1.9,-29.98)) ;
#117152=CARTESIAN_POINT('',(-0.899999999999999,-1.9,-29.98)) ;
#117153=CARTESIAN_POINT('',(0.600000000000001,-1.9,-29.98)) ;
#117154=CARTESIAN_POINT('',(-0.899999999999999,0.4,-29.98)) ;
#117155=CARTESIAN_POINT('',(-0.899999999999999,0.5,-29.98)) ;
#117156=CARTESIAN_POINT('',(0.500000000000001,0.4,-29.98)) ;
#117157=CARTESIAN_POINT('',(0.600000000000001,0.4,-29.98)) ;
#117158=CARTESIAN_POINT('',(0.500000000000001,-2.,-29.98)) ;
#117159=CARTESIAN_POINT('Origin',(0.600000000000001,-2.,-29.105)) ;
#117160=CARTESIAN_POINT('',(0.500000000000001,-2.,-29.205)) ;
#117161=CARTESIAN_POINT('',(-0.899999999999999,-2.,-29.205)) ;
#117162=CARTESIAN_POINT('',(-0.999999999999999,-2.,-29.205)) ;
#117163=CARTESIAN_POINT('',(-0.899999999999999,-2.,-29.88)) ;
#117164=CARTESIAN_POINT('',(-0.899999999999999,-2.,-29.98)) ;
#117165=CARTESIAN_POINT('',(0.500000000000001,-2.,-29.88)) ;
#117166=CARTESIAN_POINT('',(0.600000000000001,-2.,-29.88)) ;
#117167=CARTESIAN_POINT('',(0.500000000000001,-2.,-29.105)) ;
#117168=CARTESIAN_POINT('Origin',(0.600000000000001,-2.,-34.79)) ;
#117169=CARTESIAN_POINT('',(0.500000000000001,-2.,-34.89)) ;
#117170=CARTESIAN_POINT('',(-0.899999999999999,-2.,-34.89)) ;
#117171=CARTESIAN_POINT('',(0.600000000000001,-2.,-34.89)) ;
#117172=CARTESIAN_POINT('',(-0.899999999999999,-2.,-35.565)) ;
#117173=CARTESIAN_POINT('',(-0.899999999999999,-2.,-35.665)) ;
#117174=CARTESIAN_POINT('',(0.500000000000001,-2.,-35.565)) ;
#117175=CARTESIAN_POINT('',(0.600000000000001,-2.,-35.565)) ;
#117176=CARTESIAN_POINT('',(0.500000000000001,-2.,-34.79)) ;
#117177=CARTESIAN_POINT('Origin',(0.600000000000001,0.5,-34.79)) ;
#117178=CARTESIAN_POINT('',(-0.899999999999999,0.4,-34.79)) ;
#117179=CARTESIAN_POINT('',(-0.999999999999999,0.4,-34.79)) ;
#117180=CARTESIAN_POINT('',(-0.899999999999999,-1.9,-34.79)) ;
#117181=CARTESIAN_POINT('',(-0.899999999999999,-2.,-34.79)) ;
#117182=CARTESIAN_POINT('',(0.600000000000001,-1.9,-34.79)) ;
#117183=CARTESIAN_POINT('Origin',(0.600000000000001,0.5,-33.79)) ;
#117184=CARTESIAN_POINT('',(0.500000000000001,0.5,-33.89)) ;
#117185=CARTESIAN_POINT('',(-0.899999999999999,0.5,-33.89)) ;
#117186=CARTESIAN_POINT('',(-0.999999999999999,0.5,-33.89)) ;
#117187=CARTESIAN_POINT('',(-0.899999999999999,0.5,-34.69)) ;
#117188=CARTESIAN_POINT('',(-0.899999999999999,0.5,-34.79)) ;
#117189=CARTESIAN_POINT('',(0.500000000000001,0.5,-34.69)) ;
#117190=CARTESIAN_POINT('',(0.600000000000001,0.5,-34.69)) ;
#117191=CARTESIAN_POINT('',(0.500000000000001,0.5,-33.79)) ;
#117192=CARTESIAN_POINT('Origin',(0.600000000000001,-2.,-33.79)) ;
#117193=CARTESIAN_POINT('',(0.500000000000001,-1.9,-33.79)) ;
#117194=CARTESIAN_POINT('',(-0.899999999999999,-1.9,-33.79)) ;
#117195=CARTESIAN_POINT('',(0.600000000000001,-1.9,-33.79)) ;
#117196=CARTESIAN_POINT('',(-0.899999999999999,0.4,-33.79)) ;
#117197=CARTESIAN_POINT('',(-0.899999999999999,0.5,-33.79)) ;
#117198=CARTESIAN_POINT('',(0.500000000000001,0.4,-33.79)) ;
#117199=CARTESIAN_POINT('',(0.600000000000001,0.4,-33.79)) ;
#117200=CARTESIAN_POINT('',(0.500000000000001,-2.,-33.79)) ;
#117201=CARTESIAN_POINT('Origin',(0.600000000000001,-2.,-32.915)) ;
#117202=CARTESIAN_POINT('',(0.500000000000001,-2.,-33.015)) ;
#117203=CARTESIAN_POINT('',(-0.899999999999999,-2.,-33.015)) ;
#117204=CARTESIAN_POINT('',(-0.999999999999999,-2.,-33.015)) ;
#117205=CARTESIAN_POINT('',(-0.899999999999999,-2.,-33.69)) ;
#117206=CARTESIAN_POINT('',(-0.899999999999999,-2.,-33.79)) ;
#117207=CARTESIAN_POINT('',(0.500000000000001,-2.,-33.69)) ;
#117208=CARTESIAN_POINT('',(0.600000000000001,-2.,-33.69)) ;
#117209=CARTESIAN_POINT('',(0.500000000000001,-2.,-32.915)) ;
#117210=CARTESIAN_POINT('Origin',(1.4,2.1,-33.69)) ;
#117211=CARTESIAN_POINT('',(1.5,2.,-33.69)) ;
#117212=CARTESIAN_POINT('',(7.9,2.,-33.69)) ;
#117213=CARTESIAN_POINT('',(1.4,2.,-33.69)) ;
#117214=CARTESIAN_POINT('',(1.5,2.1,-33.79)) ;
#117215=CARTESIAN_POINT('Origin',(1.5,2.1,-33.69)) ;
#117216=CARTESIAN_POINT('',(7.9,2.1,-33.79)) ;
#117217=CARTESIAN_POINT('',(1.4,2.1,-33.79)) ;
#117218=CARTESIAN_POINT('Origin',(7.9,2.1,-33.69)) ;
#117219=CARTESIAN_POINT('Origin',(1.4,2.4,-33.79)) ;
#117220=CARTESIAN_POINT('',(1.5,2.4,-33.79)) ;
#117221=CARTESIAN_POINT('',(1.5,2.4,-33.79)) ;
#117222=CARTESIAN_POINT('',(7.9,2.4,-33.79)) ;
#117223=CARTESIAN_POINT('',(1.4,2.4,-33.79)) ;
#117224=CARTESIAN_POINT('',(7.9,2.1,-33.79)) ;
#117225=CARTESIAN_POINT('Origin',(1.4,2.4,-33.69)) ;
#117226=CARTESIAN_POINT('',(1.5,2.5,-33.69)) ;
#117227=CARTESIAN_POINT('Origin',(1.5,2.4,-33.69)) ;
#117228=CARTESIAN_POINT('',(7.9,2.5,-33.69)) ;
#117229=CARTESIAN_POINT('',(1.4,2.5,-33.69)) ;
#117230=CARTESIAN_POINT('Origin',(7.9,2.4,-33.69)) ;
#117231=CARTESIAN_POINT('Origin',(1.4,2.5,-33.5814213562373)) ;
#117232=CARTESIAN_POINT('',(1.5,2.5,-33.5814213562373)) ;
#117233=CARTESIAN_POINT('',(1.5,2.5,-33.5814213562373)) ;
#117234=CARTESIAN_POINT('',(7.9,2.5,-33.5814213562373)) ;
#117235=CARTESIAN_POINT('',(1.4,2.5,-33.5814213562373)) ;
#117236=CARTESIAN_POINT('',(7.9,2.5,-33.69)) ;
#117237=CARTESIAN_POINT('Origin',(1.4,2.6,-33.5814213562373)) ;
#117238=CARTESIAN_POINT('',(1.5,2.52928932188135,-33.5107106781187)) ;
#117239=CARTESIAN_POINT('Origin',(1.5,2.6,-33.5814213562373)) ;
#117240=CARTESIAN_POINT('',(7.9,2.52928932188135,-33.5107106781187)) ;
#117241=CARTESIAN_POINT('',(1.4,2.52928932188135,-33.5107106781187)) ;
#117242=CARTESIAN_POINT('Origin',(7.9,2.6,-33.5814213562373)) ;
#117243=CARTESIAN_POINT('Origin',(1.4,3.07928932188135,-32.9607106781187)) ;
#117244=CARTESIAN_POINT('',(1.5,3.07928932188135,-32.9607106781187)) ;
#117245=CARTESIAN_POINT('',(7.9,3.07928932188135,-32.9607106781187)) ;
#117246=CARTESIAN_POINT('',(1.4,3.07928932188135,-32.9607106781187)) ;
#117247=CARTESIAN_POINT('',(7.9,2.52928932188135,-33.5107106781187)) ;
#117248=CARTESIAN_POINT('Origin',(1.4,3.15,-33.0314213562373)) ;
#117249=CARTESIAN_POINT('',(7.9,3.25,-33.0314213562373)) ;
#117250=CARTESIAN_POINT('',(1.4,3.25,-33.0314213562373)) ;
#117251=CARTESIAN_POINT('Origin',(7.9,3.15,-33.0314213562373)) ;
#117252=CARTESIAN_POINT('Origin',(1.4,3.25,-35.5485786437627)) ;
#117253=CARTESIAN_POINT('',(1.5,3.25,-35.5485786437627)) ;
#117254=CARTESIAN_POINT('',(7.9,3.25,-33.0314213562373)) ;
#117255=CARTESIAN_POINT('Origin',(1.4,2.52928932188134,-35.0692893218813)) ;
#117256=CARTESIAN_POINT('',(1.5,2.52928932188134,-35.0692893218813)) ;
#117257=CARTESIAN_POINT('',(1.5,2.52928932188134,-35.0692893218813)) ;
#117258=CARTESIAN_POINT('',(7.9,2.52928932188134,-35.0692893218813)) ;
#117259=CARTESIAN_POINT('',(1.4,2.52928932188134,-35.0692893218813)) ;
#117260=CARTESIAN_POINT('',(7.9,3.07928932188135,-35.6192893218813)) ;
#117261=CARTESIAN_POINT('Origin',(1.4,2.6,-34.9985786437627)) ;
#117262=CARTESIAN_POINT('',(1.5,2.5,-34.9985786437627)) ;
#117263=CARTESIAN_POINT('Origin',(1.5,2.6,-34.9985786437627)) ;
#117264=CARTESIAN_POINT('',(7.9,2.5,-34.9985786437627)) ;
#117265=CARTESIAN_POINT('',(1.4,2.5,-34.9985786437627)) ;
#117266=CARTESIAN_POINT('Origin',(7.9,2.6,-34.9985786437627)) ;
#117267=CARTESIAN_POINT('Origin',(1.4,2.5,-34.89)) ;
#117268=CARTESIAN_POINT('',(1.5,2.5,-34.89)) ;
#117269=CARTESIAN_POINT('',(1.5,2.5,-34.89)) ;
#117270=CARTESIAN_POINT('',(7.9,2.5,-34.89)) ;
#117271=CARTESIAN_POINT('',(1.4,2.5,-34.89)) ;
#117272=CARTESIAN_POINT('',(7.9,2.5,-34.9985786437627)) ;
#117273=CARTESIAN_POINT('Origin',(1.4,2.4,-34.89)) ;
#117274=CARTESIAN_POINT('',(1.5,2.4,-34.79)) ;
#117275=CARTESIAN_POINT('Origin',(1.5,2.4,-34.89)) ;
#117276=CARTESIAN_POINT('',(7.9,2.4,-34.79)) ;
#117277=CARTESIAN_POINT('',(1.4,2.4,-34.79)) ;
#117278=CARTESIAN_POINT('Origin',(7.9,2.4,-34.89)) ;
#117279=CARTESIAN_POINT('Origin',(1.4,2.1,-34.79)) ;
#117280=CARTESIAN_POINT('',(1.5,2.1,-34.79)) ;
#117281=CARTESIAN_POINT('',(1.5,2.1,-34.79)) ;
#117282=CARTESIAN_POINT('',(7.9,2.1,-34.79)) ;
#117283=CARTESIAN_POINT('',(1.4,2.1,-34.79)) ;
#117284=CARTESIAN_POINT('',(7.9,2.4,-34.79)) ;
#117285=CARTESIAN_POINT('Origin',(1.4,2.1,-34.89)) ;
#117286=CARTESIAN_POINT('',(1.5,2.,-34.89)) ;
#117287=CARTESIAN_POINT('Origin',(1.5,2.1,-34.89)) ;
#117288=CARTESIAN_POINT('',(7.9,2.,-34.89)) ;
#117289=CARTESIAN_POINT('',(1.4,2.,-34.89)) ;
#117290=CARTESIAN_POINT('Origin',(7.9,2.1,-34.89)) ;
#117291=CARTESIAN_POINT('Origin',(1.4,2.,-34.89)) ;
#117292=CARTESIAN_POINT('',(1.5,2.,-35.84)) ;
#117293=CARTESIAN_POINT('',(1.5,2.,-35.84)) ;
#117294=CARTESIAN_POINT('',(7.9,2.,-35.84)) ;
#117295=CARTESIAN_POINT('',(1.4,2.,-35.84)) ;
#117296=CARTESIAN_POINT('',(7.9,2.,-34.89)) ;
#117297=CARTESIAN_POINT('Origin',(1.4,1.9,-35.84)) ;
#117298=CARTESIAN_POINT('',(1.5,1.9,-35.94)) ;
#117299=CARTESIAN_POINT('Origin',(1.5,1.9,-35.84)) ;
#117300=CARTESIAN_POINT('',(7.9,1.9,-35.94)) ;
#117301=CARTESIAN_POINT('',(1.4,1.9,-35.94)) ;
#117302=CARTESIAN_POINT('Origin',(7.9,1.9,-35.84)) ;
#117303=CARTESIAN_POINT('Origin',(1.4,1.9,-35.94)) ;
#117304=CARTESIAN_POINT('',(1.5,-2.15,-35.94)) ;
#117305=CARTESIAN_POINT('',(1.5,-2.15,-35.94)) ;
#117306=CARTESIAN_POINT('',(7.9,-2.15,-35.94)) ;
#117307=CARTESIAN_POINT('',(1.4,-2.15,-35.94)) ;
#117308=CARTESIAN_POINT('',(7.9,1.9,-35.94)) ;
#117309=CARTESIAN_POINT('Origin',(1.4,-2.15,-35.84)) ;
#117310=CARTESIAN_POINT('',(1.5,-2.25,-35.84)) ;
#117311=CARTESIAN_POINT('Origin',(1.5,-2.15,-35.84)) ;
#117312=CARTESIAN_POINT('',(7.9,-2.25,-35.84)) ;
#117313=CARTESIAN_POINT('',(1.4,-2.25,-35.84)) ;
#117314=CARTESIAN_POINT('Origin',(7.9,-2.15,-35.84)) ;
#117315=CARTESIAN_POINT('Origin',(1.4,-2.25,-35.1931195934094)) ;
#117316=CARTESIAN_POINT('',(1.5,-2.25,-35.1931195934094)) ;
#117317=CARTESIAN_POINT('',(1.5,-2.25,-35.1931195934094)) ;
#117318=CARTESIAN_POINT('',(7.9,-2.25,-35.1931195934094)) ;
#117319=CARTESIAN_POINT('',(1.4,-2.25,-35.1931195934094)) ;
#117320=CARTESIAN_POINT('',(7.9,-2.25,-35.84)) ;
#117321=CARTESIAN_POINT('Origin',(1.4,-2.15,-35.1931195934094)) ;
#117322=CARTESIAN_POINT('',(1.5,-2.23576512455516,-35.1416964137135)) ;
#117323=CARTESIAN_POINT('Origin',(1.5,-2.15,-35.1931195934094)) ;
#117324=CARTESIAN_POINT('',(7.9,-2.23576512455516,-35.1416964137135)) ;
#117325=CARTESIAN_POINT('',(1.4,-2.23576512455516,-35.1416964137135)) ;
#117326=CARTESIAN_POINT('Origin',(7.9,-2.15,-35.1931195934094)) ;
#117327=CARTESIAN_POINT('Origin',(1.4,-3.65625,-34.29)) ;
#117328=CARTESIAN_POINT('',(1.5,-2.23576512455516,-33.4383035862865)) ;
#117329=CARTESIAN_POINT('Origin',(1.5,-3.65625,-34.29)) ;
#117330=CARTESIAN_POINT('',(7.9,-2.23576512455516,-33.4383035862865)) ;
#117331=CARTESIAN_POINT('',(1.4,-2.23576512455516,-33.4383035862865)) ;
#117332=CARTESIAN_POINT('Origin',(7.9,-3.65625,-34.29)) ;
#117333=CARTESIAN_POINT('Origin',(1.4,-2.15,-33.3868804065906)) ;
#117334=CARTESIAN_POINT('',(1.5,-2.25,-33.3868804065906)) ;
#117335=CARTESIAN_POINT('Origin',(1.5,-2.15,-33.3868804065906)) ;
#117336=CARTESIAN_POINT('',(7.9,-2.25,-33.3868804065906)) ;
#117337=CARTESIAN_POINT('',(1.4,-2.25,-33.3868804065906)) ;
#117338=CARTESIAN_POINT('Origin',(7.9,-2.15,-33.3868804065906)) ;
#117339=CARTESIAN_POINT('Origin',(1.4,-2.25,-32.74)) ;
#117340=CARTESIAN_POINT('',(1.5,-2.25,-32.74)) ;
#117341=CARTESIAN_POINT('',(1.5,-2.25,-32.74)) ;
#117342=CARTESIAN_POINT('',(7.9,-2.25,-32.74)) ;
#117343=CARTESIAN_POINT('',(1.4,-2.25,-32.74)) ;
#117344=CARTESIAN_POINT('',(7.9,-2.25,-33.3868804065906)) ;
#117345=CARTESIAN_POINT('Origin',(1.4,-2.15,-32.74)) ;
#117346=CARTESIAN_POINT('',(1.5,-2.15,-32.64)) ;
#117347=CARTESIAN_POINT('Origin',(1.5,-2.15,-32.74)) ;
#117348=CARTESIAN_POINT('',(7.9,-2.15,-32.64)) ;
#117349=CARTESIAN_POINT('',(1.4,-2.15,-32.64)) ;
#117350=CARTESIAN_POINT('Origin',(7.9,-2.15,-32.74)) ;
#117351=CARTESIAN_POINT('Origin',(1.4,1.9,-32.64)) ;
#117352=CARTESIAN_POINT('',(1.5,1.9,-32.64)) ;
#117353=CARTESIAN_POINT('',(1.5,1.9,-32.64)) ;
#117354=CARTESIAN_POINT('',(7.9,1.9,-32.64)) ;
#117355=CARTESIAN_POINT('',(1.4,1.9,-32.64)) ;
#117356=CARTESIAN_POINT('',(7.9,-2.15,-32.64)) ;
#117357=CARTESIAN_POINT('Origin',(1.4,1.9,-32.74)) ;
#117358=CARTESIAN_POINT('',(1.5,2.,-32.74)) ;
#117359=CARTESIAN_POINT('Origin',(1.5,1.9,-32.74)) ;
#117360=CARTESIAN_POINT('',(7.9,2.,-32.74)) ;
#117361=CARTESIAN_POINT('',(1.4,2.,-32.74)) ;
#117362=CARTESIAN_POINT('Origin',(7.9,1.9,-32.74)) ;
#117363=CARTESIAN_POINT('Origin',(1.4,2.,-32.74)) ;
#117364=CARTESIAN_POINT('',(1.5,2.,-33.69)) ;
#117365=CARTESIAN_POINT('',(7.9,2.,-32.74)) ;
#117366=CARTESIAN_POINT('Origin',(1.4,2.1,-33.69)) ;
#117367=CARTESIAN_POINT('',(1.4,2.6,-33.69)) ;
#117368=CARTESIAN_POINT('',(1.4,2.4,-33.89)) ;
#117369=CARTESIAN_POINT('Origin',(1.4,2.4,-33.69)) ;
#117370=CARTESIAN_POINT('',(1.4,2.1,-33.89)) ;
#117371=CARTESIAN_POINT('',(1.4,2.1,-33.89)) ;
#117372=CARTESIAN_POINT('',(1.4,1.9,-33.69)) ;
#117373=CARTESIAN_POINT('Origin',(1.4,2.1,-33.69)) ;
#117374=CARTESIAN_POINT('',(1.4,1.9,-32.74)) ;
#117375=CARTESIAN_POINT('',(1.4,1.9,-32.74)) ;
#117376=CARTESIAN_POINT('',(1.4,-2.15,-32.74)) ;
#117377=CARTESIAN_POINT('',(1.4,-2.15,-32.74)) ;
#117378=CARTESIAN_POINT('',(1.4,-2.15,-33.3868804065906)) ;
#117379=CARTESIAN_POINT('',(1.4,-2.15,-33.3868804065906)) ;
#117380=CARTESIAN_POINT('',(1.4,-2.15,-35.1931195934094)) ;
#117381=CARTESIAN_POINT('Origin',(1.4,-3.65625,-34.29)) ;
#117382=CARTESIAN_POINT('',(1.4,-2.15,-35.84)) ;
#117383=CARTESIAN_POINT('',(1.4,-2.15,-35.84)) ;
#117384=CARTESIAN_POINT('',(1.4,1.9,-35.84)) ;
#117385=CARTESIAN_POINT('',(1.4,1.9,-35.84)) ;
#117386=CARTESIAN_POINT('',(1.4,1.9,-34.89)) ;
#117387=CARTESIAN_POINT('',(1.4,1.9,-34.89)) ;
#117388=CARTESIAN_POINT('',(1.4,2.1,-34.69)) ;
#117389=CARTESIAN_POINT('Origin',(1.4,2.1,-34.89)) ;
#117390=CARTESIAN_POINT('',(1.4,2.4,-34.69)) ;
#117391=CARTESIAN_POINT('',(1.4,2.4,-34.69)) ;
#117392=CARTESIAN_POINT('',(1.4,2.6,-34.89)) ;
#117393=CARTESIAN_POINT('Origin',(1.4,2.4,-34.89)) ;
#117394=CARTESIAN_POINT('',(1.4,2.6,-34.9985786437627)) ;
#117395=CARTESIAN_POINT('',(1.4,2.6,-34.9985786437627)) ;
#117396=CARTESIAN_POINT('',(1.4,3.15,-35.5485786437627)) ;
#117397=CARTESIAN_POINT('',(1.4,3.15,-35.5485786437627)) ;
#117398=CARTESIAN_POINT('',(1.4,3.15,-33.0314213562373)) ;
#117399=CARTESIAN_POINT('',(1.4,2.6,-33.5814213562373)) ;
#117400=CARTESIAN_POINT('',(1.4,2.6,-33.5814213562373)) ;
#117401=CARTESIAN_POINT('',(1.4,2.6,-33.69)) ;
#117402=CARTESIAN_POINT('Origin',(1.4,2.1,-29.88)) ;
#117403=CARTESIAN_POINT('',(1.5,2.,-29.88)) ;
#117404=CARTESIAN_POINT('',(7.9,2.,-29.88)) ;
#117405=CARTESIAN_POINT('',(1.4,2.,-29.88)) ;
#117406=CARTESIAN_POINT('',(1.5,2.1,-29.98)) ;
#117407=CARTESIAN_POINT('Origin',(1.5,2.1,-29.88)) ;
#117408=CARTESIAN_POINT('',(7.9,2.1,-29.98)) ;
#117409=CARTESIAN_POINT('',(1.4,2.1,-29.98)) ;
#117410=CARTESIAN_POINT('Origin',(7.9,2.1,-29.88)) ;
#117411=CARTESIAN_POINT('Origin',(1.4,2.4,-29.98)) ;
#117412=CARTESIAN_POINT('',(1.5,2.4,-29.98)) ;
#117413=CARTESIAN_POINT('',(1.5,2.4,-29.98)) ;
#117414=CARTESIAN_POINT('',(7.9,2.4,-29.98)) ;
#117415=CARTESIAN_POINT('',(1.4,2.4,-29.98)) ;
#117416=CARTESIAN_POINT('',(7.9,2.1,-29.98)) ;
#117417=CARTESIAN_POINT('Origin',(1.4,2.4,-29.88)) ;
#117418=CARTESIAN_POINT('',(1.5,2.5,-29.88)) ;
#117419=CARTESIAN_POINT('Origin',(1.5,2.4,-29.88)) ;
#117420=CARTESIAN_POINT('',(7.9,2.5,-29.88)) ;
#117421=CARTESIAN_POINT('',(1.4,2.5,-29.88)) ;
#117422=CARTESIAN_POINT('Origin',(7.9,2.4,-29.88)) ;
#117423=CARTESIAN_POINT('Origin',(1.4,2.5,-29.7714213562373)) ;
#117424=CARTESIAN_POINT('',(1.5,2.5,-29.7714213562373)) ;
#117425=CARTESIAN_POINT('',(1.5,2.5,-29.7714213562373)) ;
#117426=CARTESIAN_POINT('',(7.9,2.5,-29.7714213562373)) ;
#117427=CARTESIAN_POINT('',(1.4,2.5,-29.7714213562373)) ;
#117428=CARTESIAN_POINT('',(7.9,2.5,-29.88)) ;
#117429=CARTESIAN_POINT('Origin',(1.4,2.6,-29.7714213562373)) ;
#117430=CARTESIAN_POINT('',(1.5,2.52928932188135,-29.7007106781187)) ;
#117431=CARTESIAN_POINT('Origin',(1.5,2.6,-29.7714213562373)) ;
#117432=CARTESIAN_POINT('',(7.9,2.52928932188135,-29.7007106781187)) ;
#117433=CARTESIAN_POINT('',(1.4,2.52928932188135,-29.7007106781187)) ;
#117434=CARTESIAN_POINT('Origin',(7.9,2.6,-29.7714213562373)) ;
#117435=CARTESIAN_POINT('Origin',(1.4,3.07928932188135,-29.1507106781187)) ;
#117436=CARTESIAN_POINT('',(1.5,3.07928932188135,-29.1507106781187)) ;
#117437=CARTESIAN_POINT('',(7.9,3.07928932188135,-29.1507106781187)) ;
#117438=CARTESIAN_POINT('',(1.4,3.07928932188135,-29.1507106781187)) ;
#117439=CARTESIAN_POINT('',(7.9,2.52928932188135,-29.7007106781187)) ;
#117440=CARTESIAN_POINT('Origin',(1.4,3.15,-29.2214213562373)) ;
#117441=CARTESIAN_POINT('',(7.9,3.25,-29.2214213562373)) ;
#117442=CARTESIAN_POINT('',(1.4,3.25,-29.2214213562373)) ;
#117443=CARTESIAN_POINT('Origin',(7.9,3.15,-29.2214213562373)) ;
#117444=CARTESIAN_POINT('Origin',(1.4,3.25,-31.7385786437627)) ;
#117445=CARTESIAN_POINT('',(1.5,3.25,-31.7385786437627)) ;
#117446=CARTESIAN_POINT('',(7.9,3.25,-29.2214213562373)) ;
#117447=CARTESIAN_POINT('Origin',(1.4,2.52928932188134,-31.2592893218813)) ;
#117448=CARTESIAN_POINT('',(1.5,2.52928932188134,-31.2592893218813)) ;
#117449=CARTESIAN_POINT('',(1.5,2.52928932188135,-31.2592893218813)) ;
#117450=CARTESIAN_POINT('',(7.9,2.52928932188134,-31.2592893218813)) ;
#117451=CARTESIAN_POINT('',(1.4,2.52928932188134,-31.2592893218813)) ;
#117452=CARTESIAN_POINT('',(7.9,3.07928932188135,-31.8092893218813)) ;
#117453=CARTESIAN_POINT('Origin',(1.4,2.6,-31.1885786437627)) ;
#117454=CARTESIAN_POINT('',(1.5,2.5,-31.1885786437627)) ;
#117455=CARTESIAN_POINT('Origin',(1.5,2.6,-31.1885786437627)) ;
#117456=CARTESIAN_POINT('',(7.9,2.5,-31.1885786437627)) ;
#117457=CARTESIAN_POINT('',(1.4,2.5,-31.1885786437627)) ;
#117458=CARTESIAN_POINT('Origin',(7.9,2.6,-31.1885786437627)) ;
#117459=CARTESIAN_POINT('Origin',(1.4,2.5,-31.08)) ;
#117460=CARTESIAN_POINT('',(1.5,2.5,-31.08)) ;
#117461=CARTESIAN_POINT('',(1.5,2.5,-31.08)) ;
#117462=CARTESIAN_POINT('',(7.9,2.5,-31.08)) ;
#117463=CARTESIAN_POINT('',(1.4,2.5,-31.08)) ;
#117464=CARTESIAN_POINT('',(7.9,2.5,-31.1885786437627)) ;
#117465=CARTESIAN_POINT('Origin',(1.4,2.4,-31.08)) ;
#117466=CARTESIAN_POINT('',(1.5,2.4,-30.98)) ;
#117467=CARTESIAN_POINT('Origin',(1.5,2.4,-31.08)) ;
#117468=CARTESIAN_POINT('',(7.9,2.4,-30.98)) ;
#117469=CARTESIAN_POINT('',(1.4,2.4,-30.98)) ;
#117470=CARTESIAN_POINT('Origin',(7.9,2.4,-31.08)) ;
#117471=CARTESIAN_POINT('Origin',(1.4,2.1,-30.98)) ;
#117472=CARTESIAN_POINT('',(1.5,2.1,-30.98)) ;
#117473=CARTESIAN_POINT('',(1.5,2.1,-30.98)) ;
#117474=CARTESIAN_POINT('',(7.9,2.1,-30.98)) ;
#117475=CARTESIAN_POINT('',(1.4,2.1,-30.98)) ;
#117476=CARTESIAN_POINT('',(7.9,2.4,-30.98)) ;
#117477=CARTESIAN_POINT('Origin',(1.4,2.1,-31.08)) ;
#117478=CARTESIAN_POINT('',(1.5,2.,-31.08)) ;
#117479=CARTESIAN_POINT('Origin',(1.5,2.1,-31.08)) ;
#117480=CARTESIAN_POINT('',(7.9,2.,-31.08)) ;
#117481=CARTESIAN_POINT('',(1.4,2.,-31.08)) ;
#117482=CARTESIAN_POINT('Origin',(7.9,2.1,-31.08)) ;
#117483=CARTESIAN_POINT('Origin',(1.4,2.,-31.08)) ;
#117484=CARTESIAN_POINT('',(1.5,2.,-32.03)) ;
#117485=CARTESIAN_POINT('',(1.5,2.,-32.03)) ;
#117486=CARTESIAN_POINT('',(7.9,2.,-32.03)) ;
#117487=CARTESIAN_POINT('',(1.4,2.,-32.03)) ;
#117488=CARTESIAN_POINT('',(7.9,2.,-31.08)) ;
#117489=CARTESIAN_POINT('Origin',(1.4,1.9,-32.03)) ;
#117490=CARTESIAN_POINT('',(1.5,1.9,-32.13)) ;
#117491=CARTESIAN_POINT('Origin',(1.5,1.9,-32.03)) ;
#117492=CARTESIAN_POINT('',(7.9,1.9,-32.13)) ;
#117493=CARTESIAN_POINT('',(1.4,1.9,-32.13)) ;
#117494=CARTESIAN_POINT('Origin',(7.9,1.9,-32.03)) ;
#117495=CARTESIAN_POINT('Origin',(1.4,1.9,-32.13)) ;
#117496=CARTESIAN_POINT('',(1.5,-2.15,-32.13)) ;
#117497=CARTESIAN_POINT('',(1.5,-2.15,-32.13)) ;
#117498=CARTESIAN_POINT('',(7.9,-2.15,-32.13)) ;
#117499=CARTESIAN_POINT('',(1.4,-2.15,-32.13)) ;
#117500=CARTESIAN_POINT('',(7.9,1.9,-32.13)) ;
#117501=CARTESIAN_POINT('Origin',(1.4,-2.15,-32.03)) ;
#117502=CARTESIAN_POINT('',(1.5,-2.25,-32.03)) ;
#117503=CARTESIAN_POINT('Origin',(1.5,-2.15,-32.03)) ;
#117504=CARTESIAN_POINT('',(7.9,-2.25,-32.03)) ;
#117505=CARTESIAN_POINT('',(1.4,-2.25,-32.03)) ;
#117506=CARTESIAN_POINT('Origin',(7.9,-2.15,-32.03)) ;
#117507=CARTESIAN_POINT('Origin',(1.4,-2.25,-31.3831195934094)) ;
#117508=CARTESIAN_POINT('',(1.5,-2.25,-31.3831195934094)) ;
#117509=CARTESIAN_POINT('',(1.5,-2.25,-31.3831195934094)) ;
#117510=CARTESIAN_POINT('',(7.9,-2.25,-31.3831195934094)) ;
#117511=CARTESIAN_POINT('',(1.4,-2.25,-31.3831195934094)) ;
#117512=CARTESIAN_POINT('',(7.9,-2.25,-32.03)) ;
#117513=CARTESIAN_POINT('Origin',(1.4,-2.15,-31.3831195934094)) ;
#117514=CARTESIAN_POINT('',(1.5,-2.23576512455516,-31.3316964137135)) ;
#117515=CARTESIAN_POINT('Origin',(1.5,-2.15,-31.3831195934094)) ;
#117516=CARTESIAN_POINT('',(7.9,-2.23576512455516,-31.3316964137135)) ;
#117517=CARTESIAN_POINT('',(1.4,-2.23576512455516,-31.3316964137135)) ;
#117518=CARTESIAN_POINT('Origin',(7.9,-2.15,-31.3831195934094)) ;
#117519=CARTESIAN_POINT('Origin',(1.4,-3.65625,-30.48)) ;
#117520=CARTESIAN_POINT('',(1.5,-2.23576512455516,-29.6283035862865)) ;
#117521=CARTESIAN_POINT('Origin',(1.5,-3.65625,-30.48)) ;
#117522=CARTESIAN_POINT('',(7.9,-2.23576512455516,-29.6283035862865)) ;
#117523=CARTESIAN_POINT('',(1.4,-2.23576512455516,-29.6283035862865)) ;
#117524=CARTESIAN_POINT('Origin',(7.9,-3.65625,-30.48)) ;
#117525=CARTESIAN_POINT('Origin',(1.4,-2.15,-29.5768804065906)) ;
#117526=CARTESIAN_POINT('',(1.5,-2.25,-29.5768804065906)) ;
#117527=CARTESIAN_POINT('Origin',(1.5,-2.15,-29.5768804065906)) ;
#117528=CARTESIAN_POINT('',(7.9,-2.25,-29.5768804065906)) ;
#117529=CARTESIAN_POINT('',(1.4,-2.25,-29.5768804065906)) ;
#117530=CARTESIAN_POINT('Origin',(7.9,-2.15,-29.5768804065906)) ;
#117531=CARTESIAN_POINT('Origin',(1.4,-2.25,-28.93)) ;
#117532=CARTESIAN_POINT('',(1.5,-2.25,-28.93)) ;
#117533=CARTESIAN_POINT('',(1.5,-2.25,-28.93)) ;
#117534=CARTESIAN_POINT('',(7.9,-2.25,-28.93)) ;
#117535=CARTESIAN_POINT('',(1.4,-2.25,-28.93)) ;
#117536=CARTESIAN_POINT('',(7.9,-2.25,-29.5768804065906)) ;
#117537=CARTESIAN_POINT('Origin',(1.4,-2.15,-28.93)) ;
#117538=CARTESIAN_POINT('',(1.5,-2.15,-28.83)) ;
#117539=CARTESIAN_POINT('Origin',(1.5,-2.15,-28.93)) ;
#117540=CARTESIAN_POINT('',(7.9,-2.15,-28.83)) ;
#117541=CARTESIAN_POINT('',(1.4,-2.15,-28.83)) ;
#117542=CARTESIAN_POINT('Origin',(7.9,-2.15,-28.93)) ;
#117543=CARTESIAN_POINT('Origin',(1.4,1.9,-28.83)) ;
#117544=CARTESIAN_POINT('',(1.5,1.9,-28.83)) ;
#117545=CARTESIAN_POINT('',(1.5,1.9,-28.83)) ;
#117546=CARTESIAN_POINT('',(7.9,1.9,-28.83)) ;
#117547=CARTESIAN_POINT('',(1.4,1.9,-28.83)) ;
#117548=CARTESIAN_POINT('',(7.9,-2.15,-28.83)) ;
#117549=CARTESIAN_POINT('Origin',(1.4,1.9,-28.93)) ;
#117550=CARTESIAN_POINT('',(1.5,2.,-28.93)) ;
#117551=CARTESIAN_POINT('Origin',(1.5,1.9,-28.93)) ;
#117552=CARTESIAN_POINT('',(7.9,2.,-28.93)) ;
#117553=CARTESIAN_POINT('',(1.4,2.,-28.93)) ;
#117554=CARTESIAN_POINT('Origin',(7.9,1.9,-28.93)) ;
#117555=CARTESIAN_POINT('Origin',(1.4,2.,-28.93)) ;
#117556=CARTESIAN_POINT('',(1.5,2.,-29.88)) ;
#117557=CARTESIAN_POINT('',(7.9,2.,-28.93)) ;
#117558=CARTESIAN_POINT('Origin',(1.4,2.1,-29.88)) ;
#117559=CARTESIAN_POINT('',(1.4,2.6,-29.88)) ;
#117560=CARTESIAN_POINT('',(1.4,2.4,-30.08)) ;
#117561=CARTESIAN_POINT('Origin',(1.4,2.4,-29.88)) ;
#117562=CARTESIAN_POINT('',(1.4,2.1,-30.08)) ;
#117563=CARTESIAN_POINT('',(1.4,2.1,-30.08)) ;
#117564=CARTESIAN_POINT('',(1.4,1.9,-29.88)) ;
#117565=CARTESIAN_POINT('Origin',(1.4,2.1,-29.88)) ;
#117566=CARTESIAN_POINT('',(1.4,1.9,-28.93)) ;
#117567=CARTESIAN_POINT('',(1.4,1.9,-28.93)) ;
#117568=CARTESIAN_POINT('',(1.4,-2.15,-28.93)) ;
#117569=CARTESIAN_POINT('',(1.4,-2.15,-28.93)) ;
#117570=CARTESIAN_POINT('',(1.4,-2.15,-29.5768804065906)) ;
#117571=CARTESIAN_POINT('',(1.4,-2.15,-29.5768804065906)) ;
#117572=CARTESIAN_POINT('',(1.4,-2.15,-31.3831195934094)) ;
#117573=CARTESIAN_POINT('Origin',(1.4,-3.65625,-30.48)) ;
#117574=CARTESIAN_POINT('',(1.4,-2.15,-32.03)) ;
#117575=CARTESIAN_POINT('',(1.4,-2.15,-32.03)) ;
#117576=CARTESIAN_POINT('',(1.4,1.9,-32.03)) ;
#117577=CARTESIAN_POINT('',(1.4,1.9,-32.03)) ;
#117578=CARTESIAN_POINT('',(1.4,1.9,-31.08)) ;
#117579=CARTESIAN_POINT('',(1.4,1.9,-31.08)) ;
#117580=CARTESIAN_POINT('',(1.4,2.1,-30.88)) ;
#117581=CARTESIAN_POINT('Origin',(1.4,2.1,-31.08)) ;
#117582=CARTESIAN_POINT('',(1.4,2.4,-30.88)) ;
#117583=CARTESIAN_POINT('',(1.4,2.4,-30.88)) ;
#117584=CARTESIAN_POINT('',(1.4,2.6,-31.08)) ;
#117585=CARTESIAN_POINT('Origin',(1.4,2.4,-31.08)) ;
#117586=CARTESIAN_POINT('',(1.4,2.6,-31.1885786437627)) ;
#117587=CARTESIAN_POINT('',(1.4,2.6,-31.1885786437627)) ;
#117588=CARTESIAN_POINT('',(1.4,3.15,-31.7385786437627)) ;
#117589=CARTESIAN_POINT('',(1.4,3.15,-31.7385786437627)) ;
#117590=CARTESIAN_POINT('',(1.4,3.15,-29.2214213562373)) ;
#117591=CARTESIAN_POINT('',(1.4,2.6,-29.7714213562373)) ;
#117592=CARTESIAN_POINT('',(1.4,2.6,-29.7714213562373)) ;
#117593=CARTESIAN_POINT('',(1.4,2.6,-29.88)) ;
#117594=CARTESIAN_POINT('Origin',(1.4,2.1,-26.07)) ;
#117595=CARTESIAN_POINT('',(1.5,2.,-26.07)) ;
#117596=CARTESIAN_POINT('',(7.9,2.,-26.07)) ;
#117597=CARTESIAN_POINT('',(1.4,2.,-26.07)) ;
#117598=CARTESIAN_POINT('',(1.5,2.1,-26.17)) ;
#117599=CARTESIAN_POINT('Origin',(1.5,2.1,-26.07)) ;
#117600=CARTESIAN_POINT('',(7.9,2.1,-26.17)) ;
#117601=CARTESIAN_POINT('',(1.4,2.1,-26.17)) ;
#117602=CARTESIAN_POINT('Origin',(7.9,2.1,-26.07)) ;
#117603=CARTESIAN_POINT('Origin',(1.4,2.4,-26.17)) ;
#117604=CARTESIAN_POINT('',(1.5,2.4,-26.17)) ;
#117605=CARTESIAN_POINT('',(1.5,2.4,-26.17)) ;
#117606=CARTESIAN_POINT('',(7.9,2.4,-26.17)) ;
#117607=CARTESIAN_POINT('',(1.4,2.4,-26.17)) ;
#117608=CARTESIAN_POINT('',(7.9,2.1,-26.17)) ;
#117609=CARTESIAN_POINT('Origin',(1.4,2.4,-26.07)) ;
#117610=CARTESIAN_POINT('',(1.5,2.5,-26.07)) ;
#117611=CARTESIAN_POINT('Origin',(1.5,2.4,-26.07)) ;
#117612=CARTESIAN_POINT('',(7.9,2.5,-26.07)) ;
#117613=CARTESIAN_POINT('',(1.4,2.5,-26.07)) ;
#117614=CARTESIAN_POINT('Origin',(7.9,2.4,-26.07)) ;
#117615=CARTESIAN_POINT('Origin',(1.4,2.5,-25.9614213562373)) ;
#117616=CARTESIAN_POINT('',(1.5,2.5,-25.9614213562373)) ;
#117617=CARTESIAN_POINT('',(1.5,2.5,-25.9614213562373)) ;
#117618=CARTESIAN_POINT('',(7.9,2.5,-25.9614213562373)) ;
#117619=CARTESIAN_POINT('',(1.4,2.5,-25.9614213562373)) ;
#117620=CARTESIAN_POINT('',(7.9,2.5,-26.07)) ;
#117621=CARTESIAN_POINT('Origin',(1.4,2.6,-25.9614213562373)) ;
#117622=CARTESIAN_POINT('',(1.5,2.52928932188135,-25.8907106781187)) ;
#117623=CARTESIAN_POINT('Origin',(1.5,2.6,-25.9614213562373)) ;
#117624=CARTESIAN_POINT('',(7.9,2.52928932188135,-25.8907106781187)) ;
#117625=CARTESIAN_POINT('',(1.4,2.52928932188135,-25.8907106781187)) ;
#117626=CARTESIAN_POINT('Origin',(7.9,2.6,-25.9614213562373)) ;
#117627=CARTESIAN_POINT('Origin',(1.4,3.07928932188135,-25.3407106781187)) ;
#117628=CARTESIAN_POINT('',(1.5,3.07928932188135,-25.3407106781187)) ;
#117629=CARTESIAN_POINT('',(7.9,3.07928932188135,-25.3407106781187)) ;
#117630=CARTESIAN_POINT('',(1.4,3.07928932188135,-25.3407106781187)) ;
#117631=CARTESIAN_POINT('',(7.9,2.52928932188135,-25.8907106781187)) ;
#117632=CARTESIAN_POINT('Origin',(1.4,3.15,-25.4114213562373)) ;
#117633=CARTESIAN_POINT('',(7.9,3.25,-25.4114213562373)) ;
#117634=CARTESIAN_POINT('',(1.4,3.25,-25.4114213562373)) ;
#117635=CARTESIAN_POINT('Origin',(7.9,3.15,-25.4114213562373)) ;
#117636=CARTESIAN_POINT('Origin',(1.4,3.25,-27.9285786437627)) ;
#117637=CARTESIAN_POINT('',(1.5,3.25,-27.9285786437627)) ;
#117638=CARTESIAN_POINT('',(7.9,3.25,-25.4114213562373)) ;
#117639=CARTESIAN_POINT('Origin',(1.4,2.52928932188134,-27.4492893218813)) ;
#117640=CARTESIAN_POINT('',(1.5,2.52928932188134,-27.4492893218813)) ;
#117641=CARTESIAN_POINT('',(1.5,2.52928932188135,-27.4492893218813)) ;
#117642=CARTESIAN_POINT('',(7.9,2.52928932188134,-27.4492893218813)) ;
#117643=CARTESIAN_POINT('',(1.4,2.52928932188134,-27.4492893218813)) ;
#117644=CARTESIAN_POINT('',(7.9,3.07928932188134,-27.9992893218813)) ;
#117645=CARTESIAN_POINT('Origin',(1.4,2.6,-27.3785786437627)) ;
#117646=CARTESIAN_POINT('',(1.5,2.5,-27.3785786437627)) ;
#117647=CARTESIAN_POINT('Origin',(1.5,2.6,-27.3785786437627)) ;
#117648=CARTESIAN_POINT('',(7.9,2.5,-27.3785786437627)) ;
#117649=CARTESIAN_POINT('',(1.4,2.5,-27.3785786437627)) ;
#117650=CARTESIAN_POINT('Origin',(7.9,2.6,-27.3785786437627)) ;
#117651=CARTESIAN_POINT('Origin',(1.4,2.5,-27.27)) ;
#117652=CARTESIAN_POINT('',(1.5,2.5,-27.27)) ;
#117653=CARTESIAN_POINT('',(1.5,2.5,-27.27)) ;
#117654=CARTESIAN_POINT('',(7.9,2.5,-27.27)) ;
#117655=CARTESIAN_POINT('',(1.4,2.5,-27.27)) ;
#117656=CARTESIAN_POINT('',(7.9,2.5,-27.3785786437627)) ;
#117657=CARTESIAN_POINT('Origin',(1.4,2.4,-27.27)) ;
#117658=CARTESIAN_POINT('',(1.5,2.4,-27.17)) ;
#117659=CARTESIAN_POINT('Origin',(1.5,2.4,-27.27)) ;
#117660=CARTESIAN_POINT('',(7.9,2.4,-27.17)) ;
#117661=CARTESIAN_POINT('',(1.4,2.4,-27.17)) ;
#117662=CARTESIAN_POINT('Origin',(7.9,2.4,-27.27)) ;
#117663=CARTESIAN_POINT('Origin',(1.4,2.1,-27.17)) ;
#117664=CARTESIAN_POINT('',(1.5,2.1,-27.17)) ;
#117665=CARTESIAN_POINT('',(1.5,2.1,-27.17)) ;
#117666=CARTESIAN_POINT('',(7.9,2.1,-27.17)) ;
#117667=CARTESIAN_POINT('',(1.4,2.1,-27.17)) ;
#117668=CARTESIAN_POINT('',(7.9,2.4,-27.17)) ;
#117669=CARTESIAN_POINT('Origin',(1.4,2.1,-27.27)) ;
#117670=CARTESIAN_POINT('',(1.5,2.,-27.27)) ;
#117671=CARTESIAN_POINT('Origin',(1.5,2.1,-27.27)) ;
#117672=CARTESIAN_POINT('',(7.9,2.,-27.27)) ;
#117673=CARTESIAN_POINT('',(1.4,2.,-27.27)) ;
#117674=CARTESIAN_POINT('Origin',(7.9,2.1,-27.27)) ;
#117675=CARTESIAN_POINT('Origin',(1.4,2.,-27.27)) ;
#117676=CARTESIAN_POINT('',(1.5,2.,-28.22)) ;
#117677=CARTESIAN_POINT('',(1.5,2.,-28.22)) ;
#117678=CARTESIAN_POINT('',(7.9,2.,-28.22)) ;
#117679=CARTESIAN_POINT('',(1.4,2.,-28.22)) ;
#117680=CARTESIAN_POINT('',(7.9,2.,-27.27)) ;
#117681=CARTESIAN_POINT('Origin',(1.4,1.9,-28.22)) ;
#117682=CARTESIAN_POINT('',(1.5,1.9,-28.32)) ;
#117683=CARTESIAN_POINT('Origin',(1.5,1.9,-28.22)) ;
#117684=CARTESIAN_POINT('',(7.9,1.9,-28.32)) ;
#117685=CARTESIAN_POINT('',(1.4,1.9,-28.32)) ;
#117686=CARTESIAN_POINT('Origin',(7.9,1.9,-28.22)) ;
#117687=CARTESIAN_POINT('Origin',(1.4,1.9,-28.32)) ;
#117688=CARTESIAN_POINT('',(1.5,-2.15,-28.32)) ;
#117689=CARTESIAN_POINT('',(1.5,-2.15,-28.32)) ;
#117690=CARTESIAN_POINT('',(7.9,-2.15,-28.32)) ;
#117691=CARTESIAN_POINT('',(1.4,-2.15,-28.32)) ;
#117692=CARTESIAN_POINT('',(7.9,1.9,-28.32)) ;
#117693=CARTESIAN_POINT('Origin',(1.4,-2.15,-28.22)) ;
#117694=CARTESIAN_POINT('',(1.5,-2.25,-28.22)) ;
#117695=CARTESIAN_POINT('Origin',(1.5,-2.15,-28.22)) ;
#117696=CARTESIAN_POINT('',(7.9,-2.25,-28.22)) ;
#117697=CARTESIAN_POINT('',(1.4,-2.25,-28.22)) ;
#117698=CARTESIAN_POINT('Origin',(7.9,-2.15,-28.22)) ;
#117699=CARTESIAN_POINT('Origin',(1.4,-2.25,-27.5731195934094)) ;
#117700=CARTESIAN_POINT('',(1.5,-2.25,-27.5731195934094)) ;
#117701=CARTESIAN_POINT('',(1.5,-2.25,-27.5731195934094)) ;
#117702=CARTESIAN_POINT('',(7.9,-2.25,-27.5731195934094)) ;
#117703=CARTESIAN_POINT('',(1.4,-2.25,-27.5731195934094)) ;
#117704=CARTESIAN_POINT('',(7.9,-2.25,-28.22)) ;
#117705=CARTESIAN_POINT('Origin',(1.4,-2.15,-27.5731195934094)) ;
#117706=CARTESIAN_POINT('',(1.5,-2.23576512455516,-27.5216964137135)) ;
#117707=CARTESIAN_POINT('Origin',(1.5,-2.15,-27.5731195934094)) ;
#117708=CARTESIAN_POINT('',(7.9,-2.23576512455516,-27.5216964137135)) ;
#117709=CARTESIAN_POINT('',(1.4,-2.23576512455516,-27.5216964137135)) ;
#117710=CARTESIAN_POINT('Origin',(7.9,-2.15,-27.5731195934094)) ;
#117711=CARTESIAN_POINT('Origin',(1.4,-3.65625,-26.67)) ;
#117712=CARTESIAN_POINT('',(1.5,-2.23576512455516,-25.8183035862865)) ;
#117713=CARTESIAN_POINT('Origin',(1.5,-3.65625,-26.67)) ;
#117714=CARTESIAN_POINT('',(7.9,-2.23576512455516,-25.8183035862865)) ;
#117715=CARTESIAN_POINT('',(1.4,-2.23576512455516,-25.8183035862865)) ;
#117716=CARTESIAN_POINT('Origin',(7.9,-3.65625,-26.67)) ;
#117717=CARTESIAN_POINT('Origin',(1.4,-2.15,-25.7668804065906)) ;
#117718=CARTESIAN_POINT('',(1.5,-2.25,-25.7668804065906)) ;
#117719=CARTESIAN_POINT('Origin',(1.5,-2.15,-25.7668804065906)) ;
#117720=CARTESIAN_POINT('',(7.9,-2.25,-25.7668804065906)) ;
#117721=CARTESIAN_POINT('',(1.4,-2.25,-25.7668804065906)) ;
#117722=CARTESIAN_POINT('Origin',(7.9,-2.15,-25.7668804065906)) ;
#117723=CARTESIAN_POINT('Origin',(1.4,-2.25,-25.12)) ;
#117724=CARTESIAN_POINT('',(1.5,-2.25,-25.12)) ;
#117725=CARTESIAN_POINT('',(1.5,-2.25,-25.12)) ;
#117726=CARTESIAN_POINT('',(7.9,-2.25,-25.12)) ;
#117727=CARTESIAN_POINT('',(1.4,-2.25,-25.12)) ;
#117728=CARTESIAN_POINT('',(7.9,-2.25,-25.7668804065906)) ;
#117729=CARTESIAN_POINT('Origin',(1.4,-2.15,-25.12)) ;
#117730=CARTESIAN_POINT('',(1.5,-2.15,-25.02)) ;
#117731=CARTESIAN_POINT('Origin',(1.5,-2.15,-25.12)) ;
#117732=CARTESIAN_POINT('',(7.9,-2.15,-25.02)) ;
#117733=CARTESIAN_POINT('',(1.4,-2.15,-25.02)) ;
#117734=CARTESIAN_POINT('Origin',(7.9,-2.15,-25.12)) ;
#117735=CARTESIAN_POINT('Origin',(1.4,1.9,-25.02)) ;
#117736=CARTESIAN_POINT('',(1.5,1.9,-25.02)) ;
#117737=CARTESIAN_POINT('',(1.5,1.9,-25.02)) ;
#117738=CARTESIAN_POINT('',(7.9,1.9,-25.02)) ;
#117739=CARTESIAN_POINT('',(1.4,1.9,-25.02)) ;
#117740=CARTESIAN_POINT('',(7.9,-2.15,-25.02)) ;
#117741=CARTESIAN_POINT('Origin',(1.4,1.9,-25.12)) ;
#117742=CARTESIAN_POINT('',(1.5,2.,-25.12)) ;
#117743=CARTESIAN_POINT('Origin',(1.5,1.9,-25.12)) ;
#117744=CARTESIAN_POINT('',(7.9,2.,-25.12)) ;
#117745=CARTESIAN_POINT('',(1.4,2.,-25.12)) ;
#117746=CARTESIAN_POINT('Origin',(7.9,1.9,-25.12)) ;
#117747=CARTESIAN_POINT('Origin',(1.4,2.,-25.12)) ;
#117748=CARTESIAN_POINT('',(1.5,2.,-26.07)) ;
#117749=CARTESIAN_POINT('',(7.9,2.,-25.12)) ;
#117750=CARTESIAN_POINT('Origin',(1.4,2.1,-26.07)) ;
#117751=CARTESIAN_POINT('',(1.4,2.6,-26.07)) ;
#117752=CARTESIAN_POINT('',(1.4,2.4,-26.27)) ;
#117753=CARTESIAN_POINT('Origin',(1.4,2.4,-26.07)) ;
#117754=CARTESIAN_POINT('',(1.4,2.1,-26.27)) ;
#117755=CARTESIAN_POINT('',(1.4,2.1,-26.27)) ;
#117756=CARTESIAN_POINT('',(1.4,1.9,-26.07)) ;
#117757=CARTESIAN_POINT('Origin',(1.4,2.1,-26.07)) ;
#117758=CARTESIAN_POINT('',(1.4,1.9,-25.12)) ;
#117759=CARTESIAN_POINT('',(1.4,1.9,-25.12)) ;
#117760=CARTESIAN_POINT('',(1.4,-2.15,-25.12)) ;
#117761=CARTESIAN_POINT('',(1.4,-2.15,-25.12)) ;
#117762=CARTESIAN_POINT('',(1.4,-2.15,-25.7668804065906)) ;
#117763=CARTESIAN_POINT('',(1.4,-2.15,-25.7668804065906)) ;
#117764=CARTESIAN_POINT('',(1.4,-2.15,-27.5731195934094)) ;
#117765=CARTESIAN_POINT('Origin',(1.4,-3.65625,-26.67)) ;
#117766=CARTESIAN_POINT('',(1.4,-2.15,-28.22)) ;
#117767=CARTESIAN_POINT('',(1.4,-2.15,-28.22)) ;
#117768=CARTESIAN_POINT('',(1.4,1.9,-28.22)) ;
#117769=CARTESIAN_POINT('',(1.4,1.9,-28.22)) ;
#117770=CARTESIAN_POINT('',(1.4,1.9,-27.27)) ;
#117771=CARTESIAN_POINT('',(1.4,1.9,-27.27)) ;
#117772=CARTESIAN_POINT('',(1.4,2.1,-27.07)) ;
#117773=CARTESIAN_POINT('Origin',(1.4,2.1,-27.27)) ;
#117774=CARTESIAN_POINT('',(1.4,2.4,-27.07)) ;
#117775=CARTESIAN_POINT('',(1.4,2.4,-27.07)) ;
#117776=CARTESIAN_POINT('',(1.4,2.6,-27.27)) ;
#117777=CARTESIAN_POINT('Origin',(1.4,2.4,-27.27)) ;
#117778=CARTESIAN_POINT('',(1.4,2.6,-27.3785786437627)) ;
#117779=CARTESIAN_POINT('',(1.4,2.6,-27.3785786437627)) ;
#117780=CARTESIAN_POINT('',(1.4,3.15,-27.9285786437627)) ;
#117781=CARTESIAN_POINT('',(1.4,3.15,-27.9285786437627)) ;
#117782=CARTESIAN_POINT('',(1.4,3.15,-25.4114213562373)) ;
#117783=CARTESIAN_POINT('',(1.4,2.6,-25.9614213562373)) ;
#117784=CARTESIAN_POINT('',(1.4,2.6,-25.9614213562373)) ;
#117785=CARTESIAN_POINT('',(1.4,2.6,-26.07)) ;
#117786=CARTESIAN_POINT('Origin',(1.4,2.1,-22.26)) ;
#117787=CARTESIAN_POINT('',(1.5,2.,-22.26)) ;
#117788=CARTESIAN_POINT('',(7.9,2.,-22.26)) ;
#117789=CARTESIAN_POINT('',(1.4,2.,-22.26)) ;
#117790=CARTESIAN_POINT('',(1.5,2.1,-22.36)) ;
#117791=CARTESIAN_POINT('Origin',(1.5,2.1,-22.26)) ;
#117792=CARTESIAN_POINT('',(7.9,2.1,-22.36)) ;
#117793=CARTESIAN_POINT('',(1.4,2.1,-22.36)) ;
#117794=CARTESIAN_POINT('Origin',(7.9,2.1,-22.26)) ;
#117795=CARTESIAN_POINT('Origin',(1.4,2.4,-22.36)) ;
#117796=CARTESIAN_POINT('',(1.5,2.4,-22.36)) ;
#117797=CARTESIAN_POINT('',(1.5,2.4,-22.36)) ;
#117798=CARTESIAN_POINT('',(7.9,2.4,-22.36)) ;
#117799=CARTESIAN_POINT('',(1.4,2.4,-22.36)) ;
#117800=CARTESIAN_POINT('',(7.9,2.1,-22.36)) ;
#117801=CARTESIAN_POINT('Origin',(1.4,2.4,-22.26)) ;
#117802=CARTESIAN_POINT('',(1.5,2.5,-22.26)) ;
#117803=CARTESIAN_POINT('Origin',(1.5,2.4,-22.26)) ;
#117804=CARTESIAN_POINT('',(7.9,2.5,-22.26)) ;
#117805=CARTESIAN_POINT('',(1.4,2.5,-22.26)) ;
#117806=CARTESIAN_POINT('Origin',(7.9,2.4,-22.26)) ;
#117807=CARTESIAN_POINT('Origin',(1.4,2.5,-22.1514213562373)) ;
#117808=CARTESIAN_POINT('',(1.5,2.5,-22.1514213562373)) ;
#117809=CARTESIAN_POINT('',(1.5,2.5,-22.1514213562373)) ;
#117810=CARTESIAN_POINT('',(7.9,2.5,-22.1514213562373)) ;
#117811=CARTESIAN_POINT('',(1.4,2.5,-22.1514213562373)) ;
#117812=CARTESIAN_POINT('',(7.9,2.5,-22.26)) ;
#117813=CARTESIAN_POINT('Origin',(1.4,2.6,-22.1514213562373)) ;
#117814=CARTESIAN_POINT('',(1.5,2.52928932188135,-22.0807106781187)) ;
#117815=CARTESIAN_POINT('Origin',(1.5,2.6,-22.1514213562373)) ;
#117816=CARTESIAN_POINT('',(7.9,2.52928932188135,-22.0807106781187)) ;
#117817=CARTESIAN_POINT('',(1.4,2.52928932188135,-22.0807106781187)) ;
#117818=CARTESIAN_POINT('Origin',(7.9,2.6,-22.1514213562373)) ;
#117819=CARTESIAN_POINT('Origin',(1.4,3.07928932188135,-21.5307106781187)) ;
#117820=CARTESIAN_POINT('',(1.5,3.07928932188135,-21.5307106781187)) ;
#117821=CARTESIAN_POINT('',(7.9,3.07928932188135,-21.5307106781187)) ;
#117822=CARTESIAN_POINT('',(1.4,3.07928932188135,-21.5307106781187)) ;
#117823=CARTESIAN_POINT('',(7.9,2.52928932188135,-22.0807106781187)) ;
#117824=CARTESIAN_POINT('Origin',(1.4,3.15,-21.6014213562373)) ;
#117825=CARTESIAN_POINT('',(7.9,3.25,-21.6014213562373)) ;
#117826=CARTESIAN_POINT('',(1.4,3.25,-21.6014213562373)) ;
#117827=CARTESIAN_POINT('Origin',(7.9,3.15,-21.6014213562373)) ;
#117828=CARTESIAN_POINT('Origin',(1.4,3.25,-24.1185786437627)) ;
#117829=CARTESIAN_POINT('',(1.5,3.25,-24.1185786437627)) ;
#117830=CARTESIAN_POINT('',(7.9,3.25,-21.6014213562373)) ;
#117831=CARTESIAN_POINT('Origin',(1.4,2.52928932188134,-23.6392893218813)) ;
#117832=CARTESIAN_POINT('',(1.5,2.52928932188134,-23.6392893218813)) ;
#117833=CARTESIAN_POINT('',(1.5,2.52928932188135,-23.6392893218813)) ;
#117834=CARTESIAN_POINT('',(7.9,2.52928932188134,-23.6392893218813)) ;
#117835=CARTESIAN_POINT('',(1.4,2.52928932188134,-23.6392893218813)) ;
#117836=CARTESIAN_POINT('',(7.9,3.07928932188134,-24.1892893218813)) ;
#117837=CARTESIAN_POINT('Origin',(1.4,2.6,-23.5685786437627)) ;
#117838=CARTESIAN_POINT('',(1.5,2.5,-23.5685786437627)) ;
#117839=CARTESIAN_POINT('Origin',(1.5,2.6,-23.5685786437627)) ;
#117840=CARTESIAN_POINT('',(7.9,2.5,-23.5685786437627)) ;
#117841=CARTESIAN_POINT('',(1.4,2.5,-23.5685786437627)) ;
#117842=CARTESIAN_POINT('Origin',(7.9,2.6,-23.5685786437627)) ;
#117843=CARTESIAN_POINT('Origin',(1.4,2.5,-23.46)) ;
#117844=CARTESIAN_POINT('',(1.5,2.5,-23.46)) ;
#117845=CARTESIAN_POINT('',(1.5,2.5,-23.46)) ;
#117846=CARTESIAN_POINT('',(7.9,2.5,-23.46)) ;
#117847=CARTESIAN_POINT('',(1.4,2.5,-23.46)) ;
#117848=CARTESIAN_POINT('',(7.9,2.5,-23.5685786437627)) ;
#117849=CARTESIAN_POINT('Origin',(1.4,2.4,-23.46)) ;
#117850=CARTESIAN_POINT('',(1.5,2.4,-23.36)) ;
#117851=CARTESIAN_POINT('Origin',(1.5,2.4,-23.46)) ;
#117852=CARTESIAN_POINT('',(7.9,2.4,-23.36)) ;
#117853=CARTESIAN_POINT('',(1.4,2.4,-23.36)) ;
#117854=CARTESIAN_POINT('Origin',(7.9,2.4,-23.46)) ;
#117855=CARTESIAN_POINT('Origin',(1.4,2.1,-23.36)) ;
#117856=CARTESIAN_POINT('',(1.5,2.1,-23.36)) ;
#117857=CARTESIAN_POINT('',(1.5,2.1,-23.36)) ;
#117858=CARTESIAN_POINT('',(7.9,2.1,-23.36)) ;
#117859=CARTESIAN_POINT('',(1.4,2.1,-23.36)) ;
#117860=CARTESIAN_POINT('',(7.9,2.4,-23.36)) ;
#117861=CARTESIAN_POINT('Origin',(1.4,2.1,-23.46)) ;
#117862=CARTESIAN_POINT('',(1.5,2.,-23.46)) ;
#117863=CARTESIAN_POINT('Origin',(1.5,2.1,-23.46)) ;
#117864=CARTESIAN_POINT('',(7.9,2.,-23.46)) ;
#117865=CARTESIAN_POINT('',(1.4,2.,-23.46)) ;
#117866=CARTESIAN_POINT('Origin',(7.9,2.1,-23.46)) ;
#117867=CARTESIAN_POINT('Origin',(1.4,2.,-23.46)) ;
#117868=CARTESIAN_POINT('',(1.5,2.,-24.41)) ;
#117869=CARTESIAN_POINT('',(1.5,2.,-24.41)) ;
#117870=CARTESIAN_POINT('',(7.9,2.,-24.41)) ;
#117871=CARTESIAN_POINT('',(1.4,2.,-24.41)) ;
#117872=CARTESIAN_POINT('',(7.9,2.,-23.46)) ;
#117873=CARTESIAN_POINT('Origin',(1.4,1.9,-24.41)) ;
#117874=CARTESIAN_POINT('',(1.5,1.9,-24.51)) ;
#117875=CARTESIAN_POINT('Origin',(1.5,1.9,-24.41)) ;
#117876=CARTESIAN_POINT('',(7.9,1.9,-24.51)) ;
#117877=CARTESIAN_POINT('',(1.4,1.9,-24.51)) ;
#117878=CARTESIAN_POINT('Origin',(7.9,1.9,-24.41)) ;
#117879=CARTESIAN_POINT('Origin',(1.4,1.9,-24.51)) ;
#117880=CARTESIAN_POINT('',(1.5,-2.15,-24.51)) ;
#117881=CARTESIAN_POINT('',(1.5,-2.15,-24.51)) ;
#117882=CARTESIAN_POINT('',(7.9,-2.15,-24.51)) ;
#117883=CARTESIAN_POINT('',(1.4,-2.15,-24.51)) ;
#117884=CARTESIAN_POINT('',(7.9,1.9,-24.51)) ;
#117885=CARTESIAN_POINT('Origin',(1.4,-2.15,-24.41)) ;
#117886=CARTESIAN_POINT('',(1.5,-2.25,-24.41)) ;
#117887=CARTESIAN_POINT('Origin',(1.5,-2.15,-24.41)) ;
#117888=CARTESIAN_POINT('',(7.9,-2.25,-24.41)) ;
#117889=CARTESIAN_POINT('',(1.4,-2.25,-24.41)) ;
#117890=CARTESIAN_POINT('Origin',(7.9,-2.15,-24.41)) ;
#117891=CARTESIAN_POINT('Origin',(1.4,-2.25,-23.7631195934094)) ;
#117892=CARTESIAN_POINT('',(1.5,-2.25,-23.7631195934094)) ;
#117893=CARTESIAN_POINT('',(1.5,-2.25,-23.7631195934094)) ;
#117894=CARTESIAN_POINT('',(7.9,-2.25,-23.7631195934094)) ;
#117895=CARTESIAN_POINT('',(1.4,-2.25,-23.7631195934094)) ;
#117896=CARTESIAN_POINT('',(7.9,-2.25,-24.41)) ;
#117897=CARTESIAN_POINT('Origin',(1.4,-2.15,-23.7631195934094)) ;
#117898=CARTESIAN_POINT('',(1.5,-2.23576512455516,-23.7116964137135)) ;
#117899=CARTESIAN_POINT('Origin',(1.5,-2.15,-23.7631195934094)) ;
#117900=CARTESIAN_POINT('',(7.9,-2.23576512455516,-23.7116964137135)) ;
#117901=CARTESIAN_POINT('',(1.4,-2.23576512455516,-23.7116964137135)) ;
#117902=CARTESIAN_POINT('Origin',(7.9,-2.15,-23.7631195934094)) ;
#117903=CARTESIAN_POINT('Origin',(1.4,-3.65625,-22.86)) ;
#117904=CARTESIAN_POINT('',(1.5,-2.23576512455516,-22.0083035862865)) ;
#117905=CARTESIAN_POINT('Origin',(1.5,-3.65625,-22.86)) ;
#117906=CARTESIAN_POINT('',(7.9,-2.23576512455516,-22.0083035862865)) ;
#117907=CARTESIAN_POINT('',(1.4,-2.23576512455516,-22.0083035862865)) ;
#117908=CARTESIAN_POINT('Origin',(7.9,-3.65625,-22.86)) ;
#117909=CARTESIAN_POINT('Origin',(1.4,-2.15,-21.9568804065906)) ;
#117910=CARTESIAN_POINT('',(1.5,-2.25,-21.9568804065906)) ;
#117911=CARTESIAN_POINT('Origin',(1.5,-2.15,-21.9568804065906)) ;
#117912=CARTESIAN_POINT('',(7.9,-2.25,-21.9568804065906)) ;
#117913=CARTESIAN_POINT('',(1.4,-2.25,-21.9568804065906)) ;
#117914=CARTESIAN_POINT('Origin',(7.9,-2.15,-21.9568804065906)) ;
#117915=CARTESIAN_POINT('Origin',(1.4,-2.25,-21.31)) ;
#117916=CARTESIAN_POINT('',(1.5,-2.25,-21.31)) ;
#117917=CARTESIAN_POINT('',(1.5,-2.25,-21.31)) ;
#117918=CARTESIAN_POINT('',(7.9,-2.25,-21.31)) ;
#117919=CARTESIAN_POINT('',(1.4,-2.25,-21.31)) ;
#117920=CARTESIAN_POINT('',(7.9,-2.25,-21.9568804065906)) ;
#117921=CARTESIAN_POINT('Origin',(1.4,-2.15,-21.31)) ;
#117922=CARTESIAN_POINT('',(1.5,-2.15,-21.21)) ;
#117923=CARTESIAN_POINT('Origin',(1.5,-2.15,-21.31)) ;
#117924=CARTESIAN_POINT('',(7.9,-2.15,-21.21)) ;
#117925=CARTESIAN_POINT('',(1.4,-2.15,-21.21)) ;
#117926=CARTESIAN_POINT('Origin',(7.9,-2.15,-21.31)) ;
#117927=CARTESIAN_POINT('Origin',(1.4,1.9,-21.21)) ;
#117928=CARTESIAN_POINT('',(1.5,1.9,-21.21)) ;
#117929=CARTESIAN_POINT('',(1.5,1.9,-21.21)) ;
#117930=CARTESIAN_POINT('',(7.9,1.9,-21.21)) ;
#117931=CARTESIAN_POINT('',(1.4,1.9,-21.21)) ;
#117932=CARTESIAN_POINT('',(7.9,-2.15,-21.21)) ;
#117933=CARTESIAN_POINT('Origin',(1.4,1.9,-21.31)) ;
#117934=CARTESIAN_POINT('',(1.5,2.,-21.31)) ;
#117935=CARTESIAN_POINT('Origin',(1.5,1.9,-21.31)) ;
#117936=CARTESIAN_POINT('',(7.9,2.,-21.31)) ;
#117937=CARTESIAN_POINT('',(1.4,2.,-21.31)) ;
#117938=CARTESIAN_POINT('Origin',(7.9,1.9,-21.31)) ;
#117939=CARTESIAN_POINT('Origin',(1.4,2.,-21.31)) ;
#117940=CARTESIAN_POINT('',(1.5,2.,-22.26)) ;
#117941=CARTESIAN_POINT('',(7.9,2.,-21.31)) ;
#117942=CARTESIAN_POINT('Origin',(1.4,2.1,-22.26)) ;
#117943=CARTESIAN_POINT('',(1.4,2.6,-22.26)) ;
#117944=CARTESIAN_POINT('',(1.4,2.4,-22.46)) ;
#117945=CARTESIAN_POINT('Origin',(1.4,2.4,-22.26)) ;
#117946=CARTESIAN_POINT('',(1.4,2.1,-22.46)) ;
#117947=CARTESIAN_POINT('',(1.4,2.1,-22.46)) ;
#117948=CARTESIAN_POINT('',(1.4,1.9,-22.26)) ;
#117949=CARTESIAN_POINT('Origin',(1.4,2.1,-22.26)) ;
#117950=CARTESIAN_POINT('',(1.4,1.9,-21.31)) ;
#117951=CARTESIAN_POINT('',(1.4,1.9,-21.31)) ;
#117952=CARTESIAN_POINT('',(1.4,-2.15,-21.31)) ;
#117953=CARTESIAN_POINT('',(1.4,-2.15,-21.31)) ;
#117954=CARTESIAN_POINT('',(1.4,-2.15,-21.9568804065906)) ;
#117955=CARTESIAN_POINT('',(1.4,-2.15,-21.9568804065906)) ;
#117956=CARTESIAN_POINT('',(1.4,-2.15,-23.7631195934094)) ;
#117957=CARTESIAN_POINT('Origin',(1.4,-3.65625,-22.86)) ;
#117958=CARTESIAN_POINT('',(1.4,-2.15,-24.41)) ;
#117959=CARTESIAN_POINT('',(1.4,-2.15,-24.41)) ;
#117960=CARTESIAN_POINT('',(1.4,1.9,-24.41)) ;
#117961=CARTESIAN_POINT('',(1.4,1.9,-24.41)) ;
#117962=CARTESIAN_POINT('',(1.4,1.9,-23.46)) ;
#117963=CARTESIAN_POINT('',(1.4,1.9,-23.46)) ;
#117964=CARTESIAN_POINT('',(1.4,2.1,-23.26)) ;
#117965=CARTESIAN_POINT('Origin',(1.4,2.1,-23.46)) ;
#117966=CARTESIAN_POINT('',(1.4,2.4,-23.26)) ;
#117967=CARTESIAN_POINT('',(1.4,2.4,-23.26)) ;
#117968=CARTESIAN_POINT('',(1.4,2.6,-23.46)) ;
#117969=CARTESIAN_POINT('Origin',(1.4,2.4,-23.46)) ;
#117970=CARTESIAN_POINT('',(1.4,2.6,-23.5685786437627)) ;
#117971=CARTESIAN_POINT('',(1.4,2.6,-23.5685786437627)) ;
#117972=CARTESIAN_POINT('',(1.4,3.15,-24.1185786437627)) ;
#117973=CARTESIAN_POINT('',(1.4,3.15,-24.1185786437627)) ;
#117974=CARTESIAN_POINT('',(1.4,3.15,-21.6014213562373)) ;
#117975=CARTESIAN_POINT('',(1.4,2.6,-22.1514213562373)) ;
#117976=CARTESIAN_POINT('',(1.4,2.6,-22.1514213562373)) ;
#117977=CARTESIAN_POINT('',(1.4,2.6,-22.26)) ;
#117978=CARTESIAN_POINT('Origin',(1.4,2.1,-18.45)) ;
#117979=CARTESIAN_POINT('',(1.5,2.,-18.45)) ;
#117980=CARTESIAN_POINT('',(7.9,2.,-18.45)) ;
#117981=CARTESIAN_POINT('',(1.4,2.,-18.45)) ;
#117982=CARTESIAN_POINT('',(1.5,2.1,-18.55)) ;
#117983=CARTESIAN_POINT('Origin',(1.5,2.1,-18.45)) ;
#117984=CARTESIAN_POINT('',(7.9,2.1,-18.55)) ;
#117985=CARTESIAN_POINT('',(1.4,2.1,-18.55)) ;
#117986=CARTESIAN_POINT('Origin',(7.9,2.1,-18.45)) ;
#117987=CARTESIAN_POINT('Origin',(1.4,2.4,-18.55)) ;
#117988=CARTESIAN_POINT('',(1.5,2.4,-18.55)) ;
#117989=CARTESIAN_POINT('',(1.5,2.4,-18.55)) ;
#117990=CARTESIAN_POINT('',(7.9,2.4,-18.55)) ;
#117991=CARTESIAN_POINT('',(1.4,2.4,-18.55)) ;
#117992=CARTESIAN_POINT('',(7.9,2.1,-18.55)) ;
#117993=CARTESIAN_POINT('Origin',(1.4,2.4,-18.45)) ;
#117994=CARTESIAN_POINT('',(1.5,2.5,-18.45)) ;
#117995=CARTESIAN_POINT('Origin',(1.5,2.4,-18.45)) ;
#117996=CARTESIAN_POINT('',(7.9,2.5,-18.45)) ;
#117997=CARTESIAN_POINT('',(1.4,2.5,-18.45)) ;
#117998=CARTESIAN_POINT('Origin',(7.9,2.4,-18.45)) ;
#117999=CARTESIAN_POINT('Origin',(1.4,2.5,-18.3414213562373)) ;
#118000=CARTESIAN_POINT('',(1.5,2.5,-18.3414213562373)) ;
#118001=CARTESIAN_POINT('',(1.5,2.5,-18.3414213562373)) ;
#118002=CARTESIAN_POINT('',(7.9,2.5,-18.3414213562373)) ;
#118003=CARTESIAN_POINT('',(1.4,2.5,-18.3414213562373)) ;
#118004=CARTESIAN_POINT('',(7.9,2.5,-18.45)) ;
#118005=CARTESIAN_POINT('Origin',(1.4,2.6,-18.3414213562373)) ;
#118006=CARTESIAN_POINT('',(1.5,2.52928932188135,-18.2707106781187)) ;
#118007=CARTESIAN_POINT('Origin',(1.5,2.6,-18.3414213562373)) ;
#118008=CARTESIAN_POINT('',(7.9,2.52928932188135,-18.2707106781187)) ;
#118009=CARTESIAN_POINT('',(1.4,2.52928932188135,-18.2707106781187)) ;
#118010=CARTESIAN_POINT('Origin',(7.9,2.6,-18.3414213562373)) ;
#118011=CARTESIAN_POINT('Origin',(1.4,3.07928932188135,-17.7207106781187)) ;
#118012=CARTESIAN_POINT('',(1.5,3.07928932188135,-17.7207106781187)) ;
#118013=CARTESIAN_POINT('',(7.9,3.07928932188135,-17.7207106781187)) ;
#118014=CARTESIAN_POINT('',(1.4,3.07928932188135,-17.7207106781187)) ;
#118015=CARTESIAN_POINT('',(7.9,2.52928932188135,-18.2707106781187)) ;
#118016=CARTESIAN_POINT('Origin',(1.4,3.15,-17.7914213562373)) ;
#118017=CARTESIAN_POINT('',(7.9,3.25,-17.7914213562373)) ;
#118018=CARTESIAN_POINT('',(1.4,3.25,-17.7914213562373)) ;
#118019=CARTESIAN_POINT('Origin',(7.9,3.15,-17.7914213562373)) ;
#118020=CARTESIAN_POINT('Origin',(1.4,3.25,-20.3085786437627)) ;
#118021=CARTESIAN_POINT('',(1.5,3.25,-20.3085786437627)) ;
#118022=CARTESIAN_POINT('',(7.9,3.25,-17.7914213562373)) ;
#118023=CARTESIAN_POINT('Origin',(1.4,2.52928932188134,-19.8292893218813)) ;
#118024=CARTESIAN_POINT('',(1.5,2.52928932188134,-19.8292893218813)) ;
#118025=CARTESIAN_POINT('',(1.5,2.52928932188135,-19.8292893218813)) ;
#118026=CARTESIAN_POINT('',(7.9,2.52928932188134,-19.8292893218813)) ;
#118027=CARTESIAN_POINT('',(1.4,2.52928932188134,-19.8292893218813)) ;
#118028=CARTESIAN_POINT('',(7.9,3.07928932188134,-20.3792893218813)) ;
#118029=CARTESIAN_POINT('Origin',(1.4,2.6,-19.7585786437627)) ;
#118030=CARTESIAN_POINT('',(1.5,2.5,-19.7585786437627)) ;
#118031=CARTESIAN_POINT('Origin',(1.5,2.6,-19.7585786437627)) ;
#118032=CARTESIAN_POINT('',(7.9,2.5,-19.7585786437627)) ;
#118033=CARTESIAN_POINT('',(1.4,2.5,-19.7585786437627)) ;
#118034=CARTESIAN_POINT('Origin',(7.9,2.6,-19.7585786437627)) ;
#118035=CARTESIAN_POINT('Origin',(1.4,2.5,-19.65)) ;
#118036=CARTESIAN_POINT('',(1.5,2.5,-19.65)) ;
#118037=CARTESIAN_POINT('',(1.5,2.5,-19.65)) ;
#118038=CARTESIAN_POINT('',(7.9,2.5,-19.65)) ;
#118039=CARTESIAN_POINT('',(1.4,2.5,-19.65)) ;
#118040=CARTESIAN_POINT('',(7.9,2.5,-19.7585786437627)) ;
#118041=CARTESIAN_POINT('Origin',(1.4,2.4,-19.65)) ;
#118042=CARTESIAN_POINT('',(1.5,2.4,-19.55)) ;
#118043=CARTESIAN_POINT('Origin',(1.5,2.4,-19.65)) ;
#118044=CARTESIAN_POINT('',(7.9,2.4,-19.55)) ;
#118045=CARTESIAN_POINT('',(1.4,2.4,-19.55)) ;
#118046=CARTESIAN_POINT('Origin',(7.9,2.4,-19.65)) ;
#118047=CARTESIAN_POINT('Origin',(1.4,2.1,-19.55)) ;
#118048=CARTESIAN_POINT('',(1.5,2.1,-19.55)) ;
#118049=CARTESIAN_POINT('',(1.5,2.1,-19.55)) ;
#118050=CARTESIAN_POINT('',(7.9,2.1,-19.55)) ;
#118051=CARTESIAN_POINT('',(1.4,2.1,-19.55)) ;
#118052=CARTESIAN_POINT('',(7.9,2.4,-19.55)) ;
#118053=CARTESIAN_POINT('Origin',(1.4,2.1,-19.65)) ;
#118054=CARTESIAN_POINT('',(1.5,2.,-19.65)) ;
#118055=CARTESIAN_POINT('Origin',(1.5,2.1,-19.65)) ;
#118056=CARTESIAN_POINT('',(7.9,2.,-19.65)) ;
#118057=CARTESIAN_POINT('',(1.4,2.,-19.65)) ;
#118058=CARTESIAN_POINT('Origin',(7.9,2.1,-19.65)) ;
#118059=CARTESIAN_POINT('Origin',(1.4,2.,-19.65)) ;
#118060=CARTESIAN_POINT('',(1.5,2.,-20.6)) ;
#118061=CARTESIAN_POINT('',(1.5,2.,-20.6)) ;
#118062=CARTESIAN_POINT('',(7.9,2.,-20.6)) ;
#118063=CARTESIAN_POINT('',(1.4,2.,-20.6)) ;
#118064=CARTESIAN_POINT('',(7.9,2.,-19.65)) ;
#118065=CARTESIAN_POINT('Origin',(1.4,1.9,-20.6)) ;
#118066=CARTESIAN_POINT('',(1.5,1.9,-20.7)) ;
#118067=CARTESIAN_POINT('Origin',(1.5,1.9,-20.6)) ;
#118068=CARTESIAN_POINT('',(7.9,1.9,-20.7)) ;
#118069=CARTESIAN_POINT('',(1.4,1.9,-20.7)) ;
#118070=CARTESIAN_POINT('Origin',(7.9,1.9,-20.6)) ;
#118071=CARTESIAN_POINT('Origin',(1.4,1.9,-20.7)) ;
#118072=CARTESIAN_POINT('',(1.5,-2.15,-20.7)) ;
#118073=CARTESIAN_POINT('',(1.5,-2.15,-20.7)) ;
#118074=CARTESIAN_POINT('',(7.9,-2.15,-20.7)) ;
#118075=CARTESIAN_POINT('',(1.4,-2.15,-20.7)) ;
#118076=CARTESIAN_POINT('',(7.9,1.9,-20.7)) ;
#118077=CARTESIAN_POINT('Origin',(1.4,-2.15,-20.6)) ;
#118078=CARTESIAN_POINT('',(1.5,-2.25,-20.6)) ;
#118079=CARTESIAN_POINT('Origin',(1.5,-2.15,-20.6)) ;
#118080=CARTESIAN_POINT('',(7.9,-2.25,-20.6)) ;
#118081=CARTESIAN_POINT('',(1.4,-2.25,-20.6)) ;
#118082=CARTESIAN_POINT('Origin',(7.9,-2.15,-20.6)) ;
#118083=CARTESIAN_POINT('Origin',(1.4,-2.25,-19.9531195934094)) ;
#118084=CARTESIAN_POINT('',(1.5,-2.25,-19.9531195934094)) ;
#118085=CARTESIAN_POINT('',(1.5,-2.25,-19.9531195934094)) ;
#118086=CARTESIAN_POINT('',(7.9,-2.25,-19.9531195934094)) ;
#118087=CARTESIAN_POINT('',(1.4,-2.25,-19.9531195934094)) ;
#118088=CARTESIAN_POINT('',(7.9,-2.25,-20.6)) ;
#118089=CARTESIAN_POINT('Origin',(1.4,-2.15,-19.9531195934094)) ;
#118090=CARTESIAN_POINT('',(1.5,-2.23576512455516,-19.9016964137135)) ;
#118091=CARTESIAN_POINT('Origin',(1.5,-2.15,-19.9531195934094)) ;
#118092=CARTESIAN_POINT('',(7.9,-2.23576512455516,-19.9016964137135)) ;
#118093=CARTESIAN_POINT('',(1.4,-2.23576512455516,-19.9016964137135)) ;
#118094=CARTESIAN_POINT('Origin',(7.9,-2.15,-19.9531195934094)) ;
#118095=CARTESIAN_POINT('Origin',(1.4,-3.65625,-19.05)) ;
#118096=CARTESIAN_POINT('',(1.5,-2.23576512455516,-18.1983035862865)) ;
#118097=CARTESIAN_POINT('Origin',(1.5,-3.65625,-19.05)) ;
#118098=CARTESIAN_POINT('',(7.9,-2.23576512455516,-18.1983035862865)) ;
#118099=CARTESIAN_POINT('',(1.4,-2.23576512455516,-18.1983035862865)) ;
#118100=CARTESIAN_POINT('Origin',(7.9,-3.65625,-19.05)) ;
#118101=CARTESIAN_POINT('Origin',(1.4,-2.15,-18.1468804065906)) ;
#118102=CARTESIAN_POINT('',(1.5,-2.25,-18.1468804065906)) ;
#118103=CARTESIAN_POINT('Origin',(1.5,-2.15,-18.1468804065906)) ;
#118104=CARTESIAN_POINT('',(7.9,-2.25,-18.1468804065906)) ;
#118105=CARTESIAN_POINT('',(1.4,-2.25,-18.1468804065906)) ;
#118106=CARTESIAN_POINT('Origin',(7.9,-2.15,-18.1468804065906)) ;
#118107=CARTESIAN_POINT('Origin',(1.4,-2.25,-17.5)) ;
#118108=CARTESIAN_POINT('',(1.5,-2.25,-17.5)) ;
#118109=CARTESIAN_POINT('',(1.5,-2.25,-17.5)) ;
#118110=CARTESIAN_POINT('',(7.9,-2.25,-17.5)) ;
#118111=CARTESIAN_POINT('',(1.4,-2.25,-17.5)) ;
#118112=CARTESIAN_POINT('',(7.9,-2.25,-18.1468804065906)) ;
#118113=CARTESIAN_POINT('Origin',(1.4,-2.15,-17.5)) ;
#118114=CARTESIAN_POINT('',(1.5,-2.15,-17.4)) ;
#118115=CARTESIAN_POINT('Origin',(1.5,-2.15,-17.5)) ;
#118116=CARTESIAN_POINT('',(7.9,-2.15,-17.4)) ;
#118117=CARTESIAN_POINT('',(1.4,-2.15,-17.4)) ;
#118118=CARTESIAN_POINT('Origin',(7.9,-2.15,-17.5)) ;
#118119=CARTESIAN_POINT('Origin',(1.4,1.9,-17.4)) ;
#118120=CARTESIAN_POINT('',(1.5,1.9,-17.4)) ;
#118121=CARTESIAN_POINT('',(1.5,1.9,-17.4)) ;
#118122=CARTESIAN_POINT('',(7.9,1.9,-17.4)) ;
#118123=CARTESIAN_POINT('',(1.4,1.9,-17.4)) ;
#118124=CARTESIAN_POINT('',(7.9,-2.15,-17.4)) ;
#118125=CARTESIAN_POINT('Origin',(1.4,1.9,-17.5)) ;
#118126=CARTESIAN_POINT('',(1.5,2.,-17.5)) ;
#118127=CARTESIAN_POINT('Origin',(1.5,1.9,-17.5)) ;
#118128=CARTESIAN_POINT('',(7.9,2.,-17.5)) ;
#118129=CARTESIAN_POINT('',(1.4,2.,-17.5)) ;
#118130=CARTESIAN_POINT('Origin',(7.9,1.9,-17.5)) ;
#118131=CARTESIAN_POINT('Origin',(1.4,2.,-17.5)) ;
#118132=CARTESIAN_POINT('',(1.5,2.,-18.45)) ;
#118133=CARTESIAN_POINT('',(7.9,2.,-17.5)) ;
#118134=CARTESIAN_POINT('Origin',(1.4,2.1,-18.45)) ;
#118135=CARTESIAN_POINT('',(1.4,2.6,-18.45)) ;
#118136=CARTESIAN_POINT('',(1.4,2.4,-18.65)) ;
#118137=CARTESIAN_POINT('Origin',(1.4,2.4,-18.45)) ;
#118138=CARTESIAN_POINT('',(1.4,2.1,-18.65)) ;
#118139=CARTESIAN_POINT('',(1.4,2.1,-18.65)) ;
#118140=CARTESIAN_POINT('',(1.4,1.9,-18.45)) ;
#118141=CARTESIAN_POINT('Origin',(1.4,2.1,-18.45)) ;
#118142=CARTESIAN_POINT('',(1.4,1.9,-17.5)) ;
#118143=CARTESIAN_POINT('',(1.4,1.9,-17.5)) ;
#118144=CARTESIAN_POINT('',(1.4,-2.15,-17.5)) ;
#118145=CARTESIAN_POINT('',(1.4,-2.15,-17.5)) ;
#118146=CARTESIAN_POINT('',(1.4,-2.15,-18.1468804065906)) ;
#118147=CARTESIAN_POINT('',(1.4,-2.15,-18.1468804065906)) ;
#118148=CARTESIAN_POINT('',(1.4,-2.15,-19.9531195934094)) ;
#118149=CARTESIAN_POINT('Origin',(1.4,-3.65625,-19.05)) ;
#118150=CARTESIAN_POINT('',(1.4,-2.15,-20.6)) ;
#118151=CARTESIAN_POINT('',(1.4,-2.15,-20.6)) ;
#118152=CARTESIAN_POINT('',(1.4,1.9,-20.6)) ;
#118153=CARTESIAN_POINT('',(1.4,1.9,-20.6)) ;
#118154=CARTESIAN_POINT('',(1.4,1.9,-19.65)) ;
#118155=CARTESIAN_POINT('',(1.4,1.9,-19.65)) ;
#118156=CARTESIAN_POINT('',(1.4,2.1,-19.45)) ;
#118157=CARTESIAN_POINT('Origin',(1.4,2.1,-19.65)) ;
#118158=CARTESIAN_POINT('',(1.4,2.4,-19.45)) ;
#118159=CARTESIAN_POINT('',(1.4,2.4,-19.45)) ;
#118160=CARTESIAN_POINT('',(1.4,2.6,-19.65)) ;
#118161=CARTESIAN_POINT('Origin',(1.4,2.4,-19.65)) ;
#118162=CARTESIAN_POINT('',(1.4,2.6,-19.7585786437627)) ;
#118163=CARTESIAN_POINT('',(1.4,2.6,-19.7585786437627)) ;
#118164=CARTESIAN_POINT('',(1.4,3.15,-20.3085786437627)) ;
#118165=CARTESIAN_POINT('',(1.4,3.15,-20.3085786437627)) ;
#118166=CARTESIAN_POINT('',(1.4,3.15,-17.7914213562373)) ;
#118167=CARTESIAN_POINT('',(1.4,2.6,-18.3414213562373)) ;
#118168=CARTESIAN_POINT('',(1.4,2.6,-18.3414213562373)) ;
#118169=CARTESIAN_POINT('',(1.4,2.6,-18.45)) ;
#118170=CARTESIAN_POINT('Origin',(1.4,2.1,-14.64)) ;
#118171=CARTESIAN_POINT('',(1.5,2.,-14.64)) ;
#118172=CARTESIAN_POINT('',(7.9,2.,-14.64)) ;
#118173=CARTESIAN_POINT('',(1.4,2.,-14.64)) ;
#118174=CARTESIAN_POINT('',(1.5,2.1,-14.74)) ;
#118175=CARTESIAN_POINT('Origin',(1.5,2.1,-14.64)) ;
#118176=CARTESIAN_POINT('',(7.9,2.1,-14.74)) ;
#118177=CARTESIAN_POINT('',(1.4,2.1,-14.74)) ;
#118178=CARTESIAN_POINT('Origin',(7.9,2.1,-14.64)) ;
#118179=CARTESIAN_POINT('Origin',(1.4,2.4,-14.74)) ;
#118180=CARTESIAN_POINT('',(1.5,2.4,-14.74)) ;
#118181=CARTESIAN_POINT('',(1.5,2.4,-14.74)) ;
#118182=CARTESIAN_POINT('',(7.9,2.4,-14.74)) ;
#118183=CARTESIAN_POINT('',(1.4,2.4,-14.74)) ;
#118184=CARTESIAN_POINT('',(7.9,2.1,-14.74)) ;
#118185=CARTESIAN_POINT('Origin',(1.4,2.4,-14.64)) ;
#118186=CARTESIAN_POINT('',(1.5,2.5,-14.64)) ;
#118187=CARTESIAN_POINT('Origin',(1.5,2.4,-14.64)) ;
#118188=CARTESIAN_POINT('',(7.9,2.5,-14.64)) ;
#118189=CARTESIAN_POINT('',(1.4,2.5,-14.64)) ;
#118190=CARTESIAN_POINT('Origin',(7.9,2.4,-14.64)) ;
#118191=CARTESIAN_POINT('Origin',(1.4,2.5,-14.5314213562373)) ;
#118192=CARTESIAN_POINT('',(1.5,2.5,-14.5314213562373)) ;
#118193=CARTESIAN_POINT('',(1.5,2.5,-14.5314213562373)) ;
#118194=CARTESIAN_POINT('',(7.9,2.5,-14.5314213562373)) ;
#118195=CARTESIAN_POINT('',(1.4,2.5,-14.5314213562373)) ;
#118196=CARTESIAN_POINT('',(7.9,2.5,-14.64)) ;
#118197=CARTESIAN_POINT('Origin',(1.4,2.6,-14.5314213562373)) ;
#118198=CARTESIAN_POINT('',(1.5,2.52928932188135,-14.4607106781187)) ;
#118199=CARTESIAN_POINT('Origin',(1.5,2.6,-14.5314213562373)) ;
#118200=CARTESIAN_POINT('',(7.9,2.52928932188135,-14.4607106781187)) ;
#118201=CARTESIAN_POINT('',(1.4,2.52928932188135,-14.4607106781187)) ;
#118202=CARTESIAN_POINT('Origin',(7.9,2.6,-14.5314213562373)) ;
#118203=CARTESIAN_POINT('Origin',(1.4,3.07928932188135,-13.9107106781187)) ;
#118204=CARTESIAN_POINT('',(1.5,3.07928932188135,-13.9107106781187)) ;
#118205=CARTESIAN_POINT('',(7.9,3.07928932188135,-13.9107106781187)) ;
#118206=CARTESIAN_POINT('',(1.4,3.07928932188135,-13.9107106781187)) ;
#118207=CARTESIAN_POINT('',(7.9,2.52928932188135,-14.4607106781187)) ;
#118208=CARTESIAN_POINT('Origin',(1.4,3.15,-13.9814213562373)) ;
#118209=CARTESIAN_POINT('',(7.9,3.25,-13.9814213562373)) ;
#118210=CARTESIAN_POINT('',(1.4,3.25,-13.9814213562373)) ;
#118211=CARTESIAN_POINT('Origin',(7.9,3.15,-13.9814213562373)) ;
#118212=CARTESIAN_POINT('Origin',(1.4,3.25,-16.4985786437627)) ;
#118213=CARTESIAN_POINT('',(1.5,3.25,-16.4985786437627)) ;
#118214=CARTESIAN_POINT('',(7.9,3.25,-13.9814213562373)) ;
#118215=CARTESIAN_POINT('Origin',(1.4,2.52928932188134,-16.0192893218813)) ;
#118216=CARTESIAN_POINT('',(1.5,2.52928932188134,-16.0192893218813)) ;
#118217=CARTESIAN_POINT('',(1.5,2.52928932188135,-16.0192893218813)) ;
#118218=CARTESIAN_POINT('',(7.9,2.52928932188134,-16.0192893218813)) ;
#118219=CARTESIAN_POINT('',(1.4,2.52928932188134,-16.0192893218813)) ;
#118220=CARTESIAN_POINT('',(7.9,3.07928932188134,-16.5692893218813)) ;
#118221=CARTESIAN_POINT('Origin',(1.4,2.6,-15.9485786437627)) ;
#118222=CARTESIAN_POINT('',(1.5,2.5,-15.9485786437627)) ;
#118223=CARTESIAN_POINT('Origin',(1.5,2.6,-15.9485786437627)) ;
#118224=CARTESIAN_POINT('',(7.9,2.5,-15.9485786437627)) ;
#118225=CARTESIAN_POINT('',(1.4,2.5,-15.9485786437627)) ;
#118226=CARTESIAN_POINT('Origin',(7.9,2.6,-15.9485786437627)) ;
#118227=CARTESIAN_POINT('Origin',(1.4,2.5,-15.84)) ;
#118228=CARTESIAN_POINT('',(1.5,2.5,-15.84)) ;
#118229=CARTESIAN_POINT('',(1.5,2.5,-15.84)) ;
#118230=CARTESIAN_POINT('',(7.9,2.5,-15.84)) ;
#118231=CARTESIAN_POINT('',(1.4,2.5,-15.84)) ;
#118232=CARTESIAN_POINT('',(7.9,2.5,-15.9485786437627)) ;
#118233=CARTESIAN_POINT('Origin',(1.4,2.4,-15.84)) ;
#118234=CARTESIAN_POINT('',(1.5,2.4,-15.74)) ;
#118235=CARTESIAN_POINT('Origin',(1.5,2.4,-15.84)) ;
#118236=CARTESIAN_POINT('',(7.9,2.4,-15.74)) ;
#118237=CARTESIAN_POINT('',(1.4,2.4,-15.74)) ;
#118238=CARTESIAN_POINT('Origin',(7.9,2.4,-15.84)) ;
#118239=CARTESIAN_POINT('Origin',(1.4,2.1,-15.74)) ;
#118240=CARTESIAN_POINT('',(1.5,2.1,-15.74)) ;
#118241=CARTESIAN_POINT('',(1.5,2.1,-15.74)) ;
#118242=CARTESIAN_POINT('',(7.9,2.1,-15.74)) ;
#118243=CARTESIAN_POINT('',(1.4,2.1,-15.74)) ;
#118244=CARTESIAN_POINT('',(7.9,2.4,-15.74)) ;
#118245=CARTESIAN_POINT('Origin',(1.4,2.1,-15.84)) ;
#118246=CARTESIAN_POINT('',(1.5,2.,-15.84)) ;
#118247=CARTESIAN_POINT('Origin',(1.5,2.1,-15.84)) ;
#118248=CARTESIAN_POINT('',(7.9,2.,-15.84)) ;
#118249=CARTESIAN_POINT('',(1.4,2.,-15.84)) ;
#118250=CARTESIAN_POINT('Origin',(7.9,2.1,-15.84)) ;
#118251=CARTESIAN_POINT('Origin',(1.4,2.,-15.84)) ;
#118252=CARTESIAN_POINT('',(1.5,2.,-16.79)) ;
#118253=CARTESIAN_POINT('',(1.5,2.,-16.79)) ;
#118254=CARTESIAN_POINT('',(7.9,2.,-16.79)) ;
#118255=CARTESIAN_POINT('',(1.4,2.,-16.79)) ;
#118256=CARTESIAN_POINT('',(7.9,2.,-15.84)) ;
#118257=CARTESIAN_POINT('Origin',(1.4,1.9,-16.79)) ;
#118258=CARTESIAN_POINT('',(1.5,1.9,-16.89)) ;
#118259=CARTESIAN_POINT('Origin',(1.5,1.9,-16.79)) ;
#118260=CARTESIAN_POINT('',(7.9,1.9,-16.89)) ;
#118261=CARTESIAN_POINT('',(1.4,1.9,-16.89)) ;
#118262=CARTESIAN_POINT('Origin',(7.9,1.9,-16.79)) ;
#118263=CARTESIAN_POINT('Origin',(1.4,1.9,-16.89)) ;
#118264=CARTESIAN_POINT('',(1.5,-2.15,-16.89)) ;
#118265=CARTESIAN_POINT('',(1.5,-2.15,-16.89)) ;
#118266=CARTESIAN_POINT('',(7.9,-2.15,-16.89)) ;
#118267=CARTESIAN_POINT('',(1.4,-2.15,-16.89)) ;
#118268=CARTESIAN_POINT('',(7.9,1.9,-16.89)) ;
#118269=CARTESIAN_POINT('Origin',(1.4,-2.15,-16.79)) ;
#118270=CARTESIAN_POINT('',(1.5,-2.25,-16.79)) ;
#118271=CARTESIAN_POINT('Origin',(1.5,-2.15,-16.79)) ;
#118272=CARTESIAN_POINT('',(7.9,-2.25,-16.79)) ;
#118273=CARTESIAN_POINT('',(1.4,-2.25,-16.79)) ;
#118274=CARTESIAN_POINT('Origin',(7.9,-2.15,-16.79)) ;
#118275=CARTESIAN_POINT('Origin',(1.4,-2.25,-16.1431195934094)) ;
#118276=CARTESIAN_POINT('',(1.5,-2.25,-16.1431195934094)) ;
#118277=CARTESIAN_POINT('',(1.5,-2.25,-16.1431195934094)) ;
#118278=CARTESIAN_POINT('',(7.9,-2.25,-16.1431195934094)) ;
#118279=CARTESIAN_POINT('',(1.4,-2.25,-16.1431195934094)) ;
#118280=CARTESIAN_POINT('',(7.9,-2.25,-16.79)) ;
#118281=CARTESIAN_POINT('Origin',(1.4,-2.15,-16.1431195934094)) ;
#118282=CARTESIAN_POINT('',(1.5,-2.23576512455516,-16.0916964137135)) ;
#118283=CARTESIAN_POINT('Origin',(1.5,-2.15,-16.1431195934094)) ;
#118284=CARTESIAN_POINT('',(7.9,-2.23576512455516,-16.0916964137135)) ;
#118285=CARTESIAN_POINT('',(1.4,-2.23576512455516,-16.0916964137135)) ;
#118286=CARTESIAN_POINT('Origin',(7.9,-2.15,-16.1431195934094)) ;
#118287=CARTESIAN_POINT('Origin',(1.4,-3.65625,-15.24)) ;
#118288=CARTESIAN_POINT('',(1.5,-2.23576512455516,-14.3883035862865)) ;
#118289=CARTESIAN_POINT('Origin',(1.5,-3.65625,-15.24)) ;
#118290=CARTESIAN_POINT('',(7.9,-2.23576512455516,-14.3883035862865)) ;
#118291=CARTESIAN_POINT('',(1.4,-2.23576512455516,-14.3883035862865)) ;
#118292=CARTESIAN_POINT('Origin',(7.9,-3.65625,-15.24)) ;
#118293=CARTESIAN_POINT('Origin',(1.4,-2.15,-14.3368804065906)) ;
#118294=CARTESIAN_POINT('',(1.5,-2.25,-14.3368804065906)) ;
#118295=CARTESIAN_POINT('Origin',(1.5,-2.15,-14.3368804065906)) ;
#118296=CARTESIAN_POINT('',(7.9,-2.25,-14.3368804065906)) ;
#118297=CARTESIAN_POINT('',(1.4,-2.25,-14.3368804065906)) ;
#118298=CARTESIAN_POINT('Origin',(7.9,-2.15,-14.3368804065906)) ;
#118299=CARTESIAN_POINT('Origin',(1.4,-2.25,-13.69)) ;
#118300=CARTESIAN_POINT('',(1.5,-2.25,-13.69)) ;
#118301=CARTESIAN_POINT('',(1.5,-2.25,-13.69)) ;
#118302=CARTESIAN_POINT('',(7.9,-2.25,-13.69)) ;
#118303=CARTESIAN_POINT('',(1.4,-2.25,-13.69)) ;
#118304=CARTESIAN_POINT('',(7.9,-2.25,-14.3368804065906)) ;
#118305=CARTESIAN_POINT('Origin',(1.4,-2.15,-13.69)) ;
#118306=CARTESIAN_POINT('',(1.5,-2.15,-13.59)) ;
#118307=CARTESIAN_POINT('Origin',(1.5,-2.15,-13.69)) ;
#118308=CARTESIAN_POINT('',(7.9,-2.15,-13.59)) ;
#118309=CARTESIAN_POINT('',(1.4,-2.15,-13.59)) ;
#118310=CARTESIAN_POINT('Origin',(7.9,-2.15,-13.69)) ;
#118311=CARTESIAN_POINT('Origin',(1.4,1.9,-13.59)) ;
#118312=CARTESIAN_POINT('',(1.5,1.9,-13.59)) ;
#118313=CARTESIAN_POINT('',(1.5,1.9,-13.59)) ;
#118314=CARTESIAN_POINT('',(7.9,1.9,-13.59)) ;
#118315=CARTESIAN_POINT('',(1.4,1.9,-13.59)) ;
#118316=CARTESIAN_POINT('',(7.9,-2.15,-13.59)) ;
#118317=CARTESIAN_POINT('Origin',(1.4,1.9,-13.69)) ;
#118318=CARTESIAN_POINT('',(1.5,2.,-13.69)) ;
#118319=CARTESIAN_POINT('Origin',(1.5,1.9,-13.69)) ;
#118320=CARTESIAN_POINT('',(7.9,2.,-13.69)) ;
#118321=CARTESIAN_POINT('',(1.4,2.,-13.69)) ;
#118322=CARTESIAN_POINT('Origin',(7.9,1.9,-13.69)) ;
#118323=CARTESIAN_POINT('Origin',(1.4,2.,-13.69)) ;
#118324=CARTESIAN_POINT('',(1.5,2.,-14.64)) ;
#118325=CARTESIAN_POINT('',(7.9,2.,-13.69)) ;
#118326=CARTESIAN_POINT('Origin',(1.4,2.1,-14.64)) ;
#118327=CARTESIAN_POINT('',(1.4,2.6,-14.64)) ;
#118328=CARTESIAN_POINT('',(1.4,2.4,-14.84)) ;
#118329=CARTESIAN_POINT('Origin',(1.4,2.4,-14.64)) ;
#118330=CARTESIAN_POINT('',(1.4,2.1,-14.84)) ;
#118331=CARTESIAN_POINT('',(1.4,2.1,-14.84)) ;
#118332=CARTESIAN_POINT('',(1.4,1.9,-14.64)) ;
#118333=CARTESIAN_POINT('Origin',(1.4,2.1,-14.64)) ;
#118334=CARTESIAN_POINT('',(1.4,1.9,-13.69)) ;
#118335=CARTESIAN_POINT('',(1.4,1.9,-13.69)) ;
#118336=CARTESIAN_POINT('',(1.4,-2.15,-13.69)) ;
#118337=CARTESIAN_POINT('',(1.4,-2.15,-13.69)) ;
#118338=CARTESIAN_POINT('',(1.4,-2.15,-14.3368804065906)) ;
#118339=CARTESIAN_POINT('',(1.4,-2.15,-14.3368804065906)) ;
#118340=CARTESIAN_POINT('',(1.4,-2.15,-16.1431195934094)) ;
#118341=CARTESIAN_POINT('Origin',(1.4,-3.65625,-15.24)) ;
#118342=CARTESIAN_POINT('',(1.4,-2.15,-16.79)) ;
#118343=CARTESIAN_POINT('',(1.4,-2.15,-16.79)) ;
#118344=CARTESIAN_POINT('',(1.4,1.9,-16.79)) ;
#118345=CARTESIAN_POINT('',(1.4,1.9,-16.79)) ;
#118346=CARTESIAN_POINT('',(1.4,1.9,-15.84)) ;
#118347=CARTESIAN_POINT('',(1.4,1.9,-15.84)) ;
#118348=CARTESIAN_POINT('',(1.4,2.1,-15.64)) ;
#118349=CARTESIAN_POINT('Origin',(1.4,2.1,-15.84)) ;
#118350=CARTESIAN_POINT('',(1.4,2.4,-15.64)) ;
#118351=CARTESIAN_POINT('',(1.4,2.4,-15.64)) ;
#118352=CARTESIAN_POINT('',(1.4,2.6,-15.84)) ;
#118353=CARTESIAN_POINT('Origin',(1.4,2.4,-15.84)) ;
#118354=CARTESIAN_POINT('',(1.4,2.6,-15.9485786437627)) ;
#118355=CARTESIAN_POINT('',(1.4,2.6,-15.9485786437627)) ;
#118356=CARTESIAN_POINT('',(1.4,3.15,-16.4985786437627)) ;
#118357=CARTESIAN_POINT('',(1.4,3.15,-16.4985786437627)) ;
#118358=CARTESIAN_POINT('',(1.4,3.15,-13.9814213562373)) ;
#118359=CARTESIAN_POINT('',(1.4,2.6,-14.5314213562373)) ;
#118360=CARTESIAN_POINT('',(1.4,2.6,-14.5314213562373)) ;
#118361=CARTESIAN_POINT('',(1.4,2.6,-14.64)) ;
#118362=CARTESIAN_POINT('Origin',(1.4,2.1,-10.83)) ;
#118363=CARTESIAN_POINT('',(1.5,2.,-10.83)) ;
#118364=CARTESIAN_POINT('',(7.9,2.,-10.83)) ;
#118365=CARTESIAN_POINT('',(1.4,2.,-10.83)) ;
#118366=CARTESIAN_POINT('',(1.5,2.1,-10.93)) ;
#118367=CARTESIAN_POINT('Origin',(1.5,2.1,-10.83)) ;
#118368=CARTESIAN_POINT('',(7.9,2.1,-10.93)) ;
#118369=CARTESIAN_POINT('',(1.4,2.1,-10.93)) ;
#118370=CARTESIAN_POINT('Origin',(7.9,2.1,-10.83)) ;
#118371=CARTESIAN_POINT('Origin',(1.4,2.4,-10.93)) ;
#118372=CARTESIAN_POINT('',(1.5,2.4,-10.93)) ;
#118373=CARTESIAN_POINT('',(1.5,2.4,-10.93)) ;
#118374=CARTESIAN_POINT('',(7.9,2.4,-10.93)) ;
#118375=CARTESIAN_POINT('',(1.4,2.4,-10.93)) ;
#118376=CARTESIAN_POINT('',(7.9,2.1,-10.93)) ;
#118377=CARTESIAN_POINT('Origin',(1.4,2.4,-10.83)) ;
#118378=CARTESIAN_POINT('',(1.5,2.5,-10.83)) ;
#118379=CARTESIAN_POINT('Origin',(1.5,2.4,-10.83)) ;
#118380=CARTESIAN_POINT('',(7.9,2.5,-10.83)) ;
#118381=CARTESIAN_POINT('',(1.4,2.5,-10.83)) ;
#118382=CARTESIAN_POINT('Origin',(7.9,2.4,-10.83)) ;
#118383=CARTESIAN_POINT('Origin',(1.4,2.5,-10.7214213562373)) ;
#118384=CARTESIAN_POINT('',(1.5,2.5,-10.7214213562373)) ;
#118385=CARTESIAN_POINT('',(1.5,2.5,-10.7214213562373)) ;
#118386=CARTESIAN_POINT('',(7.9,2.5,-10.7214213562373)) ;
#118387=CARTESIAN_POINT('',(1.4,2.5,-10.7214213562373)) ;
#118388=CARTESIAN_POINT('',(7.9,2.5,-10.83)) ;
#118389=CARTESIAN_POINT('Origin',(1.4,2.6,-10.7214213562373)) ;
#118390=CARTESIAN_POINT('',(1.5,2.52928932188135,-10.6507106781187)) ;
#118391=CARTESIAN_POINT('Origin',(1.5,2.6,-10.7214213562373)) ;
#118392=CARTESIAN_POINT('',(7.9,2.52928932188135,-10.6507106781187)) ;
#118393=CARTESIAN_POINT('',(1.4,2.52928932188135,-10.6507106781187)) ;
#118394=CARTESIAN_POINT('Origin',(7.9,2.6,-10.7214213562373)) ;
#118395=CARTESIAN_POINT('Origin',(1.4,3.07928932188135,-10.1007106781187)) ;
#118396=CARTESIAN_POINT('',(1.5,3.07928932188135,-10.1007106781187)) ;
#118397=CARTESIAN_POINT('',(7.9,3.07928932188135,-10.1007106781187)) ;
#118398=CARTESIAN_POINT('',(1.4,3.07928932188135,-10.1007106781187)) ;
#118399=CARTESIAN_POINT('',(7.9,2.52928932188135,-10.6507106781187)) ;
#118400=CARTESIAN_POINT('Origin',(1.4,3.15,-10.1714213562373)) ;
#118401=CARTESIAN_POINT('',(7.9,3.25,-10.1714213562373)) ;
#118402=CARTESIAN_POINT('',(1.4,3.25,-10.1714213562373)) ;
#118403=CARTESIAN_POINT('Origin',(7.9,3.15,-10.1714213562373)) ;
#118404=CARTESIAN_POINT('Origin',(1.4,3.25,-12.6885786437627)) ;
#118405=CARTESIAN_POINT('',(1.5,3.25,-12.6885786437627)) ;
#118406=CARTESIAN_POINT('',(7.9,3.25,-10.1714213562373)) ;
#118407=CARTESIAN_POINT('Origin',(1.4,2.52928932188134,-12.2092893218813)) ;
#118408=CARTESIAN_POINT('',(1.5,2.52928932188134,-12.2092893218813)) ;
#118409=CARTESIAN_POINT('',(1.5,2.52928932188134,-12.2092893218813)) ;
#118410=CARTESIAN_POINT('',(7.9,2.52928932188134,-12.2092893218813)) ;
#118411=CARTESIAN_POINT('',(1.4,2.52928932188134,-12.2092893218813)) ;
#118412=CARTESIAN_POINT('',(7.9,3.07928932188135,-12.7592893218813)) ;
#118413=CARTESIAN_POINT('Origin',(1.4,2.6,-12.1385786437627)) ;
#118414=CARTESIAN_POINT('',(1.5,2.5,-12.1385786437627)) ;
#118415=CARTESIAN_POINT('Origin',(1.5,2.6,-12.1385786437627)) ;
#118416=CARTESIAN_POINT('',(7.9,2.5,-12.1385786437627)) ;
#118417=CARTESIAN_POINT('',(1.4,2.5,-12.1385786437627)) ;
#118418=CARTESIAN_POINT('Origin',(7.9,2.6,-12.1385786437627)) ;
#118419=CARTESIAN_POINT('Origin',(1.4,2.5,-12.03)) ;
#118420=CARTESIAN_POINT('',(1.5,2.5,-12.03)) ;
#118421=CARTESIAN_POINT('',(1.5,2.5,-12.03)) ;
#118422=CARTESIAN_POINT('',(7.9,2.5,-12.03)) ;
#118423=CARTESIAN_POINT('',(1.4,2.5,-12.03)) ;
#118424=CARTESIAN_POINT('',(7.9,2.5,-12.1385786437627)) ;
#118425=CARTESIAN_POINT('Origin',(1.4,2.4,-12.03)) ;
#118426=CARTESIAN_POINT('',(1.5,2.4,-11.93)) ;
#118427=CARTESIAN_POINT('Origin',(1.5,2.4,-12.03)) ;
#118428=CARTESIAN_POINT('',(7.9,2.4,-11.93)) ;
#118429=CARTESIAN_POINT('',(1.4,2.4,-11.93)) ;
#118430=CARTESIAN_POINT('Origin',(7.9,2.4,-12.03)) ;
#118431=CARTESIAN_POINT('Origin',(1.4,2.1,-11.93)) ;
#118432=CARTESIAN_POINT('',(1.5,2.1,-11.93)) ;
#118433=CARTESIAN_POINT('',(1.5,2.1,-11.93)) ;
#118434=CARTESIAN_POINT('',(7.9,2.1,-11.93)) ;
#118435=CARTESIAN_POINT('',(1.4,2.1,-11.93)) ;
#118436=CARTESIAN_POINT('',(7.9,2.4,-11.93)) ;
#118437=CARTESIAN_POINT('Origin',(1.4,2.1,-12.03)) ;
#118438=CARTESIAN_POINT('',(1.5,2.,-12.03)) ;
#118439=CARTESIAN_POINT('Origin',(1.5,2.1,-12.03)) ;
#118440=CARTESIAN_POINT('',(7.9,2.,-12.03)) ;
#118441=CARTESIAN_POINT('',(1.4,2.,-12.03)) ;
#118442=CARTESIAN_POINT('Origin',(7.9,2.1,-12.03)) ;
#118443=CARTESIAN_POINT('Origin',(1.4,2.,-12.03)) ;
#118444=CARTESIAN_POINT('',(1.5,2.,-12.98)) ;
#118445=CARTESIAN_POINT('',(1.5,2.,-12.98)) ;
#118446=CARTESIAN_POINT('',(7.9,2.,-12.98)) ;
#118447=CARTESIAN_POINT('',(1.4,2.,-12.98)) ;
#118448=CARTESIAN_POINT('',(7.9,2.,-12.03)) ;
#118449=CARTESIAN_POINT('Origin',(1.4,1.9,-12.98)) ;
#118450=CARTESIAN_POINT('',(1.5,1.9,-13.08)) ;
#118451=CARTESIAN_POINT('Origin',(1.5,1.9,-12.98)) ;
#118452=CARTESIAN_POINT('',(7.9,1.9,-13.08)) ;
#118453=CARTESIAN_POINT('',(1.4,1.9,-13.08)) ;
#118454=CARTESIAN_POINT('Origin',(7.9,1.9,-12.98)) ;
#118455=CARTESIAN_POINT('Origin',(1.4,1.9,-13.08)) ;
#118456=CARTESIAN_POINT('',(1.5,-2.15,-13.08)) ;
#118457=CARTESIAN_POINT('',(1.5,-2.15,-13.08)) ;
#118458=CARTESIAN_POINT('',(7.9,-2.15,-13.08)) ;
#118459=CARTESIAN_POINT('',(1.4,-2.15,-13.08)) ;
#118460=CARTESIAN_POINT('',(7.9,1.9,-13.08)) ;
#118461=CARTESIAN_POINT('Origin',(1.4,-2.15,-12.98)) ;
#118462=CARTESIAN_POINT('',(1.5,-2.25,-12.98)) ;
#118463=CARTESIAN_POINT('Origin',(1.5,-2.15,-12.98)) ;
#118464=CARTESIAN_POINT('',(7.9,-2.25,-12.98)) ;
#118465=CARTESIAN_POINT('',(1.4,-2.25,-12.98)) ;
#118466=CARTESIAN_POINT('Origin',(7.9,-2.15,-12.98)) ;
#118467=CARTESIAN_POINT('Origin',(1.4,-2.25,-12.3331195934094)) ;
#118468=CARTESIAN_POINT('',(1.5,-2.25,-12.3331195934094)) ;
#118469=CARTESIAN_POINT('',(1.5,-2.25,-12.3331195934094)) ;
#118470=CARTESIAN_POINT('',(7.9,-2.25,-12.3331195934094)) ;
#118471=CARTESIAN_POINT('',(1.4,-2.25,-12.3331195934094)) ;
#118472=CARTESIAN_POINT('',(7.9,-2.25,-12.98)) ;
#118473=CARTESIAN_POINT('Origin',(1.4,-2.15,-12.3331195934094)) ;
#118474=CARTESIAN_POINT('',(1.5,-2.23576512455516,-12.2816964137135)) ;
#118475=CARTESIAN_POINT('Origin',(1.5,-2.15,-12.3331195934094)) ;
#118476=CARTESIAN_POINT('',(7.9,-2.23576512455516,-12.2816964137135)) ;
#118477=CARTESIAN_POINT('',(1.4,-2.23576512455516,-12.2816964137135)) ;
#118478=CARTESIAN_POINT('Origin',(7.9,-2.15,-12.3331195934094)) ;
#118479=CARTESIAN_POINT('Origin',(1.4,-3.65625,-11.43)) ;
#118480=CARTESIAN_POINT('',(1.5,-2.23576512455516,-10.5783035862865)) ;
#118481=CARTESIAN_POINT('Origin',(1.5,-3.65625,-11.43)) ;
#118482=CARTESIAN_POINT('',(7.9,-2.23576512455516,-10.5783035862865)) ;
#118483=CARTESIAN_POINT('',(1.4,-2.23576512455516,-10.5783035862865)) ;
#118484=CARTESIAN_POINT('Origin',(7.9,-3.65625,-11.43)) ;
#118485=CARTESIAN_POINT('Origin',(1.4,-2.15,-10.5268804065906)) ;
#118486=CARTESIAN_POINT('',(1.5,-2.25,-10.5268804065906)) ;
#118487=CARTESIAN_POINT('Origin',(1.5,-2.15,-10.5268804065906)) ;
#118488=CARTESIAN_POINT('',(7.9,-2.25,-10.5268804065906)) ;
#118489=CARTESIAN_POINT('',(1.4,-2.25,-10.5268804065906)) ;
#118490=CARTESIAN_POINT('Origin',(7.9,-2.15,-10.5268804065906)) ;
#118491=CARTESIAN_POINT('Origin',(1.4,-2.25,-9.88)) ;
#118492=CARTESIAN_POINT('',(1.5,-2.25,-9.88)) ;
#118493=CARTESIAN_POINT('',(1.5,-2.25,-9.88)) ;
#118494=CARTESIAN_POINT('',(7.9,-2.25,-9.88)) ;
#118495=CARTESIAN_POINT('',(1.4,-2.25,-9.88)) ;
#118496=CARTESIAN_POINT('',(7.9,-2.25,-10.5268804065906)) ;
#118497=CARTESIAN_POINT('Origin',(1.4,-2.15,-9.88)) ;
#118498=CARTESIAN_POINT('',(1.5,-2.15,-9.78)) ;
#118499=CARTESIAN_POINT('Origin',(1.5,-2.15,-9.88)) ;
#118500=CARTESIAN_POINT('',(7.9,-2.15,-9.78)) ;
#118501=CARTESIAN_POINT('',(1.4,-2.15,-9.78)) ;
#118502=CARTESIAN_POINT('Origin',(7.9,-2.15,-9.88)) ;
#118503=CARTESIAN_POINT('Origin',(1.4,1.9,-9.78)) ;
#118504=CARTESIAN_POINT('',(1.5,1.9,-9.78)) ;
#118505=CARTESIAN_POINT('',(1.5,1.9,-9.78)) ;
#118506=CARTESIAN_POINT('',(7.9,1.9,-9.78)) ;
#118507=CARTESIAN_POINT('',(1.4,1.9,-9.78)) ;
#118508=CARTESIAN_POINT('',(7.9,-2.15,-9.78)) ;
#118509=CARTESIAN_POINT('Origin',(1.4,1.9,-9.88)) ;
#118510=CARTESIAN_POINT('',(1.5,2.,-9.88)) ;
#118511=CARTESIAN_POINT('Origin',(1.5,1.9,-9.88)) ;
#118512=CARTESIAN_POINT('',(7.9,2.,-9.88)) ;
#118513=CARTESIAN_POINT('',(1.4,2.,-9.88)) ;
#118514=CARTESIAN_POINT('Origin',(7.9,1.9,-9.88)) ;
#118515=CARTESIAN_POINT('Origin',(1.4,2.,-9.88)) ;
#118516=CARTESIAN_POINT('',(1.5,2.,-10.83)) ;
#118517=CARTESIAN_POINT('',(7.9,2.,-9.88)) ;
#118518=CARTESIAN_POINT('Origin',(1.4,2.1,-10.83)) ;
#118519=CARTESIAN_POINT('',(1.4,2.6,-10.83)) ;
#118520=CARTESIAN_POINT('',(1.4,2.4,-11.03)) ;
#118521=CARTESIAN_POINT('Origin',(1.4,2.4,-10.83)) ;
#118522=CARTESIAN_POINT('',(1.4,2.1,-11.03)) ;
#118523=CARTESIAN_POINT('',(1.4,2.1,-11.03)) ;
#118524=CARTESIAN_POINT('',(1.4,1.9,-10.83)) ;
#118525=CARTESIAN_POINT('Origin',(1.4,2.1,-10.83)) ;
#118526=CARTESIAN_POINT('',(1.4,1.9,-9.88)) ;
#118527=CARTESIAN_POINT('',(1.4,1.9,-9.88)) ;
#118528=CARTESIAN_POINT('',(1.4,-2.15,-9.88)) ;
#118529=CARTESIAN_POINT('',(1.4,-2.15,-9.88)) ;
#118530=CARTESIAN_POINT('',(1.4,-2.15,-10.5268804065906)) ;
#118531=CARTESIAN_POINT('',(1.4,-2.15,-10.5268804065906)) ;
#118532=CARTESIAN_POINT('',(1.4,-2.15,-12.3331195934094)) ;
#118533=CARTESIAN_POINT('Origin',(1.4,-3.65625,-11.43)) ;
#118534=CARTESIAN_POINT('',(1.4,-2.15,-12.98)) ;
#118535=CARTESIAN_POINT('',(1.4,-2.15,-12.98)) ;
#118536=CARTESIAN_POINT('',(1.4,1.9,-12.98)) ;
#118537=CARTESIAN_POINT('',(1.4,1.9,-12.98)) ;
#118538=CARTESIAN_POINT('',(1.4,1.9,-12.03)) ;
#118539=CARTESIAN_POINT('',(1.4,1.9,-12.03)) ;
#118540=CARTESIAN_POINT('',(1.4,2.1,-11.83)) ;
#118541=CARTESIAN_POINT('Origin',(1.4,2.1,-12.03)) ;
#118542=CARTESIAN_POINT('',(1.4,2.4,-11.83)) ;
#118543=CARTESIAN_POINT('',(1.4,2.4,-11.83)) ;
#118544=CARTESIAN_POINT('',(1.4,2.6,-12.03)) ;
#118545=CARTESIAN_POINT('Origin',(1.4,2.4,-12.03)) ;
#118546=CARTESIAN_POINT('',(1.4,2.6,-12.1385786437627)) ;
#118547=CARTESIAN_POINT('',(1.4,2.6,-12.1385786437627)) ;
#118548=CARTESIAN_POINT('',(1.4,3.15,-12.6885786437627)) ;
#118549=CARTESIAN_POINT('',(1.4,3.15,-12.6885786437627)) ;
#118550=CARTESIAN_POINT('',(1.4,3.15,-10.1714213562373)) ;
#118551=CARTESIAN_POINT('',(1.4,2.6,-10.7214213562373)) ;
#118552=CARTESIAN_POINT('',(1.4,2.6,-10.7214213562373)) ;
#118553=CARTESIAN_POINT('',(1.4,2.6,-10.83)) ;
#118554=CARTESIAN_POINT('Origin',(1.4,2.1,-7.02)) ;
#118555=CARTESIAN_POINT('',(1.5,2.,-7.02)) ;
#118556=CARTESIAN_POINT('',(7.9,2.,-7.02)) ;
#118557=CARTESIAN_POINT('',(1.4,2.,-7.02)) ;
#118558=CARTESIAN_POINT('',(1.5,2.1,-7.12)) ;
#118559=CARTESIAN_POINT('Origin',(1.5,2.1,-7.02)) ;
#118560=CARTESIAN_POINT('',(7.9,2.1,-7.12)) ;
#118561=CARTESIAN_POINT('',(1.4,2.1,-7.12)) ;
#118562=CARTESIAN_POINT('Origin',(7.9,2.1,-7.02)) ;
#118563=CARTESIAN_POINT('Origin',(1.4,2.4,-7.12)) ;
#118564=CARTESIAN_POINT('',(1.5,2.4,-7.12)) ;
#118565=CARTESIAN_POINT('',(1.5,2.4,-7.12)) ;
#118566=CARTESIAN_POINT('',(7.9,2.4,-7.12)) ;
#118567=CARTESIAN_POINT('',(1.4,2.4,-7.12)) ;
#118568=CARTESIAN_POINT('',(7.9,2.1,-7.12)) ;
#118569=CARTESIAN_POINT('Origin',(1.4,2.4,-7.02)) ;
#118570=CARTESIAN_POINT('',(1.5,2.5,-7.02)) ;
#118571=CARTESIAN_POINT('Origin',(1.5,2.4,-7.02)) ;
#118572=CARTESIAN_POINT('',(7.9,2.5,-7.02)) ;
#118573=CARTESIAN_POINT('',(1.4,2.5,-7.02)) ;
#118574=CARTESIAN_POINT('Origin',(7.9,2.4,-7.02)) ;
#118575=CARTESIAN_POINT('Origin',(1.4,2.5,-6.91142135623731)) ;
#118576=CARTESIAN_POINT('',(1.5,2.5,-6.91142135623731)) ;
#118577=CARTESIAN_POINT('',(1.5,2.5,-6.91142135623731)) ;
#118578=CARTESIAN_POINT('',(7.9,2.5,-6.91142135623731)) ;
#118579=CARTESIAN_POINT('',(1.4,2.5,-6.91142135623731)) ;
#118580=CARTESIAN_POINT('',(7.9,2.5,-7.02)) ;
#118581=CARTESIAN_POINT('Origin',(1.4,2.6,-6.91142135623731)) ;
#118582=CARTESIAN_POINT('',(1.5,2.52928932188135,-6.84071067811866)) ;
#118583=CARTESIAN_POINT('Origin',(1.5,2.6,-6.91142135623731)) ;
#118584=CARTESIAN_POINT('',(7.9,2.52928932188135,-6.84071067811866)) ;
#118585=CARTESIAN_POINT('',(1.4,2.52928932188135,-6.84071067811866)) ;
#118586=CARTESIAN_POINT('Origin',(7.9,2.6,-6.91142135623731)) ;
#118587=CARTESIAN_POINT('Origin',(1.4,3.07928932188135,-6.29071067811866)) ;
#118588=CARTESIAN_POINT('',(1.5,3.07928932188135,-6.29071067811866)) ;
#118589=CARTESIAN_POINT('',(7.9,3.07928932188135,-6.29071067811866)) ;
#118590=CARTESIAN_POINT('',(1.4,3.07928932188135,-6.29071067811866)) ;
#118591=CARTESIAN_POINT('',(7.9,2.52928932188135,-6.84071067811866)) ;
#118592=CARTESIAN_POINT('Origin',(1.4,3.15,-6.36142135623731)) ;
#118593=CARTESIAN_POINT('',(7.9,3.25,-6.36142135623731)) ;
#118594=CARTESIAN_POINT('',(1.4,3.25,-6.36142135623731)) ;
#118595=CARTESIAN_POINT('Origin',(7.9,3.15,-6.36142135623731)) ;
#118596=CARTESIAN_POINT('Origin',(1.4,3.25,-8.87857864376269)) ;
#118597=CARTESIAN_POINT('',(1.5,3.25,-8.87857864376269)) ;
#118598=CARTESIAN_POINT('',(7.9,3.25,-6.36142135623731)) ;
#118599=CARTESIAN_POINT('Origin',(1.4,2.52928932188134,-8.39928932188135)) ;
#118600=CARTESIAN_POINT('',(1.5,2.52928932188134,-8.39928932188135)) ;
#118601=CARTESIAN_POINT('',(1.5,2.52928932188134,-8.39928932188135)) ;
#118602=CARTESIAN_POINT('',(7.9,2.52928932188134,-8.39928932188135)) ;
#118603=CARTESIAN_POINT('',(1.4,2.52928932188134,-8.39928932188135)) ;
#118604=CARTESIAN_POINT('',(7.9,3.07928932188135,-8.94928932188134)) ;
#118605=CARTESIAN_POINT('Origin',(1.4,2.6,-8.32857864376269)) ;
#118606=CARTESIAN_POINT('',(1.5,2.5,-8.32857864376269)) ;
#118607=CARTESIAN_POINT('Origin',(1.5,2.6,-8.32857864376269)) ;
#118608=CARTESIAN_POINT('',(7.9,2.5,-8.32857864376269)) ;
#118609=CARTESIAN_POINT('',(1.4,2.5,-8.32857864376269)) ;
#118610=CARTESIAN_POINT('Origin',(7.9,2.6,-8.32857864376269)) ;
#118611=CARTESIAN_POINT('Origin',(1.4,2.5,-8.22)) ;
#118612=CARTESIAN_POINT('',(1.5,2.5,-8.22)) ;
#118613=CARTESIAN_POINT('',(1.5,2.5,-8.22)) ;
#118614=CARTESIAN_POINT('',(7.9,2.5,-8.22)) ;
#118615=CARTESIAN_POINT('',(1.4,2.5,-8.22)) ;
#118616=CARTESIAN_POINT('',(7.9,2.5,-8.32857864376269)) ;
#118617=CARTESIAN_POINT('Origin',(1.4,2.4,-8.22)) ;
#118618=CARTESIAN_POINT('',(1.5,2.4,-8.12)) ;
#118619=CARTESIAN_POINT('Origin',(1.5,2.4,-8.22)) ;
#118620=CARTESIAN_POINT('',(7.9,2.4,-8.12)) ;
#118621=CARTESIAN_POINT('',(1.4,2.4,-8.12)) ;
#118622=CARTESIAN_POINT('Origin',(7.9,2.4,-8.22)) ;
#118623=CARTESIAN_POINT('Origin',(1.4,2.1,-8.12)) ;
#118624=CARTESIAN_POINT('',(1.5,2.1,-8.12)) ;
#118625=CARTESIAN_POINT('',(1.5,2.1,-8.12)) ;
#118626=CARTESIAN_POINT('',(7.9,2.1,-8.12)) ;
#118627=CARTESIAN_POINT('',(1.4,2.1,-8.12)) ;
#118628=CARTESIAN_POINT('',(7.9,2.4,-8.12)) ;
#118629=CARTESIAN_POINT('Origin',(1.4,2.1,-8.22)) ;
#118630=CARTESIAN_POINT('',(1.5,2.,-8.22)) ;
#118631=CARTESIAN_POINT('Origin',(1.5,2.1,-8.22)) ;
#118632=CARTESIAN_POINT('',(7.9,2.,-8.22)) ;
#118633=CARTESIAN_POINT('',(1.4,2.,-8.22)) ;
#118634=CARTESIAN_POINT('Origin',(7.9,2.1,-8.22)) ;
#118635=CARTESIAN_POINT('Origin',(1.4,2.,-8.22)) ;
#118636=CARTESIAN_POINT('',(1.5,2.,-9.17)) ;
#118637=CARTESIAN_POINT('',(1.5,2.,-9.17)) ;
#118638=CARTESIAN_POINT('',(7.9,2.,-9.17)) ;
#118639=CARTESIAN_POINT('',(1.4,2.,-9.17)) ;
#118640=CARTESIAN_POINT('',(7.9,2.,-8.22)) ;
#118641=CARTESIAN_POINT('Origin',(1.4,1.9,-9.17)) ;
#118642=CARTESIAN_POINT('',(1.5,1.9,-9.27)) ;
#118643=CARTESIAN_POINT('Origin',(1.5,1.9,-9.17)) ;
#118644=CARTESIAN_POINT('',(7.9,1.9,-9.27)) ;
#118645=CARTESIAN_POINT('',(1.4,1.9,-9.27)) ;
#118646=CARTESIAN_POINT('Origin',(7.9,1.9,-9.17)) ;
#118647=CARTESIAN_POINT('Origin',(1.4,1.9,-9.27)) ;
#118648=CARTESIAN_POINT('',(1.5,-2.15,-9.27)) ;
#118649=CARTESIAN_POINT('',(1.5,-2.15,-9.27)) ;
#118650=CARTESIAN_POINT('',(7.9,-2.15,-9.27)) ;
#118651=CARTESIAN_POINT('',(1.4,-2.15,-9.27)) ;
#118652=CARTESIAN_POINT('',(7.9,1.9,-9.27)) ;
#118653=CARTESIAN_POINT('Origin',(1.4,-2.15,-9.17)) ;
#118654=CARTESIAN_POINT('',(1.5,-2.25,-9.17)) ;
#118655=CARTESIAN_POINT('Origin',(1.5,-2.15,-9.17)) ;
#118656=CARTESIAN_POINT('',(7.9,-2.25,-9.17)) ;
#118657=CARTESIAN_POINT('',(1.4,-2.25,-9.17)) ;
#118658=CARTESIAN_POINT('Origin',(7.9,-2.15,-9.17)) ;
#118659=CARTESIAN_POINT('Origin',(1.4,-2.25,-8.52311959340942)) ;
#118660=CARTESIAN_POINT('',(1.5,-2.25,-8.52311959340942)) ;
#118661=CARTESIAN_POINT('',(1.5,-2.25,-8.52311959340942)) ;
#118662=CARTESIAN_POINT('',(7.9,-2.25,-8.52311959340942)) ;
#118663=CARTESIAN_POINT('',(1.4,-2.25,-8.52311959340942)) ;
#118664=CARTESIAN_POINT('',(7.9,-2.25,-9.17)) ;
#118665=CARTESIAN_POINT('Origin',(1.4,-2.15,-8.52311959340942)) ;
#118666=CARTESIAN_POINT('',(1.5,-2.23576512455516,-8.47169641371351)) ;
#118667=CARTESIAN_POINT('Origin',(1.5,-2.15,-8.52311959340942)) ;
#118668=CARTESIAN_POINT('',(7.9,-2.23576512455516,-8.47169641371351)) ;
#118669=CARTESIAN_POINT('',(1.4,-2.23576512455516,-8.47169641371351)) ;
#118670=CARTESIAN_POINT('Origin',(7.9,-2.15,-8.52311959340942)) ;
#118671=CARTESIAN_POINT('Origin',(1.4,-3.65625,-7.62)) ;
#118672=CARTESIAN_POINT('',(1.5,-2.23576512455516,-6.76830358628649)) ;
#118673=CARTESIAN_POINT('Origin',(1.5,-3.65625,-7.62)) ;
#118674=CARTESIAN_POINT('',(7.9,-2.23576512455516,-6.76830358628649)) ;
#118675=CARTESIAN_POINT('',(1.4,-2.23576512455516,-6.76830358628649)) ;
#118676=CARTESIAN_POINT('Origin',(7.9,-3.65625,-7.62)) ;
#118677=CARTESIAN_POINT('Origin',(1.4,-2.15,-6.71688040659058)) ;
#118678=CARTESIAN_POINT('',(1.5,-2.25,-6.71688040659058)) ;
#118679=CARTESIAN_POINT('Origin',(1.5,-2.15,-6.71688040659058)) ;
#118680=CARTESIAN_POINT('',(7.9,-2.25,-6.71688040659058)) ;
#118681=CARTESIAN_POINT('',(1.4,-2.25,-6.71688040659058)) ;
#118682=CARTESIAN_POINT('Origin',(7.9,-2.15,-6.71688040659058)) ;
#118683=CARTESIAN_POINT('Origin',(1.4,-2.25,-6.07)) ;
#118684=CARTESIAN_POINT('',(1.5,-2.25,-6.07)) ;
#118685=CARTESIAN_POINT('',(1.5,-2.25,-6.07)) ;
#118686=CARTESIAN_POINT('',(7.9,-2.25,-6.07)) ;
#118687=CARTESIAN_POINT('',(1.4,-2.25,-6.07)) ;
#118688=CARTESIAN_POINT('',(7.9,-2.25,-6.71688040659058)) ;
#118689=CARTESIAN_POINT('Origin',(1.4,-2.15,-6.07)) ;
#118690=CARTESIAN_POINT('',(1.5,-2.15,-5.97)) ;
#118691=CARTESIAN_POINT('Origin',(1.5,-2.15,-6.07)) ;
#118692=CARTESIAN_POINT('',(7.9,-2.15,-5.97)) ;
#118693=CARTESIAN_POINT('',(1.4,-2.15,-5.97)) ;
#118694=CARTESIAN_POINT('Origin',(7.9,-2.15,-6.07)) ;
#118695=CARTESIAN_POINT('Origin',(1.4,1.9,-5.97)) ;
#118696=CARTESIAN_POINT('',(1.5,1.9,-5.97)) ;
#118697=CARTESIAN_POINT('',(1.5,1.9,-5.97)) ;
#118698=CARTESIAN_POINT('',(7.9,1.9,-5.97)) ;
#118699=CARTESIAN_POINT('',(1.4,1.9,-5.97)) ;
#118700=CARTESIAN_POINT('',(7.9,-2.15,-5.97)) ;
#118701=CARTESIAN_POINT('Origin',(1.4,1.9,-6.07)) ;
#118702=CARTESIAN_POINT('',(1.5,2.,-6.07)) ;
#118703=CARTESIAN_POINT('Origin',(1.5,1.9,-6.07)) ;
#118704=CARTESIAN_POINT('',(7.9,2.,-6.07)) ;
#118705=CARTESIAN_POINT('',(1.4,2.,-6.07)) ;
#118706=CARTESIAN_POINT('Origin',(7.9,1.9,-6.07)) ;
#118707=CARTESIAN_POINT('Origin',(1.4,2.,-6.07)) ;
#118708=CARTESIAN_POINT('',(1.5,2.,-7.02)) ;
#118709=CARTESIAN_POINT('',(7.9,2.,-6.07)) ;
#118710=CARTESIAN_POINT('Origin',(1.4,2.1,-7.02)) ;
#118711=CARTESIAN_POINT('',(1.4,2.6,-7.02)) ;
#118712=CARTESIAN_POINT('',(1.4,2.4,-7.22)) ;
#118713=CARTESIAN_POINT('Origin',(1.4,2.4,-7.02)) ;
#118714=CARTESIAN_POINT('',(1.4,2.1,-7.22)) ;
#118715=CARTESIAN_POINT('',(1.4,2.1,-7.22)) ;
#118716=CARTESIAN_POINT('',(1.4,1.9,-7.02)) ;
#118717=CARTESIAN_POINT('Origin',(1.4,2.1,-7.02)) ;
#118718=CARTESIAN_POINT('',(1.4,1.9,-6.07)) ;
#118719=CARTESIAN_POINT('',(1.4,1.9,-6.07)) ;
#118720=CARTESIAN_POINT('',(1.4,-2.15,-6.07)) ;
#118721=CARTESIAN_POINT('',(1.4,-2.15,-6.07)) ;
#118722=CARTESIAN_POINT('',(1.4,-2.15,-6.71688040659058)) ;
#118723=CARTESIAN_POINT('',(1.4,-2.15,-6.71688040659058)) ;
#118724=CARTESIAN_POINT('',(1.4,-2.15,-8.52311959340942)) ;
#118725=CARTESIAN_POINT('Origin',(1.4,-3.65625,-7.62)) ;
#118726=CARTESIAN_POINT('',(1.4,-2.15,-9.17)) ;
#118727=CARTESIAN_POINT('',(1.4,-2.15,-9.17)) ;
#118728=CARTESIAN_POINT('',(1.4,1.9,-9.17)) ;
#118729=CARTESIAN_POINT('',(1.4,1.9,-9.17)) ;
#118730=CARTESIAN_POINT('',(1.4,1.9,-8.22)) ;
#118731=CARTESIAN_POINT('',(1.4,1.9,-8.22)) ;
#118732=CARTESIAN_POINT('',(1.4,2.1,-8.02)) ;
#118733=CARTESIAN_POINT('Origin',(1.4,2.1,-8.22)) ;
#118734=CARTESIAN_POINT('',(1.4,2.4,-8.02)) ;
#118735=CARTESIAN_POINT('',(1.4,2.4,-8.02)) ;
#118736=CARTESIAN_POINT('',(1.4,2.6,-8.22)) ;
#118737=CARTESIAN_POINT('Origin',(1.4,2.4,-8.22)) ;
#118738=CARTESIAN_POINT('',(1.4,2.6,-8.32857864376269)) ;
#118739=CARTESIAN_POINT('',(1.4,2.6,-8.32857864376269)) ;
#118740=CARTESIAN_POINT('',(1.4,3.15,-8.87857864376269)) ;
#118741=CARTESIAN_POINT('',(1.4,3.15,-8.87857864376269)) ;
#118742=CARTESIAN_POINT('',(1.4,3.15,-6.36142135623731)) ;
#118743=CARTESIAN_POINT('',(1.4,2.6,-6.91142135623731)) ;
#118744=CARTESIAN_POINT('',(1.4,2.6,-6.91142135623731)) ;
#118745=CARTESIAN_POINT('',(1.4,2.6,-7.02)) ;
#118746=CARTESIAN_POINT('Origin',(1.4,2.1,-3.21)) ;
#118747=CARTESIAN_POINT('',(1.5,2.,-3.21)) ;
#118748=CARTESIAN_POINT('',(7.9,2.,-3.21)) ;
#118749=CARTESIAN_POINT('',(1.4,2.,-3.21)) ;
#118750=CARTESIAN_POINT('',(1.5,2.1,-3.31)) ;
#118751=CARTESIAN_POINT('Origin',(1.5,2.1,-3.21)) ;
#118752=CARTESIAN_POINT('',(7.9,2.1,-3.31)) ;
#118753=CARTESIAN_POINT('',(1.4,2.1,-3.31)) ;
#118754=CARTESIAN_POINT('Origin',(7.9,2.1,-3.21)) ;
#118755=CARTESIAN_POINT('Origin',(1.4,2.4,-3.31)) ;
#118756=CARTESIAN_POINT('',(1.5,2.4,-3.31)) ;
#118757=CARTESIAN_POINT('',(1.5,2.4,-3.31)) ;
#118758=CARTESIAN_POINT('',(7.9,2.4,-3.31)) ;
#118759=CARTESIAN_POINT('',(1.4,2.4,-3.31)) ;
#118760=CARTESIAN_POINT('',(7.9,2.1,-3.31)) ;
#118761=CARTESIAN_POINT('Origin',(1.4,2.4,-3.21)) ;
#118762=CARTESIAN_POINT('',(1.5,2.5,-3.21)) ;
#118763=CARTESIAN_POINT('Origin',(1.5,2.4,-3.21)) ;
#118764=CARTESIAN_POINT('',(7.9,2.5,-3.21)) ;
#118765=CARTESIAN_POINT('',(1.4,2.5,-3.21)) ;
#118766=CARTESIAN_POINT('Origin',(7.9,2.4,-3.21)) ;
#118767=CARTESIAN_POINT('Origin',(1.4,2.5,-3.10142135623731)) ;
#118768=CARTESIAN_POINT('',(1.5,2.5,-3.10142135623731)) ;
#118769=CARTESIAN_POINT('',(1.5,2.5,-3.10142135623731)) ;
#118770=CARTESIAN_POINT('',(7.9,2.5,-3.10142135623731)) ;
#118771=CARTESIAN_POINT('',(1.4,2.5,-3.10142135623731)) ;
#118772=CARTESIAN_POINT('',(7.9,2.5,-3.21)) ;
#118773=CARTESIAN_POINT('Origin',(1.4,2.6,-3.10142135623731)) ;
#118774=CARTESIAN_POINT('',(1.5,2.52928932188135,-3.03071067811866)) ;
#118775=CARTESIAN_POINT('Origin',(1.5,2.6,-3.10142135623731)) ;
#118776=CARTESIAN_POINT('',(7.9,2.52928932188135,-3.03071067811866)) ;
#118777=CARTESIAN_POINT('',(1.4,2.52928932188135,-3.03071067811866)) ;
#118778=CARTESIAN_POINT('Origin',(7.9,2.6,-3.10142135623731)) ;
#118779=CARTESIAN_POINT('Origin',(1.4,3.07928932188135,-2.48071067811865)) ;
#118780=CARTESIAN_POINT('',(1.5,3.07928932188135,-2.48071067811865)) ;
#118781=CARTESIAN_POINT('',(7.9,3.07928932188135,-2.48071067811865)) ;
#118782=CARTESIAN_POINT('',(1.4,3.07928932188135,-2.48071067811865)) ;
#118783=CARTESIAN_POINT('',(7.9,2.52928932188135,-3.03071067811866)) ;
#118784=CARTESIAN_POINT('Origin',(1.4,3.15,-2.55142135623731)) ;
#118785=CARTESIAN_POINT('',(7.9,3.25,-2.55142135623731)) ;
#118786=CARTESIAN_POINT('',(1.4,3.25,-2.55142135623731)) ;
#118787=CARTESIAN_POINT('Origin',(7.9,3.15,-2.55142135623731)) ;
#118788=CARTESIAN_POINT('Origin',(1.4,3.25,-5.06857864376269)) ;
#118789=CARTESIAN_POINT('',(1.5,3.25,-5.06857864376269)) ;
#118790=CARTESIAN_POINT('',(7.9,3.25,-2.55142135623731)) ;
#118791=CARTESIAN_POINT('Origin',(1.4,2.52928932188134,-4.58928932188135)) ;
#118792=CARTESIAN_POINT('',(1.5,2.52928932188134,-4.58928932188135)) ;
#118793=CARTESIAN_POINT('',(1.5,2.52928932188134,-4.58928932188135)) ;
#118794=CARTESIAN_POINT('',(7.9,2.52928932188134,-4.58928932188135)) ;
#118795=CARTESIAN_POINT('',(1.4,2.52928932188134,-4.58928932188135)) ;
#118796=CARTESIAN_POINT('',(7.9,3.07928932188135,-5.13928932188135)) ;
#118797=CARTESIAN_POINT('Origin',(1.4,2.6,-4.51857864376269)) ;
#118798=CARTESIAN_POINT('',(1.5,2.5,-4.51857864376269)) ;
#118799=CARTESIAN_POINT('Origin',(1.5,2.6,-4.51857864376269)) ;
#118800=CARTESIAN_POINT('',(7.9,2.5,-4.51857864376269)) ;
#118801=CARTESIAN_POINT('',(1.4,2.5,-4.51857864376269)) ;
#118802=CARTESIAN_POINT('Origin',(7.9,2.6,-4.51857864376269)) ;
#118803=CARTESIAN_POINT('Origin',(1.4,2.5,-4.41)) ;
#118804=CARTESIAN_POINT('',(1.5,2.5,-4.41)) ;
#118805=CARTESIAN_POINT('',(1.5,2.5,-4.41)) ;
#118806=CARTESIAN_POINT('',(7.9,2.5,-4.41)) ;
#118807=CARTESIAN_POINT('',(1.4,2.5,-4.41)) ;
#118808=CARTESIAN_POINT('',(7.9,2.5,-4.51857864376269)) ;
#118809=CARTESIAN_POINT('Origin',(1.4,2.4,-4.41)) ;
#118810=CARTESIAN_POINT('',(1.5,2.4,-4.31)) ;
#118811=CARTESIAN_POINT('Origin',(1.5,2.4,-4.41)) ;
#118812=CARTESIAN_POINT('',(7.9,2.4,-4.31)) ;
#118813=CARTESIAN_POINT('',(1.4,2.4,-4.31)) ;
#118814=CARTESIAN_POINT('Origin',(7.9,2.4,-4.41)) ;
#118815=CARTESIAN_POINT('Origin',(1.4,2.1,-4.31)) ;
#118816=CARTESIAN_POINT('',(1.5,2.1,-4.31)) ;
#118817=CARTESIAN_POINT('',(1.5,2.1,-4.31)) ;
#118818=CARTESIAN_POINT('',(7.9,2.1,-4.31)) ;
#118819=CARTESIAN_POINT('',(1.4,2.1,-4.31)) ;
#118820=CARTESIAN_POINT('',(7.9,2.4,-4.31)) ;
#118821=CARTESIAN_POINT('Origin',(1.4,2.1,-4.41)) ;
#118822=CARTESIAN_POINT('',(1.5,2.,-4.41)) ;
#118823=CARTESIAN_POINT('Origin',(1.5,2.1,-4.41)) ;
#118824=CARTESIAN_POINT('',(7.9,2.,-4.41)) ;
#118825=CARTESIAN_POINT('',(1.4,2.,-4.41)) ;
#118826=CARTESIAN_POINT('Origin',(7.9,2.1,-4.41)) ;
#118827=CARTESIAN_POINT('Origin',(1.4,2.,-4.41)) ;
#118828=CARTESIAN_POINT('',(1.5,2.,-5.36)) ;
#118829=CARTESIAN_POINT('',(1.5,2.,-5.36)) ;
#118830=CARTESIAN_POINT('',(7.9,2.,-5.36)) ;
#118831=CARTESIAN_POINT('',(1.4,2.,-5.36)) ;
#118832=CARTESIAN_POINT('',(7.9,2.,-4.41)) ;
#118833=CARTESIAN_POINT('Origin',(1.4,1.9,-5.36)) ;
#118834=CARTESIAN_POINT('',(1.5,1.9,-5.46)) ;
#118835=CARTESIAN_POINT('Origin',(1.5,1.9,-5.36)) ;
#118836=CARTESIAN_POINT('',(7.9,1.9,-5.46)) ;
#118837=CARTESIAN_POINT('',(1.4,1.9,-5.46)) ;
#118838=CARTESIAN_POINT('Origin',(7.9,1.9,-5.36)) ;
#118839=CARTESIAN_POINT('Origin',(1.4,1.9,-5.46)) ;
#118840=CARTESIAN_POINT('',(1.5,-2.15,-5.46)) ;
#118841=CARTESIAN_POINT('',(1.5,-2.15,-5.46)) ;
#118842=CARTESIAN_POINT('',(7.9,-2.15,-5.46)) ;
#118843=CARTESIAN_POINT('',(1.4,-2.15,-5.46)) ;
#118844=CARTESIAN_POINT('',(7.9,1.9,-5.46)) ;
#118845=CARTESIAN_POINT('Origin',(1.4,-2.15,-5.36)) ;
#118846=CARTESIAN_POINT('',(1.5,-2.25,-5.36)) ;
#118847=CARTESIAN_POINT('Origin',(1.5,-2.15,-5.36)) ;
#118848=CARTESIAN_POINT('',(7.9,-2.25,-5.36)) ;
#118849=CARTESIAN_POINT('',(1.4,-2.25,-5.36)) ;
#118850=CARTESIAN_POINT('Origin',(7.9,-2.15,-5.36)) ;
#118851=CARTESIAN_POINT('Origin',(1.4,-2.25,-4.71311959340942)) ;
#118852=CARTESIAN_POINT('',(1.5,-2.25,-4.71311959340942)) ;
#118853=CARTESIAN_POINT('',(1.5,-2.25,-4.71311959340942)) ;
#118854=CARTESIAN_POINT('',(7.9,-2.25,-4.71311959340942)) ;
#118855=CARTESIAN_POINT('',(1.4,-2.25,-4.71311959340942)) ;
#118856=CARTESIAN_POINT('',(7.9,-2.25,-5.36)) ;
#118857=CARTESIAN_POINT('Origin',(1.4,-2.15,-4.71311959340942)) ;
#118858=CARTESIAN_POINT('',(1.5,-2.23576512455516,-4.66169641371351)) ;
#118859=CARTESIAN_POINT('Origin',(1.5,-2.15,-4.71311959340942)) ;
#118860=CARTESIAN_POINT('',(7.9,-2.23576512455516,-4.66169641371351)) ;
#118861=CARTESIAN_POINT('',(1.4,-2.23576512455516,-4.66169641371351)) ;
#118862=CARTESIAN_POINT('Origin',(7.9,-2.15,-4.71311959340942)) ;
#118863=CARTESIAN_POINT('Origin',(1.4,-3.65625,-3.81)) ;
#118864=CARTESIAN_POINT('',(1.5,-2.23576512455516,-2.95830358628649)) ;
#118865=CARTESIAN_POINT('Origin',(1.5,-3.65625,-3.81)) ;
#118866=CARTESIAN_POINT('',(7.9,-2.23576512455516,-2.95830358628649)) ;
#118867=CARTESIAN_POINT('',(1.4,-2.23576512455516,-2.95830358628649)) ;
#118868=CARTESIAN_POINT('Origin',(7.9,-3.65625,-3.81)) ;
#118869=CARTESIAN_POINT('Origin',(1.4,-2.15,-2.90688040659058)) ;
#118870=CARTESIAN_POINT('',(1.5,-2.25,-2.90688040659058)) ;
#118871=CARTESIAN_POINT('Origin',(1.5,-2.15,-2.90688040659058)) ;
#118872=CARTESIAN_POINT('',(7.9,-2.25,-2.90688040659058)) ;
#118873=CARTESIAN_POINT('',(1.4,-2.25,-2.90688040659058)) ;
#118874=CARTESIAN_POINT('Origin',(7.9,-2.15,-2.90688040659058)) ;
#118875=CARTESIAN_POINT('Origin',(1.4,-2.25,-2.26)) ;
#118876=CARTESIAN_POINT('',(1.5,-2.25,-2.26)) ;
#118877=CARTESIAN_POINT('',(1.5,-2.25,-2.26)) ;
#118878=CARTESIAN_POINT('',(7.9,-2.25,-2.26)) ;
#118879=CARTESIAN_POINT('',(1.4,-2.25,-2.26)) ;
#118880=CARTESIAN_POINT('',(7.9,-2.25,-2.90688040659058)) ;
#118881=CARTESIAN_POINT('Origin',(1.4,-2.15,-2.26)) ;
#118882=CARTESIAN_POINT('',(1.5,-2.15,-2.16)) ;
#118883=CARTESIAN_POINT('Origin',(1.5,-2.15,-2.26)) ;
#118884=CARTESIAN_POINT('',(7.9,-2.15,-2.16)) ;
#118885=CARTESIAN_POINT('',(1.4,-2.15,-2.16)) ;
#118886=CARTESIAN_POINT('Origin',(7.9,-2.15,-2.26)) ;
#118887=CARTESIAN_POINT('Origin',(1.4,1.9,-2.16)) ;
#118888=CARTESIAN_POINT('',(1.5,1.9,-2.16)) ;
#118889=CARTESIAN_POINT('',(1.5,1.9,-2.16)) ;
#118890=CARTESIAN_POINT('',(7.9,1.9,-2.16)) ;
#118891=CARTESIAN_POINT('',(1.4,1.9,-2.16)) ;
#118892=CARTESIAN_POINT('',(7.9,-2.15,-2.16)) ;
#118893=CARTESIAN_POINT('Origin',(1.4,1.9,-2.26)) ;
#118894=CARTESIAN_POINT('',(1.5,2.,-2.26)) ;
#118895=CARTESIAN_POINT('Origin',(1.5,1.9,-2.26)) ;
#118896=CARTESIAN_POINT('',(7.9,2.,-2.26)) ;
#118897=CARTESIAN_POINT('',(1.4,2.,-2.26)) ;
#118898=CARTESIAN_POINT('Origin',(7.9,1.9,-2.26)) ;
#118899=CARTESIAN_POINT('Origin',(1.4,2.,-2.26)) ;
#118900=CARTESIAN_POINT('',(1.5,2.,-3.21)) ;
#118901=CARTESIAN_POINT('',(7.9,2.,-2.26)) ;
#118902=CARTESIAN_POINT('Origin',(1.4,2.1,-3.21)) ;
#118903=CARTESIAN_POINT('',(1.4,2.6,-3.21)) ;
#118904=CARTESIAN_POINT('',(1.4,2.4,-3.41)) ;
#118905=CARTESIAN_POINT('Origin',(1.4,2.4,-3.21)) ;
#118906=CARTESIAN_POINT('',(1.4,2.1,-3.41)) ;
#118907=CARTESIAN_POINT('',(1.4,2.1,-3.41)) ;
#118908=CARTESIAN_POINT('',(1.4,1.9,-3.21)) ;
#118909=CARTESIAN_POINT('Origin',(1.4,2.1,-3.21)) ;
#118910=CARTESIAN_POINT('',(1.4,1.9,-2.26)) ;
#118911=CARTESIAN_POINT('',(1.4,1.9,-2.26)) ;
#118912=CARTESIAN_POINT('',(1.4,-2.15,-2.26)) ;
#118913=CARTESIAN_POINT('',(1.4,-2.15,-2.26)) ;
#118914=CARTESIAN_POINT('',(1.4,-2.15,-2.90688040659058)) ;
#118915=CARTESIAN_POINT('',(1.4,-2.15,-2.90688040659058)) ;
#118916=CARTESIAN_POINT('',(1.4,-2.15,-4.71311959340942)) ;
#118917=CARTESIAN_POINT('Origin',(1.4,-3.65625,-3.81)) ;
#118918=CARTESIAN_POINT('',(1.4,-2.15,-5.36)) ;
#118919=CARTESIAN_POINT('',(1.4,-2.15,-5.36)) ;
#118920=CARTESIAN_POINT('',(1.4,1.9,-5.36)) ;
#118921=CARTESIAN_POINT('',(1.4,1.9,-5.36)) ;
#118922=CARTESIAN_POINT('',(1.4,1.9,-4.41)) ;
#118923=CARTESIAN_POINT('',(1.4,1.9,-4.41)) ;
#118924=CARTESIAN_POINT('',(1.4,2.1,-4.21)) ;
#118925=CARTESIAN_POINT('Origin',(1.4,2.1,-4.41)) ;
#118926=CARTESIAN_POINT('',(1.4,2.4,-4.21)) ;
#118927=CARTESIAN_POINT('',(1.4,2.4,-4.21)) ;
#118928=CARTESIAN_POINT('',(1.4,2.6,-4.41)) ;
#118929=CARTESIAN_POINT('Origin',(1.4,2.4,-4.41)) ;
#118930=CARTESIAN_POINT('',(1.4,2.6,-4.51857864376269)) ;
#118931=CARTESIAN_POINT('',(1.4,2.6,-4.51857864376269)) ;
#118932=CARTESIAN_POINT('',(1.4,3.15,-5.06857864376269)) ;
#118933=CARTESIAN_POINT('',(1.4,3.15,-5.06857864376269)) ;
#118934=CARTESIAN_POINT('',(1.4,3.15,-2.55142135623731)) ;
#118935=CARTESIAN_POINT('',(1.4,2.6,-3.10142135623731)) ;
#118936=CARTESIAN_POINT('',(1.4,2.6,-3.10142135623731)) ;
#118937=CARTESIAN_POINT('',(1.4,2.6,-3.21)) ;
#118938=CARTESIAN_POINT('Origin',(2.4,0.,-3.81)) ;
#118939=CARTESIAN_POINT('',(2.4,0.3,-3.41)) ;
#118940=CARTESIAN_POINT('',(2.4,-0.3,-3.41)) ;
#118941=CARTESIAN_POINT('',(2.4,0.,-3.41)) ;
#118942=CARTESIAN_POINT('',(2.4,0.4,-3.51)) ;
#118943=CARTESIAN_POINT('Origin',(2.4,0.3,-3.51)) ;
#118944=CARTESIAN_POINT('',(2.4,0.4,-4.11)) ;
#118945=CARTESIAN_POINT('',(2.4,0.4,-3.81)) ;
#118946=CARTESIAN_POINT('',(2.4,0.3,-4.21)) ;
#118947=CARTESIAN_POINT('Origin',(2.4,0.3,-4.11)) ;
#118948=CARTESIAN_POINT('',(2.4,-0.3,-4.21)) ;
#118949=CARTESIAN_POINT('',(2.4,0.,-4.21)) ;
#118950=CARTESIAN_POINT('',(2.4,-0.4,-4.11)) ;
#118951=CARTESIAN_POINT('Origin',(2.4,-0.3,-4.11)) ;
#118952=CARTESIAN_POINT('',(2.4,-0.4,-3.51)) ;
#118953=CARTESIAN_POINT('',(2.4,-0.4,-3.81)) ;
#118954=CARTESIAN_POINT('Origin',(2.4,-0.3,-3.51)) ;
#118955=CARTESIAN_POINT('Origin',(2.4,0.,-7.62)) ;
#118956=CARTESIAN_POINT('',(2.4,0.3,-7.22)) ;
#118957=CARTESIAN_POINT('',(2.4,-0.3,-7.22)) ;
#118958=CARTESIAN_POINT('',(2.4,0.,-7.22)) ;
#118959=CARTESIAN_POINT('',(2.4,0.4,-7.32)) ;
#118960=CARTESIAN_POINT('Origin',(2.4,0.3,-7.32)) ;
#118961=CARTESIAN_POINT('',(2.4,0.4,-7.92)) ;
#118962=CARTESIAN_POINT('',(2.4,0.4,-7.62)) ;
#118963=CARTESIAN_POINT('',(2.4,0.3,-8.02)) ;
#118964=CARTESIAN_POINT('Origin',(2.4,0.3,-7.92)) ;
#118965=CARTESIAN_POINT('',(2.4,-0.3,-8.02)) ;
#118966=CARTESIAN_POINT('',(2.4,0.,-8.02)) ;
#118967=CARTESIAN_POINT('',(2.4,-0.4,-7.92)) ;
#118968=CARTESIAN_POINT('Origin',(2.4,-0.3,-7.92)) ;
#118969=CARTESIAN_POINT('',(2.4,-0.4,-7.32)) ;
#118970=CARTESIAN_POINT('',(2.4,-0.4,-7.62)) ;
#118971=CARTESIAN_POINT('Origin',(2.4,-0.3,-7.32)) ;
#118972=CARTESIAN_POINT('Origin',(2.4,0.,-11.43)) ;
#118973=CARTESIAN_POINT('',(2.4,0.3,-11.03)) ;
#118974=CARTESIAN_POINT('',(2.4,-0.3,-11.03)) ;
#118975=CARTESIAN_POINT('',(2.4,0.,-11.03)) ;
#118976=CARTESIAN_POINT('',(2.4,0.4,-11.13)) ;
#118977=CARTESIAN_POINT('Origin',(2.4,0.3,-11.13)) ;
#118978=CARTESIAN_POINT('',(2.4,0.4,-11.73)) ;
#118979=CARTESIAN_POINT('',(2.4,0.4,-11.43)) ;
#118980=CARTESIAN_POINT('',(2.4,0.3,-11.83)) ;
#118981=CARTESIAN_POINT('Origin',(2.4,0.3,-11.73)) ;
#118982=CARTESIAN_POINT('',(2.4,-0.3,-11.83)) ;
#118983=CARTESIAN_POINT('',(2.4,0.,-11.83)) ;
#118984=CARTESIAN_POINT('',(2.4,-0.4,-11.73)) ;
#118985=CARTESIAN_POINT('Origin',(2.4,-0.3,-11.73)) ;
#118986=CARTESIAN_POINT('',(2.4,-0.4,-11.13)) ;
#118987=CARTESIAN_POINT('',(2.4,-0.4,-11.43)) ;
#118988=CARTESIAN_POINT('Origin',(2.4,-0.3,-11.13)) ;
#118989=CARTESIAN_POINT('Origin',(2.4,0.,-15.24)) ;
#118990=CARTESIAN_POINT('',(2.4,0.3,-14.84)) ;
#118991=CARTESIAN_POINT('',(2.4,-0.3,-14.84)) ;
#118992=CARTESIAN_POINT('',(2.4,0.,-14.84)) ;
#118993=CARTESIAN_POINT('',(2.4,0.4,-14.94)) ;
#118994=CARTESIAN_POINT('Origin',(2.4,0.3,-14.94)) ;
#118995=CARTESIAN_POINT('',(2.4,0.4,-15.54)) ;
#118996=CARTESIAN_POINT('',(2.4,0.4,-15.24)) ;
#118997=CARTESIAN_POINT('',(2.4,0.3,-15.64)) ;
#118998=CARTESIAN_POINT('Origin',(2.4,0.3,-15.54)) ;
#118999=CARTESIAN_POINT('',(2.4,-0.3,-15.64)) ;
#119000=CARTESIAN_POINT('',(2.4,0.,-15.64)) ;
#119001=CARTESIAN_POINT('',(2.4,-0.4,-15.54)) ;
#119002=CARTESIAN_POINT('Origin',(2.4,-0.3,-15.54)) ;
#119003=CARTESIAN_POINT('',(2.4,-0.4,-14.94)) ;
#119004=CARTESIAN_POINT('',(2.4,-0.4,-15.24)) ;
#119005=CARTESIAN_POINT('Origin',(2.4,-0.3,-14.94)) ;
#119006=CARTESIAN_POINT('Origin',(2.4,0.,-19.05)) ;
#119007=CARTESIAN_POINT('',(2.4,0.3,-18.65)) ;
#119008=CARTESIAN_POINT('',(2.4,-0.3,-18.65)) ;
#119009=CARTESIAN_POINT('',(2.4,0.,-18.65)) ;
#119010=CARTESIAN_POINT('',(2.4,0.4,-18.75)) ;
#119011=CARTESIAN_POINT('Origin',(2.4,0.3,-18.75)) ;
#119012=CARTESIAN_POINT('',(2.4,0.4,-19.35)) ;
#119013=CARTESIAN_POINT('',(2.4,0.4,-19.05)) ;
#119014=CARTESIAN_POINT('',(2.4,0.3,-19.45)) ;
#119015=CARTESIAN_POINT('Origin',(2.4,0.3,-19.35)) ;
#119016=CARTESIAN_POINT('',(2.4,-0.3,-19.45)) ;
#119017=CARTESIAN_POINT('',(2.4,0.,-19.45)) ;
#119018=CARTESIAN_POINT('',(2.4,-0.4,-19.35)) ;
#119019=CARTESIAN_POINT('Origin',(2.4,-0.3,-19.35)) ;
#119020=CARTESIAN_POINT('',(2.4,-0.4,-18.75)) ;
#119021=CARTESIAN_POINT('',(2.4,-0.4,-19.05)) ;
#119022=CARTESIAN_POINT('Origin',(2.4,-0.3,-18.75)) ;
#119023=CARTESIAN_POINT('Origin',(2.4,0.,-22.86)) ;
#119024=CARTESIAN_POINT('',(2.4,0.3,-22.46)) ;
#119025=CARTESIAN_POINT('',(2.4,-0.3,-22.46)) ;
#119026=CARTESIAN_POINT('',(2.4,0.,-22.46)) ;
#119027=CARTESIAN_POINT('',(2.4,0.4,-22.56)) ;
#119028=CARTESIAN_POINT('Origin',(2.4,0.3,-22.56)) ;
#119029=CARTESIAN_POINT('',(2.4,0.4,-23.16)) ;
#119030=CARTESIAN_POINT('',(2.4,0.4,-22.86)) ;
#119031=CARTESIAN_POINT('',(2.4,0.3,-23.26)) ;
#119032=CARTESIAN_POINT('Origin',(2.4,0.3,-23.16)) ;
#119033=CARTESIAN_POINT('',(2.4,-0.3,-23.26)) ;
#119034=CARTESIAN_POINT('',(2.4,0.,-23.26)) ;
#119035=CARTESIAN_POINT('',(2.4,-0.4,-23.16)) ;
#119036=CARTESIAN_POINT('Origin',(2.4,-0.3,-23.16)) ;
#119037=CARTESIAN_POINT('',(2.4,-0.4,-22.56)) ;
#119038=CARTESIAN_POINT('',(2.4,-0.4,-22.86)) ;
#119039=CARTESIAN_POINT('Origin',(2.4,-0.3,-22.56)) ;
#119040=CARTESIAN_POINT('Origin',(2.4,0.,-26.67)) ;
#119041=CARTESIAN_POINT('',(2.4,0.3,-26.27)) ;
#119042=CARTESIAN_POINT('',(2.4,-0.3,-26.27)) ;
#119043=CARTESIAN_POINT('',(2.4,0.,-26.27)) ;
#119044=CARTESIAN_POINT('',(2.4,0.4,-26.37)) ;
#119045=CARTESIAN_POINT('Origin',(2.4,0.3,-26.37)) ;
#119046=CARTESIAN_POINT('',(2.4,0.4,-26.97)) ;
#119047=CARTESIAN_POINT('',(2.4,0.4,-26.67)) ;
#119048=CARTESIAN_POINT('',(2.4,0.3,-27.07)) ;
#119049=CARTESIAN_POINT('Origin',(2.4,0.3,-26.97)) ;
#119050=CARTESIAN_POINT('',(2.4,-0.3,-27.07)) ;
#119051=CARTESIAN_POINT('',(2.4,0.,-27.07)) ;
#119052=CARTESIAN_POINT('',(2.4,-0.4,-26.97)) ;
#119053=CARTESIAN_POINT('Origin',(2.4,-0.3,-26.97)) ;
#119054=CARTESIAN_POINT('',(2.4,-0.4,-26.37)) ;
#119055=CARTESIAN_POINT('',(2.4,-0.4,-26.67)) ;
#119056=CARTESIAN_POINT('Origin',(2.4,-0.3,-26.37)) ;
#119057=CARTESIAN_POINT('Origin',(2.4,0.,-30.48)) ;
#119058=CARTESIAN_POINT('',(2.4,0.3,-30.08)) ;
#119059=CARTESIAN_POINT('',(2.4,-0.3,-30.08)) ;
#119060=CARTESIAN_POINT('',(2.4,0.,-30.08)) ;
#119061=CARTESIAN_POINT('',(2.4,0.4,-30.18)) ;
#119062=CARTESIAN_POINT('Origin',(2.4,0.3,-30.18)) ;
#119063=CARTESIAN_POINT('',(2.4,0.4,-30.78)) ;
#119064=CARTESIAN_POINT('',(2.4,0.4,-30.48)) ;
#119065=CARTESIAN_POINT('',(2.4,0.3,-30.88)) ;
#119066=CARTESIAN_POINT('Origin',(2.4,0.3,-30.78)) ;
#119067=CARTESIAN_POINT('',(2.4,-0.3,-30.88)) ;
#119068=CARTESIAN_POINT('',(2.4,0.,-30.88)) ;
#119069=CARTESIAN_POINT('',(2.4,-0.4,-30.78)) ;
#119070=CARTESIAN_POINT('Origin',(2.4,-0.3,-30.78)) ;
#119071=CARTESIAN_POINT('',(2.4,-0.4,-30.18)) ;
#119072=CARTESIAN_POINT('',(2.4,-0.4,-30.48)) ;
#119073=CARTESIAN_POINT('Origin',(2.4,-0.3,-30.18)) ;
#119074=CARTESIAN_POINT('Origin',(2.4,0.,-34.29)) ;
#119075=CARTESIAN_POINT('',(2.4,0.3,-33.89)) ;
#119076=CARTESIAN_POINT('',(2.4,-0.3,-33.89)) ;
#119077=CARTESIAN_POINT('',(2.4,0.,-33.89)) ;
#119078=CARTESIAN_POINT('',(2.4,0.4,-33.99)) ;
#119079=CARTESIAN_POINT('Origin',(2.4,0.3,-33.99)) ;
#119080=CARTESIAN_POINT('',(2.4,0.4,-34.59)) ;
#119081=CARTESIAN_POINT('',(2.4,0.4,-34.29)) ;
#119082=CARTESIAN_POINT('',(2.4,0.3,-34.69)) ;
#119083=CARTESIAN_POINT('Origin',(2.4,0.3,-34.59)) ;
#119084=CARTESIAN_POINT('',(2.4,-0.3,-34.69)) ;
#119085=CARTESIAN_POINT('',(2.4,0.,-34.69)) ;
#119086=CARTESIAN_POINT('',(2.4,-0.4,-34.59)) ;
#119087=CARTESIAN_POINT('Origin',(2.4,-0.3,-34.59)) ;
#119088=CARTESIAN_POINT('',(2.4,-0.4,-33.99)) ;
#119089=CARTESIAN_POINT('',(2.4,-0.4,-34.29)) ;
#119090=CARTESIAN_POINT('Origin',(2.4,-0.3,-33.99)) ;
#119091=CARTESIAN_POINT('Origin',(-0.899999999999999,-2.,-3.21)) ;
#119092=CARTESIAN_POINT('Origin',(-0.899999999999999,0.4,-3.21)) ;
#119093=CARTESIAN_POINT('Origin',(-0.899999999999999,-1.9,-3.21)) ;
#119094=CARTESIAN_POINT('Origin',(0.600000000000001,0.4,-3.41)) ;
#119095=CARTESIAN_POINT('Origin',(0.500000000000001,0.4,-3.41)) ;
#119096=CARTESIAN_POINT('Origin',(-0.899999999999999,0.4,-3.41)) ;
#119097=CARTESIAN_POINT('Origin',(0.500000000000001,0.4,-3.41)) ;
#119098=CARTESIAN_POINT('',(0.600000000000001,0.4,-3.41)) ;
#119099=CARTESIAN_POINT('Origin',(0.500000000000001,0.4,-3.41)) ;
#119100=CARTESIAN_POINT('Origin',(0.500000000000001,0.4,-3.41)) ;
#119101=CARTESIAN_POINT('Origin',(-0.899999999999999,-1.9,-3.21)) ;
#119102=CARTESIAN_POINT('Origin',(-0.899999999999999,-1.9,-3.21)) ;
#119103=CARTESIAN_POINT('Origin',(-0.899999999999999,-1.9,-3.21)) ;
#119104=CARTESIAN_POINT('Origin',(-0.899999999999999,0.4,-3.41)) ;
#119105=CARTESIAN_POINT('Origin',(-0.899999999999999,0.6,-3.41)) ;
#119106=CARTESIAN_POINT('Origin',(0.500000000000001,0.4,-3.81)) ;
#119107=CARTESIAN_POINT('Origin',(0.500000000000001,0.4,-4.21)) ;
#119108=CARTESIAN_POINT('',(0.600000000000001,0.4,-4.11)) ;
#119109=CARTESIAN_POINT('Ctrl Pts',(0.595612997216081,0.370705721320404,
-4.1807057213204)) ;
#119110=CARTESIAN_POINT('Ctrl Pts',(0.596180587760892,0.372558268494358,
-4.17885549883217)) ;
#119111=CARTESIAN_POINT('Ctrl Pts',(0.596672461925686,0.374355839771985,
-4.17691417986631)) ;
#119112=CARTESIAN_POINT('Ctrl Pts',(0.599015141889212,0.383869350930066,
-4.16576499365627)) ;
#119113=CARTESIAN_POINT('Ctrl Pts',(0.599609996542525,0.390224332900452,
-4.15497260265412)) ;
#119114=CARTESIAN_POINT('Ctrl Pts',(0.600050586298726,0.398117439141561,
-4.13233105320467)) ;
#119115=CARTESIAN_POINT('Ctrl Pts',(0.600000000000001,0.399999999999999,
-4.12120125063352)) ;
#119116=CARTESIAN_POINT('Ctrl Pts',(0.600000000000001,0.399999999999999,
-4.11)) ;
#119117=CARTESIAN_POINT('',(0.600000000000001,0.4,-3.81)) ;
#119118=CARTESIAN_POINT('Origin',(0.500000000000001,-4.56640444411541E-17,
-3.41)) ;
#119119=CARTESIAN_POINT('',(0.500000000000001,0.394987437106619,-3.51)) ;
#119120=CARTESIAN_POINT('Ctrl Pts',(0.500000000000001,0.394987437106619,
-3.51)) ;
#119121=CARTESIAN_POINT('Ctrl Pts',(0.505940567948953,0.3955844866499,-3.51)) ;
#119122=CARTESIAN_POINT('Ctrl Pts',(0.511931971019142,0.396132036079018,
-3.50946630032796)) ;
#119123=CARTESIAN_POINT('Ctrl Pts',(0.517829015308552,0.396618246075354,
-3.50839779577372)) ;
#119124=CARTESIAN_POINT('Ctrl Pts',(0.522982218721203,0.397043126556053,
-3.50746407015711)) ;
#119125=CARTESIAN_POINT('Ctrl Pts',(0.528062648970231,0.397421319341388,
-3.50612282679706)) ;
#119126=CARTESIAN_POINT('Ctrl Pts',(0.532978106724,0.397751505046071,-3.50440574387663)) ;
#119127=CARTESIAN_POINT('Ctrl Pts',(0.538583536338964,0.398128038182999,
-3.50244763784955)) ;
#119128=CARTESIAN_POINT('Ctrl Pts',(0.544059405914891,0.398447721828295,
-3.49997000831105)) ;
#119129=CARTESIAN_POINT('Ctrl Pts',(0.549268572255782,0.398712331108983,
-3.49702073194289)) ;
#119130=CARTESIAN_POINT('Ctrl Pts',(0.553856850427147,0.398945401221756,
-3.49442298414684)) ;
#119131=CARTESIAN_POINT('Ctrl Pts',(0.558237825069328,0.399135987683843,
-3.49146038497999)) ;
#119132=CARTESIAN_POINT('Ctrl Pts',(0.562333836086213,0.399290378266507,
-3.48819522286417)) ;
#119133=CARTESIAN_POINT('Ctrl Pts',(0.56699032895789,0.399465895042381,
-3.48448326895231)) ;
#119134=CARTESIAN_POINT('Ctrl Pts',(0.571349096493424,0.399597278936107,
-3.4803228064848)) ;
#119135=CARTESIAN_POINT('Ctrl Pts',(0.57529692005671,0.399694832180837,
-3.47580557597935)) ;
#119136=CARTESIAN_POINT('Ctrl Pts',(0.578744263667905,0.399780018245913,
-3.47186101121508)) ;
#119137=CARTESIAN_POINT('Ctrl Pts',(0.581878314560428,0.399839626289636,
-3.46764552184211)) ;
#119138=CARTESIAN_POINT('Ctrl Pts',(0.584648147334855,0.399882153365958,
-3.4632418177073)) ;
#119139=CARTESIAN_POINT('Ctrl Pts',(0.587839270208174,0.399931148788079,
-3.4581683125045)) ;
#119140=CARTESIAN_POINT('Ctrl Pts',(0.590595054415095,0.399958289583404,
-3.45276663624445)) ;
#119141=CARTESIAN_POINT('Ctrl Pts',(0.592838618943107,0.399974357003159,
-3.44716168500939)) ;
#119142=CARTESIAN_POINT('Ctrl Pts',(0.594777336851657,0.399988241245861,
-3.44231831224239)) ;
#119143=CARTESIAN_POINT('Ctrl Pts',(0.59633405150619,0.399993946552814,
-3.43732416622712)) ;
#119144=CARTESIAN_POINT('Ctrl Pts',(0.597488309822309,0.39999684570125,
-3.43227171856839)) ;
#119145=CARTESIAN_POINT('Ctrl Pts',(0.598804024094397,0.400000150378306,
-3.42651254196058)) ;
#119146=CARTESIAN_POINT('Ctrl Pts',(0.599612685195426,0.399999963509465,
-3.42060284389063)) ;
#119147=CARTESIAN_POINT('Ctrl Pts',(0.599890230999718,0.399999993975383,
-3.41468420226113)) ;
#119148=CARTESIAN_POINT('Ctrl Pts',(0.599963464549399,0.400000002014155,
-3.41312250278986)) ;
#119149=CARTESIAN_POINT('Ctrl Pts',(0.600000000000001,0.399999999999999,
-3.4115602215092)) ;
#119150=CARTESIAN_POINT('Ctrl Pts',(0.600000000000001,0.399999999999999,
-3.41)) ;
#119151=CARTESIAN_POINT('',(0.600000000000001,0.299999999999999,-3.41)) ;
#119152=CARTESIAN_POINT('Ctrl Pts',(0.500000000000001,0.394987437106619,
-3.51)) ;
#119153=CARTESIAN_POINT('Ctrl Pts',(0.500454935589683,0.395033159853733,
-3.51)) ;
#119154=CARTESIAN_POINT('Ctrl Pts',(0.500909898680391,0.395078570329052,
-3.50999689549113)) ;
#119155=CARTESIAN_POINT('Ctrl Pts',(0.502892456245154,0.395275075889088,
-3.50996983394194)) ;
#119156=CARTESIAN_POINT('Ctrl Pts',(0.504418747482365,0.395422812032198,
-3.50991398542099)) ;
#119157=CARTESIAN_POINT('Ctrl Pts',(0.508462199543374,0.395804395682036,
-3.50967328105664)) ;
#119158=CARTESIAN_POINT('Ctrl Pts',(0.51097495334332,0.396031485023319,
-3.50942793914505)) ;
#119159=CARTESIAN_POINT('Ctrl Pts',(0.521160739721337,0.396903453186241,
-3.50804279449155)) ;
#119160=CARTESIAN_POINT('Ctrl Pts',(0.528708678528462,0.397444933153163,
-3.50610421770467)) ;
#119161=CARTESIAN_POINT('Ctrl Pts',(0.545943206358151,0.398105551684111,
-3.49946463945111)) ;
#119162=CARTESIAN_POINT('Ctrl Pts',(0.555229535466881,0.397987646678422,
-3.49403535883592)) ;
#119163=CARTESIAN_POINT('Ctrl Pts',(0.571394604995817,0.395490482808027,
-3.4807755133638)) ;
#119164=CARTESIAN_POINT('Ctrl Pts',(0.578055313702888,0.393198948698317,
-3.47324074563169)) ;
#119165=CARTESIAN_POINT('Ctrl Pts',(0.588559132202554,0.385442756729274,
-3.45739223398396)) ;
#119166=CARTESIAN_POINT('Ctrl Pts',(0.592167355639999,0.380240075126842,
-3.44954826560675)) ;
#119167=CARTESIAN_POINT('Ctrl Pts',(0.597496615531132,0.365892753466902,
-3.43392552179521)) ;
#119168=CARTESIAN_POINT('Ctrl Pts',(0.598734255154207,0.35666056430058,
-3.42677274172686)) ;
#119169=CARTESIAN_POINT('Ctrl Pts',(0.600012754681691,0.335223914398476,
-3.41558230586558)) ;
#119170=CARTESIAN_POINT('Ctrl Pts',(0.59999390055981,0.322655037091807,
-3.41166151936557)) ;
#119171=CARTESIAN_POINT('Ctrl Pts',(0.600000296204999,0.306106913582338,
-3.41013962634704)) ;
#119172=CARTESIAN_POINT('Ctrl Pts',(0.600000000000001,0.303050992413427,
-3.41)) ;
#119173=CARTESIAN_POINT('Ctrl Pts',(0.600000000000001,0.299999999999999,
-3.41)) ;
#119174=CARTESIAN_POINT('',(0.600000000000001,-2.3980000991444E-17,-3.41)) ;
#119175=CARTESIAN_POINT('Origin',(0.500000000000001,-1.9,-3.41)) ;
#119176=CARTESIAN_POINT('Origin',(0.600000000000001,-1.9,-3.21)) ;
#119177=CARTESIAN_POINT('Origin',(0.500000000000001,-1.9,-3.21)) ;
#119178=CARTESIAN_POINT('Origin',(-0.899999999999999,-1.9,-2.435)) ;
#119179=CARTESIAN_POINT('Origin',(-0.899999999999999,-1.9,-2.535)) ;
#119180=CARTESIAN_POINT('Origin',(-0.899999999999999,0.6,-3.31)) ;
#119181=CARTESIAN_POINT('Origin',(-0.899999999999999,0.6,-4.21)) ;
#119182=CARTESIAN_POINT('Origin',(0.600000000000001,0.4,-4.21)) ;
#119183=CARTESIAN_POINT('Origin',(0.500000000000001,0.4,-4.21)) ;
#119184=CARTESIAN_POINT('Origin',(-0.899999999999999,0.4,-4.21)) ;
#119185=CARTESIAN_POINT('Origin',(0.500000000000001,0.4,-4.21)) ;
#119186=CARTESIAN_POINT('Origin',(0.500000000000001,-1.9,-3.21)) ;
#119187=CARTESIAN_POINT('Origin',(0.500000000000001,-2.1,-3.21)) ;
#119188=CARTESIAN_POINT('Origin',(-0.899999999999999,-1.9,-2.535)) ;
#119189=CARTESIAN_POINT('Origin',(-1.1,-1.9,-2.535)) ;
#119190=CARTESIAN_POINT('Origin',(-0.899999999999999,-2.1,-2.535)) ;
#119191=CARTESIAN_POINT('Origin',(-0.899999999999999,0.4,-4.21)) ;
#119192=CARTESIAN_POINT('Origin',(-0.899999999999999,0.4,-4.41)) ;
#119193=CARTESIAN_POINT('Origin',(0.500000000000001,-2.1,-3.81)) ;
#119194=CARTESIAN_POINT('Origin',(0.500000000000001,-2.1,-2.535)) ;
#119195=CARTESIAN_POINT('Origin',(0.600000000000001,-2.1,-2.535)) ;
#119196=CARTESIAN_POINT('Origin',(0.500000000000001,-2.1,-2.535)) ;
#119197=CARTESIAN_POINT('Origin',(-1.1,-4.42727195005761E-17,-2.535)) ;
#119198=CARTESIAN_POINT('',(-1.1,1.15,-2.435)) ;
#119199=CARTESIAN_POINT('',(-1.1,1.25,-2.435)) ;
#119200=CARTESIAN_POINT('Origin',(-1.1,1.15,-2.535)) ;
#119201=CARTESIAN_POINT('Origin',(-0.899999999999999,0.5,-4.41)) ;
#119202=CARTESIAN_POINT('Origin',(-0.899999999999999,-1.9,-4.41)) ;
#119203=CARTESIAN_POINT('Origin',(0.600000000000001,-1.9,-4.41)) ;
#119204=CARTESIAN_POINT('Origin',(0.500000000000001,-1.9,-4.41)) ;
#119205=CARTESIAN_POINT('Origin',(-0.899999999999999,-1.9,-4.41)) ;
#119206=CARTESIAN_POINT('Origin',(0.500000000000001,-1.9,-4.41)) ;
#119207=CARTESIAN_POINT('Origin',(0.500000000000001,-2.1,-4.41)) ;
#119208=CARTESIAN_POINT('Origin',(0.500000000000001,-2.1,-2.535)) ;
#119209=CARTESIAN_POINT('Origin',(0.500000000000001,-2.1,-2.535)) ;
#119210=CARTESIAN_POINT('Origin',(-1.1,-2.9,-2.335)) ;
#119211=CARTESIAN_POINT('Origin',(-1.1,-2.9,-2.335)) ;
#119212=CARTESIAN_POINT('Origin',(-1.1,-2.9,-2.335)) ;
#119213=CARTESIAN_POINT('Origin',(-1.1,1.25,-2.335)) ;
#119214=CARTESIAN_POINT('Origin',(-1.1,1.15,-2.335)) ;
#119215=CARTESIAN_POINT('Origin',(-1.1,1.15,-2.535)) ;
#119216=CARTESIAN_POINT('',(-1.1,1.25,-2.535)) ;
#119217=CARTESIAN_POINT('Origin',(-1.1,1.15,-2.535)) ;
#119218=CARTESIAN_POINT('Origin',(-1.1,1.15,-2.535)) ;
#119219=CARTESIAN_POINT('Origin',(-0.899999999999999,-1.9,-4.41)) ;
#119220=CARTESIAN_POINT('Origin',(-0.899999999999999,-1.9,-4.41)) ;
#119221=CARTESIAN_POINT('Origin',(0.500000000000001,-2.1,-3.81)) ;
#119222=CARTESIAN_POINT('Origin',(0.500000000000001,-2.1,-5.085)) ;
#119223=CARTESIAN_POINT('Origin',(0.500000000000001,1.36481920536411E-16,
-2.535)) ;
#119224=CARTESIAN_POINT('Origin',(0.500000000000001,-2.9,-2.535)) ;
#119225=CARTESIAN_POINT('Origin',(-0.999999999999999,-2.9,-2.335)) ;
#119226=CARTESIAN_POINT('Origin',(0.500000000000001,-2.9,-2.335)) ;
#119227=CARTESIAN_POINT('Origin',(-1.1,1.15,-2.535)) ;
#119228=CARTESIAN_POINT('Origin',(-1.1,1.35,-2.535)) ;
#119229=CARTESIAN_POINT('Origin',(-1.1,1.15,-3.81)) ;
#119230=CARTESIAN_POINT('',(-1.1,1.25,-5.085)) ;
#119231=CARTESIAN_POINT('',(-1.1,1.25,-5.185)) ;
#119232=CARTESIAN_POINT('Origin',(-1.1,1.15,-5.085)) ;
#119233=CARTESIAN_POINT('Origin',(-0.899999999999999,-1.9,-4.31)) ;
#119234=CARTESIAN_POINT('Origin',(-0.899999999999999,-1.9,-5.085)) ;
#119235=CARTESIAN_POINT('Origin',(-0.999999999999999,-2.1,-5.085)) ;
#119236=CARTESIAN_POINT('Origin',(0.500000000000001,-2.1,-5.085)) ;
#119237=CARTESIAN_POINT('Origin',(-0.899999999999999,-2.1,-5.085)) ;
#119238=CARTESIAN_POINT('Origin',(0.500000000000001,-2.1,-5.085)) ;
#119239=CARTESIAN_POINT('Origin',(0.500000000000001,-2.1,-5.085)) ;
#119240=CARTESIAN_POINT('Origin',(0.500000000000001,-2.9,-2.535)) ;
#119241=CARTESIAN_POINT('Origin',(0.700000000000002,-2.9,-2.535)) ;
#119242=CARTESIAN_POINT('Origin',(-1.1,1.35,-5.185)) ;
#119243=CARTESIAN_POINT('Origin',(-1.1,1.35,-5.085)) ;
#119244=CARTESIAN_POINT('Origin',(-1.1,1.15,-5.085)) ;
#119245=CARTESIAN_POINT('',(-1.1,1.15,-5.185)) ;
#119246=CARTESIAN_POINT('Origin',(-1.1,1.15,-5.085)) ;
#119247=CARTESIAN_POINT('Origin',(-1.1,1.15,-5.085)) ;
#119248=CARTESIAN_POINT('Origin',(-0.899999999999999,-1.9,-5.085)) ;
#119249=CARTESIAN_POINT('Origin',(-1.1,-1.9,-5.085)) ;
#119250=CARTESIAN_POINT('Origin',(0.500000000000001,-5.86744705109801E-17,
-5.085)) ;
#119251=CARTESIAN_POINT('Origin',(0.500000000000001,-2.9,-5.085)) ;
#119252=CARTESIAN_POINT('Origin',(0.700000000000002,-2.9,-3.81)) ;
#119253=CARTESIAN_POINT('Origin',(0.700000000000002,-2.9,-5.085)) ;
#119254=CARTESIAN_POINT('Origin',(-1.1,1.15,-5.085)) ;
#119255=CARTESIAN_POINT('Origin',(-1.1,1.15,-5.285)) ;
#119256=CARTESIAN_POINT('Origin',(-1.1,-2.39429110547967E-16,-5.085)) ;
#119257=CARTESIAN_POINT('',(-1.1,1.25,-5.185)) ;
#119258=CARTESIAN_POINT('Origin',(0.500000000000001,-2.9,-5.085)) ;
#119259=CARTESIAN_POINT('Origin',(0.500000000000001,-2.9,-5.285)) ;
#119260=CARTESIAN_POINT('Origin',(-1.1,1.25,-5.285)) ;
#119261=CARTESIAN_POINT('Origin',(-1.1,-2.9,-5.285)) ;
#119262=CARTESIAN_POINT('Origin',(-1.1,-2.9,-5.285)) ;
#119263=CARTESIAN_POINT('Origin',(-1.1,-2.9,-5.285)) ;
#119264=CARTESIAN_POINT('Origin',(-1.1,-2.9,-5.285)) ;
#119265=CARTESIAN_POINT('Origin',(1.5,1.9,-3.21)) ;
#119266=CARTESIAN_POINT('Origin',(1.5,1.9,-5.36)) ;
#119267=CARTESIAN_POINT('Origin',(1.5,1.9,-4.41)) ;
#119268=CARTESIAN_POINT('Origin',(1.5,2.1,-4.41)) ;
#119269=CARTESIAN_POINT('Origin',(1.5,2.1,-4.21)) ;
#119270=CARTESIAN_POINT('Origin',(1.5,1.9,-5.36)) ;
#119271=CARTESIAN_POINT('Origin',(1.5,1.9,-5.36)) ;
#119272=CARTESIAN_POINT('Origin',(1.5,2.1,-4.21)) ;
#119273=CARTESIAN_POINT('Origin',(1.5,2.4,-4.21)) ;
#119274=CARTESIAN_POINT('Origin',(1.5,2.1,-5.36)) ;
#119275=CARTESIAN_POINT('Origin',(1.5,-2.15,-5.36)) ;
#119276=CARTESIAN_POINT('Origin',(1.5,2.4,-4.41)) ;
#119277=CARTESIAN_POINT('Origin',(1.5,2.6,-4.41)) ;
#119278=CARTESIAN_POINT('Origin',(1.5,-2.15,-5.36)) ;
#119279=CARTESIAN_POINT('Origin',(1.5,-2.15,-5.36)) ;
#119280=CARTESIAN_POINT('Origin',(1.5,2.6,-3.21)) ;
#119281=CARTESIAN_POINT('Origin',(1.5,2.6,-4.51857864376269)) ;
#119282=CARTESIAN_POINT('Origin',(1.5,-2.15,-3.21)) ;
#119283=CARTESIAN_POINT('Origin',(1.5,-2.15,-4.71311959340942)) ;
#119284=CARTESIAN_POINT('Origin',(1.5,2.6,-4.51857864376269)) ;
#119285=CARTESIAN_POINT('Origin',(1.5,2.6,-4.51857864376269)) ;
#119286=CARTESIAN_POINT('Origin',(1.5,-2.15,-4.71311959340942)) ;
#119287=CARTESIAN_POINT('Origin',(1.5,-2.15,-4.71311959340942)) ;
#119288=CARTESIAN_POINT('Origin',(1.5,1.69571067811865,-3.61428932188135)) ;
#119289=CARTESIAN_POINT('Origin',(1.5,3.15,-5.06857864376269)) ;
#119290=CARTESIAN_POINT('Origin',(1.5,-3.65625,-3.81)) ;
#119291=CARTESIAN_POINT('Origin',(1.5,-2.15,-2.90688040659058)) ;
#119292=CARTESIAN_POINT('Origin',(1.5,3.15,-5.06857864376269)) ;
#119293=CARTESIAN_POINT('Origin',(1.5,3.15,-5.06857864376269)) ;
#119294=CARTESIAN_POINT('Origin',(1.5,-2.15,-2.90688040659058)) ;
#119295=CARTESIAN_POINT('Origin',(1.5,-2.15,-2.90688040659058)) ;
#119296=CARTESIAN_POINT('Origin',(1.5,3.15,-3.21)) ;
#119297=CARTESIAN_POINT('Origin',(1.5,-2.15,-3.21)) ;
#119298=CARTESIAN_POINT('Origin',(1.5,-2.15,-2.26)) ;
#119299=CARTESIAN_POINT('Origin',(1.5,-2.15,-2.26)) ;
#119300=CARTESIAN_POINT('Origin',(1.5,-2.15,-2.26)) ;
#119301=CARTESIAN_POINT('Origin',(1.5,2.29571067811866,-3.40571067811866)) ;
#119302=CARTESIAN_POINT('Origin',(1.5,2.6,-3.10142135623731)) ;
#119303=CARTESIAN_POINT('Origin',(1.5,2.1,-2.26)) ;
#119304=CARTESIAN_POINT('Origin',(1.5,1.9,-2.26)) ;
#119305=CARTESIAN_POINT('Origin',(1.5,2.6,-3.10142135623731)) ;
#119306=CARTESIAN_POINT('Origin',(1.5,2.6,-3.10142135623731)) ;
#119307=CARTESIAN_POINT('Origin',(1.5,1.9,-2.26)) ;
#119308=CARTESIAN_POINT('Origin',(1.5,1.9,-2.26)) ;
#119309=CARTESIAN_POINT('Origin',(1.5,2.6,-3.21)) ;
#119310=CARTESIAN_POINT('Origin',(1.5,2.6,-3.21)) ;
#119311=CARTESIAN_POINT('Origin',(1.5,1.9,-3.21)) ;
#119312=CARTESIAN_POINT('Origin',(1.5,1.9,-3.21)) ;
#119313=CARTESIAN_POINT('Origin',(1.5,2.4,-3.21)) ;
#119314=CARTESIAN_POINT('Origin',(1.5,2.4,-3.41)) ;
#119315=CARTESIAN_POINT('Origin',(1.5,2.1,-3.21)) ;
#119316=CARTESIAN_POINT('Origin',(1.5,2.1,-3.41)) ;
#119317=CARTESIAN_POINT('Origin',(1.5,2.1,-3.41)) ;
#119318=CARTESIAN_POINT('Origin',(7.9,2.1,-34.89)) ;
#119319=CARTESIAN_POINT('Origin',(7.9,2.4,-34.89)) ;
#119320=CARTESIAN_POINT('Origin',(7.9,2.1,-34.89)) ;
#119321=CARTESIAN_POINT('Origin',(7.9,2.4,-34.89)) ;
#119322=CARTESIAN_POINT('Origin',(7.9,2.4,-34.89)) ;
#119323=CARTESIAN_POINT('Origin',(7.9,2.1,-34.89)) ;
#119324=CARTESIAN_POINT('Origin',(7.9,2.1,-34.89)) ;
#119325=CARTESIAN_POINT('Origin',(7.9,2.4,-34.89)) ;
#119326=CARTESIAN_POINT('Origin',(7.9,2.4,-34.9985786437627)) ;
#119327=CARTESIAN_POINT('Origin',(7.9,2.1,-34.89)) ;
#119328=CARTESIAN_POINT('Origin',(7.9,2.1,-35.84)) ;
#119329=CARTESIAN_POINT('Origin',(7.9,2.6,-34.9985786437627)) ;
#119330=CARTESIAN_POINT('Origin',(7.9,2.45857864376269,-35.14)) ;
#119331=CARTESIAN_POINT('Origin',(7.9,1.9,-35.84)) ;
#119332=CARTESIAN_POINT('Origin',(7.9,1.9,-36.04)) ;
#119333=CARTESIAN_POINT('Origin',(7.9,2.45857864376269,-35.14)) ;
#119334=CARTESIAN_POINT('Origin',(7.9,1.9,-36.04)) ;
#119335=CARTESIAN_POINT('Origin',(7.9,-2.15,-36.04)) ;
#119336=CARTESIAN_POINT('Origin',(7.9,-2.15,-35.84)) ;
#119337=CARTESIAN_POINT('Origin',(7.9,-2.35,-35.84)) ;
#119338=CARTESIAN_POINT('Origin',(7.9,3.35,-35.5485786437627)) ;
#119339=CARTESIAN_POINT('Origin',(7.9,3.35,-33.0314213562373)) ;
#119340=CARTESIAN_POINT('Origin',(7.9,-2.35,-35.1931195934094)) ;
#119341=CARTESIAN_POINT('Origin',(7.9,-2.35,-35.1931195934094)) ;
#119342=CARTESIAN_POINT('Origin',(7.9,3.15,-33.0314213562373)) ;
#119343=CARTESIAN_POINT('Origin',(7.9,3.00857864376269,-32.89)) ;
#119344=CARTESIAN_POINT('Origin',(7.9,-2.15,-35.1931195934094)) ;
#119345=CARTESIAN_POINT('Origin',(7.9,-2.32153024911032,-35.0902732340176)) ;
#119346=CARTESIAN_POINT('Origin',(7.9,3.00857864376269,-32.89)) ;
#119347=CARTESIAN_POINT('Origin',(7.9,2.45857864376269,-33.44)) ;
#119348=CARTESIAN_POINT('Origin',(7.9,-3.65625,-34.29)) ;
#119349=CARTESIAN_POINT('Origin',(7.9,-2.32153024911033,-33.4897267659824)) ;
#119350=CARTESIAN_POINT('Origin',(7.9,2.6,-33.5814213562373)) ;
#119351=CARTESIAN_POINT('Origin',(7.9,2.4,-33.5814213562373)) ;
#119352=CARTESIAN_POINT('Origin',(7.9,-2.15,-33.3868804065906)) ;
#119353=CARTESIAN_POINT('Origin',(7.9,-2.35,-33.3868804065906)) ;
#119354=CARTESIAN_POINT('Origin',(7.9,2.4,-33.5814213562373)) ;
#119355=CARTESIAN_POINT('Origin',(7.9,2.4,-33.69)) ;
#119356=CARTESIAN_POINT('Origin',(7.9,-2.35,-32.74)) ;
#119357=CARTESIAN_POINT('Origin',(7.9,-2.35,-32.74)) ;
#119358=CARTESIAN_POINT('Origin',(7.9,2.4,-33.69)) ;
#119359=CARTESIAN_POINT('Origin',(7.9,2.4,-33.69)) ;
#119360=CARTESIAN_POINT('Origin',(7.9,-2.15,-32.74)) ;
#119361=CARTESIAN_POINT('Origin',(7.9,-2.15,-32.54)) ;
#119362=CARTESIAN_POINT('Origin',(7.9,2.4,-33.69)) ;
#119363=CARTESIAN_POINT('Origin',(7.9,2.1,-33.69)) ;
#119364=CARTESIAN_POINT('Origin',(7.9,1.9,-32.54)) ;
#119365=CARTESIAN_POINT('Origin',(7.9,1.9,-32.54)) ;
#119366=CARTESIAN_POINT('Origin',(7.9,2.1,-33.69)) ;
#119367=CARTESIAN_POINT('Origin',(7.9,2.1,-33.69)) ;
#119368=CARTESIAN_POINT('Origin',(7.9,1.9,-32.74)) ;
#119369=CARTESIAN_POINT('Origin',(7.9,2.1,-32.74)) ;
#119370=CARTESIAN_POINT('Origin',(7.9,2.1,-32.74)) ;
#119371=CARTESIAN_POINT('Origin',(7.9,2.1,-31.08)) ;
#119372=CARTESIAN_POINT('Origin',(7.9,2.4,-31.08)) ;
#119373=CARTESIAN_POINT('Origin',(7.9,2.1,-31.08)) ;
#119374=CARTESIAN_POINT('Origin',(7.9,2.4,-31.08)) ;
#119375=CARTESIAN_POINT('Origin',(7.9,2.4,-31.08)) ;
#119376=CARTESIAN_POINT('Origin',(7.9,2.1,-31.08)) ;
#119377=CARTESIAN_POINT('Origin',(7.9,2.1,-31.08)) ;
#119378=CARTESIAN_POINT('Origin',(7.9,2.4,-31.08)) ;
#119379=CARTESIAN_POINT('Origin',(7.9,2.4,-31.1885786437627)) ;
#119380=CARTESIAN_POINT('Origin',(7.9,2.1,-31.08)) ;
#119381=CARTESIAN_POINT('Origin',(7.9,2.1,-32.03)) ;
#119382=CARTESIAN_POINT('Origin',(7.9,2.6,-31.1885786437627)) ;
#119383=CARTESIAN_POINT('Origin',(7.9,2.45857864376269,-31.33)) ;
#119384=CARTESIAN_POINT('Origin',(7.9,1.9,-32.03)) ;
#119385=CARTESIAN_POINT('Origin',(7.9,1.9,-32.23)) ;
#119386=CARTESIAN_POINT('Origin',(7.9,2.45857864376269,-31.33)) ;
#119387=CARTESIAN_POINT('Origin',(7.9,1.9,-32.23)) ;
#119388=CARTESIAN_POINT('Origin',(7.9,-2.15,-32.23)) ;
#119389=CARTESIAN_POINT('Origin',(7.9,-2.15,-32.03)) ;
#119390=CARTESIAN_POINT('Origin',(7.9,-2.35,-32.03)) ;
#119391=CARTESIAN_POINT('Origin',(7.9,3.35,-31.7385786437627)) ;
#119392=CARTESIAN_POINT('Origin',(7.9,3.35,-29.2214213562373)) ;
#119393=CARTESIAN_POINT('Origin',(7.9,-2.35,-31.3831195934094)) ;
#119394=CARTESIAN_POINT('Origin',(7.9,-2.35,-31.3831195934094)) ;
#119395=CARTESIAN_POINT('Origin',(7.9,3.15,-29.2214213562373)) ;
#119396=CARTESIAN_POINT('Origin',(7.9,3.00857864376269,-29.08)) ;
#119397=CARTESIAN_POINT('Origin',(7.9,-2.15,-31.3831195934094)) ;
#119398=CARTESIAN_POINT('Origin',(7.9,-2.32153024911032,-31.2802732340176)) ;
#119399=CARTESIAN_POINT('Origin',(7.9,3.00857864376269,-29.08)) ;
#119400=CARTESIAN_POINT('Origin',(7.9,2.45857864376269,-29.63)) ;
#119401=CARTESIAN_POINT('Origin',(7.9,-3.65625,-30.48)) ;
#119402=CARTESIAN_POINT('Origin',(7.9,-2.32153024911032,-29.6797267659824)) ;
#119403=CARTESIAN_POINT('Origin',(7.9,2.6,-29.7714213562373)) ;
#119404=CARTESIAN_POINT('Origin',(7.9,2.4,-29.7714213562373)) ;
#119405=CARTESIAN_POINT('Origin',(7.9,-2.15,-29.5768804065906)) ;
#119406=CARTESIAN_POINT('Origin',(7.9,-2.35,-29.5768804065906)) ;
#119407=CARTESIAN_POINT('Origin',(7.9,2.4,-29.7714213562373)) ;
#119408=CARTESIAN_POINT('Origin',(7.9,2.4,-29.88)) ;
#119409=CARTESIAN_POINT('Origin',(7.9,-2.35,-28.93)) ;
#119410=CARTESIAN_POINT('Origin',(7.9,-2.35,-28.93)) ;
#119411=CARTESIAN_POINT('Origin',(7.9,2.4,-29.88)) ;
#119412=CARTESIAN_POINT('Origin',(7.9,2.4,-29.88)) ;
#119413=CARTESIAN_POINT('Origin',(7.9,-2.15,-28.93)) ;
#119414=CARTESIAN_POINT('Origin',(7.9,-2.15,-28.73)) ;
#119415=CARTESIAN_POINT('Origin',(7.9,2.4,-29.88)) ;
#119416=CARTESIAN_POINT('Origin',(7.9,2.1,-29.88)) ;
#119417=CARTESIAN_POINT('Origin',(7.9,1.9,-28.73)) ;
#119418=CARTESIAN_POINT('Origin',(7.9,1.9,-28.73)) ;
#119419=CARTESIAN_POINT('Origin',(7.9,2.1,-29.88)) ;
#119420=CARTESIAN_POINT('Origin',(7.9,2.1,-29.88)) ;
#119421=CARTESIAN_POINT('Origin',(7.9,1.9,-28.93)) ;
#119422=CARTESIAN_POINT('Origin',(7.9,2.1,-28.93)) ;
#119423=CARTESIAN_POINT('Origin',(7.9,2.1,-28.93)) ;
#119424=CARTESIAN_POINT('Origin',(7.9,2.1,-27.27)) ;
#119425=CARTESIAN_POINT('Origin',(7.9,2.4,-27.27)) ;
#119426=CARTESIAN_POINT('Origin',(7.9,2.1,-27.27)) ;
#119427=CARTESIAN_POINT('Origin',(7.9,2.4,-27.27)) ;
#119428=CARTESIAN_POINT('Origin',(7.9,2.4,-27.27)) ;
#119429=CARTESIAN_POINT('Origin',(7.9,2.1,-27.27)) ;
#119430=CARTESIAN_POINT('Origin',(7.9,2.1,-27.27)) ;
#119431=CARTESIAN_POINT('Origin',(7.9,2.4,-27.27)) ;
#119432=CARTESIAN_POINT('Origin',(7.9,2.4,-27.3785786437627)) ;
#119433=CARTESIAN_POINT('Origin',(7.9,2.1,-27.27)) ;
#119434=CARTESIAN_POINT('Origin',(7.9,2.1,-28.22)) ;
#119435=CARTESIAN_POINT('Origin',(7.9,2.6,-27.3785786437627)) ;
#119436=CARTESIAN_POINT('Origin',(7.9,2.45857864376269,-27.52)) ;
#119437=CARTESIAN_POINT('Origin',(7.9,1.9,-28.22)) ;
#119438=CARTESIAN_POINT('Origin',(7.9,1.9,-28.42)) ;
#119439=CARTESIAN_POINT('Origin',(7.9,2.45857864376269,-27.52)) ;
#119440=CARTESIAN_POINT('Origin',(7.9,1.9,-28.42)) ;
#119441=CARTESIAN_POINT('Origin',(7.9,-2.15,-28.42)) ;
#119442=CARTESIAN_POINT('Origin',(7.9,-2.15,-28.22)) ;
#119443=CARTESIAN_POINT('Origin',(7.9,-2.35,-28.22)) ;
#119444=CARTESIAN_POINT('Origin',(7.9,3.35,-27.9285786437627)) ;
#119445=CARTESIAN_POINT('Origin',(7.9,3.35,-25.4114213562373)) ;
#119446=CARTESIAN_POINT('Origin',(7.9,-2.35,-27.5731195934094)) ;
#119447=CARTESIAN_POINT('Origin',(7.9,-2.35,-27.5731195934094)) ;
#119448=CARTESIAN_POINT('Origin',(7.9,3.15,-25.4114213562373)) ;
#119449=CARTESIAN_POINT('Origin',(7.9,3.00857864376269,-25.27)) ;
#119450=CARTESIAN_POINT('Origin',(7.9,-2.15,-27.5731195934094)) ;
#119451=CARTESIAN_POINT('Origin',(7.9,-2.32153024911032,-27.4702732340176)) ;
#119452=CARTESIAN_POINT('Origin',(7.9,3.00857864376269,-25.27)) ;
#119453=CARTESIAN_POINT('Origin',(7.9,2.45857864376269,-25.82)) ;
#119454=CARTESIAN_POINT('Origin',(7.9,-3.65625,-26.67)) ;
#119455=CARTESIAN_POINT('Origin',(7.9,-2.32153024911032,-25.8697267659824)) ;
#119456=CARTESIAN_POINT('Origin',(7.9,2.6,-25.9614213562373)) ;
#119457=CARTESIAN_POINT('Origin',(7.9,2.4,-25.9614213562373)) ;
#119458=CARTESIAN_POINT('Origin',(7.9,-2.15,-25.7668804065906)) ;
#119459=CARTESIAN_POINT('Origin',(7.9,-2.35,-25.7668804065906)) ;
#119460=CARTESIAN_POINT('Origin',(7.9,2.4,-25.9614213562373)) ;
#119461=CARTESIAN_POINT('Origin',(7.9,2.4,-26.07)) ;
#119462=CARTESIAN_POINT('Origin',(7.9,-2.35,-25.12)) ;
#119463=CARTESIAN_POINT('Origin',(7.9,-2.35,-25.12)) ;
#119464=CARTESIAN_POINT('Origin',(7.9,2.4,-26.07)) ;
#119465=CARTESIAN_POINT('Origin',(7.9,2.4,-26.07)) ;
#119466=CARTESIAN_POINT('Origin',(7.9,-2.15,-25.12)) ;
#119467=CARTESIAN_POINT('Origin',(7.9,-2.15,-24.92)) ;
#119468=CARTESIAN_POINT('Origin',(7.9,2.4,-26.07)) ;
#119469=CARTESIAN_POINT('Origin',(7.9,2.1,-26.07)) ;
#119470=CARTESIAN_POINT('Origin',(7.9,1.9,-24.92)) ;
#119471=CARTESIAN_POINT('Origin',(7.9,1.9,-24.92)) ;
#119472=CARTESIAN_POINT('Origin',(7.9,2.1,-26.07)) ;
#119473=CARTESIAN_POINT('Origin',(7.9,2.1,-26.07)) ;
#119474=CARTESIAN_POINT('Origin',(7.9,1.9,-25.12)) ;
#119475=CARTESIAN_POINT('Origin',(7.9,2.1,-25.12)) ;
#119476=CARTESIAN_POINT('Origin',(7.9,2.1,-25.12)) ;
#119477=CARTESIAN_POINT('Origin',(7.9,2.1,-23.46)) ;
#119478=CARTESIAN_POINT('Origin',(7.9,2.4,-23.46)) ;
#119479=CARTESIAN_POINT('Origin',(7.9,2.1,-23.46)) ;
#119480=CARTESIAN_POINT('Origin',(7.9,2.4,-23.46)) ;
#119481=CARTESIAN_POINT('Origin',(7.9,2.4,-23.46)) ;
#119482=CARTESIAN_POINT('Origin',(7.9,2.1,-23.46)) ;
#119483=CARTESIAN_POINT('Origin',(7.9,2.1,-23.46)) ;
#119484=CARTESIAN_POINT('Origin',(7.9,2.4,-23.46)) ;
#119485=CARTESIAN_POINT('Origin',(7.9,2.4,-23.5685786437627)) ;
#119486=CARTESIAN_POINT('Origin',(7.9,2.1,-23.46)) ;
#119487=CARTESIAN_POINT('Origin',(7.9,2.1,-24.41)) ;
#119488=CARTESIAN_POINT('Origin',(7.9,2.6,-23.5685786437627)) ;
#119489=CARTESIAN_POINT('Origin',(7.9,2.45857864376269,-23.71)) ;
#119490=CARTESIAN_POINT('Origin',(7.9,1.9,-24.41)) ;
#119491=CARTESIAN_POINT('Origin',(7.9,1.9,-24.61)) ;
#119492=CARTESIAN_POINT('Origin',(7.9,2.45857864376269,-23.71)) ;
#119493=CARTESIAN_POINT('Origin',(7.9,1.9,-24.61)) ;
#119494=CARTESIAN_POINT('Origin',(7.9,-2.15,-24.61)) ;
#119495=CARTESIAN_POINT('Origin',(7.9,-2.15,-24.41)) ;
#119496=CARTESIAN_POINT('Origin',(7.9,-2.35,-24.41)) ;
#119497=CARTESIAN_POINT('Origin',(7.9,3.35,-24.1185786437627)) ;
#119498=CARTESIAN_POINT('Origin',(7.9,3.35,-21.6014213562373)) ;
#119499=CARTESIAN_POINT('Origin',(7.9,-2.35,-23.7631195934094)) ;
#119500=CARTESIAN_POINT('Origin',(7.9,-2.35,-23.7631195934094)) ;
#119501=CARTESIAN_POINT('Origin',(7.9,3.15,-21.6014213562373)) ;
#119502=CARTESIAN_POINT('Origin',(7.9,3.00857864376269,-21.46)) ;
#119503=CARTESIAN_POINT('Origin',(7.9,-2.15,-23.7631195934094)) ;
#119504=CARTESIAN_POINT('Origin',(7.9,-2.32153024911032,-23.6602732340176)) ;
#119505=CARTESIAN_POINT('Origin',(7.9,3.00857864376269,-21.46)) ;
#119506=CARTESIAN_POINT('Origin',(7.9,2.45857864376269,-22.01)) ;
#119507=CARTESIAN_POINT('Origin',(7.9,-3.65625,-22.86)) ;
#119508=CARTESIAN_POINT('Origin',(7.9,-2.32153024911032,-22.0597267659824)) ;
#119509=CARTESIAN_POINT('Origin',(7.9,2.6,-22.1514213562373)) ;
#119510=CARTESIAN_POINT('Origin',(7.9,2.4,-22.1514213562373)) ;
#119511=CARTESIAN_POINT('Origin',(7.9,-2.15,-21.9568804065906)) ;
#119512=CARTESIAN_POINT('Origin',(7.9,-2.35,-21.9568804065906)) ;
#119513=CARTESIAN_POINT('Origin',(7.9,2.4,-22.1514213562373)) ;
#119514=CARTESIAN_POINT('Origin',(7.9,2.4,-22.26)) ;
#119515=CARTESIAN_POINT('Origin',(7.9,-2.35,-21.31)) ;
#119516=CARTESIAN_POINT('Origin',(7.9,-2.35,-21.31)) ;
#119517=CARTESIAN_POINT('Origin',(7.9,2.4,-22.26)) ;
#119518=CARTESIAN_POINT('Origin',(7.9,2.4,-22.26)) ;
#119519=CARTESIAN_POINT('Origin',(7.9,-2.15,-21.31)) ;
#119520=CARTESIAN_POINT('Origin',(7.9,-2.15,-21.11)) ;
#119521=CARTESIAN_POINT('Origin',(7.9,2.4,-22.26)) ;
#119522=CARTESIAN_POINT('Origin',(7.9,2.1,-22.26)) ;
#119523=CARTESIAN_POINT('Origin',(7.9,1.9,-21.11)) ;
#119524=CARTESIAN_POINT('Origin',(7.9,1.9,-21.11)) ;
#119525=CARTESIAN_POINT('Origin',(7.9,2.1,-22.26)) ;
#119526=CARTESIAN_POINT('Origin',(7.9,2.1,-22.26)) ;
#119527=CARTESIAN_POINT('Origin',(7.9,1.9,-21.31)) ;
#119528=CARTESIAN_POINT('Origin',(7.9,2.1,-21.31)) ;
#119529=CARTESIAN_POINT('Origin',(7.9,2.1,-21.31)) ;
#119530=CARTESIAN_POINT('Origin',(7.9,2.1,-19.65)) ;
#119531=CARTESIAN_POINT('Origin',(7.9,2.4,-19.65)) ;
#119532=CARTESIAN_POINT('Origin',(7.9,2.1,-19.65)) ;
#119533=CARTESIAN_POINT('Origin',(7.9,2.4,-19.65)) ;
#119534=CARTESIAN_POINT('Origin',(7.9,2.4,-19.65)) ;
#119535=CARTESIAN_POINT('Origin',(7.9,2.1,-19.65)) ;
#119536=CARTESIAN_POINT('Origin',(7.9,2.1,-19.65)) ;
#119537=CARTESIAN_POINT('Origin',(7.9,2.4,-19.65)) ;
#119538=CARTESIAN_POINT('Origin',(7.9,2.4,-19.7585786437627)) ;
#119539=CARTESIAN_POINT('Origin',(7.9,2.1,-19.65)) ;
#119540=CARTESIAN_POINT('Origin',(7.9,2.1,-20.6)) ;
#119541=CARTESIAN_POINT('Origin',(7.9,2.6,-19.7585786437627)) ;
#119542=CARTESIAN_POINT('Origin',(7.9,2.45857864376269,-19.9)) ;
#119543=CARTESIAN_POINT('Origin',(7.9,1.9,-20.6)) ;
#119544=CARTESIAN_POINT('Origin',(7.9,1.9,-20.8)) ;
#119545=CARTESIAN_POINT('Origin',(7.9,2.45857864376269,-19.9)) ;
#119546=CARTESIAN_POINT('Origin',(7.9,1.9,-20.8)) ;
#119547=CARTESIAN_POINT('Origin',(7.9,-2.15,-20.8)) ;
#119548=CARTESIAN_POINT('Origin',(7.9,-2.15,-20.6)) ;
#119549=CARTESIAN_POINT('Origin',(7.9,-2.35,-20.6)) ;
#119550=CARTESIAN_POINT('Origin',(7.9,3.35,-20.3085786437627)) ;
#119551=CARTESIAN_POINT('Origin',(7.9,3.35,-17.7914213562373)) ;
#119552=CARTESIAN_POINT('Origin',(7.9,-2.35,-19.9531195934094)) ;
#119553=CARTESIAN_POINT('Origin',(7.9,-2.35,-19.9531195934094)) ;
#119554=CARTESIAN_POINT('Origin',(7.9,3.15,-17.7914213562373)) ;
#119555=CARTESIAN_POINT('Origin',(7.9,3.00857864376269,-17.65)) ;
#119556=CARTESIAN_POINT('Origin',(7.9,-2.15,-19.9531195934094)) ;
#119557=CARTESIAN_POINT('Origin',(7.9,-2.32153024911032,-19.8502732340176)) ;
#119558=CARTESIAN_POINT('Origin',(7.9,3.00857864376269,-17.65)) ;
#119559=CARTESIAN_POINT('Origin',(7.9,2.45857864376269,-18.2)) ;
#119560=CARTESIAN_POINT('Origin',(7.9,-3.65625,-19.05)) ;
#119561=CARTESIAN_POINT('Origin',(7.9,-2.32153024911032,-18.2497267659824)) ;
#119562=CARTESIAN_POINT('Origin',(7.9,2.6,-18.3414213562373)) ;
#119563=CARTESIAN_POINT('Origin',(7.9,2.4,-18.3414213562373)) ;
#119564=CARTESIAN_POINT('Origin',(7.9,-2.15,-18.1468804065906)) ;
#119565=CARTESIAN_POINT('Origin',(7.9,-2.35,-18.1468804065906)) ;
#119566=CARTESIAN_POINT('Origin',(7.9,2.4,-18.3414213562373)) ;
#119567=CARTESIAN_POINT('Origin',(7.9,2.4,-18.45)) ;
#119568=CARTESIAN_POINT('Origin',(7.9,-2.35,-17.5)) ;
#119569=CARTESIAN_POINT('Origin',(7.9,-2.35,-17.5)) ;
#119570=CARTESIAN_POINT('Origin',(7.9,2.4,-18.45)) ;
#119571=CARTESIAN_POINT('Origin',(7.9,2.4,-18.45)) ;
#119572=CARTESIAN_POINT('Origin',(7.9,-2.15,-17.5)) ;
#119573=CARTESIAN_POINT('Origin',(7.9,-2.15,-17.3)) ;
#119574=CARTESIAN_POINT('Origin',(7.9,2.4,-18.45)) ;
#119575=CARTESIAN_POINT('Origin',(7.9,2.1,-18.45)) ;
#119576=CARTESIAN_POINT('Origin',(7.9,1.9,-17.3)) ;
#119577=CARTESIAN_POINT('Origin',(7.9,1.9,-17.3)) ;
#119578=CARTESIAN_POINT('Origin',(7.9,2.1,-18.45)) ;
#119579=CARTESIAN_POINT('Origin',(7.9,2.1,-18.45)) ;
#119580=CARTESIAN_POINT('Origin',(7.9,1.9,-17.5)) ;
#119581=CARTESIAN_POINT('Origin',(7.9,2.1,-17.5)) ;
#119582=CARTESIAN_POINT('Origin',(7.9,2.1,-17.5)) ;
#119583=CARTESIAN_POINT('Origin',(7.9,2.1,-15.84)) ;
#119584=CARTESIAN_POINT('Origin',(7.9,2.4,-15.84)) ;
#119585=CARTESIAN_POINT('Origin',(7.9,2.1,-15.84)) ;
#119586=CARTESIAN_POINT('Origin',(7.9,2.4,-15.84)) ;
#119587=CARTESIAN_POINT('Origin',(7.9,2.4,-15.84)) ;
#119588=CARTESIAN_POINT('Origin',(7.9,2.1,-15.84)) ;
#119589=CARTESIAN_POINT('Origin',(7.9,2.1,-15.84)) ;
#119590=CARTESIAN_POINT('Origin',(7.9,2.4,-15.84)) ;
#119591=CARTESIAN_POINT('Origin',(7.9,2.4,-15.9485786437627)) ;
#119592=CARTESIAN_POINT('Origin',(7.9,2.1,-15.84)) ;
#119593=CARTESIAN_POINT('Origin',(7.9,2.1,-16.79)) ;
#119594=CARTESIAN_POINT('Origin',(7.9,2.6,-15.9485786437627)) ;
#119595=CARTESIAN_POINT('Origin',(7.9,2.45857864376269,-16.09)) ;
#119596=CARTESIAN_POINT('Origin',(7.9,1.9,-16.79)) ;
#119597=CARTESIAN_POINT('Origin',(7.9,1.9,-16.99)) ;
#119598=CARTESIAN_POINT('Origin',(7.9,2.45857864376269,-16.09)) ;
#119599=CARTESIAN_POINT('Origin',(7.9,1.9,-16.99)) ;
#119600=CARTESIAN_POINT('Origin',(7.9,-2.15,-16.99)) ;
#119601=CARTESIAN_POINT('Origin',(7.9,-2.15,-16.79)) ;
#119602=CARTESIAN_POINT('Origin',(7.9,-2.35,-16.79)) ;
#119603=CARTESIAN_POINT('Origin',(7.9,3.35,-16.4985786437627)) ;
#119604=CARTESIAN_POINT('Origin',(7.9,3.35,-13.9814213562373)) ;
#119605=CARTESIAN_POINT('Origin',(7.9,-2.35,-16.1431195934094)) ;
#119606=CARTESIAN_POINT('Origin',(7.9,-2.35,-16.1431195934094)) ;
#119607=CARTESIAN_POINT('Origin',(7.9,3.15,-13.9814213562373)) ;
#119608=CARTESIAN_POINT('Origin',(7.9,3.00857864376269,-13.84)) ;
#119609=CARTESIAN_POINT('Origin',(7.9,-2.15,-16.1431195934094)) ;
#119610=CARTESIAN_POINT('Origin',(7.9,-2.32153024911032,-16.0402732340176)) ;
#119611=CARTESIAN_POINT('Origin',(7.9,3.00857864376269,-13.84)) ;
#119612=CARTESIAN_POINT('Origin',(7.9,2.45857864376269,-14.39)) ;
#119613=CARTESIAN_POINT('Origin',(7.9,-3.65625,-15.24)) ;
#119614=CARTESIAN_POINT('Origin',(7.9,-2.32153024911032,-14.4397267659824)) ;
#119615=CARTESIAN_POINT('Origin',(7.9,2.6,-14.5314213562373)) ;
#119616=CARTESIAN_POINT('Origin',(7.9,2.4,-14.5314213562373)) ;
#119617=CARTESIAN_POINT('Origin',(7.9,-2.15,-14.3368804065906)) ;
#119618=CARTESIAN_POINT('Origin',(7.9,-2.35,-14.3368804065906)) ;
#119619=CARTESIAN_POINT('Origin',(7.9,2.4,-14.5314213562373)) ;
#119620=CARTESIAN_POINT('Origin',(7.9,2.4,-14.64)) ;
#119621=CARTESIAN_POINT('Origin',(7.9,-2.35,-13.69)) ;
#119622=CARTESIAN_POINT('Origin',(7.9,-2.35,-13.69)) ;
#119623=CARTESIAN_POINT('Origin',(7.9,2.4,-14.64)) ;
#119624=CARTESIAN_POINT('Origin',(7.9,2.4,-14.64)) ;
#119625=CARTESIAN_POINT('Origin',(7.9,-2.15,-13.69)) ;
#119626=CARTESIAN_POINT('Origin',(7.9,-2.15,-13.49)) ;
#119627=CARTESIAN_POINT('Origin',(7.9,2.4,-14.64)) ;
#119628=CARTESIAN_POINT('Origin',(7.9,2.1,-14.64)) ;
#119629=CARTESIAN_POINT('Origin',(7.9,1.9,-13.49)) ;
#119630=CARTESIAN_POINT('Origin',(7.9,1.9,-13.49)) ;
#119631=CARTESIAN_POINT('Origin',(7.9,2.1,-14.64)) ;
#119632=CARTESIAN_POINT('Origin',(7.9,2.1,-14.64)) ;
#119633=CARTESIAN_POINT('Origin',(7.9,1.9,-13.69)) ;
#119634=CARTESIAN_POINT('Origin',(7.9,2.1,-13.69)) ;
#119635=CARTESIAN_POINT('Origin',(7.9,2.1,-13.69)) ;
#119636=CARTESIAN_POINT('Origin',(7.9,2.1,-12.03)) ;
#119637=CARTESIAN_POINT('Origin',(7.9,2.4,-12.03)) ;
#119638=CARTESIAN_POINT('Origin',(7.9,2.1,-12.03)) ;
#119639=CARTESIAN_POINT('Origin',(7.9,2.4,-12.03)) ;
#119640=CARTESIAN_POINT('Origin',(7.9,2.4,-12.03)) ;
#119641=CARTESIAN_POINT('Origin',(7.9,2.1,-12.03)) ;
#119642=CARTESIAN_POINT('Origin',(7.9,2.1,-12.03)) ;
#119643=CARTESIAN_POINT('Origin',(7.9,2.4,-12.03)) ;
#119644=CARTESIAN_POINT('Origin',(7.9,2.4,-12.1385786437627)) ;
#119645=CARTESIAN_POINT('Origin',(7.9,2.1,-12.03)) ;
#119646=CARTESIAN_POINT('Origin',(7.9,2.1,-12.98)) ;
#119647=CARTESIAN_POINT('Origin',(7.9,2.6,-12.1385786437627)) ;
#119648=CARTESIAN_POINT('Origin',(7.9,2.45857864376269,-12.28)) ;
#119649=CARTESIAN_POINT('Origin',(7.9,1.9,-12.98)) ;
#119650=CARTESIAN_POINT('Origin',(7.9,1.9,-13.18)) ;
#119651=CARTESIAN_POINT('Origin',(7.9,2.45857864376269,-12.28)) ;
#119652=CARTESIAN_POINT('Origin',(7.9,1.9,-13.18)) ;
#119653=CARTESIAN_POINT('Origin',(7.9,-2.15,-13.18)) ;
#119654=CARTESIAN_POINT('Origin',(7.9,-2.15,-12.98)) ;
#119655=CARTESIAN_POINT('Origin',(7.9,-2.35,-12.98)) ;
#119656=CARTESIAN_POINT('Origin',(7.9,3.35,-12.6885786437627)) ;
#119657=CARTESIAN_POINT('Origin',(7.9,3.35,-10.1714213562373)) ;
#119658=CARTESIAN_POINT('Origin',(7.9,-2.35,-12.3331195934094)) ;
#119659=CARTESIAN_POINT('Origin',(7.9,-2.35,-12.3331195934094)) ;
#119660=CARTESIAN_POINT('Origin',(7.9,3.15,-10.1714213562373)) ;
#119661=CARTESIAN_POINT('Origin',(7.9,3.00857864376269,-10.03)) ;
#119662=CARTESIAN_POINT('Origin',(7.9,-2.15,-12.3331195934094)) ;
#119663=CARTESIAN_POINT('Origin',(7.9,-2.32153024911032,-12.2302732340176)) ;
#119664=CARTESIAN_POINT('Origin',(7.9,3.00857864376269,-10.03)) ;
#119665=CARTESIAN_POINT('Origin',(7.9,2.45857864376269,-10.58)) ;
#119666=CARTESIAN_POINT('Origin',(7.9,-3.65625,-11.43)) ;
#119667=CARTESIAN_POINT('Origin',(7.9,-2.32153024911032,-10.6297267659824)) ;
#119668=CARTESIAN_POINT('Origin',(7.9,2.6,-10.7214213562373)) ;
#119669=CARTESIAN_POINT('Origin',(7.9,2.4,-10.7214213562373)) ;
#119670=CARTESIAN_POINT('Origin',(7.9,-2.15,-10.5268804065906)) ;
#119671=CARTESIAN_POINT('Origin',(7.9,-2.35,-10.5268804065906)) ;
#119672=CARTESIAN_POINT('Origin',(7.9,2.4,-10.7214213562373)) ;
#119673=CARTESIAN_POINT('Origin',(7.9,2.4,-10.83)) ;
#119674=CARTESIAN_POINT('Origin',(7.9,-2.35,-9.88)) ;
#119675=CARTESIAN_POINT('Origin',(7.9,-2.35,-9.88)) ;
#119676=CARTESIAN_POINT('Origin',(7.9,2.4,-10.83)) ;
#119677=CARTESIAN_POINT('Origin',(7.9,2.4,-10.83)) ;
#119678=CARTESIAN_POINT('Origin',(7.9,-2.15,-9.88)) ;
#119679=CARTESIAN_POINT('Origin',(7.9,-2.15,-9.68)) ;
#119680=CARTESIAN_POINT('Origin',(7.9,2.4,-10.83)) ;
#119681=CARTESIAN_POINT('Origin',(7.9,2.1,-10.83)) ;
#119682=CARTESIAN_POINT('Origin',(7.9,1.9,-9.68)) ;
#119683=CARTESIAN_POINT('Origin',(7.9,1.9,-9.68)) ;
#119684=CARTESIAN_POINT('Origin',(7.9,2.1,-10.83)) ;
#119685=CARTESIAN_POINT('Origin',(7.9,2.1,-10.83)) ;
#119686=CARTESIAN_POINT('Origin',(7.9,1.9,-9.88)) ;
#119687=CARTESIAN_POINT('Origin',(7.9,2.1,-9.88)) ;
#119688=CARTESIAN_POINT('Origin',(7.9,2.1,-9.88)) ;
#119689=CARTESIAN_POINT('Origin',(7.9,2.1,-8.22)) ;
#119690=CARTESIAN_POINT('Origin',(7.9,2.4,-8.22)) ;
#119691=CARTESIAN_POINT('Origin',(7.9,2.1,-8.22)) ;
#119692=CARTESIAN_POINT('Origin',(7.9,2.4,-8.22)) ;
#119693=CARTESIAN_POINT('Origin',(7.9,2.4,-8.22)) ;
#119694=CARTESIAN_POINT('Origin',(7.9,2.1,-8.22)) ;
#119695=CARTESIAN_POINT('Origin',(7.9,2.1,-8.22)) ;
#119696=CARTESIAN_POINT('Origin',(7.9,2.4,-8.22)) ;
#119697=CARTESIAN_POINT('Origin',(7.9,2.4,-8.32857864376269)) ;
#119698=CARTESIAN_POINT('Origin',(7.9,2.1,-8.22)) ;
#119699=CARTESIAN_POINT('Origin',(7.9,2.1,-9.17)) ;
#119700=CARTESIAN_POINT('Origin',(7.9,2.6,-8.32857864376269)) ;
#119701=CARTESIAN_POINT('Origin',(7.9,2.45857864376269,-8.47)) ;
#119702=CARTESIAN_POINT('Origin',(7.9,1.9,-9.17)) ;
#119703=CARTESIAN_POINT('Origin',(7.9,1.9,-9.37)) ;
#119704=CARTESIAN_POINT('Origin',(7.9,2.45857864376269,-8.47)) ;
#119705=CARTESIAN_POINT('Origin',(7.9,1.9,-9.37)) ;
#119706=CARTESIAN_POINT('Origin',(7.9,-2.15,-9.37)) ;
#119707=CARTESIAN_POINT('Origin',(7.9,-2.15,-9.17)) ;
#119708=CARTESIAN_POINT('Origin',(7.9,-2.35,-9.17)) ;
#119709=CARTESIAN_POINT('Origin',(7.9,3.35,-8.87857864376269)) ;
#119710=CARTESIAN_POINT('Origin',(7.9,3.35,-6.36142135623731)) ;
#119711=CARTESIAN_POINT('Origin',(7.9,-2.35,-8.52311959340942)) ;
#119712=CARTESIAN_POINT('Origin',(7.9,-2.35,-8.52311959340942)) ;
#119713=CARTESIAN_POINT('Origin',(7.9,3.15,-6.36142135623731)) ;
#119714=CARTESIAN_POINT('Origin',(7.9,3.00857864376269,-6.22)) ;
#119715=CARTESIAN_POINT('Origin',(7.9,-2.15,-8.52311959340942)) ;
#119716=CARTESIAN_POINT('Origin',(7.9,-2.32153024911032,-8.4202732340176)) ;
#119717=CARTESIAN_POINT('Origin',(7.9,3.00857864376269,-6.22)) ;
#119718=CARTESIAN_POINT('Origin',(7.9,2.45857864376269,-6.77)) ;
#119719=CARTESIAN_POINT('Origin',(7.9,-3.65625,-7.62)) ;
#119720=CARTESIAN_POINT('Origin',(7.9,-2.32153024911032,-6.8197267659824)) ;
#119721=CARTESIAN_POINT('Origin',(7.9,2.6,-6.91142135623731)) ;
#119722=CARTESIAN_POINT('Origin',(7.9,2.4,-6.91142135623731)) ;
#119723=CARTESIAN_POINT('Origin',(7.9,-2.15,-6.71688040659058)) ;
#119724=CARTESIAN_POINT('Origin',(7.9,-2.35,-6.71688040659058)) ;
#119725=CARTESIAN_POINT('Origin',(7.9,2.4,-6.91142135623731)) ;
#119726=CARTESIAN_POINT('Origin',(7.9,2.4,-7.02)) ;
#119727=CARTESIAN_POINT('Origin',(7.9,-2.35,-6.07)) ;
#119728=CARTESIAN_POINT('Origin',(7.9,-2.35,-6.07)) ;
#119729=CARTESIAN_POINT('Origin',(7.9,2.4,-7.02)) ;
#119730=CARTESIAN_POINT('Origin',(7.9,2.4,-7.02)) ;
#119731=CARTESIAN_POINT('Origin',(7.9,-2.15,-6.07)) ;
#119732=CARTESIAN_POINT('Origin',(7.9,-2.15,-5.87)) ;
#119733=CARTESIAN_POINT('Origin',(7.9,2.4,-7.02)) ;
#119734=CARTESIAN_POINT('Origin',(7.9,2.1,-7.02)) ;
#119735=CARTESIAN_POINT('Origin',(7.9,1.9,-5.87)) ;
#119736=CARTESIAN_POINT('Origin',(7.9,1.9,-5.87)) ;
#119737=CARTESIAN_POINT('Origin',(7.9,2.1,-7.02)) ;
#119738=CARTESIAN_POINT('Origin',(7.9,2.1,-7.02)) ;
#119739=CARTESIAN_POINT('Origin',(7.9,1.9,-6.07)) ;
#119740=CARTESIAN_POINT('Origin',(7.9,2.1,-6.07)) ;
#119741=CARTESIAN_POINT('Origin',(7.9,2.1,-6.07)) ;
#119742=CARTESIAN_POINT('Origin',(7.9,2.1,-4.41)) ;
#119743=CARTESIAN_POINT('Origin',(7.9,2.4,-4.41)) ;
#119744=CARTESIAN_POINT('Origin',(7.9,2.1,-4.41)) ;
#119745=CARTESIAN_POINT('Origin',(7.9,2.4,-4.41)) ;
#119746=CARTESIAN_POINT('Origin',(7.9,2.4,-4.41)) ;
#119747=CARTESIAN_POINT('Origin',(7.9,2.1,-4.41)) ;
#119748=CARTESIAN_POINT('Origin',(7.9,2.1,-4.41)) ;
#119749=CARTESIAN_POINT('Origin',(7.9,2.4,-4.41)) ;
#119750=CARTESIAN_POINT('Origin',(7.9,2.4,-4.51857864376269)) ;
#119751=CARTESIAN_POINT('Origin',(7.9,2.1,-4.41)) ;
#119752=CARTESIAN_POINT('Origin',(7.9,2.1,-5.36)) ;
#119753=CARTESIAN_POINT('Origin',(7.9,2.6,-4.51857864376269)) ;
#119754=CARTESIAN_POINT('Origin',(7.9,2.45857864376269,-4.66)) ;
#119755=CARTESIAN_POINT('Origin',(7.9,1.9,-5.36)) ;
#119756=CARTESIAN_POINT('Origin',(7.9,1.9,-5.56)) ;
#119757=CARTESIAN_POINT('Origin',(7.9,2.45857864376269,-4.66)) ;
#119758=CARTESIAN_POINT('Origin',(7.9,1.9,-5.56)) ;
#119759=CARTESIAN_POINT('Origin',(7.9,-2.15,-5.56)) ;
#119760=CARTESIAN_POINT('Origin',(7.9,-2.15,-5.36)) ;
#119761=CARTESIAN_POINT('Origin',(7.9,-2.35,-5.36)) ;
#119762=CARTESIAN_POINT('Origin',(7.9,3.35,-5.06857864376269)) ;
#119763=CARTESIAN_POINT('Origin',(7.9,3.35,-2.55142135623731)) ;
#119764=CARTESIAN_POINT('Origin',(7.9,-2.35,-4.71311959340942)) ;
#119765=CARTESIAN_POINT('Origin',(7.9,-2.35,-4.71311959340942)) ;
#119766=CARTESIAN_POINT('Origin',(7.9,3.15,-2.55142135623731)) ;
#119767=CARTESIAN_POINT('Origin',(7.9,3.00857864376269,-2.41)) ;
#119768=CARTESIAN_POINT('Origin',(7.9,-2.15,-4.71311959340942)) ;
#119769=CARTESIAN_POINT('Origin',(7.9,-2.32153024911032,-4.6102732340176)) ;
#119770=CARTESIAN_POINT('Origin',(7.9,3.00857864376269,-2.41)) ;
#119771=CARTESIAN_POINT('Origin',(7.9,2.45857864376269,-2.96)) ;
#119772=CARTESIAN_POINT('Origin',(7.9,-3.65625,-3.81)) ;
#119773=CARTESIAN_POINT('Origin',(7.9,-2.32153024911032,-3.0097267659824)) ;
#119774=CARTESIAN_POINT('Origin',(7.9,2.6,-3.10142135623731)) ;
#119775=CARTESIAN_POINT('Origin',(7.9,2.4,-3.10142135623731)) ;
#119776=CARTESIAN_POINT('Origin',(7.9,-2.15,-2.90688040659058)) ;
#119777=CARTESIAN_POINT('Origin',(7.9,-2.35,-2.90688040659058)) ;
#119778=CARTESIAN_POINT('Origin',(7.9,2.4,-3.10142135623731)) ;
#119779=CARTESIAN_POINT('Origin',(7.9,2.4,-3.21)) ;
#119780=CARTESIAN_POINT('Origin',(7.9,-2.35,-2.26)) ;
#119781=CARTESIAN_POINT('Origin',(7.9,-2.35,-2.26)) ;
#119782=CARTESIAN_POINT('Origin',(7.9,2.4,-3.21)) ;
#119783=CARTESIAN_POINT('Origin',(7.9,2.4,-3.21)) ;
#119784=CARTESIAN_POINT('Origin',(7.9,-2.15,-2.26)) ;
#119785=CARTESIAN_POINT('Origin',(7.9,-2.15,-2.06)) ;
#119786=CARTESIAN_POINT('Origin',(7.9,2.4,-3.21)) ;
#119787=CARTESIAN_POINT('Origin',(7.9,2.1,-3.21)) ;
#119788=CARTESIAN_POINT('Origin',(7.9,1.9,-2.06)) ;
#119789=CARTESIAN_POINT('Origin',(7.9,1.9,-2.06)) ;
#119790=CARTESIAN_POINT('Origin',(7.9,2.1,-3.21)) ;
#119791=CARTESIAN_POINT('Origin',(7.9,2.1,-3.21)) ;
#119792=CARTESIAN_POINT('Origin',(7.9,1.9,-2.26)) ;
#119793=CARTESIAN_POINT('Origin',(7.9,2.1,-2.26)) ;
#119794=CARTESIAN_POINT('Origin',(7.9,2.1,-2.26)) ;
#119795=CARTESIAN_POINT('Origin',(-0.899999999999999,-2.,-7.02)) ;
#119796=CARTESIAN_POINT('Origin',(-0.899999999999999,0.4,-7.02)) ;
#119797=CARTESIAN_POINT('Origin',(-0.899999999999999,-1.9,-7.02)) ;
#119798=CARTESIAN_POINT('Origin',(0.600000000000001,0.4,-7.22)) ;
#119799=CARTESIAN_POINT('Origin',(0.500000000000001,0.4,-7.22)) ;
#119800=CARTESIAN_POINT('Origin',(-0.899999999999999,0.4,-7.22)) ;
#119801=CARTESIAN_POINT('Origin',(0.500000000000001,0.4,-7.22)) ;
#119802=CARTESIAN_POINT('',(0.600000000000001,0.4,-7.22)) ;
#119803=CARTESIAN_POINT('Origin',(0.500000000000001,0.4,-7.22)) ;
#119804=CARTESIAN_POINT('Origin',(0.500000000000001,0.4,-7.22)) ;
#119805=CARTESIAN_POINT('Origin',(-0.899999999999999,-1.9,-7.02)) ;
#119806=CARTESIAN_POINT('Origin',(-0.899999999999999,-1.9,-7.02)) ;
#119807=CARTESIAN_POINT('Origin',(-0.899999999999999,-1.9,-7.02)) ;
#119808=CARTESIAN_POINT('Origin',(-0.899999999999999,0.4,-7.22)) ;
#119809=CARTESIAN_POINT('Origin',(-0.899999999999999,0.6,-7.22)) ;
#119810=CARTESIAN_POINT('Origin',(0.500000000000001,0.4,-7.62)) ;
#119811=CARTESIAN_POINT('Origin',(0.500000000000001,0.4,-8.02)) ;
#119812=CARTESIAN_POINT('',(0.600000000000001,0.4,-7.92)) ;
#119813=CARTESIAN_POINT('Ctrl Pts',(0.595612997216081,0.370705721320404,
-7.9907057213204)) ;
#119814=CARTESIAN_POINT('Ctrl Pts',(0.596180587760891,0.372558268494353,
-7.98885549883217)) ;
#119815=CARTESIAN_POINT('Ctrl Pts',(0.596672461925684,0.374355839771976,
-7.98691417986632)) ;
#119816=CARTESIAN_POINT('Ctrl Pts',(0.599015141889213,0.383869350930064,
-7.97576499365627)) ;
#119817=CARTESIAN_POINT('Ctrl Pts',(0.599609996542524,0.390224332900447,
-7.96497260265412)) ;
#119818=CARTESIAN_POINT('Ctrl Pts',(0.600050586298725,0.398117439141558,
-7.94233105320469)) ;
#119819=CARTESIAN_POINT('Ctrl Pts',(0.600000000000001,0.399999999999999,
-7.93120125063353)) ;
#119820=CARTESIAN_POINT('Ctrl Pts',(0.600000000000001,0.399999999999999,
-7.92)) ;
#119821=CARTESIAN_POINT('',(0.600000000000001,0.4,-7.62)) ;
#119822=CARTESIAN_POINT('Origin',(0.500000000000001,-4.5664044441154E-17,
-7.22)) ;
#119823=CARTESIAN_POINT('',(0.500000000000001,0.394987437106619,-7.32)) ;
#119824=CARTESIAN_POINT('Ctrl Pts',(0.500000000000001,0.394987437106619,
-7.32)) ;
#119825=CARTESIAN_POINT('Ctrl Pts',(0.505940567948952,0.3955844866499,-7.32)) ;
#119826=CARTESIAN_POINT('Ctrl Pts',(0.51193197101914,0.396132036079018,
-7.31946630032796)) ;
#119827=CARTESIAN_POINT('Ctrl Pts',(0.517829015308548,0.396618246075354,
-7.31839779577372)) ;
#119828=CARTESIAN_POINT('Ctrl Pts',(0.522982218721201,0.397043126556053,
-7.31746407015711)) ;
#119829=CARTESIAN_POINT('Ctrl Pts',(0.52806264897023,0.397421319341388,
-7.31612282679706)) ;
#119830=CARTESIAN_POINT('Ctrl Pts',(0.532978106724,0.397751505046071,-7.31440574387663)) ;
#119831=CARTESIAN_POINT('Ctrl Pts',(0.538583536338966,0.398128038182999,
-7.31244763784955)) ;
#119832=CARTESIAN_POINT('Ctrl Pts',(0.544059405914893,0.398447721828296,
-7.30997000831105)) ;
#119833=CARTESIAN_POINT('Ctrl Pts',(0.549268572255785,0.398712331108984,
-7.30702073194289)) ;
#119834=CARTESIAN_POINT('Ctrl Pts',(0.553856850427149,0.398945401221756,
-7.30442298414684)) ;
#119835=CARTESIAN_POINT('Ctrl Pts',(0.558237825069329,0.399135987683843,
-7.30146038497999)) ;
#119836=CARTESIAN_POINT('Ctrl Pts',(0.562333836086214,0.399290378266507,
-7.29819522286417)) ;
#119837=CARTESIAN_POINT('Ctrl Pts',(0.566990328957901,0.399465895042381,
-7.2944832689523)) ;
#119838=CARTESIAN_POINT('Ctrl Pts',(0.571349096493437,0.399597278936107,
-7.29032280648479)) ;
#119839=CARTESIAN_POINT('Ctrl Pts',(0.57529692005673,0.399694832180838,
-7.28580557597932)) ;
#119840=CARTESIAN_POINT('Ctrl Pts',(0.578744263667919,0.399780018245914,
-7.28186101121506)) ;
#119841=CARTESIAN_POINT('Ctrl Pts',(0.581878314560434,0.399839626289636,
-7.2776455218421)) ;
#119842=CARTESIAN_POINT('Ctrl Pts',(0.584648147334856,0.399882153365958,
-7.27324181770729)) ;
#119843=CARTESIAN_POINT('Ctrl Pts',(0.587839270208173,0.399931148788079,
-7.2681683125045)) ;
#119844=CARTESIAN_POINT('Ctrl Pts',(0.590595054415089,0.399958289583404,
-7.26276663624446)) ;
#119845=CARTESIAN_POINT('Ctrl Pts',(0.5928386189431,0.399974357003159,-7.2571616850094)) ;
#119846=CARTESIAN_POINT('Ctrl Pts',(0.594777336851653,0.399988241245861,
-7.2523183122424)) ;
#119847=CARTESIAN_POINT('Ctrl Pts',(0.596334051506188,0.399993946552814,
-7.24732416622713)) ;
#119848=CARTESIAN_POINT('Ctrl Pts',(0.597488309822308,0.39999684570125,
-7.24227171856839)) ;
#119849=CARTESIAN_POINT('Ctrl Pts',(0.598804024094406,0.400000150378306,
-7.23651254196053)) ;
#119850=CARTESIAN_POINT('Ctrl Pts',(0.599612685195437,0.399999963509465,
-7.23060284389055)) ;
#119851=CARTESIAN_POINT('Ctrl Pts',(0.599890230999724,0.399999993975383,
-7.224684202261)) ;
#119852=CARTESIAN_POINT('Ctrl Pts',(0.599963464549401,0.400000002014155,
-7.22312250278977)) ;
#119853=CARTESIAN_POINT('Ctrl Pts',(0.600000000000001,0.399999999999999,
-7.22156022150916)) ;
#119854=CARTESIAN_POINT('Ctrl Pts',(0.600000000000001,0.399999999999999,
-7.22)) ;
#119855=CARTESIAN_POINT('',(0.600000000000001,0.299999999999999,-7.22)) ;
#119856=CARTESIAN_POINT('Ctrl Pts',(0.500000000000001,0.394987437106619,
-7.32)) ;
#119857=CARTESIAN_POINT('Ctrl Pts',(0.500454935589846,0.395033159853749,
-7.32)) ;
#119858=CARTESIAN_POINT('Ctrl Pts',(0.500909898680472,0.39507857032906,
-7.31999689549112)) ;
#119859=CARTESIAN_POINT('Ctrl Pts',(0.502892456245169,0.39527507588909,
-7.31996983394194)) ;
#119860=CARTESIAN_POINT('Ctrl Pts',(0.504418747482366,0.395422812032198,
-7.31991398542099)) ;
#119861=CARTESIAN_POINT('Ctrl Pts',(0.508462199543345,0.395804395682033,
-7.31967328105664)) ;
#119862=CARTESIAN_POINT('Ctrl Pts',(0.510974953343295,0.396031485023317,
-7.31942793914506)) ;
#119863=CARTESIAN_POINT('Ctrl Pts',(0.521160739721272,0.396903453186235,
-7.31804279449156)) ;
#119864=CARTESIAN_POINT('Ctrl Pts',(0.528708678528402,0.397444933153161,
-7.31610421770469)) ;
#119865=CARTESIAN_POINT('Ctrl Pts',(0.545943206358073,0.398105551684108,
-7.30946463945115)) ;
#119866=CARTESIAN_POINT('Ctrl Pts',(0.555229535466813,0.397987646678431,
-7.30403535883597)) ;
#119867=CARTESIAN_POINT('Ctrl Pts',(0.571394604995744,0.395490482808038,
-7.29077551336386)) ;
#119868=CARTESIAN_POINT('Ctrl Pts',(0.578055313702842,0.39319894869835,
-7.28324074563176)) ;
#119869=CARTESIAN_POINT('Ctrl Pts',(0.588559132202514,0.385442756729305,
-7.26739223398403)) ;
#119870=CARTESIAN_POINT('Ctrl Pts',(0.592167355639978,0.380240075126892,
-7.2595482656068)) ;
#119871=CARTESIAN_POINT('Ctrl Pts',(0.597496615531108,0.365892753466966,
-7.24392552179528)) ;
#119872=CARTESIAN_POINT('Ctrl Pts',(0.598734255154202,0.356660564300668,
-7.23677274172691)) ;
#119873=CARTESIAN_POINT('Ctrl Pts',(0.600012754681688,0.335223914398549,
-7.22558230586562)) ;
#119874=CARTESIAN_POINT('Ctrl Pts',(0.59999390055981,0.322655037091896,
-7.22166151936558)) ;
#119875=CARTESIAN_POINT('Ctrl Pts',(0.600000296204999,0.30610691358235,
-7.22013962634704)) ;
#119876=CARTESIAN_POINT('Ctrl Pts',(0.600000000000001,0.303050992413436,
-7.22)) ;
#119877=CARTESIAN_POINT('Ctrl Pts',(0.600000000000001,0.299999999999999,
-7.22)) ;
#119878=CARTESIAN_POINT('',(0.600000000000001,-2.39800009914439E-17,-7.22)) ;
#119879=CARTESIAN_POINT('Origin',(0.500000000000001,-1.9,-7.22)) ;
#119880=CARTESIAN_POINT('Origin',(0.600000000000001,-1.9,-7.02)) ;
#119881=CARTESIAN_POINT('Origin',(0.500000000000001,-1.9,-7.02)) ;
#119882=CARTESIAN_POINT('Origin',(-0.899999999999999,-1.9,-6.245)) ;
#119883=CARTESIAN_POINT('Origin',(-0.899999999999999,-1.9,-6.345)) ;
#119884=CARTESIAN_POINT('Origin',(-0.899999999999999,0.6,-7.12)) ;
#119885=CARTESIAN_POINT('Origin',(-0.899999999999999,0.6,-8.02)) ;
#119886=CARTESIAN_POINT('Origin',(0.600000000000001,0.4,-8.02)) ;
#119887=CARTESIAN_POINT('Origin',(0.500000000000001,0.4,-8.02)) ;
#119888=CARTESIAN_POINT('Origin',(-0.899999999999999,0.4,-8.02)) ;
#119889=CARTESIAN_POINT('Origin',(0.500000000000001,0.4,-8.02)) ;
#119890=CARTESIAN_POINT('Origin',(0.500000000000001,-1.9,-7.02)) ;
#119891=CARTESIAN_POINT('Origin',(0.500000000000001,-2.1,-7.02)) ;
#119892=CARTESIAN_POINT('Origin',(-0.899999999999999,-1.9,-6.345)) ;
#119893=CARTESIAN_POINT('Origin',(-1.1,-1.9,-6.345)) ;
#119894=CARTESIAN_POINT('Origin',(-0.899999999999999,-2.1,-6.345)) ;
#119895=CARTESIAN_POINT('Origin',(-0.899999999999999,0.4,-8.02)) ;
#119896=CARTESIAN_POINT('Origin',(-0.899999999999999,0.4,-8.22)) ;
#119897=CARTESIAN_POINT('Origin',(0.500000000000001,-2.1,-7.62)) ;
#119898=CARTESIAN_POINT('Origin',(0.500000000000001,-2.1,-6.345)) ;
#119899=CARTESIAN_POINT('Origin',(0.600000000000001,-2.1,-6.345)) ;
#119900=CARTESIAN_POINT('Origin',(0.500000000000001,-2.1,-6.345)) ;
#119901=CARTESIAN_POINT('Origin',(-1.1,-4.42727195005761E-17,-6.345)) ;
#119902=CARTESIAN_POINT('',(-1.1,1.15,-6.245)) ;
#119903=CARTESIAN_POINT('',(-1.1,1.25,-6.245)) ;
#119904=CARTESIAN_POINT('Origin',(-1.1,1.15,-6.345)) ;
#119905=CARTESIAN_POINT('Origin',(-0.899999999999999,0.5,-8.22)) ;
#119906=CARTESIAN_POINT('Origin',(-0.899999999999999,-1.9,-8.22)) ;
#119907=CARTESIAN_POINT('Origin',(0.600000000000001,-1.9,-8.22)) ;
#119908=CARTESIAN_POINT('Origin',(0.500000000000001,-1.9,-8.22)) ;
#119909=CARTESIAN_POINT('Origin',(-0.899999999999999,-1.9,-8.22)) ;
#119910=CARTESIAN_POINT('Origin',(0.500000000000001,-1.9,-8.22)) ;
#119911=CARTESIAN_POINT('Origin',(0.500000000000001,-2.1,-8.22)) ;
#119912=CARTESIAN_POINT('Origin',(0.500000000000001,-2.1,-6.345)) ;
#119913=CARTESIAN_POINT('Origin',(0.500000000000001,-2.1,-6.345)) ;
#119914=CARTESIAN_POINT('Origin',(-1.1,-2.9,-6.145)) ;
#119915=CARTESIAN_POINT('Origin',(-1.1,-2.9,-6.145)) ;
#119916=CARTESIAN_POINT('Origin',(-1.1,-2.9,-6.145)) ;
#119917=CARTESIAN_POINT('Origin',(-1.1,1.25,-6.145)) ;
#119918=CARTESIAN_POINT('Origin',(-1.1,1.15,-6.145)) ;
#119919=CARTESIAN_POINT('Origin',(-1.1,1.15,-6.345)) ;
#119920=CARTESIAN_POINT('',(-1.1,1.25,-6.345)) ;
#119921=CARTESIAN_POINT('Origin',(-1.1,1.15,-6.345)) ;
#119922=CARTESIAN_POINT('Origin',(-1.1,1.15,-6.345)) ;
#119923=CARTESIAN_POINT('Origin',(-0.899999999999999,-1.9,-8.22)) ;
#119924=CARTESIAN_POINT('Origin',(-0.899999999999999,-1.9,-8.22)) ;
#119925=CARTESIAN_POINT('Origin',(0.500000000000001,-2.1,-7.62)) ;
#119926=CARTESIAN_POINT('Origin',(0.500000000000001,-2.1,-8.895)) ;
#119927=CARTESIAN_POINT('Origin',(0.500000000000001,1.36481920536411E-16,
-6.345)) ;
#119928=CARTESIAN_POINT('Origin',(0.500000000000001,-2.9,-6.345)) ;
#119929=CARTESIAN_POINT('Origin',(-0.999999999999999,-2.9,-6.145)) ;
#119930=CARTESIAN_POINT('Origin',(0.500000000000001,-2.9,-6.145)) ;
#119931=CARTESIAN_POINT('Origin',(-1.1,1.15,-6.345)) ;
#119932=CARTESIAN_POINT('Origin',(-1.1,1.35,-6.345)) ;
#119933=CARTESIAN_POINT('Origin',(-1.1,1.15,-7.62)) ;
#119934=CARTESIAN_POINT('',(-1.1,1.25,-8.895)) ;
#119935=CARTESIAN_POINT('',(-1.1,1.25,-8.995)) ;
#119936=CARTESIAN_POINT('Origin',(-1.1,1.15,-8.895)) ;
#119937=CARTESIAN_POINT('Origin',(-0.899999999999999,-1.9,-8.12)) ;
#119938=CARTESIAN_POINT('Origin',(-0.899999999999999,-1.9,-8.895)) ;
#119939=CARTESIAN_POINT('Origin',(-0.999999999999999,-2.1,-8.895)) ;
#119940=CARTESIAN_POINT('Origin',(0.500000000000001,-2.1,-8.895)) ;
#119941=CARTESIAN_POINT('Origin',(-0.899999999999999,-2.1,-8.895)) ;
#119942=CARTESIAN_POINT('Origin',(0.500000000000001,-2.1,-8.895)) ;
#119943=CARTESIAN_POINT('Origin',(0.500000000000001,-2.1,-8.895)) ;
#119944=CARTESIAN_POINT('Origin',(0.500000000000001,-2.9,-6.345)) ;
#119945=CARTESIAN_POINT('Origin',(0.700000000000002,-2.9,-6.345)) ;
#119946=CARTESIAN_POINT('Origin',(-1.1,1.35,-8.995)) ;
#119947=CARTESIAN_POINT('Origin',(-1.1,1.35,-8.895)) ;
#119948=CARTESIAN_POINT('Origin',(-1.1,1.15,-8.895)) ;
#119949=CARTESIAN_POINT('',(-1.1,1.15,-8.995)) ;
#119950=CARTESIAN_POINT('Origin',(-1.1,1.15,-8.895)) ;
#119951=CARTESIAN_POINT('Origin',(-1.1,1.15,-8.895)) ;
#119952=CARTESIAN_POINT('Origin',(-0.899999999999999,-1.9,-8.895)) ;
#119953=CARTESIAN_POINT('Origin',(-1.1,-1.9,-8.895)) ;
#119954=CARTESIAN_POINT('Origin',(0.500000000000001,-5.86744705109802E-17,
-8.895)) ;
#119955=CARTESIAN_POINT('Origin',(0.500000000000001,-2.9,-8.895)) ;
#119956=CARTESIAN_POINT('Origin',(0.700000000000002,-2.9,-7.62)) ;
#119957=CARTESIAN_POINT('Origin',(0.700000000000002,-2.9,-8.895)) ;
#119958=CARTESIAN_POINT('Origin',(-1.1,1.15,-8.895)) ;
#119959=CARTESIAN_POINT('Origin',(-1.1,1.15,-9.095)) ;
#119960=CARTESIAN_POINT('Origin',(-1.1,-2.39429110547967E-16,-8.895)) ;
#119961=CARTESIAN_POINT('',(-1.1,1.25,-8.995)) ;
#119962=CARTESIAN_POINT('Origin',(0.500000000000001,-2.9,-8.895)) ;
#119963=CARTESIAN_POINT('Origin',(0.500000000000001,-2.9,-9.095)) ;
#119964=CARTESIAN_POINT('Origin',(-1.1,1.25,-9.095)) ;
#119965=CARTESIAN_POINT('Origin',(-1.1,-2.9,-9.095)) ;
#119966=CARTESIAN_POINT('Origin',(-1.1,-2.9,-9.095)) ;
#119967=CARTESIAN_POINT('Origin',(-1.1,-2.9,-9.095)) ;
#119968=CARTESIAN_POINT('Origin',(-1.1,-2.9,-9.095)) ;
#119969=CARTESIAN_POINT('Origin',(1.5,1.9,-7.02)) ;
#119970=CARTESIAN_POINT('Origin',(1.5,1.9,-9.17)) ;
#119971=CARTESIAN_POINT('Origin',(1.5,1.9,-8.22)) ;
#119972=CARTESIAN_POINT('Origin',(1.5,2.1,-8.22)) ;
#119973=CARTESIAN_POINT('Origin',(1.5,2.1,-8.02)) ;
#119974=CARTESIAN_POINT('Origin',(1.5,1.9,-9.17)) ;
#119975=CARTESIAN_POINT('Origin',(1.5,1.9,-9.17)) ;
#119976=CARTESIAN_POINT('Origin',(1.5,2.1,-8.02)) ;
#119977=CARTESIAN_POINT('Origin',(1.5,2.4,-8.02)) ;
#119978=CARTESIAN_POINT('Origin',(1.5,2.1,-9.17)) ;
#119979=CARTESIAN_POINT('Origin',(1.5,-2.15,-9.17)) ;
#119980=CARTESIAN_POINT('Origin',(1.5,2.4,-8.22)) ;
#119981=CARTESIAN_POINT('Origin',(1.5,2.6,-8.22)) ;
#119982=CARTESIAN_POINT('Origin',(1.5,-2.15,-9.17)) ;
#119983=CARTESIAN_POINT('Origin',(1.5,-2.15,-9.17)) ;
#119984=CARTESIAN_POINT('Origin',(1.5,2.6,-7.02)) ;
#119985=CARTESIAN_POINT('Origin',(1.5,2.6,-8.32857864376269)) ;
#119986=CARTESIAN_POINT('Origin',(1.5,-2.15,-7.02)) ;
#119987=CARTESIAN_POINT('Origin',(1.5,-2.15,-8.52311959340942)) ;
#119988=CARTESIAN_POINT('Origin',(1.5,2.6,-8.32857864376269)) ;
#119989=CARTESIAN_POINT('Origin',(1.5,2.6,-8.32857864376269)) ;
#119990=CARTESIAN_POINT('Origin',(1.5,-2.15,-8.52311959340942)) ;
#119991=CARTESIAN_POINT('Origin',(1.5,-2.15,-8.52311959340942)) ;
#119992=CARTESIAN_POINT('Origin',(1.5,1.69571067811865,-7.42428932188135)) ;
#119993=CARTESIAN_POINT('Origin',(1.5,3.15,-8.87857864376269)) ;
#119994=CARTESIAN_POINT('Origin',(1.5,-3.65625,-7.62)) ;
#119995=CARTESIAN_POINT('Origin',(1.5,-2.15,-6.71688040659058)) ;
#119996=CARTESIAN_POINT('Origin',(1.5,3.15,-8.87857864376269)) ;
#119997=CARTESIAN_POINT('Origin',(1.5,3.15,-8.87857864376269)) ;
#119998=CARTESIAN_POINT('Origin',(1.5,-2.15,-6.71688040659058)) ;
#119999=CARTESIAN_POINT('Origin',(1.5,-2.15,-6.71688040659058)) ;
#120000=CARTESIAN_POINT('Origin',(1.5,3.15,-7.02)) ;
#120001=CARTESIAN_POINT('Origin',(1.5,-2.15,-7.02)) ;
#120002=CARTESIAN_POINT('Origin',(1.5,-2.15,-6.07)) ;
#120003=CARTESIAN_POINT('Origin',(1.5,-2.15,-6.07)) ;
#120004=CARTESIAN_POINT('Origin',(1.5,-2.15,-6.07)) ;
#120005=CARTESIAN_POINT('Origin',(1.5,2.29571067811866,-7.21571067811866)) ;
#120006=CARTESIAN_POINT('Origin',(1.5,2.6,-6.91142135623731)) ;
#120007=CARTESIAN_POINT('Origin',(1.5,2.1,-6.07)) ;
#120008=CARTESIAN_POINT('Origin',(1.5,1.9,-6.07)) ;
#120009=CARTESIAN_POINT('Origin',(1.5,2.6,-6.91142135623731)) ;
#120010=CARTESIAN_POINT('Origin',(1.5,2.6,-6.91142135623731)) ;
#120011=CARTESIAN_POINT('Origin',(1.5,1.9,-6.07)) ;
#120012=CARTESIAN_POINT('Origin',(1.5,1.9,-6.07)) ;
#120013=CARTESIAN_POINT('Origin',(1.5,2.6,-7.02)) ;
#120014=CARTESIAN_POINT('Origin',(1.5,2.6,-7.02)) ;
#120015=CARTESIAN_POINT('Origin',(1.5,1.9,-7.02)) ;
#120016=CARTESIAN_POINT('Origin',(1.5,1.9,-7.02)) ;
#120017=CARTESIAN_POINT('Origin',(1.5,2.4,-7.02)) ;
#120018=CARTESIAN_POINT('Origin',(1.5,2.4,-7.22)) ;
#120019=CARTESIAN_POINT('Origin',(1.5,2.1,-7.02)) ;
#120020=CARTESIAN_POINT('Origin',(1.5,2.1,-7.22)) ;
#120021=CARTESIAN_POINT('Origin',(1.5,2.1,-7.22)) ;
#120022=CARTESIAN_POINT('Origin',(-0.899999999999999,-2.,-10.83)) ;
#120023=CARTESIAN_POINT('Origin',(-0.899999999999999,0.4,-10.83)) ;
#120024=CARTESIAN_POINT('Origin',(-0.899999999999999,-1.9,-10.83)) ;
#120025=CARTESIAN_POINT('Origin',(0.600000000000001,0.4,-11.03)) ;
#120026=CARTESIAN_POINT('Origin',(0.500000000000001,0.4,-11.03)) ;
#120027=CARTESIAN_POINT('Origin',(-0.899999999999999,0.4,-11.03)) ;
#120028=CARTESIAN_POINT('Origin',(0.500000000000001,0.4,-11.03)) ;
#120029=CARTESIAN_POINT('',(0.600000000000001,0.4,-11.03)) ;
#120030=CARTESIAN_POINT('Origin',(0.500000000000001,0.4,-11.03)) ;
#120031=CARTESIAN_POINT('Origin',(0.500000000000001,0.4,-11.03)) ;
#120032=CARTESIAN_POINT('Origin',(-0.899999999999999,-1.9,-10.83)) ;
#120033=CARTESIAN_POINT('Origin',(-0.899999999999999,-1.9,-10.83)) ;
#120034=CARTESIAN_POINT('Origin',(-0.899999999999999,-1.9,-10.83)) ;
#120035=CARTESIAN_POINT('Origin',(-0.899999999999999,0.4,-11.03)) ;
#120036=CARTESIAN_POINT('Origin',(-0.899999999999999,0.6,-11.03)) ;
#120037=CARTESIAN_POINT('Origin',(0.500000000000001,0.4,-11.43)) ;
#120038=CARTESIAN_POINT('Origin',(0.500000000000001,0.4,-11.83)) ;
#120039=CARTESIAN_POINT('',(0.600000000000001,0.4,-11.73)) ;
#120040=CARTESIAN_POINT('Ctrl Pts',(0.595612997216082,0.370705721320405,
-11.8007057213204)) ;
#120041=CARTESIAN_POINT('Ctrl Pts',(0.596180587760892,0.372558268494355,
-11.7988554988322)) ;
#120042=CARTESIAN_POINT('Ctrl Pts',(0.596672461925685,0.374355839771978,
-11.7969141798663)) ;
#120043=CARTESIAN_POINT('Ctrl Pts',(0.599015141889211,0.383869350930053,
-11.7857649936563)) ;
#120044=CARTESIAN_POINT('Ctrl Pts',(0.599609996542523,0.390224332900442,
-11.7749726026541)) ;
#120045=CARTESIAN_POINT('Ctrl Pts',(0.600050586298725,0.398117439141559,
-11.7523310532047)) ;
#120046=CARTESIAN_POINT('Ctrl Pts',(0.600000000000001,0.399999999999999,
-11.7412012506335)) ;
#120047=CARTESIAN_POINT('Ctrl Pts',(0.600000000000001,0.399999999999999,
-11.73)) ;
#120048=CARTESIAN_POINT('',(0.600000000000001,0.4,-11.43)) ;
#120049=CARTESIAN_POINT('Origin',(0.500000000000001,-4.56640444411542E-17,
-11.03)) ;
#120050=CARTESIAN_POINT('',(0.500000000000001,0.394987437106619,-11.13)) ;
#120051=CARTESIAN_POINT('Ctrl Pts',(0.500000000000001,0.394987437106619,
-11.13)) ;
#120052=CARTESIAN_POINT('Ctrl Pts',(0.505940567948954,0.395584486649901,
-11.13)) ;
#120053=CARTESIAN_POINT('Ctrl Pts',(0.511931971019137,0.396132036079018,
-11.129466300328)) ;
#120054=CARTESIAN_POINT('Ctrl Pts',(0.51782901530855,0.396618246075355,
-11.1283977957737)) ;
#120055=CARTESIAN_POINT('Ctrl Pts',(0.522982218721202,0.397043126556054,
-11.1274640701571)) ;
#120056=CARTESIAN_POINT('Ctrl Pts',(0.528062648970239,0.397421319341388,
-11.1261228267971)) ;
#120057=CARTESIAN_POINT('Ctrl Pts',(0.532978106724003,0.397751505046071,
-11.1244057438766)) ;
#120058=CARTESIAN_POINT('Ctrl Pts',(0.538583536338951,0.398128038182998,
-11.1224476378496)) ;
#120059=CARTESIAN_POINT('Ctrl Pts',(0.544059405914855,0.398447721828294,
-11.1199700083111)) ;
#120060=CARTESIAN_POINT('Ctrl Pts',(0.549268572255748,0.398712331108982,
-11.1170207319429)) ;
#120061=CARTESIAN_POINT('Ctrl Pts',(0.553856850427136,0.398945401221755,
-11.1144229841468)) ;
#120062=CARTESIAN_POINT('Ctrl Pts',(0.558237825069313,0.399135987683842,
-11.11146038498)) ;
#120063=CARTESIAN_POINT('Ctrl Pts',(0.562333836086205,0.399290378266507,
-11.1081952228642)) ;
#120064=CARTESIAN_POINT('Ctrl Pts',(0.566990328957881,0.399465895042381,
-11.1044832689523)) ;
#120065=CARTESIAN_POINT('Ctrl Pts',(0.571349096493411,0.399597278936107,
-11.1003228064848)) ;
#120066=CARTESIAN_POINT('Ctrl Pts',(0.575296920056702,0.399694832180837,
-11.0958055759794)) ;
#120067=CARTESIAN_POINT('Ctrl Pts',(0.578744263667896,0.399780018245913,
-11.0918610112151)) ;
#120068=CARTESIAN_POINT('Ctrl Pts',(0.581878314560452,0.399839626289636,
-11.0876455218421)) ;
#120069=CARTESIAN_POINT('Ctrl Pts',(0.584648147334861,0.399882153365958,
-11.0832418177073)) ;
#120070=CARTESIAN_POINT('Ctrl Pts',(0.587839270208171,0.399931148788079,
-11.0781683125045)) ;
#120071=CARTESIAN_POINT('Ctrl Pts',(0.590595054415094,0.399958289583404,
-11.0727666362445)) ;
#120072=CARTESIAN_POINT('Ctrl Pts',(0.59283861894311,0.399974357003159,
-11.0671616850094)) ;
#120073=CARTESIAN_POINT('Ctrl Pts',(0.594777336851653,0.399988241245861,
-11.0623183122424)) ;
#120074=CARTESIAN_POINT('Ctrl Pts',(0.596334051506183,0.399993946552814,
-11.0573241662271)) ;
#120075=CARTESIAN_POINT('Ctrl Pts',(0.597488309822303,0.39999684570125,
-11.0522717185684)) ;
#120076=CARTESIAN_POINT('Ctrl Pts',(0.598804024094406,0.400000150378306,
-11.0465125419605)) ;
#120077=CARTESIAN_POINT('Ctrl Pts',(0.599612685195435,0.399999963509465,
-11.0406028438906)) ;
#120078=CARTESIAN_POINT('Ctrl Pts',(0.599890230999722,0.399999993975383,
-11.034684202261)) ;
#120079=CARTESIAN_POINT('Ctrl Pts',(0.5999634645494,0.400000002014155,-11.0331225027898)) ;
#120080=CARTESIAN_POINT('Ctrl Pts',(0.600000000000001,0.399999999999999,
-11.0315602215092)) ;
#120081=CARTESIAN_POINT('Ctrl Pts',(0.600000000000001,0.399999999999999,
-11.03)) ;
#120082=CARTESIAN_POINT('',(0.600000000000001,0.299999999999999,-11.03)) ;
#120083=CARTESIAN_POINT('Ctrl Pts',(0.500000000000001,0.394987437106619,
-11.13)) ;
#120084=CARTESIAN_POINT('Ctrl Pts',(0.50045493559049,0.395033159853814,
-11.13)) ;
#120085=CARTESIAN_POINT('Ctrl Pts',(0.500909898680794,0.395078570329092,
-11.1299968954911)) ;
#120086=CARTESIAN_POINT('Ctrl Pts',(0.502892456245032,0.395275075889076,
-11.1299698339419)) ;
#120087=CARTESIAN_POINT('Ctrl Pts',(0.504418747482277,0.395422812032189,
-11.129913985421)) ;
#120088=CARTESIAN_POINT('Ctrl Pts',(0.508462199543281,0.395804395682027,
-11.1296732810566)) ;
#120089=CARTESIAN_POINT('Ctrl Pts',(0.510974953343229,0.396031485023311,
-11.1294279391451)) ;
#120090=CARTESIAN_POINT('Ctrl Pts',(0.521160739721084,0.396903453186219,
-11.1280427944916)) ;
#120091=CARTESIAN_POINT('Ctrl Pts',(0.528708678528227,0.397444933153154,
-11.1261042177048)) ;
#120092=CARTESIAN_POINT('Ctrl Pts',(0.545943206357832,0.398105551684098,
-11.1194646394512)) ;
#120093=CARTESIAN_POINT('Ctrl Pts',(0.555229535466621,0.397987646678464,
-11.1140353588361)) ;
#120094=CARTESIAN_POINT('Ctrl Pts',(0.571394604995555,0.395490482808064,
-11.100775513364)) ;
#120095=CARTESIAN_POINT('Ctrl Pts',(0.57805531370272,0.393198948698444,
-11.093240745632)) ;
#120096=CARTESIAN_POINT('Ctrl Pts',(0.588559132202387,0.385442756729392,
-11.0773922339842)) ;
#120097=CARTESIAN_POINT('Ctrl Pts',(0.592167355639922,0.380240075127053,
-11.069548265607)) ;
#120098=CARTESIAN_POINT('Ctrl Pts',(0.597496615531038,0.36589275346714,
-11.0539255217955)) ;
#120099=CARTESIAN_POINT('Ctrl Pts',(0.598734255154188,0.356660564300906,
-11.046772741727)) ;
#120100=CARTESIAN_POINT('Ctrl Pts',(0.60001275468167,0.335223914398785,
-11.0355823058657)) ;
#120101=CARTESIAN_POINT('Ctrl Pts',(0.59999390055981,0.322655037092193,
-11.0316615193656)) ;
#120102=CARTESIAN_POINT('Ctrl Pts',(0.600000296204999,0.30610691358234,
-11.030139626347)) ;
#120103=CARTESIAN_POINT('Ctrl Pts',(0.600000000000001,0.303050992413441,
-11.03)) ;
#120104=CARTESIAN_POINT('Ctrl Pts',(0.600000000000001,0.299999999999999,
-11.03)) ;
#120105=CARTESIAN_POINT('',(0.600000000000001,-2.39800009914441E-17,-11.03)) ;
#120106=CARTESIAN_POINT('Origin',(0.500000000000001,-1.9,-11.03)) ;
#120107=CARTESIAN_POINT('Origin',(0.600000000000001,-1.9,-10.83)) ;
#120108=CARTESIAN_POINT('Origin',(0.500000000000001,-1.9,-10.83)) ;
#120109=CARTESIAN_POINT('Origin',(-0.899999999999999,-1.9,-10.055)) ;
#120110=CARTESIAN_POINT('Origin',(-0.899999999999999,-1.9,-10.155)) ;
#120111=CARTESIAN_POINT('Origin',(-0.899999999999999,0.6,-10.93)) ;
#120112=CARTESIAN_POINT('Origin',(-0.899999999999999,0.6,-11.83)) ;
#120113=CARTESIAN_POINT('Origin',(0.600000000000001,0.4,-11.83)) ;
#120114=CARTESIAN_POINT('Origin',(0.500000000000001,0.4,-11.83)) ;
#120115=CARTESIAN_POINT('Origin',(-0.899999999999999,0.4,-11.83)) ;
#120116=CARTESIAN_POINT('Origin',(0.500000000000001,0.4,-11.83)) ;
#120117=CARTESIAN_POINT('Origin',(0.500000000000001,-1.9,-10.83)) ;
#120118=CARTESIAN_POINT('Origin',(0.500000000000001,-2.1,-10.83)) ;
#120119=CARTESIAN_POINT('Origin',(-0.899999999999999,-1.9,-10.155)) ;
#120120=CARTESIAN_POINT('Origin',(-1.1,-1.9,-10.155)) ;
#120121=CARTESIAN_POINT('Origin',(-0.899999999999999,-2.1,-10.155)) ;
#120122=CARTESIAN_POINT('Origin',(-0.899999999999999,0.4,-11.83)) ;
#120123=CARTESIAN_POINT('Origin',(-0.899999999999999,0.4,-12.03)) ;
#120124=CARTESIAN_POINT('Origin',(0.500000000000001,-2.1,-11.43)) ;
#120125=CARTESIAN_POINT('Origin',(0.500000000000001,-2.1,-10.155)) ;
#120126=CARTESIAN_POINT('Origin',(0.600000000000001,-2.1,-10.155)) ;
#120127=CARTESIAN_POINT('Origin',(0.500000000000001,-2.1,-10.155)) ;
#120128=CARTESIAN_POINT('Origin',(-1.1,-4.4272719500576E-17,-10.155)) ;
#120129=CARTESIAN_POINT('',(-1.1,1.15,-10.055)) ;
#120130=CARTESIAN_POINT('',(-1.1,1.25,-10.055)) ;
#120131=CARTESIAN_POINT('Origin',(-1.1,1.15,-10.155)) ;
#120132=CARTESIAN_POINT('Origin',(-0.899999999999999,0.5,-12.03)) ;
#120133=CARTESIAN_POINT('Origin',(-0.899999999999999,-1.9,-12.03)) ;
#120134=CARTESIAN_POINT('Origin',(0.600000000000001,-1.9,-12.03)) ;
#120135=CARTESIAN_POINT('Origin',(0.500000000000001,-1.9,-12.03)) ;
#120136=CARTESIAN_POINT('Origin',(-0.899999999999999,-1.9,-12.03)) ;
#120137=CARTESIAN_POINT('Origin',(0.500000000000001,-1.9,-12.03)) ;
#120138=CARTESIAN_POINT('Origin',(0.500000000000001,-2.1,-12.03)) ;
#120139=CARTESIAN_POINT('Origin',(0.500000000000001,-2.1,-10.155)) ;
#120140=CARTESIAN_POINT('Origin',(0.500000000000001,-2.1,-10.155)) ;
#120141=CARTESIAN_POINT('Origin',(-1.1,-2.9,-9.955)) ;
#120142=CARTESIAN_POINT('Origin',(-1.1,-2.9,-9.955)) ;
#120143=CARTESIAN_POINT('Origin',(-1.1,-2.9,-9.955)) ;
#120144=CARTESIAN_POINT('Origin',(-1.1,1.25,-9.955)) ;
#120145=CARTESIAN_POINT('Origin',(-1.1,1.15,-9.955)) ;
#120146=CARTESIAN_POINT('Origin',(-1.1,1.15,-10.155)) ;
#120147=CARTESIAN_POINT('',(-1.1,1.25,-10.155)) ;
#120148=CARTESIAN_POINT('Origin',(-1.1,1.15,-10.155)) ;
#120149=CARTESIAN_POINT('Origin',(-1.1,1.15,-10.155)) ;
#120150=CARTESIAN_POINT('Origin',(-0.899999999999999,-1.9,-12.03)) ;
#120151=CARTESIAN_POINT('Origin',(-0.899999999999999,-1.9,-12.03)) ;
#120152=CARTESIAN_POINT('Origin',(0.500000000000001,-2.1,-11.43)) ;
#120153=CARTESIAN_POINT('Origin',(0.500000000000001,-2.1,-12.705)) ;
#120154=CARTESIAN_POINT('Origin',(0.500000000000001,1.36481920536411E-16,
-10.155)) ;
#120155=CARTESIAN_POINT('Origin',(0.500000000000001,-2.9,-10.155)) ;
#120156=CARTESIAN_POINT('Origin',(-0.999999999999999,-2.9,-9.955)) ;
#120157=CARTESIAN_POINT('Origin',(0.500000000000001,-2.9,-9.955)) ;
#120158=CARTESIAN_POINT('Origin',(-1.1,1.15,-10.155)) ;
#120159=CARTESIAN_POINT('Origin',(-1.1,1.35,-10.155)) ;
#120160=CARTESIAN_POINT('Origin',(-1.1,1.15,-11.43)) ;
#120161=CARTESIAN_POINT('',(-1.1,1.25,-12.705)) ;
#120162=CARTESIAN_POINT('',(-1.1,1.25,-12.805)) ;
#120163=CARTESIAN_POINT('Origin',(-1.1,1.15,-12.705)) ;
#120164=CARTESIAN_POINT('Origin',(-0.899999999999999,-1.9,-11.93)) ;
#120165=CARTESIAN_POINT('Origin',(-0.899999999999999,-1.9,-12.705)) ;
#120166=CARTESIAN_POINT('Origin',(-0.999999999999999,-2.1,-12.705)) ;
#120167=CARTESIAN_POINT('Origin',(0.500000000000001,-2.1,-12.705)) ;
#120168=CARTESIAN_POINT('Origin',(-0.899999999999999,-2.1,-12.705)) ;
#120169=CARTESIAN_POINT('Origin',(0.500000000000001,-2.1,-12.705)) ;
#120170=CARTESIAN_POINT('Origin',(0.500000000000001,-2.1,-12.705)) ;
#120171=CARTESIAN_POINT('Origin',(0.500000000000001,-2.9,-10.155)) ;
#120172=CARTESIAN_POINT('Origin',(0.700000000000002,-2.9,-10.155)) ;
#120173=CARTESIAN_POINT('Origin',(-1.1,1.35,-12.805)) ;
#120174=CARTESIAN_POINT('Origin',(-1.1,1.35,-12.705)) ;
#120175=CARTESIAN_POINT('Origin',(-1.1,1.15,-12.705)) ;
#120176=CARTESIAN_POINT('',(-1.1,1.15,-12.805)) ;
#120177=CARTESIAN_POINT('Origin',(-1.1,1.15,-12.705)) ;
#120178=CARTESIAN_POINT('Origin',(-1.1,1.15,-12.705)) ;
#120179=CARTESIAN_POINT('Origin',(-0.899999999999999,-1.9,-12.705)) ;
#120180=CARTESIAN_POINT('Origin',(-1.1,-1.9,-12.705)) ;
#120181=CARTESIAN_POINT('Origin',(0.500000000000001,-5.86744705109802E-17,
-12.705)) ;
#120182=CARTESIAN_POINT('Origin',(0.500000000000001,-2.9,-12.705)) ;
#120183=CARTESIAN_POINT('Origin',(0.700000000000002,-2.9,-11.43)) ;
#120184=CARTESIAN_POINT('Origin',(0.700000000000002,-2.9,-12.705)) ;
#120185=CARTESIAN_POINT('Origin',(-1.1,1.15,-12.705)) ;
#120186=CARTESIAN_POINT('Origin',(-1.1,1.15,-12.905)) ;
#120187=CARTESIAN_POINT('Origin',(-1.1,-2.39429110547967E-16,-12.705)) ;
#120188=CARTESIAN_POINT('',(-1.1,1.25,-12.805)) ;
#120189=CARTESIAN_POINT('Origin',(0.500000000000001,-2.9,-12.705)) ;
#120190=CARTESIAN_POINT('Origin',(0.500000000000001,-2.9,-12.905)) ;
#120191=CARTESIAN_POINT('Origin',(-1.1,1.25,-12.905)) ;
#120192=CARTESIAN_POINT('Origin',(-1.1,-2.9,-12.905)) ;
#120193=CARTESIAN_POINT('Origin',(-1.1,-2.9,-12.905)) ;
#120194=CARTESIAN_POINT('Origin',(-1.1,-2.9,-12.905)) ;
#120195=CARTESIAN_POINT('Origin',(-1.1,-2.9,-12.905)) ;
#120196=CARTESIAN_POINT('Origin',(1.5,1.9,-10.83)) ;
#120197=CARTESIAN_POINT('Origin',(1.5,1.9,-12.98)) ;
#120198=CARTESIAN_POINT('Origin',(1.5,1.9,-12.03)) ;
#120199=CARTESIAN_POINT('Origin',(1.5,2.1,-12.03)) ;
#120200=CARTESIAN_POINT('Origin',(1.5,2.1,-11.83)) ;
#120201=CARTESIAN_POINT('Origin',(1.5,1.9,-12.98)) ;
#120202=CARTESIAN_POINT('Origin',(1.5,1.9,-12.98)) ;
#120203=CARTESIAN_POINT('Origin',(1.5,2.1,-11.83)) ;
#120204=CARTESIAN_POINT('Origin',(1.5,2.4,-11.83)) ;
#120205=CARTESIAN_POINT('Origin',(1.5,2.1,-12.98)) ;
#120206=CARTESIAN_POINT('Origin',(1.5,-2.15,-12.98)) ;
#120207=CARTESIAN_POINT('Origin',(1.5,2.4,-12.03)) ;
#120208=CARTESIAN_POINT('Origin',(1.5,2.6,-12.03)) ;
#120209=CARTESIAN_POINT('Origin',(1.5,-2.15,-12.98)) ;
#120210=CARTESIAN_POINT('Origin',(1.5,-2.15,-12.98)) ;
#120211=CARTESIAN_POINT('Origin',(1.5,2.6,-10.83)) ;
#120212=CARTESIAN_POINT('Origin',(1.5,2.6,-12.1385786437627)) ;
#120213=CARTESIAN_POINT('Origin',(1.5,-2.15,-10.83)) ;
#120214=CARTESIAN_POINT('Origin',(1.5,-2.15,-12.3331195934094)) ;
#120215=CARTESIAN_POINT('Origin',(1.5,2.6,-12.1385786437627)) ;
#120216=CARTESIAN_POINT('Origin',(1.5,2.6,-12.1385786437627)) ;
#120217=CARTESIAN_POINT('Origin',(1.5,-2.15,-12.3331195934094)) ;
#120218=CARTESIAN_POINT('Origin',(1.5,-2.15,-12.3331195934094)) ;
#120219=CARTESIAN_POINT('Origin',(1.5,1.69571067811865,-11.2342893218813)) ;
#120220=CARTESIAN_POINT('Origin',(1.5,3.15,-12.6885786437627)) ;
#120221=CARTESIAN_POINT('Origin',(1.5,-3.65625,-11.43)) ;
#120222=CARTESIAN_POINT('Origin',(1.5,-2.15,-10.5268804065906)) ;
#120223=CARTESIAN_POINT('Origin',(1.5,3.15,-12.6885786437627)) ;
#120224=CARTESIAN_POINT('Origin',(1.5,3.15,-12.6885786437627)) ;
#120225=CARTESIAN_POINT('Origin',(1.5,-2.15,-10.5268804065906)) ;
#120226=CARTESIAN_POINT('Origin',(1.5,-2.15,-10.5268804065906)) ;
#120227=CARTESIAN_POINT('Origin',(1.5,3.15,-10.83)) ;
#120228=CARTESIAN_POINT('Origin',(1.5,-2.15,-10.83)) ;
#120229=CARTESIAN_POINT('Origin',(1.5,-2.15,-9.88)) ;
#120230=CARTESIAN_POINT('Origin',(1.5,-2.15,-9.88)) ;
#120231=CARTESIAN_POINT('Origin',(1.5,-2.15,-9.88)) ;
#120232=CARTESIAN_POINT('Origin',(1.5,2.29571067811866,-11.0257106781187)) ;
#120233=CARTESIAN_POINT('Origin',(1.5,2.6,-10.7214213562373)) ;
#120234=CARTESIAN_POINT('Origin',(1.5,2.1,-9.88)) ;
#120235=CARTESIAN_POINT('Origin',(1.5,1.9,-9.88)) ;
#120236=CARTESIAN_POINT('Origin',(1.5,2.6,-10.7214213562373)) ;
#120237=CARTESIAN_POINT('Origin',(1.5,2.6,-10.7214213562373)) ;
#120238=CARTESIAN_POINT('Origin',(1.5,1.9,-9.88)) ;
#120239=CARTESIAN_POINT('Origin',(1.5,1.9,-9.88)) ;
#120240=CARTESIAN_POINT('Origin',(1.5,2.6,-10.83)) ;
#120241=CARTESIAN_POINT('Origin',(1.5,2.6,-10.83)) ;
#120242=CARTESIAN_POINT('Origin',(1.5,1.9,-10.83)) ;
#120243=CARTESIAN_POINT('Origin',(1.5,1.9,-10.83)) ;
#120244=CARTESIAN_POINT('Origin',(1.5,2.4,-10.83)) ;
#120245=CARTESIAN_POINT('Origin',(1.5,2.4,-11.03)) ;
#120246=CARTESIAN_POINT('Origin',(1.5,2.1,-10.83)) ;
#120247=CARTESIAN_POINT('Origin',(1.5,2.1,-11.03)) ;
#120248=CARTESIAN_POINT('Origin',(1.5,2.1,-11.03)) ;
#120249=CARTESIAN_POINT('Origin',(-0.899999999999999,-2.,-14.64)) ;
#120250=CARTESIAN_POINT('Origin',(-0.899999999999999,0.4,-14.64)) ;
#120251=CARTESIAN_POINT('Origin',(-0.899999999999999,-1.9,-14.64)) ;
#120252=CARTESIAN_POINT('Origin',(0.600000000000001,0.4,-14.84)) ;
#120253=CARTESIAN_POINT('Origin',(0.500000000000001,0.4,-14.84)) ;
#120254=CARTESIAN_POINT('Origin',(-0.899999999999999,0.4,-14.84)) ;
#120255=CARTESIAN_POINT('Origin',(0.500000000000001,0.4,-14.84)) ;
#120256=CARTESIAN_POINT('',(0.600000000000001,0.4,-14.84)) ;
#120257=CARTESIAN_POINT('Origin',(0.500000000000001,0.4,-14.84)) ;
#120258=CARTESIAN_POINT('Origin',(0.500000000000001,0.4,-14.84)) ;
#120259=CARTESIAN_POINT('Origin',(-0.899999999999999,-1.9,-14.64)) ;
#120260=CARTESIAN_POINT('Origin',(-0.899999999999999,-1.9,-14.64)) ;
#120261=CARTESIAN_POINT('Origin',(-0.899999999999999,-1.9,-14.64)) ;
#120262=CARTESIAN_POINT('Origin',(-0.899999999999999,0.4,-14.84)) ;
#120263=CARTESIAN_POINT('Origin',(-0.899999999999999,0.6,-14.84)) ;
#120264=CARTESIAN_POINT('Origin',(0.500000000000001,0.4,-15.24)) ;
#120265=CARTESIAN_POINT('Origin',(0.500000000000001,0.4,-15.64)) ;
#120266=CARTESIAN_POINT('',(0.600000000000001,0.4,-15.54)) ;
#120267=CARTESIAN_POINT('Ctrl Pts',(0.595612997216082,0.370705721320405,
-15.6107057213204)) ;
#120268=CARTESIAN_POINT('Ctrl Pts',(0.596180587760893,0.372558268494361,
-15.6088554988322)) ;
#120269=CARTESIAN_POINT('Ctrl Pts',(0.596672461925687,0.374355839771988,
-15.6069141798663)) ;
#120270=CARTESIAN_POINT('Ctrl Pts',(0.599015141889213,0.383869350930072,
-15.5957649936563)) ;
#120271=CARTESIAN_POINT('Ctrl Pts',(0.599609996542525,0.390224332900456,
-15.5849726026541)) ;
#120272=CARTESIAN_POINT('Ctrl Pts',(0.600050586298725,0.398117439141561,
-15.5623310532047)) ;
#120273=CARTESIAN_POINT('Ctrl Pts',(0.600000000000001,0.4,-15.5512012506335)) ;
#120274=CARTESIAN_POINT('Ctrl Pts',(0.600000000000001,0.399999999999999,
-15.54)) ;
#120275=CARTESIAN_POINT('',(0.600000000000001,0.4,-15.24)) ;
#120276=CARTESIAN_POINT('Origin',(0.500000000000001,-4.56640444411542E-17,
-14.84)) ;
#120277=CARTESIAN_POINT('',(0.500000000000001,0.394987437106619,-14.94)) ;
#120278=CARTESIAN_POINT('Ctrl Pts',(0.500000000000001,0.394987437106619,
-14.94)) ;
#120279=CARTESIAN_POINT('Ctrl Pts',(0.505940567948958,0.395584486649901,
-14.94)) ;
#120280=CARTESIAN_POINT('Ctrl Pts',(0.511931971019147,0.396132036079019,
-14.939466300328)) ;
#120281=CARTESIAN_POINT('Ctrl Pts',(0.517829015308562,0.396618246075356,
-14.9383977957737)) ;
#120282=CARTESIAN_POINT('Ctrl Pts',(0.522982218721209,0.397043126556054,
-14.9374640701571)) ;
#120283=CARTESIAN_POINT('Ctrl Pts',(0.528062648970245,0.397421319341388,
-14.9361228267971)) ;
#120284=CARTESIAN_POINT('Ctrl Pts',(0.532978106724004,0.397751505046071,
-14.9344057438766)) ;
#120285=CARTESIAN_POINT('Ctrl Pts',(0.538583536338963,0.398128038182999,
-14.9324476378495)) ;
#120286=CARTESIAN_POINT('Ctrl Pts',(0.544059405914874,0.398447721828296,
-14.9299700083111)) ;
#120287=CARTESIAN_POINT('Ctrl Pts',(0.549268572255776,0.398712331108984,
-14.9270207319429)) ;
#120288=CARTESIAN_POINT('Ctrl Pts',(0.553856850427151,0.398945401221756,
-14.9244229841468)) ;
#120289=CARTESIAN_POINT('Ctrl Pts',(0.558237825069319,0.399135987683843,
-14.92146038498)) ;
#120290=CARTESIAN_POINT('Ctrl Pts',(0.562333836086205,0.399290378266507,
-14.9181952228642)) ;
#120291=CARTESIAN_POINT('Ctrl Pts',(0.56699032895788,0.399465895042381,
-14.9144832689523)) ;
#120292=CARTESIAN_POINT('Ctrl Pts',(0.571349096493406,0.399597278936107,
-14.9103228064848)) ;
#120293=CARTESIAN_POINT('Ctrl Pts',(0.575296920056693,0.399694832180837,
-14.9058055759794)) ;
#120294=CARTESIAN_POINT('Ctrl Pts',(0.578744263667893,0.399780018245913,
-14.9018610112151)) ;
#120295=CARTESIAN_POINT('Ctrl Pts',(0.581878314560404,0.399839626289636,
-14.8976455218421)) ;
#120296=CARTESIAN_POINT('Ctrl Pts',(0.584648147334845,0.399882153365958,
-14.8932418177073)) ;
#120297=CARTESIAN_POINT('Ctrl Pts',(0.587839270208164,0.399931148788079,
-14.8881683125045)) ;
#120298=CARTESIAN_POINT('Ctrl Pts',(0.590595054415084,0.399958289583404,
-14.8827666362445)) ;
#120299=CARTESIAN_POINT('Ctrl Pts',(0.592838618943089,0.399974357003159,
-14.8771616850094)) ;
#120300=CARTESIAN_POINT('Ctrl Pts',(0.594777336851653,0.399988241245861,
-14.8723183122424)) ;
#120301=CARTESIAN_POINT('Ctrl Pts',(0.596334051506184,0.399993946552814,
-14.8673241662272)) ;
#120302=CARTESIAN_POINT('Ctrl Pts',(0.597488309822312,0.39999684570125,
-14.8622717185684)) ;
#120303=CARTESIAN_POINT('Ctrl Pts',(0.598804024094403,0.400000150378306,
-14.8565125419605)) ;
#120304=CARTESIAN_POINT('Ctrl Pts',(0.599612685195422,0.399999963509465,
-14.8506028438907)) ;
#120305=CARTESIAN_POINT('Ctrl Pts',(0.599890230999715,0.399999993975383,
-14.8446842022612)) ;
#120306=CARTESIAN_POINT('Ctrl Pts',(0.599963464549397,0.400000002014155,
-14.8431225027899)) ;
#120307=CARTESIAN_POINT('Ctrl Pts',(0.600000000000001,0.399999999999999,
-14.8415602215092)) ;
#120308=CARTESIAN_POINT('Ctrl Pts',(0.600000000000001,0.399999999999999,
-14.84)) ;
#120309=CARTESIAN_POINT('',(0.600000000000001,0.299999999999999,-14.84)) ;
#120310=CARTESIAN_POINT('Ctrl Pts',(0.500000000000001,0.394987437106619,
-14.94)) ;
#120311=CARTESIAN_POINT('Ctrl Pts',(0.500454935590171,0.395033159853782,
-14.94)) ;
#120312=CARTESIAN_POINT('Ctrl Pts',(0.500909898680634,0.395078570329076,
-14.9399968954911)) ;
#120313=CARTESIAN_POINT('Ctrl Pts',(0.502892456245054,0.395275075889078,
-14.9399698339419)) ;
#120314=CARTESIAN_POINT('Ctrl Pts',(0.504418747482298,0.395422812032191,
-14.939913985421)) ;
#120315=CARTESIAN_POINT('Ctrl Pts',(0.508462199543321,0.395804395682031,
-14.9396732810566)) ;
#120316=CARTESIAN_POINT('Ctrl Pts',(0.510974953343265,0.396031485023314,
-14.9394279391451)) ;
#120317=CARTESIAN_POINT('Ctrl Pts',(0.521160739721169,0.396903453186227,
-14.9380427944916)) ;
#120318=CARTESIAN_POINT('Ctrl Pts',(0.528708678528302,0.397444933153157,
-14.9361042177047)) ;
#120319=CARTESIAN_POINT('Ctrl Pts',(0.54594320635793,0.398105551684103,
-14.9294646394512)) ;
#120320=CARTESIAN_POINT('Ctrl Pts',(0.555229535466698,0.397987646678449,
-14.9240353588361)) ;
#120321=CARTESIAN_POINT('Ctrl Pts',(0.571394604995641,0.395490482808055,
-14.9107755133639)) ;
#120322=CARTESIAN_POINT('Ctrl Pts',(0.578055313702769,0.393198948698403,
-14.9032407456319)) ;
#120323=CARTESIAN_POINT('Ctrl Pts',(0.58855913220244,0.385442756729361,
-14.8873922339841)) ;
#120324=CARTESIAN_POINT('Ctrl Pts',(0.592167355639942,0.380240075126989,
-14.8795482656069)) ;
#120325=CARTESIAN_POINT('Ctrl Pts',(0.59749661553107,0.365892753467073,
-14.8639255217954)) ;
#120326=CARTESIAN_POINT('Ctrl Pts',(0.598734255154193,0.356660564300806,
-14.856772741727)) ;
#120327=CARTESIAN_POINT('Ctrl Pts',(0.600012754681677,0.335223914398739,
-14.8455823058657)) ;
#120328=CARTESIAN_POINT('Ctrl Pts',(0.59999390055981,0.322655037092125,
-14.8416615193656)) ;
#120329=CARTESIAN_POINT('Ctrl Pts',(0.600000296204999,0.306106913582367,
-14.840139626347)) ;
#120330=CARTESIAN_POINT('Ctrl Pts',(0.600000000000001,0.303050992413449,
-14.84)) ;
#120331=CARTESIAN_POINT('Ctrl Pts',(0.600000000000001,0.299999999999999,
-14.84)) ;
#120332=CARTESIAN_POINT('',(0.600000000000001,-2.39800009914441E-17,-14.84)) ;
#120333=CARTESIAN_POINT('Origin',(0.500000000000001,-1.9,-14.84)) ;
#120334=CARTESIAN_POINT('Origin',(0.600000000000001,-1.9,-14.64)) ;
#120335=CARTESIAN_POINT('Origin',(0.500000000000001,-1.9,-14.64)) ;
#120336=CARTESIAN_POINT('Origin',(-0.899999999999999,-1.9,-13.865)) ;
#120337=CARTESIAN_POINT('Origin',(-0.899999999999999,-1.9,-13.965)) ;
#120338=CARTESIAN_POINT('Origin',(-0.899999999999999,0.6,-14.74)) ;
#120339=CARTESIAN_POINT('Origin',(-0.899999999999999,0.6,-15.64)) ;
#120340=CARTESIAN_POINT('Origin',(0.600000000000001,0.4,-15.64)) ;
#120341=CARTESIAN_POINT('Origin',(0.500000000000001,0.4,-15.64)) ;
#120342=CARTESIAN_POINT('Origin',(-0.899999999999999,0.4,-15.64)) ;
#120343=CARTESIAN_POINT('Origin',(0.500000000000001,0.4,-15.64)) ;
#120344=CARTESIAN_POINT('Origin',(0.500000000000001,-1.9,-14.64)) ;
#120345=CARTESIAN_POINT('Origin',(0.500000000000001,-2.1,-14.64)) ;
#120346=CARTESIAN_POINT('Origin',(-0.899999999999999,-1.9,-13.965)) ;
#120347=CARTESIAN_POINT('Origin',(-1.1,-1.9,-13.965)) ;
#120348=CARTESIAN_POINT('Origin',(-0.899999999999999,-2.1,-13.965)) ;
#120349=CARTESIAN_POINT('Origin',(-0.899999999999999,0.4,-15.64)) ;
#120350=CARTESIAN_POINT('Origin',(-0.899999999999999,0.4,-15.84)) ;
#120351=CARTESIAN_POINT('Origin',(0.500000000000001,-2.1,-15.24)) ;
#120352=CARTESIAN_POINT('Origin',(0.500000000000001,-2.1,-13.965)) ;
#120353=CARTESIAN_POINT('Origin',(0.600000000000001,-2.1,-13.965)) ;
#120354=CARTESIAN_POINT('Origin',(0.500000000000001,-2.1,-13.965)) ;
#120355=CARTESIAN_POINT('Origin',(-1.1,-4.4272719500576E-17,-13.965)) ;
#120356=CARTESIAN_POINT('',(-1.1,1.15,-13.865)) ;
#120357=CARTESIAN_POINT('',(-1.1,1.25,-13.865)) ;
#120358=CARTESIAN_POINT('Origin',(-1.1,1.15,-13.965)) ;
#120359=CARTESIAN_POINT('Origin',(-0.899999999999999,0.5,-15.84)) ;
#120360=CARTESIAN_POINT('Origin',(-0.899999999999999,-1.9,-15.84)) ;
#120361=CARTESIAN_POINT('Origin',(0.600000000000001,-1.9,-15.84)) ;
#120362=CARTESIAN_POINT('Origin',(0.500000000000001,-1.9,-15.84)) ;
#120363=CARTESIAN_POINT('Origin',(-0.899999999999999,-1.9,-15.84)) ;
#120364=CARTESIAN_POINT('Origin',(0.500000000000001,-1.9,-15.84)) ;
#120365=CARTESIAN_POINT('Origin',(0.500000000000001,-2.1,-15.84)) ;
#120366=CARTESIAN_POINT('Origin',(0.500000000000001,-2.1,-13.965)) ;
#120367=CARTESIAN_POINT('Origin',(0.500000000000001,-2.1,-13.965)) ;
#120368=CARTESIAN_POINT('Origin',(-1.1,-2.9,-13.765)) ;
#120369=CARTESIAN_POINT('Origin',(-1.1,-2.9,-13.765)) ;
#120370=CARTESIAN_POINT('Origin',(-1.1,-2.9,-13.765)) ;
#120371=CARTESIAN_POINT('Origin',(-1.1,1.25,-13.765)) ;
#120372=CARTESIAN_POINT('Origin',(-1.1,1.15,-13.765)) ;
#120373=CARTESIAN_POINT('Origin',(-1.1,1.15,-13.965)) ;
#120374=CARTESIAN_POINT('',(-1.1,1.25,-13.965)) ;
#120375=CARTESIAN_POINT('Origin',(-1.1,1.15,-13.965)) ;
#120376=CARTESIAN_POINT('Origin',(-1.1,1.15,-13.965)) ;
#120377=CARTESIAN_POINT('Origin',(-0.899999999999999,-1.9,-15.84)) ;
#120378=CARTESIAN_POINT('Origin',(-0.899999999999999,-1.9,-15.84)) ;
#120379=CARTESIAN_POINT('Origin',(0.500000000000001,-2.1,-15.24)) ;
#120380=CARTESIAN_POINT('Origin',(0.500000000000001,-2.1,-16.515)) ;
#120381=CARTESIAN_POINT('Origin',(0.500000000000001,1.36481920536411E-16,
-13.965)) ;
#120382=CARTESIAN_POINT('Origin',(0.500000000000001,-2.9,-13.965)) ;
#120383=CARTESIAN_POINT('Origin',(-0.999999999999999,-2.9,-13.765)) ;
#120384=CARTESIAN_POINT('Origin',(0.500000000000001,-2.9,-13.765)) ;
#120385=CARTESIAN_POINT('Origin',(-1.1,1.15,-13.965)) ;
#120386=CARTESIAN_POINT('Origin',(-1.1,1.35,-13.965)) ;
#120387=CARTESIAN_POINT('Origin',(-1.1,1.15,-15.24)) ;
#120388=CARTESIAN_POINT('',(-1.1,1.25,-16.515)) ;
#120389=CARTESIAN_POINT('',(-1.1,1.25,-16.615)) ;
#120390=CARTESIAN_POINT('Origin',(-1.1,1.15,-16.515)) ;
#120391=CARTESIAN_POINT('Origin',(-0.899999999999999,-1.9,-15.74)) ;
#120392=CARTESIAN_POINT('Origin',(-0.899999999999999,-1.9,-16.515)) ;
#120393=CARTESIAN_POINT('Origin',(-0.999999999999999,-2.1,-16.515)) ;
#120394=CARTESIAN_POINT('Origin',(0.500000000000001,-2.1,-16.515)) ;
#120395=CARTESIAN_POINT('Origin',(-0.899999999999999,-2.1,-16.515)) ;
#120396=CARTESIAN_POINT('Origin',(0.500000000000001,-2.1,-16.515)) ;
#120397=CARTESIAN_POINT('Origin',(0.500000000000001,-2.1,-16.515)) ;
#120398=CARTESIAN_POINT('Origin',(0.500000000000001,-2.9,-13.965)) ;
#120399=CARTESIAN_POINT('Origin',(0.700000000000002,-2.9,-13.965)) ;
#120400=CARTESIAN_POINT('Origin',(-1.1,1.35,-16.615)) ;
#120401=CARTESIAN_POINT('Origin',(-1.1,1.35,-16.515)) ;
#120402=CARTESIAN_POINT('Origin',(-1.1,1.15,-16.515)) ;
#120403=CARTESIAN_POINT('',(-1.1,1.15,-16.615)) ;
#120404=CARTESIAN_POINT('Origin',(-1.1,1.15,-16.515)) ;
#120405=CARTESIAN_POINT('Origin',(-1.1,1.15,-16.515)) ;
#120406=CARTESIAN_POINT('Origin',(-0.899999999999999,-1.9,-16.515)) ;
#120407=CARTESIAN_POINT('Origin',(-1.1,-1.9,-16.515)) ;
#120408=CARTESIAN_POINT('Origin',(0.500000000000001,-5.86744705109802E-17,
-16.515)) ;
#120409=CARTESIAN_POINT('Origin',(0.500000000000001,-2.9,-16.515)) ;
#120410=CARTESIAN_POINT('Origin',(0.700000000000002,-2.9,-15.24)) ;
#120411=CARTESIAN_POINT('Origin',(0.700000000000002,-2.9,-16.515)) ;
#120412=CARTESIAN_POINT('Origin',(-1.1,1.15,-16.515)) ;
#120413=CARTESIAN_POINT('Origin',(-1.1,1.15,-16.715)) ;
#120414=CARTESIAN_POINT('Origin',(-1.1,-2.39429110547967E-16,-16.515)) ;
#120415=CARTESIAN_POINT('',(-1.1,1.25,-16.615)) ;
#120416=CARTESIAN_POINT('Origin',(0.500000000000001,-2.9,-16.515)) ;
#120417=CARTESIAN_POINT('Origin',(0.500000000000001,-2.9,-16.715)) ;
#120418=CARTESIAN_POINT('Origin',(-1.1,1.25,-16.715)) ;
#120419=CARTESIAN_POINT('Origin',(-1.1,-2.9,-16.715)) ;
#120420=CARTESIAN_POINT('Origin',(-1.1,-2.9,-16.715)) ;
#120421=CARTESIAN_POINT('Origin',(-1.1,-2.9,-16.715)) ;
#120422=CARTESIAN_POINT('Origin',(-1.1,-2.9,-16.715)) ;
#120423=CARTESIAN_POINT('Origin',(1.5,1.9,-14.64)) ;
#120424=CARTESIAN_POINT('Origin',(1.5,1.9,-16.79)) ;
#120425=CARTESIAN_POINT('Origin',(1.5,1.9,-15.84)) ;
#120426=CARTESIAN_POINT('Origin',(1.5,2.1,-15.84)) ;
#120427=CARTESIAN_POINT('Origin',(1.5,2.1,-15.64)) ;
#120428=CARTESIAN_POINT('Origin',(1.5,1.9,-16.79)) ;
#120429=CARTESIAN_POINT('Origin',(1.5,1.9,-16.79)) ;
#120430=CARTESIAN_POINT('Origin',(1.5,2.1,-15.64)) ;
#120431=CARTESIAN_POINT('Origin',(1.5,2.4,-15.64)) ;
#120432=CARTESIAN_POINT('Origin',(1.5,2.1,-16.79)) ;
#120433=CARTESIAN_POINT('Origin',(1.5,-2.15,-16.79)) ;
#120434=CARTESIAN_POINT('Origin',(1.5,2.4,-15.84)) ;
#120435=CARTESIAN_POINT('Origin',(1.5,2.6,-15.84)) ;
#120436=CARTESIAN_POINT('Origin',(1.5,-2.15,-16.79)) ;
#120437=CARTESIAN_POINT('Origin',(1.5,-2.15,-16.79)) ;
#120438=CARTESIAN_POINT('Origin',(1.5,2.6,-14.64)) ;
#120439=CARTESIAN_POINT('Origin',(1.5,2.6,-15.9485786437627)) ;
#120440=CARTESIAN_POINT('Origin',(1.5,-2.15,-14.64)) ;
#120441=CARTESIAN_POINT('Origin',(1.5,-2.15,-16.1431195934094)) ;
#120442=CARTESIAN_POINT('Origin',(1.5,2.6,-15.9485786437627)) ;
#120443=CARTESIAN_POINT('Origin',(1.5,2.6,-15.9485786437627)) ;
#120444=CARTESIAN_POINT('Origin',(1.5,-2.15,-16.1431195934094)) ;
#120445=CARTESIAN_POINT('Origin',(1.5,-2.15,-16.1431195934094)) ;
#120446=CARTESIAN_POINT('Origin',(1.5,1.69571067811865,-15.0442893218814)) ;
#120447=CARTESIAN_POINT('Origin',(1.5,3.15,-16.4985786437627)) ;
#120448=CARTESIAN_POINT('Origin',(1.5,-3.65625,-15.24)) ;
#120449=CARTESIAN_POINT('Origin',(1.5,-2.15,-14.3368804065906)) ;
#120450=CARTESIAN_POINT('Origin',(1.5,3.15,-16.4985786437627)) ;
#120451=CARTESIAN_POINT('Origin',(1.5,3.15,-16.4985786437627)) ;
#120452=CARTESIAN_POINT('Origin',(1.5,-2.15,-14.3368804065906)) ;
#120453=CARTESIAN_POINT('Origin',(1.5,-2.15,-14.3368804065906)) ;
#120454=CARTESIAN_POINT('Origin',(1.5,3.15,-14.64)) ;
#120455=CARTESIAN_POINT('Origin',(1.5,-2.15,-14.64)) ;
#120456=CARTESIAN_POINT('Origin',(1.5,-2.15,-13.69)) ;
#120457=CARTESIAN_POINT('Origin',(1.5,-2.15,-13.69)) ;
#120458=CARTESIAN_POINT('Origin',(1.5,-2.15,-13.69)) ;
#120459=CARTESIAN_POINT('Origin',(1.5,2.29571067811866,-14.8357106781187)) ;
#120460=CARTESIAN_POINT('Origin',(1.5,2.6,-14.5314213562373)) ;
#120461=CARTESIAN_POINT('Origin',(1.5,2.1,-13.69)) ;
#120462=CARTESIAN_POINT('Origin',(1.5,1.9,-13.69)) ;
#120463=CARTESIAN_POINT('Origin',(1.5,2.6,-14.5314213562373)) ;
#120464=CARTESIAN_POINT('Origin',(1.5,2.6,-14.5314213562373)) ;
#120465=CARTESIAN_POINT('Origin',(1.5,1.9,-13.69)) ;
#120466=CARTESIAN_POINT('Origin',(1.5,1.9,-13.69)) ;
#120467=CARTESIAN_POINT('Origin',(1.5,2.6,-14.64)) ;
#120468=CARTESIAN_POINT('Origin',(1.5,2.6,-14.64)) ;
#120469=CARTESIAN_POINT('Origin',(1.5,1.9,-14.64)) ;
#120470=CARTESIAN_POINT('Origin',(1.5,1.9,-14.64)) ;
#120471=CARTESIAN_POINT('Origin',(1.5,2.4,-14.64)) ;
#120472=CARTESIAN_POINT('Origin',(1.5,2.4,-14.84)) ;
#120473=CARTESIAN_POINT('Origin',(1.5,2.1,-14.64)) ;
#120474=CARTESIAN_POINT('Origin',(1.5,2.1,-14.84)) ;
#120475=CARTESIAN_POINT('Origin',(1.5,2.1,-14.84)) ;
#120476=CARTESIAN_POINT('Origin',(-0.899999999999999,-2.,-18.45)) ;
#120477=CARTESIAN_POINT('Origin',(-0.899999999999999,0.4,-18.45)) ;
#120478=CARTESIAN_POINT('Origin',(-0.899999999999999,-1.9,-18.45)) ;
#120479=CARTESIAN_POINT('Origin',(0.600000000000001,0.4,-18.65)) ;
#120480=CARTESIAN_POINT('Origin',(0.500000000000001,0.4,-18.65)) ;
#120481=CARTESIAN_POINT('Origin',(-0.899999999999999,0.4,-18.65)) ;
#120482=CARTESIAN_POINT('Origin',(0.500000000000001,0.4,-18.65)) ;
#120483=CARTESIAN_POINT('',(0.600000000000001,0.4,-18.65)) ;
#120484=CARTESIAN_POINT('Origin',(0.500000000000001,0.4,-18.65)) ;
#120485=CARTESIAN_POINT('Origin',(0.500000000000001,0.4,-18.65)) ;
#120486=CARTESIAN_POINT('Origin',(-0.899999999999999,-1.9,-18.45)) ;
#120487=CARTESIAN_POINT('Origin',(-0.899999999999999,-1.9,-18.45)) ;
#120488=CARTESIAN_POINT('Origin',(-0.899999999999999,-1.9,-18.45)) ;
#120489=CARTESIAN_POINT('Origin',(-0.899999999999999,0.4,-18.65)) ;
#120490=CARTESIAN_POINT('Origin',(-0.899999999999999,0.6,-18.65)) ;
#120491=CARTESIAN_POINT('Origin',(0.500000000000001,0.4,-19.05)) ;
#120492=CARTESIAN_POINT('Origin',(0.500000000000001,0.4,-19.45)) ;
#120493=CARTESIAN_POINT('',(0.600000000000001,0.4,-19.35)) ;
#120494=CARTESIAN_POINT('Ctrl Pts',(0.595612997216082,0.370705721320406,
-19.4207057213204)) ;
#120495=CARTESIAN_POINT('Ctrl Pts',(0.596180587760892,0.372558268494356,
-19.4188554988322)) ;
#120496=CARTESIAN_POINT('Ctrl Pts',(0.596672461925685,0.374355839771979,
-19.4169141798663)) ;
#120497=CARTESIAN_POINT('Ctrl Pts',(0.599015141889215,0.38386935093007,
-19.4057649936563)) ;
#120498=CARTESIAN_POINT('Ctrl Pts',(0.599609996542524,0.390224332900451,
-19.3949726026541)) ;
#120499=CARTESIAN_POINT('Ctrl Pts',(0.600050586298725,0.398117439141558,
-19.3723310532047)) ;
#120500=CARTESIAN_POINT('Ctrl Pts',(0.600000000000001,0.399999999999999,
-19.3612012506335)) ;
#120501=CARTESIAN_POINT('Ctrl Pts',(0.600000000000001,0.399999999999999,
-19.35)) ;
#120502=CARTESIAN_POINT('',(0.600000000000001,0.4,-19.05)) ;
#120503=CARTESIAN_POINT('Origin',(0.500000000000001,-4.56640444411542E-17,
-18.65)) ;
#120504=CARTESIAN_POINT('',(0.500000000000001,0.394987437106619,-18.75)) ;
#120505=CARTESIAN_POINT('Ctrl Pts',(0.500000000000001,0.394987437106619,
-18.75)) ;
#120506=CARTESIAN_POINT('Ctrl Pts',(0.505940567948962,0.395584486649901,
-18.75)) ;
#120507=CARTESIAN_POINT('Ctrl Pts',(0.511931971019156,0.39613203607902,
-18.749466300328)) ;
#120508=CARTESIAN_POINT('Ctrl Pts',(0.517829015308575,0.396618246075357,
-18.7483977957737)) ;
#120509=CARTESIAN_POINT('Ctrl Pts',(0.522982218721217,0.397043126556055,
-18.7474640701571)) ;
#120510=CARTESIAN_POINT('Ctrl Pts',(0.528062648970247,0.397421319341388,
-18.7461228267971)) ;
#120511=CARTESIAN_POINT('Ctrl Pts',(0.532978106724002,0.39775150504607,
-18.7444057438766)) ;
#120512=CARTESIAN_POINT('Ctrl Pts',(0.538583536338963,0.398128038182999,
-18.7424476378495)) ;
#120513=CARTESIAN_POINT('Ctrl Pts',(0.544059405914878,0.398447721828296,
-18.7399700083111)) ;
#120514=CARTESIAN_POINT('Ctrl Pts',(0.549268572255783,0.398712331108984,
-18.7370207319429)) ;
#120515=CARTESIAN_POINT('Ctrl Pts',(0.553856850427154,0.398945401221756,
-18.7344229841468)) ;
#120516=CARTESIAN_POINT('Ctrl Pts',(0.558237825069319,0.399135987683843,
-18.73146038498)) ;
#120517=CARTESIAN_POINT('Ctrl Pts',(0.5623338360862,0.399290378266507,-18.7281952228642)) ;
#120518=CARTESIAN_POINT('Ctrl Pts',(0.566990328957884,0.399465895042381,
-18.7244832689523)) ;
#120519=CARTESIAN_POINT('Ctrl Pts',(0.571349096493418,0.399597278936107,
-18.7203228064848)) ;
#120520=CARTESIAN_POINT('Ctrl Pts',(0.575296920056713,0.399694832180838,
-18.7158055759793)) ;
#120521=CARTESIAN_POINT('Ctrl Pts',(0.5787442636679,0.399780018245914,-18.7118610112151)) ;
#120522=CARTESIAN_POINT('Ctrl Pts',(0.581878314560451,0.399839626289636,
-18.7076455218421)) ;
#120523=CARTESIAN_POINT('Ctrl Pts',(0.584648147334859,0.399882153365958,
-18.7032418177073)) ;
#120524=CARTESIAN_POINT('Ctrl Pts',(0.587839270208173,0.399931148788079,
-18.6981683125045)) ;
#120525=CARTESIAN_POINT('Ctrl Pts',(0.590595054415093,0.399958289583404,
-18.6927666362444)) ;
#120526=CARTESIAN_POINT('Ctrl Pts',(0.59283861894311,0.399974357003159,
-18.6871616850094)) ;
#120527=CARTESIAN_POINT('Ctrl Pts',(0.594777336851653,0.399988241245861,
-18.6823183122424)) ;
#120528=CARTESIAN_POINT('Ctrl Pts',(0.596334051506184,0.399993946552814,
-18.6773241662271)) ;
#120529=CARTESIAN_POINT('Ctrl Pts',(0.597488309822305,0.39999684570125,
-18.6722717185684)) ;
#120530=CARTESIAN_POINT('Ctrl Pts',(0.598804024094405,0.400000150378306,
-18.6665125419605)) ;
#120531=CARTESIAN_POINT('Ctrl Pts',(0.599612685195428,0.399999963509465,
-18.6606028438907)) ;
#120532=CARTESIAN_POINT('Ctrl Pts',(0.59989023099972,0.399999993975383,
-18.6546842022611)) ;
#120533=CARTESIAN_POINT('Ctrl Pts',(0.5999634645494,0.400000002014155,-18.6531225027898)) ;
#120534=CARTESIAN_POINT('Ctrl Pts',(0.600000000000001,0.399999999999999,
-18.6515602215092)) ;
#120535=CARTESIAN_POINT('Ctrl Pts',(0.600000000000001,0.399999999999999,
-18.65)) ;
#120536=CARTESIAN_POINT('',(0.600000000000001,0.299999999999999,-18.65)) ;
#120537=CARTESIAN_POINT('Ctrl Pts',(0.500000000000001,0.394987437106619,
-18.75)) ;
#120538=CARTESIAN_POINT('Ctrl Pts',(0.500454935590171,0.395033159853782,
-18.75)) ;
#120539=CARTESIAN_POINT('Ctrl Pts',(0.500909898680634,0.395078570329076,
-18.7499968954911)) ;
#120540=CARTESIAN_POINT('Ctrl Pts',(0.502892456245054,0.395275075889078,
-18.7499698339419)) ;
#120541=CARTESIAN_POINT('Ctrl Pts',(0.504418747482298,0.395422812032191,
-18.749913985421)) ;
#120542=CARTESIAN_POINT('Ctrl Pts',(0.508462199543321,0.395804395682031,
-18.7496732810566)) ;
#120543=CARTESIAN_POINT('Ctrl Pts',(0.510974953343265,0.396031485023314,
-18.7494279391451)) ;
#120544=CARTESIAN_POINT('Ctrl Pts',(0.521160739721169,0.396903453186227,
-18.7480427944916)) ;
#120545=CARTESIAN_POINT('Ctrl Pts',(0.528708678528302,0.397444933153157,
-18.7461042177047)) ;
#120546=CARTESIAN_POINT('Ctrl Pts',(0.54594320635793,0.398105551684103,
-18.7394646394512)) ;
#120547=CARTESIAN_POINT('Ctrl Pts',(0.555229535466698,0.397987646678449,
-18.7340353588361)) ;
#120548=CARTESIAN_POINT('Ctrl Pts',(0.571394604995641,0.395490482808055,
-18.7207755133639)) ;
#120549=CARTESIAN_POINT('Ctrl Pts',(0.578055313702769,0.393198948698403,
-18.7132407456319)) ;
#120550=CARTESIAN_POINT('Ctrl Pts',(0.58855913220244,0.385442756729361,
-18.6973922339841)) ;
#120551=CARTESIAN_POINT('Ctrl Pts',(0.592167355639942,0.380240075126989,
-18.6895482656069)) ;
#120552=CARTESIAN_POINT('Ctrl Pts',(0.59749661553107,0.365892753467073,
-18.6739255217954)) ;
#120553=CARTESIAN_POINT('Ctrl Pts',(0.598734255154193,0.356660564300806,
-18.666772741727)) ;
#120554=CARTESIAN_POINT('Ctrl Pts',(0.600012754681677,0.335223914398739,
-18.6555823058657)) ;
#120555=CARTESIAN_POINT('Ctrl Pts',(0.59999390055981,0.322655037092125,
-18.6516615193656)) ;
#120556=CARTESIAN_POINT('Ctrl Pts',(0.600000296204999,0.306106913582367,
-18.650139626347)) ;
#120557=CARTESIAN_POINT('Ctrl Pts',(0.600000000000001,0.303050992413449,
-18.65)) ;
#120558=CARTESIAN_POINT('Ctrl Pts',(0.600000000000001,0.299999999999999,
-18.65)) ;
#120559=CARTESIAN_POINT('',(0.600000000000001,-2.39800009914441E-17,-18.65)) ;
#120560=CARTESIAN_POINT('Origin',(0.500000000000001,-1.9,-18.65)) ;
#120561=CARTESIAN_POINT('Origin',(0.600000000000001,-1.9,-18.45)) ;
#120562=CARTESIAN_POINT('Origin',(0.500000000000001,-1.9,-18.45)) ;
#120563=CARTESIAN_POINT('Origin',(-0.899999999999999,-1.9,-17.675)) ;
#120564=CARTESIAN_POINT('Origin',(-0.899999999999999,-1.9,-17.775)) ;
#120565=CARTESIAN_POINT('Origin',(-0.899999999999999,0.6,-18.55)) ;
#120566=CARTESIAN_POINT('Origin',(-0.899999999999999,0.6,-19.45)) ;
#120567=CARTESIAN_POINT('Origin',(0.600000000000001,0.4,-19.45)) ;
#120568=CARTESIAN_POINT('Origin',(0.500000000000001,0.4,-19.45)) ;
#120569=CARTESIAN_POINT('Origin',(-0.899999999999999,0.4,-19.45)) ;
#120570=CARTESIAN_POINT('Origin',(0.500000000000001,0.4,-19.45)) ;
#120571=CARTESIAN_POINT('Origin',(0.500000000000001,-1.9,-18.45)) ;
#120572=CARTESIAN_POINT('Origin',(0.500000000000001,-2.1,-18.45)) ;
#120573=CARTESIAN_POINT('Origin',(-0.899999999999999,-1.9,-17.775)) ;
#120574=CARTESIAN_POINT('Origin',(-1.1,-1.9,-17.775)) ;
#120575=CARTESIAN_POINT('Origin',(-0.899999999999999,-2.1,-17.775)) ;
#120576=CARTESIAN_POINT('Origin',(-0.899999999999999,0.4,-19.45)) ;
#120577=CARTESIAN_POINT('Origin',(-0.899999999999999,0.4,-19.65)) ;
#120578=CARTESIAN_POINT('Origin',(0.500000000000001,-2.1,-19.05)) ;
#120579=CARTESIAN_POINT('Origin',(0.500000000000001,-2.1,-17.775)) ;
#120580=CARTESIAN_POINT('Origin',(0.600000000000001,-2.1,-17.775)) ;
#120581=CARTESIAN_POINT('Origin',(0.500000000000001,-2.1,-17.775)) ;
#120582=CARTESIAN_POINT('Origin',(-1.1,-4.42727195005762E-17,-17.775)) ;
#120583=CARTESIAN_POINT('',(-1.1,1.15,-17.675)) ;
#120584=CARTESIAN_POINT('',(-1.1,1.25,-17.675)) ;
#120585=CARTESIAN_POINT('Origin',(-1.1,1.15,-17.775)) ;
#120586=CARTESIAN_POINT('Origin',(-0.899999999999999,0.5,-19.65)) ;
#120587=CARTESIAN_POINT('Origin',(-0.899999999999999,-1.9,-19.65)) ;
#120588=CARTESIAN_POINT('Origin',(0.600000000000001,-1.9,-19.65)) ;
#120589=CARTESIAN_POINT('Origin',(0.500000000000001,-1.9,-19.65)) ;
#120590=CARTESIAN_POINT('Origin',(-0.899999999999999,-1.9,-19.65)) ;
#120591=CARTESIAN_POINT('Origin',(0.500000000000001,-1.9,-19.65)) ;
#120592=CARTESIAN_POINT('Origin',(0.500000000000001,-2.1,-19.65)) ;
#120593=CARTESIAN_POINT('Origin',(0.500000000000001,-2.1,-17.775)) ;
#120594=CARTESIAN_POINT('Origin',(0.500000000000001,-2.1,-17.775)) ;
#120595=CARTESIAN_POINT('Origin',(-1.1,-2.9,-17.575)) ;
#120596=CARTESIAN_POINT('Origin',(-1.1,-2.9,-17.575)) ;
#120597=CARTESIAN_POINT('Origin',(-1.1,-2.9,-17.575)) ;
#120598=CARTESIAN_POINT('Origin',(-1.1,1.25,-17.575)) ;
#120599=CARTESIAN_POINT('Origin',(-1.1,1.15,-17.575)) ;
#120600=CARTESIAN_POINT('Origin',(-1.1,1.15,-17.775)) ;
#120601=CARTESIAN_POINT('',(-1.1,1.25,-17.775)) ;
#120602=CARTESIAN_POINT('Origin',(-1.1,1.15,-17.775)) ;
#120603=CARTESIAN_POINT('Origin',(-1.1,1.15,-17.775)) ;
#120604=CARTESIAN_POINT('Origin',(-0.899999999999999,-1.9,-19.65)) ;
#120605=CARTESIAN_POINT('Origin',(-0.899999999999999,-1.9,-19.65)) ;
#120606=CARTESIAN_POINT('Origin',(0.500000000000001,-2.1,-19.05)) ;
#120607=CARTESIAN_POINT('Origin',(0.500000000000001,-2.1,-20.325)) ;
#120608=CARTESIAN_POINT('Origin',(0.500000000000001,1.36481920536411E-16,
-17.775)) ;
#120609=CARTESIAN_POINT('Origin',(0.500000000000001,-2.9,-17.775)) ;
#120610=CARTESIAN_POINT('Origin',(-0.999999999999999,-2.9,-17.575)) ;
#120611=CARTESIAN_POINT('Origin',(0.500000000000001,-2.9,-17.575)) ;
#120612=CARTESIAN_POINT('Origin',(-1.1,1.15,-17.775)) ;
#120613=CARTESIAN_POINT('Origin',(-1.1,1.35,-17.775)) ;
#120614=CARTESIAN_POINT('Origin',(-1.1,1.15,-19.05)) ;
#120615=CARTESIAN_POINT('',(-1.1,1.25,-20.325)) ;
#120616=CARTESIAN_POINT('',(-1.1,1.25,-20.425)) ;
#120617=CARTESIAN_POINT('Origin',(-1.1,1.15,-20.325)) ;
#120618=CARTESIAN_POINT('Origin',(-0.899999999999999,-1.9,-19.55)) ;
#120619=CARTESIAN_POINT('Origin',(-0.899999999999999,-1.9,-20.325)) ;
#120620=CARTESIAN_POINT('Origin',(-0.999999999999999,-2.1,-20.325)) ;
#120621=CARTESIAN_POINT('Origin',(0.500000000000001,-2.1,-20.325)) ;
#120622=CARTESIAN_POINT('Origin',(-0.899999999999999,-2.1,-20.325)) ;
#120623=CARTESIAN_POINT('Origin',(0.500000000000001,-2.1,-20.325)) ;
#120624=CARTESIAN_POINT('Origin',(0.500000000000001,-2.1,-20.325)) ;
#120625=CARTESIAN_POINT('Origin',(0.500000000000001,-2.9,-17.775)) ;
#120626=CARTESIAN_POINT('Origin',(0.700000000000002,-2.9,-17.775)) ;
#120627=CARTESIAN_POINT('Origin',(-1.1,1.35,-20.425)) ;
#120628=CARTESIAN_POINT('Origin',(-1.1,1.35,-20.325)) ;
#120629=CARTESIAN_POINT('Origin',(-1.1,1.15,-20.325)) ;
#120630=CARTESIAN_POINT('',(-1.1,1.15,-20.425)) ;
#120631=CARTESIAN_POINT('Origin',(-1.1,1.15,-20.325)) ;
#120632=CARTESIAN_POINT('Origin',(-1.1,1.15,-20.325)) ;
#120633=CARTESIAN_POINT('Origin',(-0.899999999999999,-1.9,-20.325)) ;
#120634=CARTESIAN_POINT('Origin',(-1.1,-1.9,-20.325)) ;
#120635=CARTESIAN_POINT('Origin',(0.500000000000001,-5.86744705109802E-17,
-20.325)) ;
#120636=CARTESIAN_POINT('Origin',(0.500000000000001,-2.9,-20.325)) ;
#120637=CARTESIAN_POINT('Origin',(0.700000000000002,-2.9,-19.05)) ;
#120638=CARTESIAN_POINT('Origin',(0.700000000000002,-2.9,-20.325)) ;
#120639=CARTESIAN_POINT('Origin',(-1.1,1.15,-20.325)) ;
#120640=CARTESIAN_POINT('Origin',(-1.1,1.15,-20.525)) ;
#120641=CARTESIAN_POINT('Origin',(-1.1,-2.39429110547967E-16,-20.325)) ;
#120642=CARTESIAN_POINT('',(-1.1,1.25,-20.425)) ;
#120643=CARTESIAN_POINT('Origin',(0.500000000000001,-2.9,-20.325)) ;
#120644=CARTESIAN_POINT('Origin',(0.500000000000001,-2.9,-20.525)) ;
#120645=CARTESIAN_POINT('Origin',(-1.1,1.25,-20.525)) ;
#120646=CARTESIAN_POINT('Origin',(-1.1,-2.9,-20.525)) ;
#120647=CARTESIAN_POINT('Origin',(-1.1,-2.9,-20.525)) ;
#120648=CARTESIAN_POINT('Origin',(-1.1,-2.9,-20.525)) ;
#120649=CARTESIAN_POINT('Origin',(-1.1,-2.9,-20.525)) ;
#120650=CARTESIAN_POINT('Origin',(1.5,1.9,-18.45)) ;
#120651=CARTESIAN_POINT('Origin',(1.5,1.9,-20.6)) ;
#120652=CARTESIAN_POINT('Origin',(1.5,1.9,-19.65)) ;
#120653=CARTESIAN_POINT('Origin',(1.5,2.1,-19.65)) ;
#120654=CARTESIAN_POINT('Origin',(1.5,2.1,-19.45)) ;
#120655=CARTESIAN_POINT('Origin',(1.5,1.9,-20.6)) ;
#120656=CARTESIAN_POINT('Origin',(1.5,1.9,-20.6)) ;
#120657=CARTESIAN_POINT('Origin',(1.5,2.1,-19.45)) ;
#120658=CARTESIAN_POINT('Origin',(1.5,2.4,-19.45)) ;
#120659=CARTESIAN_POINT('Origin',(1.5,2.1,-20.6)) ;
#120660=CARTESIAN_POINT('Origin',(1.5,-2.15,-20.6)) ;
#120661=CARTESIAN_POINT('Origin',(1.5,2.4,-19.65)) ;
#120662=CARTESIAN_POINT('Origin',(1.5,2.6,-19.65)) ;
#120663=CARTESIAN_POINT('Origin',(1.5,-2.15,-20.6)) ;
#120664=CARTESIAN_POINT('Origin',(1.5,-2.15,-20.6)) ;
#120665=CARTESIAN_POINT('Origin',(1.5,2.6,-18.45)) ;
#120666=CARTESIAN_POINT('Origin',(1.5,2.6,-19.7585786437627)) ;
#120667=CARTESIAN_POINT('Origin',(1.5,-2.15,-18.45)) ;
#120668=CARTESIAN_POINT('Origin',(1.5,-2.15,-19.9531195934094)) ;
#120669=CARTESIAN_POINT('Origin',(1.5,2.6,-19.7585786437627)) ;
#120670=CARTESIAN_POINT('Origin',(1.5,2.6,-19.7585786437627)) ;
#120671=CARTESIAN_POINT('Origin',(1.5,-2.15,-19.9531195934094)) ;
#120672=CARTESIAN_POINT('Origin',(1.5,-2.15,-19.9531195934094)) ;
#120673=CARTESIAN_POINT('Origin',(1.5,1.69571067811865,-18.8542893218813)) ;
#120674=CARTESIAN_POINT('Origin',(1.5,3.15,-20.3085786437627)) ;
#120675=CARTESIAN_POINT('Origin',(1.5,-3.65625,-19.05)) ;
#120676=CARTESIAN_POINT('Origin',(1.5,-2.15,-18.1468804065906)) ;
#120677=CARTESIAN_POINT('Origin',(1.5,3.15,-20.3085786437627)) ;
#120678=CARTESIAN_POINT('Origin',(1.5,3.15,-20.3085786437627)) ;
#120679=CARTESIAN_POINT('Origin',(1.5,-2.15,-18.1468804065906)) ;
#120680=CARTESIAN_POINT('Origin',(1.5,-2.15,-18.1468804065906)) ;
#120681=CARTESIAN_POINT('Origin',(1.5,3.15,-18.45)) ;
#120682=CARTESIAN_POINT('Origin',(1.5,-2.15,-18.45)) ;
#120683=CARTESIAN_POINT('Origin',(1.5,-2.15,-17.5)) ;
#120684=CARTESIAN_POINT('Origin',(1.5,-2.15,-17.5)) ;
#120685=CARTESIAN_POINT('Origin',(1.5,-2.15,-17.5)) ;
#120686=CARTESIAN_POINT('Origin',(1.5,2.29571067811866,-18.6457106781187)) ;
#120687=CARTESIAN_POINT('Origin',(1.5,2.6,-18.3414213562373)) ;
#120688=CARTESIAN_POINT('Origin',(1.5,2.1,-17.5)) ;
#120689=CARTESIAN_POINT('Origin',(1.5,1.9,-17.5)) ;
#120690=CARTESIAN_POINT('Origin',(1.5,2.6,-18.3414213562373)) ;
#120691=CARTESIAN_POINT('Origin',(1.5,2.6,-18.3414213562373)) ;
#120692=CARTESIAN_POINT('Origin',(1.5,1.9,-17.5)) ;
#120693=CARTESIAN_POINT('Origin',(1.5,1.9,-17.5)) ;
#120694=CARTESIAN_POINT('Origin',(1.5,2.6,-18.45)) ;
#120695=CARTESIAN_POINT('Origin',(1.5,2.6,-18.45)) ;
#120696=CARTESIAN_POINT('Origin',(1.5,1.9,-18.45)) ;
#120697=CARTESIAN_POINT('Origin',(1.5,1.9,-18.45)) ;
#120698=CARTESIAN_POINT('Origin',(1.5,2.4,-18.45)) ;
#120699=CARTESIAN_POINT('Origin',(1.5,2.4,-18.65)) ;
#120700=CARTESIAN_POINT('Origin',(1.5,2.1,-18.45)) ;
#120701=CARTESIAN_POINT('Origin',(1.5,2.1,-18.65)) ;
#120702=CARTESIAN_POINT('Origin',(1.5,2.1,-18.65)) ;
#120703=CARTESIAN_POINT('Origin',(-0.899999999999999,-2.,-22.26)) ;
#120704=CARTESIAN_POINT('Origin',(-0.899999999999999,0.4,-22.26)) ;
#120705=CARTESIAN_POINT('Origin',(-0.899999999999999,-1.9,-22.26)) ;
#120706=CARTESIAN_POINT('Origin',(0.600000000000001,0.4,-22.46)) ;
#120707=CARTESIAN_POINT('Origin',(0.500000000000001,0.4,-22.46)) ;
#120708=CARTESIAN_POINT('Origin',(-0.899999999999999,0.4,-22.46)) ;
#120709=CARTESIAN_POINT('Origin',(0.500000000000001,0.4,-22.46)) ;
#120710=CARTESIAN_POINT('',(0.600000000000001,0.4,-22.46)) ;
#120711=CARTESIAN_POINT('Origin',(0.500000000000001,0.4,-22.46)) ;
#120712=CARTESIAN_POINT('Origin',(0.500000000000001,0.4,-22.46)) ;
#120713=CARTESIAN_POINT('Origin',(-0.899999999999999,-1.9,-22.26)) ;
#120714=CARTESIAN_POINT('Origin',(-0.899999999999999,-1.9,-22.26)) ;
#120715=CARTESIAN_POINT('Origin',(-0.899999999999999,-1.9,-22.26)) ;
#120716=CARTESIAN_POINT('Origin',(-0.899999999999999,0.4,-22.46)) ;
#120717=CARTESIAN_POINT('Origin',(-0.899999999999999,0.6,-22.46)) ;
#120718=CARTESIAN_POINT('Origin',(0.500000000000001,0.4,-22.86)) ;
#120719=CARTESIAN_POINT('Origin',(0.500000000000001,0.4,-23.26)) ;
#120720=CARTESIAN_POINT('',(0.600000000000001,0.4,-23.16)) ;
#120721=CARTESIAN_POINT('Ctrl Pts',(0.595612997216081,0.370705721320404,
-23.2307057213204)) ;
#120722=CARTESIAN_POINT('Ctrl Pts',(0.596180587760893,0.372558268494359,
-23.2288554988322)) ;
#120723=CARTESIAN_POINT('Ctrl Pts',(0.596672461925686,0.374355839771986,
-23.2269141798663)) ;
#120724=CARTESIAN_POINT('Ctrl Pts',(0.599015141889206,0.38386935093004,
-23.2157649936563)) ;
#120725=CARTESIAN_POINT('Ctrl Pts',(0.599609996542524,0.390224332900438,
-23.2049726026542)) ;
#120726=CARTESIAN_POINT('Ctrl Pts',(0.600050586298726,0.398117439141562,
-23.1823310532047)) ;
#120727=CARTESIAN_POINT('Ctrl Pts',(0.600000000000001,0.4,-23.1712012506335)) ;
#120728=CARTESIAN_POINT('Ctrl Pts',(0.600000000000001,0.399999999999999,
-23.16)) ;
#120729=CARTESIAN_POINT('',(0.600000000000001,0.4,-22.86)) ;
#120730=CARTESIAN_POINT('Origin',(0.500000000000001,-4.56640444411542E-17,
-22.46)) ;
#120731=CARTESIAN_POINT('',(0.500000000000001,0.394987437106619,-22.56)) ;
#120732=CARTESIAN_POINT('Ctrl Pts',(0.500000000000001,0.394987437106619,
-22.56)) ;
#120733=CARTESIAN_POINT('Ctrl Pts',(0.50594056794894,0.395584486649899,
-22.56)) ;
#120734=CARTESIAN_POINT('Ctrl Pts',(0.511931971019111,0.396132036079016,
-22.559466300328)) ;
#120735=CARTESIAN_POINT('Ctrl Pts',(0.517829015308511,0.396618246075352,
-22.5583977957737)) ;
#120736=CARTESIAN_POINT('Ctrl Pts',(0.522982218721178,0.397043126556052,
-22.5574640701571)) ;
#120737=CARTESIAN_POINT('Ctrl Pts',(0.528062648970232,0.397421319341387,
-22.5561228267971)) ;
#120738=CARTESIAN_POINT('Ctrl Pts',(0.532978106724004,0.397751505046071,
-22.5544057438766)) ;
#120739=CARTESIAN_POINT('Ctrl Pts',(0.538583536338997,0.398128038183002,
-22.5524476378495)) ;
#120740=CARTESIAN_POINT('Ctrl Pts',(0.544059405914977,0.3984477218283,-22.549970008311)) ;
#120741=CARTESIAN_POINT('Ctrl Pts',(0.549268572255885,0.398712331108989,
-22.5470207319428)) ;
#120742=CARTESIAN_POINT('Ctrl Pts',(0.553856850427199,0.398945401221759,
-22.5444229841468)) ;
#120743=CARTESIAN_POINT('Ctrl Pts',(0.558237825069336,0.399135987683844,
-22.54146038498)) ;
#120744=CARTESIAN_POINT('Ctrl Pts',(0.562333836086193,0.399290378266507,
-22.5381952228642)) ;
#120745=CARTESIAN_POINT('Ctrl Pts',(0.56699032895789,0.399465895042382,
-22.5344832689523)) ;
#120746=CARTESIAN_POINT('Ctrl Pts',(0.571349096493477,0.399597278936108,
-22.5303228064847)) ;
#120747=CARTESIAN_POINT('Ctrl Pts',(0.575296920056774,0.399694832180838,
-22.5258055759793)) ;
#120748=CARTESIAN_POINT('Ctrl Pts',(0.578744263667953,0.399780018245914,
-22.521861011215)) ;
#120749=CARTESIAN_POINT('Ctrl Pts',(0.581878314560456,0.399839626289636,
-22.5176455218421)) ;
#120750=CARTESIAN_POINT('Ctrl Pts',(0.584648147334871,0.399882153365958,
-22.5132418177073)) ;
#120751=CARTESIAN_POINT('Ctrl Pts',(0.587839270208222,0.39993114878808,
-22.5081683125044)) ;
#120752=CARTESIAN_POINT('Ctrl Pts',(0.590595054415142,0.399958289583405,
-22.5027666362444)) ;
#120753=CARTESIAN_POINT('Ctrl Pts',(0.592838618943166,0.39997435700316,
-22.4971616850092)) ;
#120754=CARTESIAN_POINT('Ctrl Pts',(0.594777336851685,0.399988241245861,
-22.4923183122423)) ;
#120755=CARTESIAN_POINT('Ctrl Pts',(0.596334051506206,0.399993946552814,
-22.4873241662271)) ;
#120756=CARTESIAN_POINT('Ctrl Pts',(0.59748830982231,0.39999684570125,-22.4822717185684)) ;
#120757=CARTESIAN_POINT('Ctrl Pts',(0.598804024094403,0.400000150378306,
-22.4765125419605)) ;
#120758=CARTESIAN_POINT('Ctrl Pts',(0.599612685195435,0.399999963509465,
-22.4706028438905)) ;
#120759=CARTESIAN_POINT('Ctrl Pts',(0.599890230999722,0.399999993975383,
-22.4646842022611)) ;
#120760=CARTESIAN_POINT('Ctrl Pts',(0.5999634645494,0.400000002014155,-22.4631225027898)) ;
#120761=CARTESIAN_POINT('Ctrl Pts',(0.600000000000001,0.399999999999999,
-22.4615602215092)) ;
#120762=CARTESIAN_POINT('Ctrl Pts',(0.600000000000001,0.399999999999999,
-22.46)) ;
#120763=CARTESIAN_POINT('',(0.600000000000001,0.299999999999999,-22.46)) ;
#120764=CARTESIAN_POINT('Ctrl Pts',(0.500000000000001,0.394987437106619,
-22.56)) ;
#120765=CARTESIAN_POINT('Ctrl Pts',(0.50045493558952,0.395033159853717,
-22.56)) ;
#120766=CARTESIAN_POINT('Ctrl Pts',(0.50090989868031,0.395078570329044,
-22.5599968954911)) ;
#120767=CARTESIAN_POINT('Ctrl Pts',(0.502892456245184,0.395275075889091,
-22.5599698339419)) ;
#120768=CARTESIAN_POINT('Ctrl Pts',(0.504418747482384,0.395422812032199,
-22.559913985421)) ;
#120769=CARTESIAN_POINT('Ctrl Pts',(0.508462199543371,0.395804395682036,
-22.5596732810566)) ;
#120770=CARTESIAN_POINT('Ctrl Pts',(0.510974953343326,0.396031485023319,
-22.5594279391451)) ;
#120771=CARTESIAN_POINT('Ctrl Pts',(0.521160739721382,0.396903453186245,
-22.5580427944915)) ;
#120772=CARTESIAN_POINT('Ctrl Pts',(0.528708678528517,0.397444933153166,
-22.5561042177046)) ;
#120773=CARTESIAN_POINT('Ctrl Pts',(0.545943206358243,0.398105551684114,
-22.5494646394511)) ;
#120774=CARTESIAN_POINT('Ctrl Pts',(0.555229535466965,0.397987646678414,
-22.5440353588359)) ;
#120775=CARTESIAN_POINT('Ctrl Pts',(0.57139460499589,0.395490482808011,
-22.5307755133637)) ;
#120776=CARTESIAN_POINT('Ctrl Pts',(0.578055313702948,0.393198948698283,
-22.5232407456316)) ;
#120777=CARTESIAN_POINT('Ctrl Pts',(0.588559132202604,0.385442756729229,
-22.5073922339839)) ;
#120778=CARTESIAN_POINT('Ctrl Pts',(0.592167355640029,0.380240075126779,
-22.4995482656067)) ;
#120779=CARTESIAN_POINT('Ctrl Pts',(0.597496615531157,0.365892753466814,
-22.4839255217951)) ;
#120780=CARTESIAN_POINT('Ctrl Pts',(0.598734255154217,0.35666056430046,
-22.4767727417268)) ;
#120781=CARTESIAN_POINT('Ctrl Pts',(0.600012754681695,0.335223914398355,
-22.4655823058655)) ;
#120782=CARTESIAN_POINT('Ctrl Pts',(0.59999390055981,0.322655037091671,
-22.4616615193655)) ;
#120783=CARTESIAN_POINT('Ctrl Pts',(0.600000296204999,0.306106913582289,
-22.460139626347)) ;
#120784=CARTESIAN_POINT('Ctrl Pts',(0.600000000000001,0.303050992413402,
-22.46)) ;
#120785=CARTESIAN_POINT('Ctrl Pts',(0.600000000000001,0.299999999999999,
-22.46)) ;
#120786=CARTESIAN_POINT('',(0.600000000000001,-2.39800009914441E-17,-22.46)) ;
#120787=CARTESIAN_POINT('Origin',(0.500000000000001,-1.9,-22.46)) ;
#120788=CARTESIAN_POINT('Origin',(0.600000000000001,-1.9,-22.26)) ;
#120789=CARTESIAN_POINT('Origin',(0.500000000000001,-1.9,-22.26)) ;
#120790=CARTESIAN_POINT('Origin',(-0.899999999999999,-1.9,-21.485)) ;
#120791=CARTESIAN_POINT('Origin',(-0.899999999999999,-1.9,-21.585)) ;
#120792=CARTESIAN_POINT('Origin',(-0.899999999999999,0.6,-22.36)) ;
#120793=CARTESIAN_POINT('Origin',(-0.899999999999999,0.6,-23.26)) ;
#120794=CARTESIAN_POINT('Origin',(0.600000000000001,0.4,-23.26)) ;
#120795=CARTESIAN_POINT('Origin',(0.500000000000001,0.4,-23.26)) ;
#120796=CARTESIAN_POINT('Origin',(-0.899999999999999,0.4,-23.26)) ;
#120797=CARTESIAN_POINT('Origin',(0.500000000000001,0.4,-23.26)) ;
#120798=CARTESIAN_POINT('Origin',(0.500000000000001,-1.9,-22.26)) ;
#120799=CARTESIAN_POINT('Origin',(0.500000000000001,-2.1,-22.26)) ;
#120800=CARTESIAN_POINT('Origin',(-0.899999999999999,-1.9,-21.585)) ;
#120801=CARTESIAN_POINT('Origin',(-1.1,-1.9,-21.585)) ;
#120802=CARTESIAN_POINT('Origin',(-0.899999999999999,-2.1,-21.585)) ;
#120803=CARTESIAN_POINT('Origin',(-0.899999999999999,0.4,-23.26)) ;
#120804=CARTESIAN_POINT('Origin',(-0.899999999999999,0.4,-23.46)) ;
#120805=CARTESIAN_POINT('Origin',(0.500000000000001,-2.1,-22.86)) ;
#120806=CARTESIAN_POINT('Origin',(0.500000000000001,-2.1,-21.585)) ;
#120807=CARTESIAN_POINT('Origin',(0.600000000000001,-2.1,-21.585)) ;
#120808=CARTESIAN_POINT('Origin',(0.500000000000001,-2.1,-21.585)) ;
#120809=CARTESIAN_POINT('Origin',(-1.1,-4.42727195005762E-17,-21.585)) ;
#120810=CARTESIAN_POINT('',(-1.1,1.15,-21.485)) ;
#120811=CARTESIAN_POINT('',(-1.1,1.25,-21.485)) ;
#120812=CARTESIAN_POINT('Origin',(-1.1,1.15,-21.585)) ;
#120813=CARTESIAN_POINT('Origin',(-0.899999999999999,0.5,-23.46)) ;
#120814=CARTESIAN_POINT('Origin',(-0.899999999999999,-1.9,-23.46)) ;
#120815=CARTESIAN_POINT('Origin',(0.600000000000001,-1.9,-23.46)) ;
#120816=CARTESIAN_POINT('Origin',(0.500000000000001,-1.9,-23.46)) ;
#120817=CARTESIAN_POINT('Origin',(-0.899999999999999,-1.9,-23.46)) ;
#120818=CARTESIAN_POINT('Origin',(0.500000000000001,-1.9,-23.46)) ;
#120819=CARTESIAN_POINT('Origin',(0.500000000000001,-2.1,-23.46)) ;
#120820=CARTESIAN_POINT('Origin',(0.500000000000001,-2.1,-21.585)) ;
#120821=CARTESIAN_POINT('Origin',(0.500000000000001,-2.1,-21.585)) ;
#120822=CARTESIAN_POINT('Origin',(-1.1,-2.9,-21.385)) ;
#120823=CARTESIAN_POINT('Origin',(-1.1,-2.9,-21.385)) ;
#120824=CARTESIAN_POINT('Origin',(-1.1,-2.9,-21.385)) ;
#120825=CARTESIAN_POINT('Origin',(-1.1,1.25,-21.385)) ;
#120826=CARTESIAN_POINT('Origin',(-1.1,1.15,-21.385)) ;
#120827=CARTESIAN_POINT('Origin',(-1.1,1.15,-21.585)) ;
#120828=CARTESIAN_POINT('',(-1.1,1.25,-21.585)) ;
#120829=CARTESIAN_POINT('Origin',(-1.1,1.15,-21.585)) ;
#120830=CARTESIAN_POINT('Origin',(-1.1,1.15,-21.585)) ;
#120831=CARTESIAN_POINT('Origin',(-0.899999999999999,-1.9,-23.46)) ;
#120832=CARTESIAN_POINT('Origin',(-0.899999999999999,-1.9,-23.46)) ;
#120833=CARTESIAN_POINT('Origin',(0.500000000000001,-2.1,-22.86)) ;
#120834=CARTESIAN_POINT('Origin',(0.500000000000001,-2.1,-24.135)) ;
#120835=CARTESIAN_POINT('Origin',(0.500000000000001,1.36481920536411E-16,
-21.585)) ;
#120836=CARTESIAN_POINT('Origin',(0.500000000000001,-2.9,-21.585)) ;
#120837=CARTESIAN_POINT('Origin',(-0.999999999999999,-2.9,-21.385)) ;
#120838=CARTESIAN_POINT('Origin',(0.500000000000001,-2.9,-21.385)) ;
#120839=CARTESIAN_POINT('Origin',(-1.1,1.15,-21.585)) ;
#120840=CARTESIAN_POINT('Origin',(-1.1,1.35,-21.585)) ;
#120841=CARTESIAN_POINT('Origin',(-1.1,1.15,-22.86)) ;
#120842=CARTESIAN_POINT('',(-1.1,1.25,-24.135)) ;
#120843=CARTESIAN_POINT('',(-1.1,1.25,-24.235)) ;
#120844=CARTESIAN_POINT('Origin',(-1.1,1.15,-24.135)) ;
#120845=CARTESIAN_POINT('Origin',(-0.899999999999999,-1.9,-23.36)) ;
#120846=CARTESIAN_POINT('Origin',(-0.899999999999999,-1.9,-24.135)) ;
#120847=CARTESIAN_POINT('Origin',(-0.999999999999999,-2.1,-24.135)) ;
#120848=CARTESIAN_POINT('Origin',(0.500000000000001,-2.1,-24.135)) ;
#120849=CARTESIAN_POINT('Origin',(-0.899999999999999,-2.1,-24.135)) ;
#120850=CARTESIAN_POINT('Origin',(0.500000000000001,-2.1,-24.135)) ;
#120851=CARTESIAN_POINT('Origin',(0.500000000000001,-2.1,-24.135)) ;
#120852=CARTESIAN_POINT('Origin',(0.500000000000001,-2.9,-21.585)) ;
#120853=CARTESIAN_POINT('Origin',(0.700000000000002,-2.9,-21.585)) ;
#120854=CARTESIAN_POINT('Origin',(-1.1,1.35,-24.235)) ;
#120855=CARTESIAN_POINT('Origin',(-1.1,1.35,-24.135)) ;
#120856=CARTESIAN_POINT('Origin',(-1.1,1.15,-24.135)) ;
#120857=CARTESIAN_POINT('',(-1.1,1.15,-24.235)) ;
#120858=CARTESIAN_POINT('Origin',(-1.1,1.15,-24.135)) ;
#120859=CARTESIAN_POINT('Origin',(-1.1,1.15,-24.135)) ;
#120860=CARTESIAN_POINT('Origin',(-0.899999999999999,-1.9,-24.135)) ;
#120861=CARTESIAN_POINT('Origin',(-1.1,-1.9,-24.135)) ;
#120862=CARTESIAN_POINT('Origin',(0.500000000000001,-5.86744705109802E-17,
-24.135)) ;
#120863=CARTESIAN_POINT('Origin',(0.500000000000001,-2.9,-24.135)) ;
#120864=CARTESIAN_POINT('Origin',(0.700000000000002,-2.9,-22.86)) ;
#120865=CARTESIAN_POINT('Origin',(0.700000000000002,-2.9,-24.135)) ;
#120866=CARTESIAN_POINT('Origin',(-1.1,1.15,-24.135)) ;
#120867=CARTESIAN_POINT('Origin',(-1.1,1.15,-24.335)) ;
#120868=CARTESIAN_POINT('Origin',(-1.1,-2.39429110547967E-16,-24.135)) ;
#120869=CARTESIAN_POINT('',(-1.1,1.25,-24.235)) ;
#120870=CARTESIAN_POINT('Origin',(0.500000000000001,-2.9,-24.135)) ;
#120871=CARTESIAN_POINT('Origin',(0.500000000000001,-2.9,-24.335)) ;
#120872=CARTESIAN_POINT('Origin',(-1.1,1.25,-24.335)) ;
#120873=CARTESIAN_POINT('Origin',(-1.1,-2.9,-24.335)) ;
#120874=CARTESIAN_POINT('Origin',(-1.1,-2.9,-24.335)) ;
#120875=CARTESIAN_POINT('Origin',(-1.1,-2.9,-24.335)) ;
#120876=CARTESIAN_POINT('Origin',(-1.1,-2.9,-24.335)) ;
#120877=CARTESIAN_POINT('Origin',(1.5,1.9,-22.26)) ;
#120878=CARTESIAN_POINT('Origin',(1.5,1.9,-24.41)) ;
#120879=CARTESIAN_POINT('Origin',(1.5,1.9,-23.46)) ;
#120880=CARTESIAN_POINT('Origin',(1.5,2.1,-23.46)) ;
#120881=CARTESIAN_POINT('Origin',(1.5,2.1,-23.26)) ;
#120882=CARTESIAN_POINT('Origin',(1.5,1.9,-24.41)) ;
#120883=CARTESIAN_POINT('Origin',(1.5,1.9,-24.41)) ;
#120884=CARTESIAN_POINT('Origin',(1.5,2.1,-23.26)) ;
#120885=CARTESIAN_POINT('Origin',(1.5,2.4,-23.26)) ;
#120886=CARTESIAN_POINT('Origin',(1.5,2.1,-24.41)) ;
#120887=CARTESIAN_POINT('Origin',(1.5,-2.15,-24.41)) ;
#120888=CARTESIAN_POINT('Origin',(1.5,2.4,-23.46)) ;
#120889=CARTESIAN_POINT('Origin',(1.5,2.6,-23.46)) ;
#120890=CARTESIAN_POINT('Origin',(1.5,-2.15,-24.41)) ;
#120891=CARTESIAN_POINT('Origin',(1.5,-2.15,-24.41)) ;
#120892=CARTESIAN_POINT('Origin',(1.5,2.6,-22.26)) ;
#120893=CARTESIAN_POINT('Origin',(1.5,2.6,-23.5685786437627)) ;
#120894=CARTESIAN_POINT('Origin',(1.5,-2.15,-22.26)) ;
#120895=CARTESIAN_POINT('Origin',(1.5,-2.15,-23.7631195934094)) ;
#120896=CARTESIAN_POINT('Origin',(1.5,2.6,-23.5685786437627)) ;
#120897=CARTESIAN_POINT('Origin',(1.5,2.6,-23.5685786437627)) ;
#120898=CARTESIAN_POINT('Origin',(1.5,-2.15,-23.7631195934094)) ;
#120899=CARTESIAN_POINT('Origin',(1.5,-2.15,-23.7631195934094)) ;
#120900=CARTESIAN_POINT('Origin',(1.5,1.69571067811865,-22.6642893218813)) ;
#120901=CARTESIAN_POINT('Origin',(1.5,3.15,-24.1185786437627)) ;
#120902=CARTESIAN_POINT('Origin',(1.5,-3.65625,-22.86)) ;
#120903=CARTESIAN_POINT('Origin',(1.5,-2.15,-21.9568804065906)) ;
#120904=CARTESIAN_POINT('Origin',(1.5,3.15,-24.1185786437627)) ;
#120905=CARTESIAN_POINT('Origin',(1.5,3.15,-24.1185786437627)) ;
#120906=CARTESIAN_POINT('Origin',(1.5,-2.15,-21.9568804065906)) ;
#120907=CARTESIAN_POINT('Origin',(1.5,-2.15,-21.9568804065906)) ;
#120908=CARTESIAN_POINT('Origin',(1.5,3.15,-22.26)) ;
#120909=CARTESIAN_POINT('Origin',(1.5,-2.15,-22.26)) ;
#120910=CARTESIAN_POINT('Origin',(1.5,-2.15,-21.31)) ;
#120911=CARTESIAN_POINT('Origin',(1.5,-2.15,-21.31)) ;
#120912=CARTESIAN_POINT('Origin',(1.5,-2.15,-21.31)) ;
#120913=CARTESIAN_POINT('Origin',(1.5,2.29571067811866,-22.4557106781187)) ;
#120914=CARTESIAN_POINT('Origin',(1.5,2.6,-22.1514213562373)) ;
#120915=CARTESIAN_POINT('Origin',(1.5,2.1,-21.31)) ;
#120916=CARTESIAN_POINT('Origin',(1.5,1.9,-21.31)) ;
#120917=CARTESIAN_POINT('Origin',(1.5,2.6,-22.1514213562373)) ;
#120918=CARTESIAN_POINT('Origin',(1.5,2.6,-22.1514213562373)) ;
#120919=CARTESIAN_POINT('Origin',(1.5,1.9,-21.31)) ;
#120920=CARTESIAN_POINT('Origin',(1.5,1.9,-21.31)) ;
#120921=CARTESIAN_POINT('Origin',(1.5,2.6,-22.26)) ;
#120922=CARTESIAN_POINT('Origin',(1.5,2.6,-22.26)) ;
#120923=CARTESIAN_POINT('Origin',(1.5,1.9,-22.26)) ;
#120924=CARTESIAN_POINT('Origin',(1.5,1.9,-22.26)) ;
#120925=CARTESIAN_POINT('Origin',(1.5,2.4,-22.26)) ;
#120926=CARTESIAN_POINT('Origin',(1.5,2.4,-22.46)) ;
#120927=CARTESIAN_POINT('Origin',(1.5,2.1,-22.26)) ;
#120928=CARTESIAN_POINT('Origin',(1.5,2.1,-22.46)) ;
#120929=CARTESIAN_POINT('Origin',(1.5,2.1,-22.46)) ;
#120930=CARTESIAN_POINT('Origin',(-0.899999999999999,-2.,-26.07)) ;
#120931=CARTESIAN_POINT('Origin',(-0.899999999999999,0.4,-26.07)) ;
#120932=CARTESIAN_POINT('Origin',(-0.899999999999999,-1.9,-26.07)) ;
#120933=CARTESIAN_POINT('Origin',(0.600000000000001,0.4,-26.27)) ;
#120934=CARTESIAN_POINT('Origin',(0.500000000000001,0.4,-26.27)) ;
#120935=CARTESIAN_POINT('Origin',(-0.899999999999999,0.4,-26.27)) ;
#120936=CARTESIAN_POINT('Origin',(0.500000000000001,0.4,-26.27)) ;
#120937=CARTESIAN_POINT('',(0.600000000000001,0.4,-26.27)) ;
#120938=CARTESIAN_POINT('Origin',(0.500000000000001,0.4,-26.27)) ;
#120939=CARTESIAN_POINT('Origin',(0.500000000000001,0.4,-26.27)) ;
#120940=CARTESIAN_POINT('Origin',(-0.899999999999999,-1.9,-26.07)) ;
#120941=CARTESIAN_POINT('Origin',(-0.899999999999999,-1.9,-26.07)) ;
#120942=CARTESIAN_POINT('Origin',(-0.899999999999999,-1.9,-26.07)) ;
#120943=CARTESIAN_POINT('Origin',(-0.899999999999999,0.4,-26.27)) ;
#120944=CARTESIAN_POINT('Origin',(-0.899999999999999,0.6,-26.27)) ;
#120945=CARTESIAN_POINT('Origin',(0.500000000000001,0.4,-26.67)) ;
#120946=CARTESIAN_POINT('Origin',(0.500000000000001,0.4,-27.07)) ;
#120947=CARTESIAN_POINT('',(0.600000000000001,0.4,-26.97)) ;
#120948=CARTESIAN_POINT('Ctrl Pts',(0.595612997216081,0.370705721320404,
-27.0407057213204)) ;
#120949=CARTESIAN_POINT('Ctrl Pts',(0.596180587760891,0.372558268494353,
-27.0388554988322)) ;
#120950=CARTESIAN_POINT('Ctrl Pts',(0.596672461925684,0.374355839771976,
-27.0369141798663)) ;
#120951=CARTESIAN_POINT('Ctrl Pts',(0.599015141889213,0.383869350930061,
-27.0257649936563)) ;
#120952=CARTESIAN_POINT('Ctrl Pts',(0.599609996542524,0.390224332900445,
-27.0149726026541)) ;
#120953=CARTESIAN_POINT('Ctrl Pts',(0.600050586298725,0.398117439141558,
-26.9923310532047)) ;
#120954=CARTESIAN_POINT('Ctrl Pts',(0.600000000000001,0.4,-26.9812012506335)) ;
#120955=CARTESIAN_POINT('Ctrl Pts',(0.600000000000001,0.399999999999999,
-26.97)) ;
#120956=CARTESIAN_POINT('',(0.600000000000001,0.4,-26.67)) ;
#120957=CARTESIAN_POINT('Origin',(0.500000000000001,-4.56640444411542E-17,
-26.27)) ;
#120958=CARTESIAN_POINT('',(0.500000000000001,0.394987437106619,-26.37)) ;
#120959=CARTESIAN_POINT('Ctrl Pts',(0.500000000000001,0.394987437106619,
-26.37)) ;
#120960=CARTESIAN_POINT('Ctrl Pts',(0.505940567948943,0.395584486649899,
-26.37)) ;
#120961=CARTESIAN_POINT('Ctrl Pts',(0.511931971019117,0.396132036079017,
-26.369466300328)) ;
#120962=CARTESIAN_POINT('Ctrl Pts',(0.517829015308519,0.396618246075352,
-26.3683977957737)) ;
#120963=CARTESIAN_POINT('Ctrl Pts',(0.522982218721183,0.397043126556052,
-26.3674640701571)) ;
#120964=CARTESIAN_POINT('Ctrl Pts',(0.528062648970233,0.397421319341387,
-26.3661228267971)) ;
#120965=CARTESIAN_POINT('Ctrl Pts',(0.532978106724005,0.397751505046071,
-26.3644057438766)) ;
#120966=CARTESIAN_POINT('Ctrl Pts',(0.538583536338987,0.398128038183001,
-26.3624476378495)) ;
#120967=CARTESIAN_POINT('Ctrl Pts',(0.544059405914956,0.398447721828298,
-26.359970008311)) ;
#120968=CARTESIAN_POINT('Ctrl Pts',(0.549268572255855,0.398712331108987,
-26.3570207319429)) ;
#120969=CARTESIAN_POINT('Ctrl Pts',(0.553856850427182,0.398945401221758,
-26.3544229841468)) ;
#120970=CARTESIAN_POINT('Ctrl Pts',(0.558237825069334,0.399135987683844,
-26.35146038498)) ;
#120971=CARTESIAN_POINT('Ctrl Pts',(0.562333836086203,0.399290378266507,
-26.3481952228642)) ;
#120972=CARTESIAN_POINT('Ctrl Pts',(0.566990328957878,0.399465895042381,
-26.3444832689523)) ;
#120973=CARTESIAN_POINT('Ctrl Pts',(0.571349096493401,0.399597278936106,
-26.3403228064848)) ;
#120974=CARTESIAN_POINT('Ctrl Pts',(0.575296920056684,0.399694832180836,
-26.3358055759794)) ;
#120975=CARTESIAN_POINT('Ctrl Pts',(0.57874426366789,0.399780018245913,
-26.3318610112151)) ;
#120976=CARTESIAN_POINT('Ctrl Pts',(0.581878314560405,0.399839626289636,
-26.3276455218421)) ;
#120977=CARTESIAN_POINT('Ctrl Pts',(0.584648147334854,0.399882153365959,
-26.3232418177073)) ;
#120978=CARTESIAN_POINT('Ctrl Pts',(0.587839270208225,0.39993114878808,
-26.3181683125044)) ;
#120979=CARTESIAN_POINT('Ctrl Pts',(0.590595054415145,0.399958289583405,
-26.3127666362444)) ;
#120980=CARTESIAN_POINT('Ctrl Pts',(0.592838618943168,0.39997435700316,
-26.3071616850092)) ;
#120981=CARTESIAN_POINT('Ctrl Pts',(0.594777336851685,0.399988241245861,
-26.3023183122423)) ;
#120982=CARTESIAN_POINT('Ctrl Pts',(0.596334051506207,0.399993946552814,
-26.2973241662271)) ;
#120983=CARTESIAN_POINT('Ctrl Pts',(0.597488309822313,0.39999684570125,
-26.2922717185684)) ;
#120984=CARTESIAN_POINT('Ctrl Pts',(0.598804024094449,0.400000150378306,
-26.2865125419603)) ;
#120985=CARTESIAN_POINT('Ctrl Pts',(0.599612685195482,0.399999963509465,
-26.2806028438903)) ;
#120986=CARTESIAN_POINT('Ctrl Pts',(0.599890230999748,0.399999993975383,
-26.2746842022605)) ;
#120987=CARTESIAN_POINT('Ctrl Pts',(0.59996346454941,0.400000002014155,
-26.2731225027894)) ;
#120988=CARTESIAN_POINT('Ctrl Pts',(0.600000000000001,0.399999999999999,
-26.271560221509)) ;
#120989=CARTESIAN_POINT('Ctrl Pts',(0.600000000000001,0.399999999999999,
-26.27)) ;
#120990=CARTESIAN_POINT('',(0.600000000000001,0.299999999999999,-26.27)) ;
#120991=CARTESIAN_POINT('Ctrl Pts',(0.500000000000001,0.394987437106619,
-26.37)) ;
#120992=CARTESIAN_POINT('Ctrl Pts',(0.500454935590171,0.395033159853782,
-26.37)) ;
#120993=CARTESIAN_POINT('Ctrl Pts',(0.500909898680634,0.395078570329076,
-26.3699968954911)) ;
#120994=CARTESIAN_POINT('Ctrl Pts',(0.502892456244958,0.395275075889069,
-26.3699698339419)) ;
#120995=CARTESIAN_POINT('Ctrl Pts',(0.50441874748225,0.395422812032187,
-26.369913985421)) ;
#120996=CARTESIAN_POINT('Ctrl Pts',(0.508462199543321,0.395804395682031,
-26.3696732810567)) ;
#120997=CARTESIAN_POINT('Ctrl Pts',(0.510974953343264,0.396031485023314,
-26.3694279391451)) ;
#120998=CARTESIAN_POINT('Ctrl Pts',(0.521160739721166,0.396903453186226,
-26.3680427944916)) ;
#120999=CARTESIAN_POINT('Ctrl Pts',(0.528708678528252,0.397444933153152,
-26.3661042177047)) ;
#121000=CARTESIAN_POINT('Ctrl Pts',(0.545943206357825,0.398105551684101,
-26.3594646394513)) ;
#121001=CARTESIAN_POINT('Ctrl Pts',(0.555229535466584,0.397987646678453,
-26.3540353588361)) ;
#121002=CARTESIAN_POINT('Ctrl Pts',(0.571394604995541,0.395490482808082,
-26.3407755133641)) ;
#121003=CARTESIAN_POINT('Ctrl Pts',(0.578055313702682,0.393198948698442,
-26.333240745632)) ;
#121004=CARTESIAN_POINT('Ctrl Pts',(0.588559132202378,0.385442756729426,
-26.3173922339843)) ;
#121005=CARTESIAN_POINT('Ctrl Pts',(0.592167355639896,0.380240075127069,
-26.309548265607)) ;
#121006=CARTESIAN_POINT('Ctrl Pts',(0.597496615531045,0.365892753467188,
-26.2939255217955)) ;
#121007=CARTESIAN_POINT('Ctrl Pts',(0.598734255154177,0.356660564300953,
-26.2867727417271)) ;
#121008=CARTESIAN_POINT('Ctrl Pts',(0.60001275468168,0.335223914398804,
-26.2755823058657)) ;
#121009=CARTESIAN_POINT('Ctrl Pts',(0.599993900559809,0.322655037092181,
-26.2716615193656)) ;
#121010=CARTESIAN_POINT('Ctrl Pts',(0.600000296204999,0.30610691358248,
-26.2701396263471)) ;
#121011=CARTESIAN_POINT('Ctrl Pts',(0.600000000000001,0.303050992413506,
-26.27)) ;
#121012=CARTESIAN_POINT('Ctrl Pts',(0.600000000000001,0.299999999999999,
-26.27)) ;
#121013=CARTESIAN_POINT('',(0.600000000000001,-2.39800009914441E-17,-26.27)) ;
#121014=CARTESIAN_POINT('Origin',(0.500000000000001,-1.9,-26.27)) ;
#121015=CARTESIAN_POINT('Origin',(0.600000000000001,-1.9,-26.07)) ;
#121016=CARTESIAN_POINT('Origin',(0.500000000000001,-1.9,-26.07)) ;
#121017=CARTESIAN_POINT('Origin',(-0.899999999999999,-1.9,-25.295)) ;
#121018=CARTESIAN_POINT('Origin',(-0.899999999999999,-1.9,-25.395)) ;
#121019=CARTESIAN_POINT('Origin',(-0.899999999999999,0.6,-26.17)) ;
#121020=CARTESIAN_POINT('Origin',(-0.899999999999999,0.6,-27.07)) ;
#121021=CARTESIAN_POINT('Origin',(0.600000000000001,0.4,-27.07)) ;
#121022=CARTESIAN_POINT('Origin',(0.500000000000001,0.4,-27.07)) ;
#121023=CARTESIAN_POINT('Origin',(-0.899999999999999,0.4,-27.07)) ;
#121024=CARTESIAN_POINT('Origin',(0.500000000000001,0.4,-27.07)) ;
#121025=CARTESIAN_POINT('Origin',(0.500000000000001,-1.9,-26.07)) ;
#121026=CARTESIAN_POINT('Origin',(0.500000000000001,-2.1,-26.07)) ;
#121027=CARTESIAN_POINT('Origin',(-0.899999999999999,-1.9,-25.395)) ;
#121028=CARTESIAN_POINT('Origin',(-1.1,-1.9,-25.395)) ;
#121029=CARTESIAN_POINT('Origin',(-0.899999999999999,-2.1,-25.395)) ;
#121030=CARTESIAN_POINT('Origin',(-0.899999999999999,0.4,-27.07)) ;
#121031=CARTESIAN_POINT('Origin',(-0.899999999999999,0.4,-27.27)) ;
#121032=CARTESIAN_POINT('Origin',(0.500000000000001,-2.1,-26.67)) ;
#121033=CARTESIAN_POINT('Origin',(0.500000000000001,-2.1,-25.395)) ;
#121034=CARTESIAN_POINT('Origin',(0.600000000000001,-2.1,-25.395)) ;
#121035=CARTESIAN_POINT('Origin',(0.500000000000001,-2.1,-25.395)) ;
#121036=CARTESIAN_POINT('Origin',(-1.1,-4.42727195005762E-17,-25.395)) ;
#121037=CARTESIAN_POINT('',(-1.1,1.15,-25.295)) ;
#121038=CARTESIAN_POINT('',(-1.1,1.25,-25.295)) ;
#121039=CARTESIAN_POINT('Origin',(-1.1,1.15,-25.395)) ;
#121040=CARTESIAN_POINT('Origin',(-0.899999999999999,0.5,-27.27)) ;
#121041=CARTESIAN_POINT('Origin',(-0.899999999999999,-1.9,-27.27)) ;
#121042=CARTESIAN_POINT('Origin',(0.600000000000001,-1.9,-27.27)) ;
#121043=CARTESIAN_POINT('Origin',(0.500000000000001,-1.9,-27.27)) ;
#121044=CARTESIAN_POINT('Origin',(-0.899999999999999,-1.9,-27.27)) ;
#121045=CARTESIAN_POINT('Origin',(0.500000000000001,-1.9,-27.27)) ;
#121046=CARTESIAN_POINT('Origin',(0.500000000000001,-2.1,-27.27)) ;
#121047=CARTESIAN_POINT('Origin',(0.500000000000001,-2.1,-25.395)) ;
#121048=CARTESIAN_POINT('Origin',(0.500000000000001,-2.1,-25.395)) ;
#121049=CARTESIAN_POINT('Origin',(-1.1,-2.9,-25.195)) ;
#121050=CARTESIAN_POINT('Origin',(-1.1,-2.9,-25.195)) ;
#121051=CARTESIAN_POINT('Origin',(-1.1,-2.9,-25.195)) ;
#121052=CARTESIAN_POINT('Origin',(-1.1,1.25,-25.195)) ;
#121053=CARTESIAN_POINT('Origin',(-1.1,1.15,-25.195)) ;
#121054=CARTESIAN_POINT('Origin',(-1.1,1.15,-25.395)) ;
#121055=CARTESIAN_POINT('',(-1.1,1.25,-25.395)) ;
#121056=CARTESIAN_POINT('Origin',(-1.1,1.15,-25.395)) ;
#121057=CARTESIAN_POINT('Origin',(-1.1,1.15,-25.395)) ;
#121058=CARTESIAN_POINT('Origin',(-0.899999999999999,-1.9,-27.27)) ;
#121059=CARTESIAN_POINT('Origin',(-0.899999999999999,-1.9,-27.27)) ;
#121060=CARTESIAN_POINT('Origin',(0.500000000000001,-2.1,-26.67)) ;
#121061=CARTESIAN_POINT('Origin',(0.500000000000001,-2.1,-27.945)) ;
#121062=CARTESIAN_POINT('Origin',(0.500000000000001,1.36481920536411E-16,
-25.395)) ;
#121063=CARTESIAN_POINT('Origin',(0.500000000000001,-2.9,-25.395)) ;
#121064=CARTESIAN_POINT('Origin',(-0.999999999999999,-2.9,-25.195)) ;
#121065=CARTESIAN_POINT('Origin',(0.500000000000001,-2.9,-25.195)) ;
#121066=CARTESIAN_POINT('Origin',(-1.1,1.15,-25.395)) ;
#121067=CARTESIAN_POINT('Origin',(-1.1,1.35,-25.395)) ;
#121068=CARTESIAN_POINT('Origin',(-1.1,1.15,-26.67)) ;
#121069=CARTESIAN_POINT('',(-1.1,1.25,-27.945)) ;
#121070=CARTESIAN_POINT('',(-1.1,1.25,-28.045)) ;
#121071=CARTESIAN_POINT('Origin',(-1.1,1.15,-27.945)) ;
#121072=CARTESIAN_POINT('Origin',(-0.899999999999999,-1.9,-27.17)) ;
#121073=CARTESIAN_POINT('Origin',(-0.899999999999999,-1.9,-27.945)) ;
#121074=CARTESIAN_POINT('Origin',(-0.999999999999999,-2.1,-27.945)) ;
#121075=CARTESIAN_POINT('Origin',(0.500000000000001,-2.1,-27.945)) ;
#121076=CARTESIAN_POINT('Origin',(-0.899999999999999,-2.1,-27.945)) ;
#121077=CARTESIAN_POINT('Origin',(0.500000000000001,-2.1,-27.945)) ;
#121078=CARTESIAN_POINT('Origin',(0.500000000000001,-2.1,-27.945)) ;
#121079=CARTESIAN_POINT('Origin',(0.500000000000001,-2.9,-25.395)) ;
#121080=CARTESIAN_POINT('Origin',(0.700000000000002,-2.9,-25.395)) ;
#121081=CARTESIAN_POINT('Origin',(-1.1,1.35,-28.045)) ;
#121082=CARTESIAN_POINT('Origin',(-1.1,1.35,-27.945)) ;
#121083=CARTESIAN_POINT('Origin',(-1.1,1.15,-27.945)) ;
#121084=CARTESIAN_POINT('',(-1.1,1.15,-28.045)) ;
#121085=CARTESIAN_POINT('Origin',(-1.1,1.15,-27.945)) ;
#121086=CARTESIAN_POINT('Origin',(-1.1,1.15,-27.945)) ;
#121087=CARTESIAN_POINT('Origin',(-0.899999999999999,-1.9,-27.945)) ;
#121088=CARTESIAN_POINT('Origin',(-1.1,-1.9,-27.945)) ;
#121089=CARTESIAN_POINT('Origin',(0.500000000000001,-5.86744705109802E-17,
-27.945)) ;
#121090=CARTESIAN_POINT('Origin',(0.500000000000001,-2.9,-27.945)) ;
#121091=CARTESIAN_POINT('Origin',(0.700000000000002,-2.9,-26.67)) ;
#121092=CARTESIAN_POINT('Origin',(0.700000000000002,-2.9,-27.945)) ;
#121093=CARTESIAN_POINT('Origin',(-1.1,1.15,-27.945)) ;
#121094=CARTESIAN_POINT('Origin',(-1.1,1.15,-28.145)) ;
#121095=CARTESIAN_POINT('Origin',(-1.1,-2.39429110547967E-16,-27.945)) ;
#121096=CARTESIAN_POINT('',(-1.1,1.25,-28.045)) ;
#121097=CARTESIAN_POINT('Origin',(0.500000000000001,-2.9,-27.945)) ;
#121098=CARTESIAN_POINT('Origin',(0.500000000000001,-2.9,-28.145)) ;
#121099=CARTESIAN_POINT('Origin',(-1.1,1.25,-28.145)) ;
#121100=CARTESIAN_POINT('Origin',(-1.1,-2.9,-28.145)) ;
#121101=CARTESIAN_POINT('Origin',(-1.1,-2.9,-28.145)) ;
#121102=CARTESIAN_POINT('Origin',(-1.1,-2.9,-28.145)) ;
#121103=CARTESIAN_POINT('Origin',(-1.1,-2.9,-28.145)) ;
#121104=CARTESIAN_POINT('Origin',(1.5,1.9,-26.07)) ;
#121105=CARTESIAN_POINT('Origin',(1.5,1.9,-28.22)) ;
#121106=CARTESIAN_POINT('Origin',(1.5,1.9,-27.27)) ;
#121107=CARTESIAN_POINT('Origin',(1.5,2.1,-27.27)) ;
#121108=CARTESIAN_POINT('Origin',(1.5,2.1,-27.07)) ;
#121109=CARTESIAN_POINT('Origin',(1.5,1.9,-28.22)) ;
#121110=CARTESIAN_POINT('Origin',(1.5,1.9,-28.22)) ;
#121111=CARTESIAN_POINT('Origin',(1.5,2.1,-27.07)) ;
#121112=CARTESIAN_POINT('Origin',(1.5,2.4,-27.07)) ;
#121113=CARTESIAN_POINT('Origin',(1.5,2.1,-28.22)) ;
#121114=CARTESIAN_POINT('Origin',(1.5,-2.15,-28.22)) ;
#121115=CARTESIAN_POINT('Origin',(1.5,2.4,-27.27)) ;
#121116=CARTESIAN_POINT('Origin',(1.5,2.6,-27.27)) ;
#121117=CARTESIAN_POINT('Origin',(1.5,-2.15,-28.22)) ;
#121118=CARTESIAN_POINT('Origin',(1.5,-2.15,-28.22)) ;
#121119=CARTESIAN_POINT('Origin',(1.5,2.6,-26.07)) ;
#121120=CARTESIAN_POINT('Origin',(1.5,2.6,-27.3785786437627)) ;
#121121=CARTESIAN_POINT('Origin',(1.5,-2.15,-26.07)) ;
#121122=CARTESIAN_POINT('Origin',(1.5,-2.15,-27.5731195934094)) ;
#121123=CARTESIAN_POINT('Origin',(1.5,2.6,-27.3785786437627)) ;
#121124=CARTESIAN_POINT('Origin',(1.5,2.6,-27.3785786437627)) ;
#121125=CARTESIAN_POINT('Origin',(1.5,-2.15,-27.5731195934094)) ;
#121126=CARTESIAN_POINT('Origin',(1.5,-2.15,-27.5731195934094)) ;
#121127=CARTESIAN_POINT('Origin',(1.5,1.69571067811865,-26.4742893218813)) ;
#121128=CARTESIAN_POINT('Origin',(1.5,3.15,-27.9285786437627)) ;
#121129=CARTESIAN_POINT('Origin',(1.5,-3.65625,-26.67)) ;
#121130=CARTESIAN_POINT('Origin',(1.5,-2.15,-25.7668804065906)) ;
#121131=CARTESIAN_POINT('Origin',(1.5,3.15,-27.9285786437627)) ;
#121132=CARTESIAN_POINT('Origin',(1.5,3.15,-27.9285786437627)) ;
#121133=CARTESIAN_POINT('Origin',(1.5,-2.15,-25.7668804065906)) ;
#121134=CARTESIAN_POINT('Origin',(1.5,-2.15,-25.7668804065906)) ;
#121135=CARTESIAN_POINT('Origin',(1.5,3.15,-26.07)) ;
#121136=CARTESIAN_POINT('Origin',(1.5,-2.15,-26.07)) ;
#121137=CARTESIAN_POINT('Origin',(1.5,-2.15,-25.12)) ;
#121138=CARTESIAN_POINT('Origin',(1.5,-2.15,-25.12)) ;
#121139=CARTESIAN_POINT('Origin',(1.5,-2.15,-25.12)) ;
#121140=CARTESIAN_POINT('Origin',(1.5,2.29571067811866,-26.2657106781187)) ;
#121141=CARTESIAN_POINT('Origin',(1.5,2.6,-25.9614213562373)) ;
#121142=CARTESIAN_POINT('Origin',(1.5,2.1,-25.12)) ;
#121143=CARTESIAN_POINT('Origin',(1.5,1.9,-25.12)) ;
#121144=CARTESIAN_POINT('Origin',(1.5,2.6,-25.9614213562373)) ;
#121145=CARTESIAN_POINT('Origin',(1.5,2.6,-25.9614213562373)) ;
#121146=CARTESIAN_POINT('Origin',(1.5,1.9,-25.12)) ;
#121147=CARTESIAN_POINT('Origin',(1.5,1.9,-25.12)) ;
#121148=CARTESIAN_POINT('Origin',(1.5,2.6,-26.07)) ;
#121149=CARTESIAN_POINT('Origin',(1.5,2.6,-26.07)) ;
#121150=CARTESIAN_POINT('Origin',(1.5,1.9,-26.07)) ;
#121151=CARTESIAN_POINT('Origin',(1.5,1.9,-26.07)) ;
#121152=CARTESIAN_POINT('Origin',(1.5,2.4,-26.07)) ;
#121153=CARTESIAN_POINT('Origin',(1.5,2.4,-26.27)) ;
#121154=CARTESIAN_POINT('Origin',(1.5,2.1,-26.07)) ;
#121155=CARTESIAN_POINT('Origin',(1.5,2.1,-26.27)) ;
#121156=CARTESIAN_POINT('Origin',(1.5,2.1,-26.27)) ;
#121157=CARTESIAN_POINT('Origin',(-0.899999999999999,-2.,-29.88)) ;
#121158=CARTESIAN_POINT('Origin',(-0.899999999999999,0.4,-29.88)) ;
#121159=CARTESIAN_POINT('Origin',(-0.899999999999999,-1.9,-29.88)) ;
#121160=CARTESIAN_POINT('Origin',(0.600000000000001,0.4,-30.08)) ;
#121161=CARTESIAN_POINT('Origin',(0.500000000000001,0.4,-30.08)) ;
#121162=CARTESIAN_POINT('Origin',(-0.899999999999999,0.4,-30.08)) ;
#121163=CARTESIAN_POINT('Origin',(0.500000000000001,0.4,-30.08)) ;
#121164=CARTESIAN_POINT('',(0.600000000000001,0.4,-30.08)) ;
#121165=CARTESIAN_POINT('Origin',(0.500000000000001,0.4,-30.08)) ;
#121166=CARTESIAN_POINT('Origin',(0.500000000000001,0.4,-30.08)) ;
#121167=CARTESIAN_POINT('Origin',(-0.899999999999999,-1.9,-29.88)) ;
#121168=CARTESIAN_POINT('Origin',(-0.899999999999999,-1.9,-29.88)) ;
#121169=CARTESIAN_POINT('Origin',(-0.899999999999999,-1.9,-29.88)) ;
#121170=CARTESIAN_POINT('Origin',(-0.899999999999999,0.4,-30.08)) ;
#121171=CARTESIAN_POINT('Origin',(-0.899999999999999,0.6,-30.08)) ;
#121172=CARTESIAN_POINT('Origin',(0.500000000000001,0.4,-30.48)) ;
#121173=CARTESIAN_POINT('Origin',(0.500000000000001,0.4,-30.88)) ;
#121174=CARTESIAN_POINT('',(0.600000000000001,0.4,-30.78)) ;
#121175=CARTESIAN_POINT('Ctrl Pts',(0.595612997216081,0.370705721320405,
-30.8507057213204)) ;
#121176=CARTESIAN_POINT('Ctrl Pts',(0.596180587760891,0.372558268494354,
-30.8488554988322)) ;
#121177=CARTESIAN_POINT('Ctrl Pts',(0.596672461925684,0.374355839771976,
-30.8469141798663)) ;
#121178=CARTESIAN_POINT('Ctrl Pts',(0.599015141889203,0.383869350930023,
-30.8357649936563)) ;
#121179=CARTESIAN_POINT('Ctrl Pts',(0.599609996542522,0.390224332900425,
-30.8249726026542)) ;
#121180=CARTESIAN_POINT('Ctrl Pts',(0.600050586298725,0.398117439141557,
-30.8023310532047)) ;
#121181=CARTESIAN_POINT('Ctrl Pts',(0.600000000000001,0.399999999999999,
-30.7912012506335)) ;
#121182=CARTESIAN_POINT('Ctrl Pts',(0.600000000000001,0.399999999999999,
-30.78)) ;
#121183=CARTESIAN_POINT('',(0.600000000000001,0.4,-30.48)) ;
#121184=CARTESIAN_POINT('Origin',(0.500000000000001,-4.56640444411542E-17,
-30.08)) ;
#121185=CARTESIAN_POINT('',(0.500000000000001,0.394987437106619,-30.18)) ;
#121186=CARTESIAN_POINT('Ctrl Pts',(0.500000000000001,0.394987437106619,
-30.18)) ;
#121187=CARTESIAN_POINT('Ctrl Pts',(0.505940567948935,0.395584486649899,
-30.18)) ;
#121188=CARTESIAN_POINT('Ctrl Pts',(0.511931971019101,0.396132036079015,
-30.179466300328)) ;
#121189=CARTESIAN_POINT('Ctrl Pts',(0.517829015308496,0.39661824607535,
-30.1783977957737)) ;
#121190=CARTESIAN_POINT('Ctrl Pts',(0.522982218721168,0.397043126556051,
-30.1774640701571)) ;
#121191=CARTESIAN_POINT('Ctrl Pts',(0.528062648970226,0.397421319341387,
-30.1761228267971)) ;
#121192=CARTESIAN_POINT('Ctrl Pts',(0.532978106724004,0.397751505046071,
-30.1744057438766)) ;
#121193=CARTESIAN_POINT('Ctrl Pts',(0.538583536338982,0.398128038183001,
-30.1724476378495)) ;
#121194=CARTESIAN_POINT('Ctrl Pts',(0.544059405914951,0.398447721828298,
-30.169970008311)) ;
#121195=CARTESIAN_POINT('Ctrl Pts',(0.549268572255847,0.398712331108986,
-30.1670207319429)) ;
#121196=CARTESIAN_POINT('Ctrl Pts',(0.553856850427178,0.398945401221757,
-30.1644229841468)) ;
#121197=CARTESIAN_POINT('Ctrl Pts',(0.558237825069329,0.399135987683843,
-30.16146038498)) ;
#121198=CARTESIAN_POINT('Ctrl Pts',(0.562333836086197,0.399290378266506,
-30.1581952228642)) ;
#121199=CARTESIAN_POINT('Ctrl Pts',(0.566990328957886,0.399465895042381,
-30.1544832689523)) ;
#121200=CARTESIAN_POINT('Ctrl Pts',(0.57134909649342,0.399597278936108,
-30.1503228064848)) ;
#121201=CARTESIAN_POINT('Ctrl Pts',(0.575296920056715,0.399694832180838,
-30.1458055759793)) ;
#121202=CARTESIAN_POINT('Ctrl Pts',(0.5787442636679,0.399780018245914,-30.1418610112151)) ;
#121203=CARTESIAN_POINT('Ctrl Pts',(0.581878314560451,0.399839626289636,
-30.1376455218421)) ;
#121204=CARTESIAN_POINT('Ctrl Pts',(0.584648147334861,0.399882153365958,
-30.1332418177073)) ;
#121205=CARTESIAN_POINT('Ctrl Pts',(0.587839270208171,0.399931148788079,
-30.1281683125045)) ;
#121206=CARTESIAN_POINT('Ctrl Pts',(0.590595054415091,0.399958289583404,
-30.1227666362445)) ;
#121207=CARTESIAN_POINT('Ctrl Pts',(0.592838618943106,0.399974357003159,
-30.1171616850094)) ;
#121208=CARTESIAN_POINT('Ctrl Pts',(0.594777336851655,0.399988241245861,
-30.1123183122424)) ;
#121209=CARTESIAN_POINT('Ctrl Pts',(0.596334051506183,0.399993946552814,
-30.1073241662271)) ;
#121210=CARTESIAN_POINT('Ctrl Pts',(0.597488309822302,0.39999684570125,
-30.1022717185684)) ;
#121211=CARTESIAN_POINT('Ctrl Pts',(0.598804024094428,0.400000150378306,
-30.0965125419604)) ;
#121212=CARTESIAN_POINT('Ctrl Pts',(0.599612685195468,0.399999963509465,
-30.0906028438904)) ;
#121213=CARTESIAN_POINT('Ctrl Pts',(0.599890230999741,0.399999993975383,
-30.0846842022606)) ;
#121214=CARTESIAN_POINT('Ctrl Pts',(0.599963464549407,0.400000002014155,
-30.0831225027895)) ;
#121215=CARTESIAN_POINT('Ctrl Pts',(0.600000000000001,0.399999999999999,
-30.081560221509)) ;
#121216=CARTESIAN_POINT('Ctrl Pts',(0.600000000000001,0.399999999999999,
-30.08)) ;
#121217=CARTESIAN_POINT('',(0.600000000000001,0.299999999999999,-30.08)) ;
#121218=CARTESIAN_POINT('Ctrl Pts',(0.500000000000001,0.394987437106619,
-30.18)) ;
#121219=CARTESIAN_POINT('Ctrl Pts',(0.500454935590171,0.395033159853782,
-30.18)) ;
#121220=CARTESIAN_POINT('Ctrl Pts',(0.500909898680634,0.395078570329076,
-30.1799968954911)) ;
#121221=CARTESIAN_POINT('Ctrl Pts',(0.502892456244958,0.395275075889069,
-30.1799698339419)) ;
#121222=CARTESIAN_POINT('Ctrl Pts',(0.50441874748225,0.395422812032187,
-30.179913985421)) ;
#121223=CARTESIAN_POINT('Ctrl Pts',(0.508462199543321,0.395804395682031,
-30.1796732810567)) ;
#121224=CARTESIAN_POINT('Ctrl Pts',(0.510974953343264,0.396031485023314,
-30.1794279391451)) ;
#121225=CARTESIAN_POINT('Ctrl Pts',(0.521160739721166,0.396903453186226,
-30.1780427944916)) ;
#121226=CARTESIAN_POINT('Ctrl Pts',(0.528708678528252,0.397444933153152,
-30.1761042177047)) ;
#121227=CARTESIAN_POINT('Ctrl Pts',(0.545943206357825,0.398105551684101,
-30.1694646394513)) ;
#121228=CARTESIAN_POINT('Ctrl Pts',(0.555229535466584,0.397987646678453,
-30.1640353588361)) ;
#121229=CARTESIAN_POINT('Ctrl Pts',(0.571394604995541,0.395490482808082,
-30.150775513364)) ;
#121230=CARTESIAN_POINT('Ctrl Pts',(0.578055313702682,0.393198948698442,
-30.143240745632)) ;
#121231=CARTESIAN_POINT('Ctrl Pts',(0.588559132202378,0.385442756729426,
-30.1273922339842)) ;
#121232=CARTESIAN_POINT('Ctrl Pts',(0.592167355639896,0.380240075127069,
-30.119548265607)) ;
#121233=CARTESIAN_POINT('Ctrl Pts',(0.597496615531045,0.365892753467188,
-30.1039255217955)) ;
#121234=CARTESIAN_POINT('Ctrl Pts',(0.598734255154177,0.356660564300953,
-30.0967727417271)) ;
#121235=CARTESIAN_POINT('Ctrl Pts',(0.60001275468168,0.335223914398804,
-30.0855823058657)) ;
#121236=CARTESIAN_POINT('Ctrl Pts',(0.599993900559809,0.322655037092181,
-30.0816615193656)) ;
#121237=CARTESIAN_POINT('Ctrl Pts',(0.600000296204999,0.30610691358248,
-30.0801396263471)) ;
#121238=CARTESIAN_POINT('Ctrl Pts',(0.600000000000001,0.303050992413506,
-30.08)) ;
#121239=CARTESIAN_POINT('Ctrl Pts',(0.600000000000001,0.299999999999999,
-30.08)) ;
#121240=CARTESIAN_POINT('',(0.600000000000001,-2.39800009914441E-17,-30.08)) ;
#121241=CARTESIAN_POINT('Origin',(0.500000000000001,-1.9,-30.08)) ;
#121242=CARTESIAN_POINT('Origin',(0.600000000000001,-1.9,-29.88)) ;
#121243=CARTESIAN_POINT('Origin',(0.500000000000001,-1.9,-29.88)) ;
#121244=CARTESIAN_POINT('Origin',(-0.899999999999999,-1.9,-29.105)) ;
#121245=CARTESIAN_POINT('Origin',(-0.899999999999999,-1.9,-29.205)) ;
#121246=CARTESIAN_POINT('Origin',(-0.899999999999999,0.6,-29.98)) ;
#121247=CARTESIAN_POINT('Origin',(-0.899999999999999,0.6,-30.88)) ;
#121248=CARTESIAN_POINT('Origin',(0.600000000000001,0.4,-30.88)) ;
#121249=CARTESIAN_POINT('Origin',(0.500000000000001,0.4,-30.88)) ;
#121250=CARTESIAN_POINT('Origin',(-0.899999999999999,0.4,-30.88)) ;
#121251=CARTESIAN_POINT('Origin',(0.500000000000001,0.4,-30.88)) ;
#121252=CARTESIAN_POINT('Origin',(0.500000000000001,-1.9,-29.88)) ;
#121253=CARTESIAN_POINT('Origin',(0.500000000000001,-2.1,-29.88)) ;
#121254=CARTESIAN_POINT('Origin',(-0.899999999999999,-1.9,-29.205)) ;
#121255=CARTESIAN_POINT('Origin',(-1.1,-1.9,-29.205)) ;
#121256=CARTESIAN_POINT('Origin',(-0.899999999999999,-2.1,-29.205)) ;
#121257=CARTESIAN_POINT('Origin',(-0.899999999999999,0.4,-30.88)) ;
#121258=CARTESIAN_POINT('Origin',(-0.899999999999999,0.4,-31.08)) ;
#121259=CARTESIAN_POINT('Origin',(0.500000000000001,-2.1,-30.48)) ;
#121260=CARTESIAN_POINT('Origin',(0.500000000000001,-2.1,-29.205)) ;
#121261=CARTESIAN_POINT('Origin',(0.600000000000001,-2.1,-29.205)) ;
#121262=CARTESIAN_POINT('Origin',(0.500000000000001,-2.1,-29.205)) ;
#121263=CARTESIAN_POINT('Origin',(-1.1,-4.42727195005762E-17,-29.205)) ;
#121264=CARTESIAN_POINT('',(-1.1,1.15,-29.105)) ;
#121265=CARTESIAN_POINT('',(-1.1,1.25,-29.105)) ;
#121266=CARTESIAN_POINT('Origin',(-1.1,1.15,-29.205)) ;
#121267=CARTESIAN_POINT('Origin',(-0.899999999999999,0.5,-31.08)) ;
#121268=CARTESIAN_POINT('Origin',(-0.899999999999999,-1.9,-31.08)) ;
#121269=CARTESIAN_POINT('Origin',(0.600000000000001,-1.9,-31.08)) ;
#121270=CARTESIAN_POINT('Origin',(0.500000000000001,-1.9,-31.08)) ;
#121271=CARTESIAN_POINT('Origin',(-0.899999999999999,-1.9,-31.08)) ;
#121272=CARTESIAN_POINT('Origin',(0.500000000000001,-1.9,-31.08)) ;
#121273=CARTESIAN_POINT('Origin',(0.500000000000001,-2.1,-31.08)) ;
#121274=CARTESIAN_POINT('Origin',(0.500000000000001,-2.1,-29.205)) ;
#121275=CARTESIAN_POINT('Origin',(0.500000000000001,-2.1,-29.205)) ;
#121276=CARTESIAN_POINT('Origin',(-1.1,-2.9,-29.005)) ;
#121277=CARTESIAN_POINT('Origin',(-1.1,-2.9,-29.005)) ;
#121278=CARTESIAN_POINT('Origin',(-1.1,-2.9,-29.005)) ;
#121279=CARTESIAN_POINT('Origin',(-1.1,1.25,-29.005)) ;
#121280=CARTESIAN_POINT('Origin',(-1.1,1.15,-29.005)) ;
#121281=CARTESIAN_POINT('Origin',(-1.1,1.15,-29.205)) ;
#121282=CARTESIAN_POINT('',(-1.1,1.25,-29.205)) ;
#121283=CARTESIAN_POINT('Origin',(-1.1,1.15,-29.205)) ;
#121284=CARTESIAN_POINT('Origin',(-1.1,1.15,-29.205)) ;
#121285=CARTESIAN_POINT('Origin',(-0.899999999999999,-1.9,-31.08)) ;
#121286=CARTESIAN_POINT('Origin',(-0.899999999999999,-1.9,-31.08)) ;
#121287=CARTESIAN_POINT('Origin',(0.500000000000001,-2.1,-30.48)) ;
#121288=CARTESIAN_POINT('Origin',(0.500000000000001,-2.1,-31.755)) ;
#121289=CARTESIAN_POINT('Origin',(0.500000000000001,1.36481920536411E-16,
-29.205)) ;
#121290=CARTESIAN_POINT('Origin',(0.500000000000001,-2.9,-29.205)) ;
#121291=CARTESIAN_POINT('Origin',(-0.999999999999999,-2.9,-29.005)) ;
#121292=CARTESIAN_POINT('Origin',(0.500000000000001,-2.9,-29.005)) ;
#121293=CARTESIAN_POINT('Origin',(-1.1,1.15,-29.205)) ;
#121294=CARTESIAN_POINT('Origin',(-1.1,1.35,-29.205)) ;
#121295=CARTESIAN_POINT('Origin',(-1.1,1.15,-30.48)) ;
#121296=CARTESIAN_POINT('',(-1.1,1.25,-31.755)) ;
#121297=CARTESIAN_POINT('',(-1.1,1.25,-31.855)) ;
#121298=CARTESIAN_POINT('Origin',(-1.1,1.15,-31.755)) ;
#121299=CARTESIAN_POINT('Origin',(-0.899999999999999,-1.9,-30.98)) ;
#121300=CARTESIAN_POINT('Origin',(-0.899999999999999,-1.9,-31.755)) ;
#121301=CARTESIAN_POINT('Origin',(-0.999999999999999,-2.1,-31.755)) ;
#121302=CARTESIAN_POINT('Origin',(0.500000000000001,-2.1,-31.755)) ;
#121303=CARTESIAN_POINT('Origin',(-0.899999999999999,-2.1,-31.755)) ;
#121304=CARTESIAN_POINT('Origin',(0.500000000000001,-2.1,-31.755)) ;
#121305=CARTESIAN_POINT('Origin',(0.500000000000001,-2.1,-31.755)) ;
#121306=CARTESIAN_POINT('Origin',(0.500000000000001,-2.9,-29.205)) ;
#121307=CARTESIAN_POINT('Origin',(0.700000000000002,-2.9,-29.205)) ;
#121308=CARTESIAN_POINT('Origin',(-1.1,1.35,-31.855)) ;
#121309=CARTESIAN_POINT('Origin',(-1.1,1.35,-31.755)) ;
#121310=CARTESIAN_POINT('Origin',(-1.1,1.15,-31.755)) ;
#121311=CARTESIAN_POINT('',(-1.1,1.15,-31.855)) ;
#121312=CARTESIAN_POINT('Origin',(-1.1,1.15,-31.755)) ;
#121313=CARTESIAN_POINT('Origin',(-1.1,1.15,-31.755)) ;
#121314=CARTESIAN_POINT('Origin',(-0.899999999999999,-1.9,-31.755)) ;
#121315=CARTESIAN_POINT('Origin',(-1.1,-1.9,-31.755)) ;
#121316=CARTESIAN_POINT('Origin',(0.500000000000001,-5.867447051098E-17,
-31.755)) ;
#121317=CARTESIAN_POINT('Origin',(0.500000000000001,-2.9,-31.755)) ;
#121318=CARTESIAN_POINT('Origin',(0.700000000000002,-2.9,-30.48)) ;
#121319=CARTESIAN_POINT('Origin',(0.700000000000002,-2.9,-31.755)) ;
#121320=CARTESIAN_POINT('Origin',(-1.1,1.15,-31.755)) ;
#121321=CARTESIAN_POINT('Origin',(-1.1,1.15,-31.955)) ;
#121322=CARTESIAN_POINT('Origin',(-1.1,-2.39429110547967E-16,-31.755)) ;
#121323=CARTESIAN_POINT('',(-1.1,1.25,-31.855)) ;
#121324=CARTESIAN_POINT('Origin',(0.500000000000001,-2.9,-31.755)) ;
#121325=CARTESIAN_POINT('Origin',(0.500000000000001,-2.9,-31.955)) ;
#121326=CARTESIAN_POINT('Origin',(-1.1,1.25,-31.955)) ;
#121327=CARTESIAN_POINT('Origin',(-1.1,-2.9,-31.955)) ;
#121328=CARTESIAN_POINT('Origin',(-1.1,-2.9,-31.955)) ;
#121329=CARTESIAN_POINT('Origin',(-1.1,-2.9,-31.955)) ;
#121330=CARTESIAN_POINT('Origin',(-1.1,-2.9,-31.955)) ;
#121331=CARTESIAN_POINT('Origin',(1.5,1.9,-29.88)) ;
#121332=CARTESIAN_POINT('Origin',(1.5,1.9,-32.03)) ;
#121333=CARTESIAN_POINT('Origin',(1.5,1.9,-31.08)) ;
#121334=CARTESIAN_POINT('Origin',(1.5,2.1,-31.08)) ;
#121335=CARTESIAN_POINT('Origin',(1.5,2.1,-30.88)) ;
#121336=CARTESIAN_POINT('Origin',(1.5,1.9,-32.03)) ;
#121337=CARTESIAN_POINT('Origin',(1.5,1.9,-32.03)) ;
#121338=CARTESIAN_POINT('Origin',(1.5,2.1,-30.88)) ;
#121339=CARTESIAN_POINT('Origin',(1.5,2.4,-30.88)) ;
#121340=CARTESIAN_POINT('Origin',(1.5,2.1,-32.03)) ;
#121341=CARTESIAN_POINT('Origin',(1.5,-2.15,-32.03)) ;
#121342=CARTESIAN_POINT('Origin',(1.5,2.4,-31.08)) ;
#121343=CARTESIAN_POINT('Origin',(1.5,2.6,-31.08)) ;
#121344=CARTESIAN_POINT('Origin',(1.5,-2.15,-32.03)) ;
#121345=CARTESIAN_POINT('Origin',(1.5,-2.15,-32.03)) ;
#121346=CARTESIAN_POINT('Origin',(1.5,2.6,-29.88)) ;
#121347=CARTESIAN_POINT('Origin',(1.5,2.6,-31.1885786437627)) ;
#121348=CARTESIAN_POINT('Origin',(1.5,-2.15,-29.88)) ;
#121349=CARTESIAN_POINT('Origin',(1.5,-2.15,-31.3831195934094)) ;
#121350=CARTESIAN_POINT('Origin',(1.5,2.6,-31.1885786437627)) ;
#121351=CARTESIAN_POINT('Origin',(1.5,2.6,-31.1885786437627)) ;
#121352=CARTESIAN_POINT('Origin',(1.5,-2.15,-31.3831195934094)) ;
#121353=CARTESIAN_POINT('Origin',(1.5,-2.15,-31.3831195934094)) ;
#121354=CARTESIAN_POINT('Origin',(1.5,1.69571067811865,-30.2842893218813)) ;
#121355=CARTESIAN_POINT('Origin',(1.5,3.15,-31.7385786437627)) ;
#121356=CARTESIAN_POINT('Origin',(1.5,-3.65625,-30.48)) ;
#121357=CARTESIAN_POINT('Origin',(1.5,-2.15,-29.5768804065906)) ;
#121358=CARTESIAN_POINT('Origin',(1.5,3.15,-31.7385786437627)) ;
#121359=CARTESIAN_POINT('Origin',(1.5,3.15,-31.7385786437627)) ;
#121360=CARTESIAN_POINT('Origin',(1.5,-2.15,-29.5768804065906)) ;
#121361=CARTESIAN_POINT('Origin',(1.5,-2.15,-29.5768804065906)) ;
#121362=CARTESIAN_POINT('Origin',(1.5,3.15,-29.88)) ;
#121363=CARTESIAN_POINT('Origin',(1.5,-2.15,-29.88)) ;
#121364=CARTESIAN_POINT('Origin',(1.5,-2.15,-28.93)) ;
#121365=CARTESIAN_POINT('Origin',(1.5,-2.15,-28.93)) ;
#121366=CARTESIAN_POINT('Origin',(1.5,-2.15,-28.93)) ;
#121367=CARTESIAN_POINT('Origin',(1.5,2.29571067811866,-30.0757106781187)) ;
#121368=CARTESIAN_POINT('Origin',(1.5,2.6,-29.7714213562373)) ;
#121369=CARTESIAN_POINT('Origin',(1.5,2.1,-28.93)) ;
#121370=CARTESIAN_POINT('Origin',(1.5,1.9,-28.93)) ;
#121371=CARTESIAN_POINT('Origin',(1.5,2.6,-29.7714213562373)) ;
#121372=CARTESIAN_POINT('Origin',(1.5,2.6,-29.7714213562373)) ;
#121373=CARTESIAN_POINT('Origin',(1.5,1.9,-28.93)) ;
#121374=CARTESIAN_POINT('Origin',(1.5,1.9,-28.93)) ;
#121375=CARTESIAN_POINT('Origin',(1.5,2.6,-29.88)) ;
#121376=CARTESIAN_POINT('Origin',(1.5,2.6,-29.88)) ;
#121377=CARTESIAN_POINT('Origin',(1.5,1.9,-29.88)) ;
#121378=CARTESIAN_POINT('Origin',(1.5,1.9,-29.88)) ;
#121379=CARTESIAN_POINT('Origin',(1.5,2.4,-29.88)) ;
#121380=CARTESIAN_POINT('Origin',(1.5,2.4,-30.08)) ;
#121381=CARTESIAN_POINT('Origin',(1.5,2.1,-29.88)) ;
#121382=CARTESIAN_POINT('Origin',(1.5,2.1,-30.08)) ;
#121383=CARTESIAN_POINT('Origin',(1.5,2.1,-30.08)) ;
#121384=CARTESIAN_POINT('Origin',(-0.899999999999999,-2.,-33.69)) ;
#121385=CARTESIAN_POINT('Origin',(-0.899999999999999,0.4,-33.69)) ;
#121386=CARTESIAN_POINT('Origin',(-0.899999999999999,-1.9,-33.69)) ;
#121387=CARTESIAN_POINT('Origin',(0.600000000000001,0.4,-33.89)) ;
#121388=CARTESIAN_POINT('Origin',(0.500000000000001,0.4,-33.89)) ;
#121389=CARTESIAN_POINT('Origin',(-0.899999999999999,0.4,-33.89)) ;
#121390=CARTESIAN_POINT('Origin',(0.500000000000001,0.4,-33.89)) ;
#121391=CARTESIAN_POINT('',(0.600000000000001,0.4,-33.89)) ;
#121392=CARTESIAN_POINT('Origin',(0.500000000000001,0.4,-33.89)) ;
#121393=CARTESIAN_POINT('Origin',(0.500000000000001,0.4,-33.89)) ;
#121394=CARTESIAN_POINT('Origin',(-0.899999999999999,-1.9,-33.69)) ;
#121395=CARTESIAN_POINT('Origin',(-0.899999999999999,-1.9,-33.69)) ;
#121396=CARTESIAN_POINT('Origin',(-0.899999999999999,-1.9,-33.69)) ;
#121397=CARTESIAN_POINT('Origin',(-0.899999999999999,0.4,-33.89)) ;
#121398=CARTESIAN_POINT('Origin',(-0.899999999999999,0.6,-33.89)) ;
#121399=CARTESIAN_POINT('Origin',(0.500000000000001,0.4,-34.29)) ;
#121400=CARTESIAN_POINT('Origin',(0.500000000000001,0.4,-34.69)) ;
#121401=CARTESIAN_POINT('',(0.600000000000001,0.4,-34.59)) ;
#121402=CARTESIAN_POINT('Ctrl Pts',(0.595612997216083,0.370705721320409,
-34.6607057213204)) ;
#121403=CARTESIAN_POINT('Ctrl Pts',(0.596180587760894,0.372558268494363,
-34.6588554988322)) ;
#121404=CARTESIAN_POINT('Ctrl Pts',(0.596672461925687,0.374355839771987,
-34.6569141798663)) ;
#121405=CARTESIAN_POINT('Ctrl Pts',(0.599015141889206,0.383869350930039,
-34.6457649936563)) ;
#121406=CARTESIAN_POINT('Ctrl Pts',(0.599609996542524,0.390224332900438,
-34.6349726026542)) ;
#121407=CARTESIAN_POINT('Ctrl Pts',(0.600050586298726,0.39811743914156,
-34.6123310532047)) ;
#121408=CARTESIAN_POINT('Ctrl Pts',(0.600000000000001,0.4,-34.6012012506335)) ;
#121409=CARTESIAN_POINT('Ctrl Pts',(0.600000000000001,0.399999999999999,
-34.59)) ;
#121410=CARTESIAN_POINT('',(0.600000000000001,0.4,-34.29)) ;
#121411=CARTESIAN_POINT('Origin',(0.500000000000001,-4.56640444411538E-17,
-33.89)) ;
#121412=CARTESIAN_POINT('',(0.500000000000001,0.394987437106619,-33.99)) ;
#121413=CARTESIAN_POINT('Ctrl Pts',(0.500000000000001,0.394987437106619,
-33.99)) ;
#121414=CARTESIAN_POINT('Ctrl Pts',(0.505940567948938,0.395584486649899,
-33.99)) ;
#121415=CARTESIAN_POINT('Ctrl Pts',(0.511931971019108,0.396132036079016,
-33.989466300328)) ;
#121416=CARTESIAN_POINT('Ctrl Pts',(0.517829015308506,0.396618246075351,
-33.9883977957737)) ;
#121417=CARTESIAN_POINT('Ctrl Pts',(0.522982218721175,0.397043126556051,
-33.9874640701571)) ;
#121418=CARTESIAN_POINT('Ctrl Pts',(0.52806264897023,0.397421319341387,
-33.9861228267971)) ;
#121419=CARTESIAN_POINT('Ctrl Pts',(0.532978106724009,0.397751505046071,
-33.9844057438766)) ;
#121420=CARTESIAN_POINT('Ctrl Pts',(0.538583536338943,0.398128038182998,
-33.9824476378496)) ;
#121421=CARTESIAN_POINT('Ctrl Pts',(0.544059405914837,0.398447721828293,
-33.9799700083111)) ;
#121422=CARTESIAN_POINT('Ctrl Pts',(0.549268572255721,0.39871233110898,
-33.9770207319429)) ;
#121423=CARTESIAN_POINT('Ctrl Pts',(0.553856850427124,0.398945401221754,
-33.9744229841469)) ;
#121424=CARTESIAN_POINT('Ctrl Pts',(0.55823782506931,0.399135987683842,
-33.97146038498)) ;
#121425=CARTESIAN_POINT('Ctrl Pts',(0.56233383608621,0.399290378266507,
-33.9681952228642)) ;
#121426=CARTESIAN_POINT('Ctrl Pts',(0.566990328957886,0.399465895042381,
-33.9644832689523)) ;
#121427=CARTESIAN_POINT('Ctrl Pts',(0.571349096493416,0.399597278936107,
-33.9603228064848)) ;
#121428=CARTESIAN_POINT('Ctrl Pts',(0.575296920056707,0.399694832180838,
-33.9558055759793)) ;
#121429=CARTESIAN_POINT('Ctrl Pts',(0.578744263667898,0.399780018245914,
-33.9518610112151)) ;
#121430=CARTESIAN_POINT('Ctrl Pts',(0.581878314560451,0.399839626289636,
-33.9476455218421)) ;
#121431=CARTESIAN_POINT('Ctrl Pts',(0.584648147334857,0.399882153365958,
-33.9432418177073)) ;
#121432=CARTESIAN_POINT('Ctrl Pts',(0.587839270208177,0.399931148788079,
-33.9381683125045)) ;
#121433=CARTESIAN_POINT('Ctrl Pts',(0.590595054415139,0.399958289583405,
-33.9327666362444)) ;
#121434=CARTESIAN_POINT('Ctrl Pts',(0.592838618943155,0.39997435700316,
-33.9271616850093)) ;
#121435=CARTESIAN_POINT('Ctrl Pts',(0.594777336851684,0.399988241245861,
-33.9223183122423)) ;
#121436=CARTESIAN_POINT('Ctrl Pts',(0.596334051506209,0.399993946552814,
-33.917324166227)) ;
#121437=CARTESIAN_POINT('Ctrl Pts',(0.597488309822315,0.39999684570125,
-33.9122717185684)) ;
#121438=CARTESIAN_POINT('Ctrl Pts',(0.598804024094335,0.400000150378306,
-33.9065125419608)) ;
#121439=CARTESIAN_POINT('Ctrl Pts',(0.599612685195353,0.399999963509465,
-33.9006028438911)) ;
#121440=CARTESIAN_POINT('Ctrl Pts',(0.599890230999679,0.399999993975383,
-33.894684202262)) ;
#121441=CARTESIAN_POINT('Ctrl Pts',(0.599963464549386,0.400000002014155,
-33.8931225027904)) ;
#121442=CARTESIAN_POINT('Ctrl Pts',(0.600000000000001,0.399999999999999,
-33.8915602215095)) ;
#121443=CARTESIAN_POINT('Ctrl Pts',(0.600000000000001,0.399999999999999,
-33.89)) ;
#121444=CARTESIAN_POINT('',(0.600000000000001,0.299999999999999,-33.89)) ;
#121445=CARTESIAN_POINT('Ctrl Pts',(0.500000000000001,0.394987437106619,
-33.99)) ;
#121446=CARTESIAN_POINT('Ctrl Pts',(0.500454935590171,0.395033159853782,
-33.99)) ;
#121447=CARTESIAN_POINT('Ctrl Pts',(0.500909898680634,0.395078570329076,
-33.9899968954911)) ;
#121448=CARTESIAN_POINT('Ctrl Pts',(0.502892456244958,0.395275075889069,
-33.9899698339419)) ;
#121449=CARTESIAN_POINT('Ctrl Pts',(0.50441874748225,0.395422812032187,
-33.989913985421)) ;
#121450=CARTESIAN_POINT('Ctrl Pts',(0.508462199543321,0.395804395682031,
-33.9896732810567)) ;
#121451=CARTESIAN_POINT('Ctrl Pts',(0.510974953343264,0.396031485023314,
-33.9894279391451)) ;
#121452=CARTESIAN_POINT('Ctrl Pts',(0.521160739721166,0.396903453186226,
-33.9880427944916)) ;
#121453=CARTESIAN_POINT('Ctrl Pts',(0.528708678528252,0.397444933153152,
-33.9861042177047)) ;
#121454=CARTESIAN_POINT('Ctrl Pts',(0.545943206357825,0.398105551684101,
-33.9794646394513)) ;
#121455=CARTESIAN_POINT('Ctrl Pts',(0.555229535466584,0.397987646678453,
-33.9740353588361)) ;
#121456=CARTESIAN_POINT('Ctrl Pts',(0.571394604995541,0.395490482808082,
-33.960775513364)) ;
#121457=CARTESIAN_POINT('Ctrl Pts',(0.578055313702682,0.393198948698442,
-33.953240745632)) ;
#121458=CARTESIAN_POINT('Ctrl Pts',(0.588559132202378,0.385442756729426,
-33.9373922339843)) ;
#121459=CARTESIAN_POINT('Ctrl Pts',(0.592167355639896,0.380240075127069,
-33.929548265607)) ;
#121460=CARTESIAN_POINT('Ctrl Pts',(0.597496615531045,0.365892753467188,
-33.9139255217955)) ;
#121461=CARTESIAN_POINT('Ctrl Pts',(0.598734255154177,0.356660564300953,
-33.9067727417271)) ;
#121462=CARTESIAN_POINT('Ctrl Pts',(0.60001275468168,0.335223914398804,
-33.8955823058657)) ;
#121463=CARTESIAN_POINT('Ctrl Pts',(0.599993900559809,0.322655037092181,
-33.8916615193656)) ;
#121464=CARTESIAN_POINT('Ctrl Pts',(0.600000296204999,0.30610691358248,
-33.8901396263471)) ;
#121465=CARTESIAN_POINT('Ctrl Pts',(0.600000000000001,0.303050992413506,
-33.89)) ;
#121466=CARTESIAN_POINT('Ctrl Pts',(0.600000000000001,0.299999999999999,
-33.89)) ;
#121467=CARTESIAN_POINT('',(0.600000000000001,-2.39800009914436E-17,-33.89)) ;
#121468=CARTESIAN_POINT('Origin',(0.500000000000001,-1.9,-33.89)) ;
#121469=CARTESIAN_POINT('Origin',(0.600000000000001,-1.9,-33.69)) ;
#121470=CARTESIAN_POINT('Origin',(0.500000000000001,-1.9,-33.69)) ;
#121471=CARTESIAN_POINT('Origin',(-0.899999999999999,-1.9,-32.915)) ;
#121472=CARTESIAN_POINT('Origin',(-0.899999999999999,-1.9,-33.015)) ;
#121473=CARTESIAN_POINT('Origin',(-0.899999999999999,0.6,-33.79)) ;
#121474=CARTESIAN_POINT('Origin',(-0.899999999999999,0.6,-34.69)) ;
#121475=CARTESIAN_POINT('Origin',(0.600000000000001,0.4,-34.69)) ;
#121476=CARTESIAN_POINT('Origin',(0.500000000000001,0.4,-34.69)) ;
#121477=CARTESIAN_POINT('Origin',(-0.899999999999999,0.4,-34.69)) ;
#121478=CARTESIAN_POINT('Origin',(0.500000000000001,0.4,-34.69)) ;
#121479=CARTESIAN_POINT('Origin',(0.500000000000001,-1.9,-33.69)) ;
#121480=CARTESIAN_POINT('Origin',(0.500000000000001,-2.1,-33.69)) ;
#121481=CARTESIAN_POINT('Origin',(-0.899999999999999,-1.9,-33.015)) ;
#121482=CARTESIAN_POINT('Origin',(-1.1,-1.9,-33.015)) ;
#121483=CARTESIAN_POINT('Origin',(-0.899999999999999,-2.1,-33.015)) ;
#121484=CARTESIAN_POINT('Origin',(-0.899999999999999,0.4,-34.69)) ;
#121485=CARTESIAN_POINT('Origin',(-0.899999999999999,0.4,-34.89)) ;
#121486=CARTESIAN_POINT('Origin',(0.500000000000001,-2.1,-34.29)) ;
#121487=CARTESIAN_POINT('Origin',(0.500000000000001,-2.1,-33.015)) ;
#121488=CARTESIAN_POINT('Origin',(0.600000000000001,-2.1,-33.015)) ;
#121489=CARTESIAN_POINT('Origin',(0.500000000000001,-2.1,-33.015)) ;
#121490=CARTESIAN_POINT('Origin',(-1.1,-4.42727195005762E-17,-33.015)) ;
#121491=CARTESIAN_POINT('',(-1.1,1.15,-32.915)) ;
#121492=CARTESIAN_POINT('',(-1.1,1.25,-32.915)) ;
#121493=CARTESIAN_POINT('Origin',(-1.1,1.15,-33.015)) ;
#121494=CARTESIAN_POINT('Origin',(-0.899999999999999,0.5,-34.89)) ;
#121495=CARTESIAN_POINT('Origin',(-0.899999999999999,-1.9,-34.89)) ;
#121496=CARTESIAN_POINT('Origin',(0.600000000000001,-1.9,-34.89)) ;
#121497=CARTESIAN_POINT('Origin',(0.500000000000001,-1.9,-34.89)) ;
#121498=CARTESIAN_POINT('Origin',(-0.899999999999999,-1.9,-34.89)) ;
#121499=CARTESIAN_POINT('Origin',(0.500000000000001,-1.9,-34.89)) ;
#121500=CARTESIAN_POINT('Origin',(0.500000000000001,-2.1,-34.89)) ;
#121501=CARTESIAN_POINT('Origin',(0.500000000000001,-2.1,-33.015)) ;
#121502=CARTESIAN_POINT('Origin',(0.500000000000001,-2.1,-33.015)) ;
#121503=CARTESIAN_POINT('Origin',(-1.1,-2.9,-32.815)) ;
#121504=CARTESIAN_POINT('Origin',(-1.1,-2.9,-32.815)) ;
#121505=CARTESIAN_POINT('Origin',(-1.1,-2.9,-32.815)) ;
#121506=CARTESIAN_POINT('Origin',(-1.1,1.25,-32.815)) ;
#121507=CARTESIAN_POINT('Origin',(-1.1,1.15,-32.815)) ;
#121508=CARTESIAN_POINT('Origin',(-1.1,1.15,-33.015)) ;
#121509=CARTESIAN_POINT('',(-1.1,1.25,-33.015)) ;
#121510=CARTESIAN_POINT('Origin',(-1.1,1.15,-33.015)) ;
#121511=CARTESIAN_POINT('Origin',(-1.1,1.15,-33.015)) ;
#121512=CARTESIAN_POINT('Origin',(-0.899999999999999,-1.9,-34.89)) ;
#121513=CARTESIAN_POINT('Origin',(-0.899999999999999,-1.9,-34.89)) ;
#121514=CARTESIAN_POINT('Origin',(0.500000000000001,-2.1,-34.29)) ;
#121515=CARTESIAN_POINT('Origin',(0.500000000000001,-2.1,-35.565)) ;
#121516=CARTESIAN_POINT('Origin',(0.500000000000001,1.36481920536411E-16,
-33.015)) ;
#121517=CARTESIAN_POINT('Origin',(0.500000000000001,-2.9,-33.015)) ;
#121518=CARTESIAN_POINT('Origin',(-0.999999999999999,-2.9,-32.815)) ;
#121519=CARTESIAN_POINT('Origin',(0.500000000000001,-2.9,-32.815)) ;
#121520=CARTESIAN_POINT('Origin',(-1.1,1.15,-33.015)) ;
#121521=CARTESIAN_POINT('Origin',(-1.1,1.35,-33.015)) ;
#121522=CARTESIAN_POINT('Origin',(-1.1,1.15,-34.29)) ;
#121523=CARTESIAN_POINT('',(-1.1,1.25,-35.565)) ;
#121524=CARTESIAN_POINT('',(-1.1,1.25,-35.665)) ;
#121525=CARTESIAN_POINT('Origin',(-1.1,1.15,-35.565)) ;
#121526=CARTESIAN_POINT('Origin',(-0.899999999999999,-1.9,-34.79)) ;
#121527=CARTESIAN_POINT('Origin',(-0.899999999999999,-1.9,-35.565)) ;
#121528=CARTESIAN_POINT('Origin',(-0.999999999999999,-2.1,-35.565)) ;
#121529=CARTESIAN_POINT('Origin',(0.500000000000001,-2.1,-35.565)) ;
#121530=CARTESIAN_POINT('Origin',(-0.899999999999999,-2.1,-35.565)) ;
#121531=CARTESIAN_POINT('Origin',(0.500000000000001,-2.1,-35.565)) ;
#121532=CARTESIAN_POINT('Origin',(0.500000000000001,-2.1,-35.565)) ;
#121533=CARTESIAN_POINT('Origin',(0.500000000000001,-2.9,-33.015)) ;
#121534=CARTESIAN_POINT('Origin',(0.700000000000002,-2.9,-33.015)) ;
#121535=CARTESIAN_POINT('Origin',(-1.1,1.35,-35.665)) ;
#121536=CARTESIAN_POINT('Origin',(-1.1,1.35,-35.565)) ;
#121537=CARTESIAN_POINT('Origin',(-1.1,1.15,-35.565)) ;
#121538=CARTESIAN_POINT('',(-1.1,1.15,-35.665)) ;
#121539=CARTESIAN_POINT('Origin',(-1.1,1.15,-35.565)) ;
#121540=CARTESIAN_POINT('Origin',(-1.1,1.15,-35.565)) ;
#121541=CARTESIAN_POINT('Origin',(-0.899999999999999,-1.9,-35.565)) ;
#121542=CARTESIAN_POINT('Origin',(-1.1,-1.9,-35.565)) ;
#121543=CARTESIAN_POINT('Origin',(0.500000000000001,-5.867447051098E-17,
-35.565)) ;
#121544=CARTESIAN_POINT('Origin',(0.500000000000001,-2.9,-35.565)) ;
#121545=CARTESIAN_POINT('Origin',(0.700000000000002,-2.9,-34.29)) ;
#121546=CARTESIAN_POINT('Origin',(0.700000000000002,-2.9,-35.565)) ;
#121547=CARTESIAN_POINT('Origin',(-1.1,1.15,-35.565)) ;
#121548=CARTESIAN_POINT('Origin',(-1.1,1.15,-35.765)) ;
#121549=CARTESIAN_POINT('Origin',(-1.1,-2.39429110547967E-16,-35.565)) ;
#121550=CARTESIAN_POINT('',(-1.1,1.25,-35.665)) ;
#121551=CARTESIAN_POINT('Origin',(0.500000000000001,-2.9,-35.565)) ;
#121552=CARTESIAN_POINT('Origin',(0.500000000000001,-2.9,-35.765)) ;
#121553=CARTESIAN_POINT('Origin',(-1.1,1.25,-35.765)) ;
#121554=CARTESIAN_POINT('Origin',(-1.1,-2.9,-35.765)) ;
#121555=CARTESIAN_POINT('Origin',(-1.1,-2.9,-35.765)) ;
#121556=CARTESIAN_POINT('Origin',(-1.1,-2.9,-35.765)) ;
#121557=CARTESIAN_POINT('Origin',(-1.1,-2.9,-35.765)) ;
#121558=CARTESIAN_POINT('Origin',(1.5,1.9,-33.69)) ;
#121559=CARTESIAN_POINT('Origin',(1.5,1.9,-35.84)) ;
#121560=CARTESIAN_POINT('Origin',(1.5,1.9,-34.89)) ;
#121561=CARTESIAN_POINT('Origin',(1.5,2.1,-34.89)) ;
#121562=CARTESIAN_POINT('Origin',(1.5,2.1,-34.69)) ;
#121563=CARTESIAN_POINT('Origin',(1.5,1.9,-35.84)) ;
#121564=CARTESIAN_POINT('Origin',(1.5,1.9,-35.84)) ;
#121565=CARTESIAN_POINT('Origin',(1.5,2.1,-34.69)) ;
#121566=CARTESIAN_POINT('Origin',(1.5,2.4,-34.69)) ;
#121567=CARTESIAN_POINT('Origin',(1.5,2.1,-35.84)) ;
#121568=CARTESIAN_POINT('Origin',(1.5,-2.15,-35.84)) ;
#121569=CARTESIAN_POINT('Origin',(1.5,2.4,-34.89)) ;
#121570=CARTESIAN_POINT('Origin',(1.5,2.6,-34.89)) ;
#121571=CARTESIAN_POINT('Origin',(1.5,-2.15,-35.84)) ;
#121572=CARTESIAN_POINT('Origin',(1.5,-2.15,-35.84)) ;
#121573=CARTESIAN_POINT('Origin',(1.5,2.6,-33.69)) ;
#121574=CARTESIAN_POINT('Origin',(1.5,2.6,-34.9985786437627)) ;
#121575=CARTESIAN_POINT('Origin',(1.5,-2.15,-33.69)) ;
#121576=CARTESIAN_POINT('Origin',(1.5,-2.15,-35.1931195934094)) ;
#121577=CARTESIAN_POINT('Origin',(1.5,2.6,-34.9985786437627)) ;
#121578=CARTESIAN_POINT('Origin',(1.5,2.6,-34.9985786437627)) ;
#121579=CARTESIAN_POINT('Origin',(1.5,-2.15,-35.1931195934094)) ;
#121580=CARTESIAN_POINT('Origin',(1.5,-2.15,-35.1931195934094)) ;
#121581=CARTESIAN_POINT('Origin',(1.5,1.69571067811865,-34.0942893218813)) ;
#121582=CARTESIAN_POINT('Origin',(1.5,3.15,-35.5485786437627)) ;
#121583=CARTESIAN_POINT('Origin',(1.5,-3.65625,-34.29)) ;
#121584=CARTESIAN_POINT('Origin',(1.5,-2.15,-33.3868804065906)) ;
#121585=CARTESIAN_POINT('Origin',(1.5,3.15,-35.5485786437627)) ;
#121586=CARTESIAN_POINT('Origin',(1.5,3.15,-35.5485786437627)) ;
#121587=CARTESIAN_POINT('Origin',(1.5,-2.15,-33.3868804065906)) ;
#121588=CARTESIAN_POINT('Origin',(1.5,-2.15,-33.3868804065906)) ;
#121589=CARTESIAN_POINT('Origin',(1.5,3.15,-33.69)) ;
#121590=CARTESIAN_POINT('Origin',(1.5,-2.15,-33.69)) ;
#121591=CARTESIAN_POINT('Origin',(1.5,-2.15,-32.74)) ;
#121592=CARTESIAN_POINT('Origin',(1.5,-2.15,-32.74)) ;
#121593=CARTESIAN_POINT('Origin',(1.5,-2.15,-32.74)) ;
#121594=CARTESIAN_POINT('Origin',(1.5,2.29571067811866,-33.8857106781187)) ;
#121595=CARTESIAN_POINT('Origin',(1.5,2.6,-33.5814213562373)) ;
#121596=CARTESIAN_POINT('Origin',(1.5,2.1,-32.74)) ;
#121597=CARTESIAN_POINT('Origin',(1.5,1.9,-32.74)) ;
#121598=CARTESIAN_POINT('Origin',(1.5,2.6,-33.5814213562373)) ;
#121599=CARTESIAN_POINT('Origin',(1.5,2.6,-33.5814213562373)) ;
#121600=CARTESIAN_POINT('Origin',(1.5,1.9,-32.74)) ;
#121601=CARTESIAN_POINT('Origin',(1.5,1.9,-32.74)) ;
#121602=CARTESIAN_POINT('Origin',(1.5,2.6,-33.69)) ;
#121603=CARTESIAN_POINT('Origin',(1.5,2.6,-33.69)) ;
#121604=CARTESIAN_POINT('Origin',(1.5,1.9,-33.69)) ;
#121605=CARTESIAN_POINT('Origin',(1.5,1.9,-33.69)) ;
#121606=CARTESIAN_POINT('Origin',(1.5,2.4,-33.69)) ;
#121607=CARTESIAN_POINT('Origin',(1.5,2.4,-33.89)) ;
#121608=CARTESIAN_POINT('Origin',(1.5,2.1,-33.69)) ;
#121609=CARTESIAN_POINT('Origin',(1.5,2.1,-33.89)) ;
#121610=CARTESIAN_POINT('Origin',(1.5,2.1,-33.89)) ;
#121611=CARTESIAN_POINT('Origin',(-0.4,-0.600000000000001,-3.41)) ;
#121612=CARTESIAN_POINT('',(-0.4,-0.600000000000001,-3.51)) ;
#121613=CARTESIAN_POINT('',(-0.4,-0.600000000000001,-4.11)) ;
#121614=CARTESIAN_POINT('',(-0.4,-0.600000000000001,-3.41)) ;
#121615=CARTESIAN_POINT('',(-0.4,-6.05857864376269,-4.11)) ;
#121616=CARTESIAN_POINT('',(-0.4,-0.600000000000001,-4.11)) ;
#121617=CARTESIAN_POINT('',(-0.4,-6.05857864376269,-3.51)) ;
#121618=CARTESIAN_POINT('',(-0.4,-6.05857864376269,-3.41)) ;
#121619=CARTESIAN_POINT('',(-0.4,-0.600000000000001,-3.51)) ;
#121620=CARTESIAN_POINT('Origin',(-0.4,-6.1,-3.41)) ;
#121621=CARTESIAN_POINT('',(-0.129289321881346,-6.37071067811866,-3.86857864376269)) ;
#121622=CARTESIAN_POINT('',(-0.129289321881346,-6.37071067811866,-3.75142135623731)) ;
#121623=CARTESIAN_POINT('',(-0.129289321881346,-6.37071067811866,-3.41)) ;
#121624=CARTESIAN_POINT('',(-0.370710678118655,-6.12928932188134,-3.51)) ;
#121625=CARTESIAN_POINT('',(-0.423570226039552,-6.07642977396045,-3.4571404520791)) ;
#121626=CARTESIAN_POINT('',(-0.370710678118655,-6.12928932188134,-4.11)) ;
#121627=CARTESIAN_POINT('',(-0.370710678118655,-6.12928932188134,-3.41)) ;
#121628=CARTESIAN_POINT('',(-0.156903559372885,-6.34309644062712,-3.89619288125423)) ;
#121629=CARTESIAN_POINT('Origin',(-0.1,-6.4,-3.41)) ;
#121630=CARTESIAN_POINT('',(0.0585786437626908,-6.4,-3.86857864376269)) ;
#121631=CARTESIAN_POINT('',(0.0585786437626908,-6.4,-3.75142135623731)) ;
#121632=CARTESIAN_POINT('',(0.0585786437626908,-6.4,-3.41)) ;
#121633=CARTESIAN_POINT('',(-0.0585786437626908,-6.4,-3.75142135623731)) ;
#121634=CARTESIAN_POINT('',(-0.1,-6.4,-3.75142135623731)) ;
#121635=CARTESIAN_POINT('',(-0.0585786437626908,-6.4,-3.86857864376269)) ;
#121636=CARTESIAN_POINT('',(-0.0585786437626908,-6.4,-3.41)) ;
#121637=CARTESIAN_POINT('',(-0.1,-6.4,-3.86857864376269)) ;
#121638=CARTESIAN_POINT('Origin',(0.1,-6.4,-3.41)) ;
#121639=CARTESIAN_POINT('',(0.370710678118655,-6.12928932188134,-4.11)) ;
#121640=CARTESIAN_POINT('',(0.370710678118655,-6.12928932188134,-3.51)) ;
#121641=CARTESIAN_POINT('',(0.370710678118655,-6.12928932188134,-3.41)) ;
#121642=CARTESIAN_POINT('',(0.129289321881346,-6.37071067811866,-3.75142135623731)) ;
#121643=CARTESIAN_POINT('',(0.223570226039552,-6.27642977396045,-3.6571404520791)) ;
#121644=CARTESIAN_POINT('',(0.129289321881346,-6.37071067811866,-3.86857864376269)) ;
#121645=CARTESIAN_POINT('',(0.129289321881346,-6.37071067811866,-3.41)) ;
#121646=CARTESIAN_POINT('',(-0.0430964406271149,-6.54309644062712,-3.69619288125423)) ;
#121647=CARTESIAN_POINT('Origin',(0.4,-6.1,-3.41)) ;
#121648=CARTESIAN_POINT('',(0.4,-6.05857864376269,-3.51)) ;
#121649=CARTESIAN_POINT('',(0.4,-6.05857864376269,-4.11)) ;
#121650=CARTESIAN_POINT('',(0.4,-6.05857864376269,-3.41)) ;
#121651=CARTESIAN_POINT('',(0.4,-0.6,-4.11)) ;
#121652=CARTESIAN_POINT('',(0.4,-6.1,-4.11)) ;
#121653=CARTESIAN_POINT('',(0.4,-0.6,-3.51)) ;
#121654=CARTESIAN_POINT('',(0.4,-0.6,-3.41)) ;
#121655=CARTESIAN_POINT('',(0.4,-6.05857864376269,-3.51)) ;
#121656=CARTESIAN_POINT('Origin',(0.6,-0.600000000000001,-3.41)) ;
#121657=CARTESIAN_POINT('',(0.3,-6.05857864376269,-3.41)) ;
#121658=CARTESIAN_POINT('',(0.3,-0.6,-3.41)) ;
#121659=CARTESIAN_POINT('',(0.3,-0.6,-3.41)) ;
#121660=CARTESIAN_POINT('Origin',(0.6,-0.6,-3.41)) ;
#121661=CARTESIAN_POINT('',(-0.3,-0.600000000000001,-3.41)) ;
#121662=CARTESIAN_POINT('Origin',(0.6,-0.600000000000001,-3.41)) ;
#121663=CARTESIAN_POINT('',(-0.299999999999999,-6.05857864376269,-3.41)) ;
#121664=CARTESIAN_POINT('',(-0.3,-0.600000000000001,-3.41)) ;
#121665=CARTESIAN_POINT('',(0.4,-6.05857864376269,-3.41)) ;
#121666=CARTESIAN_POINT('Origin',(0.6,-0.600000000000001,-4.21)) ;
#121667=CARTESIAN_POINT('',(-0.300000000000001,-6.05857864376269,-4.21)) ;
#121668=CARTESIAN_POINT('',(-0.3,-0.600000000000001,-4.21)) ;
#121669=CARTESIAN_POINT('',(-0.3,-0.600000000000001,-4.21)) ;
#121670=CARTESIAN_POINT('Origin',(0.6,-0.600000000000001,-4.21)) ;
#121671=CARTESIAN_POINT('',(0.3,-0.6,-4.21)) ;
#121672=CARTESIAN_POINT('Origin',(0.6,-0.6,-4.21)) ;
#121673=CARTESIAN_POINT('',(0.3,-6.05857864376269,-4.21)) ;
#121674=CARTESIAN_POINT('',(0.3,-0.600000000000001,-4.21)) ;
#121675=CARTESIAN_POINT('',(0.6,-6.05857864376269,-4.21)) ;
#121676=CARTESIAN_POINT('Origin',(0.6,-0.600000000000001,-3.41)) ;
#121677=CARTESIAN_POINT('Origin',(0.6,-0.600000000000001,-4.11)) ;
#121678=CARTESIAN_POINT('Origin',(0.6,-0.600000000000001,-3.51)) ;
#121679=CARTESIAN_POINT('Origin',(0.6,-0.6,-3.41)) ;
#121680=CARTESIAN_POINT('Origin',(0.6,-0.6,-4.11)) ;
#121681=CARTESIAN_POINT('Origin',(0.6,-0.6,-3.51)) ;
#121682=CARTESIAN_POINT('Origin',(7.,0.1,-3.41)) ;
#121683=CARTESIAN_POINT('',(6.72928932188135,0.370710678118655,-4.11)) ;
#121684=CARTESIAN_POINT('',(6.72928932188135,0.370710678118655,-3.51)) ;
#121685=CARTESIAN_POINT('',(6.72928932188135,0.370710678118655,-3.41)) ;
#121686=CARTESIAN_POINT('',(6.97071067811866,0.129289321881346,-3.75142135623731)) ;
#121687=CARTESIAN_POINT('',(6.87642977396045,0.223570226039552,-3.6571404520791)) ;
#121688=CARTESIAN_POINT('',(6.97071067811866,0.129289321881346,-3.86857864376269)) ;
#121689=CARTESIAN_POINT('',(6.97071067811866,0.129289321881346,-3.41)) ;
#121690=CARTESIAN_POINT('',(7.14309644062712,-0.0430964406271146,-3.69619288125423)) ;
#121691=CARTESIAN_POINT('Origin',(6.7,0.400000000000001,-3.41)) ;
#121692=CARTESIAN_POINT('',(6.65857864376269,0.400000000000001,-3.51)) ;
#121693=CARTESIAN_POINT('',(6.65857864376269,0.400000000000001,-4.11)) ;
#121694=CARTESIAN_POINT('',(6.65857864376269,0.400000000000001,-3.41)) ;
#121695=CARTESIAN_POINT('',(6.7,0.400000000000001,-4.11)) ;
#121696=CARTESIAN_POINT('',(6.65857864376269,0.400000000000001,-3.51)) ;
#121697=CARTESIAN_POINT('Origin',(0.6,-0.4,-3.41)) ;
#121698=CARTESIAN_POINT('',(6.65857864376269,-0.400000000000001,-4.11)) ;
#121699=CARTESIAN_POINT('',(0.6,-0.4,-4.11)) ;
#121700=CARTESIAN_POINT('',(6.65857864376269,-0.400000000000001,-3.51)) ;
#121701=CARTESIAN_POINT('',(6.65857864376269,-0.400000000000001,-3.41)) ;
#121702=CARTESIAN_POINT('',(2.4,-0.4,-3.51)) ;
#121703=CARTESIAN_POINT('Origin',(6.7,-0.400000000000001,-3.41)) ;
#121704=CARTESIAN_POINT('',(6.97071067811866,-0.129289321881346,-3.86857864376269)) ;
#121705=CARTESIAN_POINT('',(6.97071067811866,-0.129289321881346,-3.75142135623731)) ;
#121706=CARTESIAN_POINT('',(6.97071067811866,-0.129289321881346,-3.41)) ;
#121707=CARTESIAN_POINT('',(6.72928932188135,-0.370710678118655,-3.51)) ;
#121708=CARTESIAN_POINT('',(6.67642977396045,-0.423570226039552,-3.4571404520791)) ;
#121709=CARTESIAN_POINT('',(6.72928932188135,-0.370710678118655,-4.11)) ;
#121710=CARTESIAN_POINT('',(6.72928932188135,-0.370710678118655,-3.41)) ;
#121711=CARTESIAN_POINT('',(6.94309644062712,-0.156903559372885,-3.89619288125423)) ;
#121712=CARTESIAN_POINT('Origin',(7.,-0.1,-3.41)) ;
#121713=CARTESIAN_POINT('',(7.,-0.0585786437626909,-3.75142135623731)) ;
#121714=CARTESIAN_POINT('',(7.,-0.0585786437626909,-3.86857864376269)) ;
#121715=CARTESIAN_POINT('',(7.,-0.0585786437626909,-3.41)) ;
#121716=CARTESIAN_POINT('',(7.,0.0585786437626909,-3.86857864376269)) ;
#121717=CARTESIAN_POINT('',(7.,-0.1,-3.86857864376269)) ;
#121718=CARTESIAN_POINT('',(7.,0.0585786437626909,-3.75142135623731)) ;
#121719=CARTESIAN_POINT('',(7.,0.0585786437626909,-3.41)) ;
#121720=CARTESIAN_POINT('',(7.,-0.1,-3.75142135623731)) ;
#121721=CARTESIAN_POINT('Origin',(0.6,-0.600000000000001,-3.41)) ;
#121722=CARTESIAN_POINT('',(6.65857864376269,-0.300000000000001,-3.41)) ;
#121723=CARTESIAN_POINT('',(6.65857864376269,0.3,-3.41)) ;
#121724=CARTESIAN_POINT('',(6.65857864376269,-0.399999999999999,-3.41)) ;
#121725=CARTESIAN_POINT('',(2.4,0.3,-3.41)) ;
#121726=CARTESIAN_POINT('',(6.65857864376269,-0.300000000000001,-3.41)) ;
#121727=CARTESIAN_POINT('Origin',(0.6,-0.600000000000001,-4.21)) ;
#121728=CARTESIAN_POINT('',(6.65857864376269,0.300000000000001,-4.21)) ;
#121729=CARTESIAN_POINT('',(0.6,0.299999999999999,-4.21)) ;
#121730=CARTESIAN_POINT('',(6.65857864376269,-0.300000000000001,-4.21)) ;
#121731=CARTESIAN_POINT('',(6.65857864376269,-0.6,-4.21)) ;
#121732=CARTESIAN_POINT('',(0.6,-0.3,-4.21)) ;
#121733=CARTESIAN_POINT('Origin',(-0.4,-0.600000000000001,-7.22)) ;
#121734=CARTESIAN_POINT('',(-0.4,-0.600000000000001,-7.32)) ;
#121735=CARTESIAN_POINT('',(-0.4,-0.600000000000001,-7.92)) ;
#121736=CARTESIAN_POINT('',(-0.4,-0.600000000000001,-7.22)) ;
#121737=CARTESIAN_POINT('',(-0.4,-6.05857864376269,-7.92)) ;
#121738=CARTESIAN_POINT('',(-0.4,-0.600000000000001,-7.92)) ;
#121739=CARTESIAN_POINT('',(-0.4,-6.05857864376269,-7.32)) ;
#121740=CARTESIAN_POINT('',(-0.4,-6.05857864376269,-7.22)) ;
#121741=CARTESIAN_POINT('',(-0.4,-0.600000000000001,-7.32)) ;
#121742=CARTESIAN_POINT('Origin',(-0.4,-6.1,-7.22)) ;
#121743=CARTESIAN_POINT('',(-0.129289321881345,-6.37071067811866,-7.67857864376269)) ;
#121744=CARTESIAN_POINT('',(-0.129289321881346,-6.37071067811866,-7.56142135623731)) ;
#121745=CARTESIAN_POINT('',(-0.129289321881346,-6.37071067811866,-7.22)) ;
#121746=CARTESIAN_POINT('',(-0.370710678118655,-6.12928932188134,-7.32)) ;
#121747=CARTESIAN_POINT('',(-0.423570226039552,-6.07642977396045,-7.2671404520791)) ;
#121748=CARTESIAN_POINT('',(-0.370710678118655,-6.12928932188134,-7.92)) ;
#121749=CARTESIAN_POINT('',(-0.370710678118655,-6.12928932188134,-7.22)) ;
#121750=CARTESIAN_POINT('',(-0.156903559372885,-6.34309644062712,-7.70619288125423)) ;
#121751=CARTESIAN_POINT('Origin',(-0.1,-6.4,-7.22)) ;
#121752=CARTESIAN_POINT('',(0.0585786437626908,-6.4,-7.67857864376269)) ;
#121753=CARTESIAN_POINT('',(0.0585786437626908,-6.4,-7.56142135623731)) ;
#121754=CARTESIAN_POINT('',(0.0585786437626908,-6.4,-7.22)) ;
#121755=CARTESIAN_POINT('',(-0.0585786437626908,-6.4,-7.56142135623731)) ;
#121756=CARTESIAN_POINT('',(-0.1,-6.4,-7.56142135623731)) ;
#121757=CARTESIAN_POINT('',(-0.0585786437626908,-6.4,-7.67857864376269)) ;
#121758=CARTESIAN_POINT('',(-0.0585786437626908,-6.4,-7.22)) ;
#121759=CARTESIAN_POINT('',(-0.1,-6.4,-7.67857864376269)) ;
#121760=CARTESIAN_POINT('Origin',(0.1,-6.4,-7.22)) ;
#121761=CARTESIAN_POINT('',(0.370710678118655,-6.12928932188134,-7.92)) ;
#121762=CARTESIAN_POINT('',(0.370710678118655,-6.12928932188134,-7.32)) ;
#121763=CARTESIAN_POINT('',(0.370710678118655,-6.12928932188134,-7.22)) ;
#121764=CARTESIAN_POINT('',(0.129289321881346,-6.37071067811866,-7.56142135623731)) ;
#121765=CARTESIAN_POINT('',(0.223570226039553,-6.27642977396045,-7.4671404520791)) ;
#121766=CARTESIAN_POINT('',(0.129289321881346,-6.37071067811866,-7.67857864376269)) ;
#121767=CARTESIAN_POINT('',(0.129289321881346,-6.37071067811866,-7.22)) ;
#121768=CARTESIAN_POINT('',(-0.0430964406271151,-6.54309644062712,-7.50619288125423)) ;
#121769=CARTESIAN_POINT('Origin',(0.4,-6.1,-7.22)) ;
#121770=CARTESIAN_POINT('',(0.4,-6.05857864376269,-7.32)) ;
#121771=CARTESIAN_POINT('',(0.4,-6.05857864376269,-7.92)) ;
#121772=CARTESIAN_POINT('',(0.4,-6.05857864376269,-7.22)) ;
#121773=CARTESIAN_POINT('',(0.4,-0.6,-7.92)) ;
#121774=CARTESIAN_POINT('',(0.4,-6.1,-7.92)) ;
#121775=CARTESIAN_POINT('',(0.4,-0.6,-7.32)) ;
#121776=CARTESIAN_POINT('',(0.4,-0.6,-7.22)) ;
#121777=CARTESIAN_POINT('',(0.4,-6.05857864376269,-7.32)) ;
#121778=CARTESIAN_POINT('Origin',(0.6,-0.600000000000001,-7.22)) ;
#121779=CARTESIAN_POINT('',(0.3,-6.05857864376269,-7.22)) ;
#121780=CARTESIAN_POINT('',(0.3,-0.6,-7.22)) ;
#121781=CARTESIAN_POINT('',(0.3,-0.6,-7.22)) ;
#121782=CARTESIAN_POINT('Origin',(0.6,-0.6,-7.22)) ;
#121783=CARTESIAN_POINT('',(-0.3,-0.600000000000001,-7.22)) ;
#121784=CARTESIAN_POINT('Origin',(0.6,-0.600000000000001,-7.22)) ;
#121785=CARTESIAN_POINT('',(-0.300000000000001,-6.05857864376269,-7.22)) ;
#121786=CARTESIAN_POINT('',(-0.3,-0.600000000000001,-7.22)) ;
#121787=CARTESIAN_POINT('',(0.4,-6.05857864376269,-7.22)) ;
#121788=CARTESIAN_POINT('Origin',(0.6,-0.600000000000001,-8.02)) ;
#121789=CARTESIAN_POINT('',(-0.299999999999999,-6.05857864376269,-8.02)) ;
#121790=CARTESIAN_POINT('',(-0.3,-0.600000000000001,-8.02)) ;
#121791=CARTESIAN_POINT('',(-0.3,-0.600000000000001,-8.02)) ;
#121792=CARTESIAN_POINT('Origin',(0.6,-0.600000000000001,-8.02)) ;
#121793=CARTESIAN_POINT('',(0.3,-0.6,-8.02)) ;
#121794=CARTESIAN_POINT('Origin',(0.6,-0.6,-8.02)) ;
#121795=CARTESIAN_POINT('',(0.3,-6.05857864376269,-8.02)) ;
#121796=CARTESIAN_POINT('',(0.3,-0.600000000000001,-8.02)) ;
#121797=CARTESIAN_POINT('',(0.6,-6.05857864376269,-8.02)) ;
#121798=CARTESIAN_POINT('Origin',(0.6,-0.600000000000001,-7.22)) ;
#121799=CARTESIAN_POINT('Origin',(0.6,-0.600000000000001,-7.92)) ;
#121800=CARTESIAN_POINT('Origin',(0.6,-0.600000000000001,-7.32)) ;
#121801=CARTESIAN_POINT('Origin',(0.6,-0.6,-7.22)) ;
#121802=CARTESIAN_POINT('Origin',(0.6,-0.6,-7.92)) ;
#121803=CARTESIAN_POINT('Origin',(0.6,-0.6,-7.32)) ;
#121804=CARTESIAN_POINT('Origin',(7.,0.1,-7.22)) ;
#121805=CARTESIAN_POINT('',(6.72928932188135,0.370710678118655,-7.92)) ;
#121806=CARTESIAN_POINT('',(6.72928932188135,0.370710678118655,-7.32)) ;
#121807=CARTESIAN_POINT('',(6.72928932188135,0.370710678118655,-7.22)) ;
#121808=CARTESIAN_POINT('',(6.97071067811866,0.129289321881346,-7.56142135623731)) ;
#121809=CARTESIAN_POINT('',(6.87642977396045,0.223570226039553,-7.4671404520791)) ;
#121810=CARTESIAN_POINT('',(6.97071067811866,0.129289321881346,-7.67857864376269)) ;
#121811=CARTESIAN_POINT('',(6.97071067811866,0.129289321881346,-7.22)) ;
#121812=CARTESIAN_POINT('',(7.14309644062712,-0.0430964406271152,-7.50619288125423)) ;
#121813=CARTESIAN_POINT('Origin',(6.7,0.400000000000001,-7.22)) ;
#121814=CARTESIAN_POINT('',(6.65857864376269,0.400000000000001,-7.32)) ;
#121815=CARTESIAN_POINT('',(6.65857864376269,0.400000000000001,-7.92)) ;
#121816=CARTESIAN_POINT('',(6.65857864376269,0.400000000000001,-7.22)) ;
#121817=CARTESIAN_POINT('',(6.7,0.400000000000001,-7.92)) ;
#121818=CARTESIAN_POINT('',(6.65857864376269,0.400000000000001,-7.32)) ;
#121819=CARTESIAN_POINT('Origin',(0.6,-0.4,-7.22)) ;
#121820=CARTESIAN_POINT('',(6.65857864376269,-0.400000000000001,-7.92)) ;
#121821=CARTESIAN_POINT('',(0.6,-0.4,-7.92)) ;
#121822=CARTESIAN_POINT('',(6.65857864376269,-0.400000000000001,-7.32)) ;
#121823=CARTESIAN_POINT('',(6.65857864376269,-0.400000000000001,-7.22)) ;
#121824=CARTESIAN_POINT('',(2.4,-0.4,-7.32)) ;
#121825=CARTESIAN_POINT('Origin',(6.7,-0.400000000000001,-7.22)) ;
#121826=CARTESIAN_POINT('',(6.97071067811866,-0.129289321881346,-7.67857864376269)) ;
#121827=CARTESIAN_POINT('',(6.97071067811866,-0.129289321881346,-7.56142135623731)) ;
#121828=CARTESIAN_POINT('',(6.97071067811866,-0.129289321881346,-7.22)) ;
#121829=CARTESIAN_POINT('',(6.72928932188135,-0.370710678118655,-7.32)) ;
#121830=CARTESIAN_POINT('',(6.67642977396045,-0.423570226039553,-7.2671404520791)) ;
#121831=CARTESIAN_POINT('',(6.72928932188135,-0.370710678118655,-7.92)) ;
#121832=CARTESIAN_POINT('',(6.72928932188135,-0.370710678118655,-7.22)) ;
#121833=CARTESIAN_POINT('',(6.94309644062712,-0.156903559372885,-7.70619288125423)) ;
#121834=CARTESIAN_POINT('Origin',(7.,-0.1,-7.22)) ;
#121835=CARTESIAN_POINT('',(7.,-0.0585786437626909,-7.56142135623731)) ;
#121836=CARTESIAN_POINT('',(7.,-0.0585786437626909,-7.67857864376269)) ;
#121837=CARTESIAN_POINT('',(7.,-0.0585786437626909,-7.22)) ;
#121838=CARTESIAN_POINT('',(7.,0.0585786437626909,-7.67857864376269)) ;
#121839=CARTESIAN_POINT('',(7.,-0.1,-7.67857864376269)) ;
#121840=CARTESIAN_POINT('',(7.,0.0585786437626909,-7.56142135623731)) ;
#121841=CARTESIAN_POINT('',(7.,0.0585786437626909,-7.22)) ;
#121842=CARTESIAN_POINT('',(7.,-0.1,-7.56142135623731)) ;
#121843=CARTESIAN_POINT('Origin',(0.6,-0.600000000000001,-7.22)) ;
#121844=CARTESIAN_POINT('',(6.65857864376269,-0.300000000000001,-7.22)) ;
#121845=CARTESIAN_POINT('',(6.65857864376269,0.300000000000002,-7.22)) ;
#121846=CARTESIAN_POINT('',(6.65857864376269,-0.399999999999999,-7.22)) ;
#121847=CARTESIAN_POINT('',(2.4,0.3,-7.22)) ;
#121848=CARTESIAN_POINT('',(6.65857864376269,-0.300000000000001,-7.22)) ;
#121849=CARTESIAN_POINT('Origin',(0.6,-0.600000000000001,-8.02)) ;
#121850=CARTESIAN_POINT('',(6.65857864376269,0.300000000000002,-8.02)) ;
#121851=CARTESIAN_POINT('',(0.6,0.299999999999999,-8.02)) ;
#121852=CARTESIAN_POINT('',(6.65857864376269,-0.300000000000001,-8.02)) ;
#121853=CARTESIAN_POINT('',(6.65857864376269,-0.6,-8.02)) ;
#121854=CARTESIAN_POINT('',(0.6,-0.3,-8.02)) ;
#121855=CARTESIAN_POINT('Origin',(-0.4,-0.600000000000001,-11.03)) ;
#121856=CARTESIAN_POINT('',(-0.4,-0.600000000000001,-11.13)) ;
#121857=CARTESIAN_POINT('',(-0.4,-0.600000000000001,-11.73)) ;
#121858=CARTESIAN_POINT('',(-0.4,-0.600000000000001,-11.03)) ;
#121859=CARTESIAN_POINT('',(-0.4,-6.05857864376269,-11.73)) ;
#121860=CARTESIAN_POINT('',(-0.4,-0.600000000000001,-11.73)) ;
#121861=CARTESIAN_POINT('',(-0.4,-6.05857864376269,-11.13)) ;
#121862=CARTESIAN_POINT('',(-0.4,-6.05857864376269,-11.03)) ;
#121863=CARTESIAN_POINT('',(-0.4,-0.600000000000001,-11.13)) ;
#121864=CARTESIAN_POINT('Origin',(-0.4,-6.1,-11.03)) ;
#121865=CARTESIAN_POINT('',(-0.129289321881346,-6.37071067811866,-11.4885786437627)) ;
#121866=CARTESIAN_POINT('',(-0.129289321881346,-6.37071067811866,-11.3714213562373)) ;
#121867=CARTESIAN_POINT('',(-0.129289321881346,-6.37071067811866,-11.03)) ;
#121868=CARTESIAN_POINT('',(-0.370710678118655,-6.12928932188134,-11.13)) ;
#121869=CARTESIAN_POINT('',(-0.423570226039552,-6.07642977396045,-11.0771404520791)) ;
#121870=CARTESIAN_POINT('',(-0.370710678118655,-6.12928932188134,-11.73)) ;
#121871=CARTESIAN_POINT('',(-0.370710678118655,-6.12928932188134,-11.03)) ;
#121872=CARTESIAN_POINT('',(-0.156903559372884,-6.34309644062712,-11.5161928812542)) ;
#121873=CARTESIAN_POINT('Origin',(-0.1,-6.4,-11.03)) ;
#121874=CARTESIAN_POINT('',(0.0585786437626908,-6.4,-11.4885786437627)) ;
#121875=CARTESIAN_POINT('',(0.0585786437626908,-6.4,-11.3714213562373)) ;
#121876=CARTESIAN_POINT('',(0.0585786437626908,-6.4,-11.03)) ;
#121877=CARTESIAN_POINT('',(-0.0585786437626908,-6.4,-11.3714213562373)) ;
#121878=CARTESIAN_POINT('',(-0.1,-6.4,-11.3714213562373)) ;
#121879=CARTESIAN_POINT('',(-0.0585786437626908,-6.4,-11.4885786437627)) ;
#121880=CARTESIAN_POINT('',(-0.0585786437626908,-6.4,-11.03)) ;
#121881=CARTESIAN_POINT('',(-0.1,-6.4,-11.4885786437627)) ;
#121882=CARTESIAN_POINT('Origin',(0.1,-6.4,-11.03)) ;
#121883=CARTESIAN_POINT('',(0.370710678118655,-6.12928932188134,-11.73)) ;
#121884=CARTESIAN_POINT('',(0.370710678118655,-6.12928932188134,-11.13)) ;
#121885=CARTESIAN_POINT('',(0.370710678118655,-6.12928932188134,-11.03)) ;
#121886=CARTESIAN_POINT('',(0.129289321881346,-6.37071067811866,-11.3714213562373)) ;
#121887=CARTESIAN_POINT('',(0.223570226039553,-6.27642977396045,-11.2771404520791)) ;
#121888=CARTESIAN_POINT('',(0.129289321881346,-6.37071067811866,-11.4885786437627)) ;
#121889=CARTESIAN_POINT('',(0.129289321881346,-6.37071067811866,-11.03)) ;
#121890=CARTESIAN_POINT('',(-0.0430964406271157,-6.54309644062712,-11.3161928812542)) ;
#121891=CARTESIAN_POINT('Origin',(0.4,-6.1,-11.03)) ;
#121892=CARTESIAN_POINT('',(0.4,-6.05857864376269,-11.13)) ;
#121893=CARTESIAN_POINT('',(0.4,-6.05857864376269,-11.73)) ;
#121894=CARTESIAN_POINT('',(0.4,-6.05857864376269,-11.03)) ;
#121895=CARTESIAN_POINT('',(0.4,-0.6,-11.73)) ;
#121896=CARTESIAN_POINT('',(0.4,-6.1,-11.73)) ;
#121897=CARTESIAN_POINT('',(0.4,-0.6,-11.13)) ;
#121898=CARTESIAN_POINT('',(0.4,-0.6,-11.03)) ;
#121899=CARTESIAN_POINT('',(0.4,-6.05857864376269,-11.13)) ;
#121900=CARTESIAN_POINT('Origin',(0.6,-0.600000000000001,-11.03)) ;
#121901=CARTESIAN_POINT('',(0.3,-6.05857864376269,-11.03)) ;
#121902=CARTESIAN_POINT('',(0.3,-0.6,-11.03)) ;
#121903=CARTESIAN_POINT('',(0.3,-0.6,-11.03)) ;
#121904=CARTESIAN_POINT('Origin',(0.6,-0.6,-11.03)) ;
#121905=CARTESIAN_POINT('',(-0.3,-0.600000000000001,-11.03)) ;
#121906=CARTESIAN_POINT('Origin',(0.6,-0.600000000000001,-11.03)) ;
#121907=CARTESIAN_POINT('',(-0.300000000000003,-6.05857864376269,-11.03)) ;
#121908=CARTESIAN_POINT('',(-0.3,-0.600000000000001,-11.03)) ;
#121909=CARTESIAN_POINT('',(0.4,-6.05857864376269,-11.03)) ;
#121910=CARTESIAN_POINT('Origin',(0.6,-0.600000000000001,-11.83)) ;
#121911=CARTESIAN_POINT('',(-0.299999999999999,-6.05857864376269,-11.83)) ;
#121912=CARTESIAN_POINT('',(-0.3,-0.600000000000001,-11.83)) ;
#121913=CARTESIAN_POINT('',(-0.3,-0.600000000000001,-11.83)) ;
#121914=CARTESIAN_POINT('Origin',(0.6,-0.600000000000001,-11.83)) ;
#121915=CARTESIAN_POINT('',(0.3,-0.6,-11.83)) ;
#121916=CARTESIAN_POINT('Origin',(0.6,-0.6,-11.83)) ;
#121917=CARTESIAN_POINT('',(0.3,-6.05857864376269,-11.83)) ;
#121918=CARTESIAN_POINT('',(0.3,-0.600000000000001,-11.83)) ;
#121919=CARTESIAN_POINT('',(0.6,-6.05857864376269,-11.83)) ;
#121920=CARTESIAN_POINT('Origin',(0.6,-0.600000000000001,-11.03)) ;
#121921=CARTESIAN_POINT('Origin',(0.6,-0.600000000000001,-11.73)) ;
#121922=CARTESIAN_POINT('Origin',(0.6,-0.600000000000001,-11.13)) ;
#121923=CARTESIAN_POINT('Origin',(0.6,-0.6,-11.03)) ;
#121924=CARTESIAN_POINT('Origin',(0.6,-0.6,-11.73)) ;
#121925=CARTESIAN_POINT('Origin',(0.6,-0.6,-11.13)) ;
#121926=CARTESIAN_POINT('Origin',(7.,0.1,-11.03)) ;
#121927=CARTESIAN_POINT('',(6.72928932188135,0.370710678118655,-11.73)) ;
#121928=CARTESIAN_POINT('',(6.72928932188135,0.370710678118655,-11.13)) ;
#121929=CARTESIAN_POINT('',(6.72928932188135,0.370710678118655,-11.03)) ;
#121930=CARTESIAN_POINT('',(6.97071067811866,0.129289321881346,-11.3714213562373)) ;
#121931=CARTESIAN_POINT('',(6.87642977396045,0.223570226039553,-11.2771404520791)) ;
#121932=CARTESIAN_POINT('',(6.97071067811866,0.129289321881346,-11.4885786437627)) ;
#121933=CARTESIAN_POINT('',(6.97071067811866,0.129289321881346,-11.03)) ;
#121934=CARTESIAN_POINT('',(7.14309644062712,-0.0430964406271147,-11.3161928812542)) ;
#121935=CARTESIAN_POINT('Origin',(6.7,0.400000000000001,-11.03)) ;
#121936=CARTESIAN_POINT('',(6.65857864376269,0.400000000000001,-11.13)) ;
#121937=CARTESIAN_POINT('',(6.65857864376269,0.400000000000001,-11.73)) ;
#121938=CARTESIAN_POINT('',(6.65857864376269,0.400000000000001,-11.03)) ;
#121939=CARTESIAN_POINT('',(6.7,0.400000000000001,-11.73)) ;
#121940=CARTESIAN_POINT('',(6.65857864376269,0.400000000000001,-11.13)) ;
#121941=CARTESIAN_POINT('Origin',(0.6,-0.4,-11.03)) ;
#121942=CARTESIAN_POINT('',(6.65857864376269,-0.400000000000001,-11.73)) ;
#121943=CARTESIAN_POINT('',(0.6,-0.4,-11.73)) ;
#121944=CARTESIAN_POINT('',(6.65857864376269,-0.400000000000001,-11.13)) ;
#121945=CARTESIAN_POINT('',(6.65857864376269,-0.400000000000001,-11.03)) ;
#121946=CARTESIAN_POINT('',(2.4,-0.4,-11.13)) ;
#121947=CARTESIAN_POINT('Origin',(6.7,-0.400000000000001,-11.03)) ;
#121948=CARTESIAN_POINT('',(6.97071067811866,-0.129289321881346,-11.4885786437627)) ;
#121949=CARTESIAN_POINT('',(6.97071067811866,-0.129289321881346,-11.3714213562373)) ;
#121950=CARTESIAN_POINT('',(6.97071067811866,-0.129289321881346,-11.03)) ;
#121951=CARTESIAN_POINT('',(6.72928932188135,-0.370710678118655,-11.13)) ;
#121952=CARTESIAN_POINT('',(6.67642977396045,-0.423570226039553,-11.0771404520791)) ;
#121953=CARTESIAN_POINT('',(6.72928932188135,-0.370710678118655,-11.73)) ;
#121954=CARTESIAN_POINT('',(6.72928932188135,-0.370710678118655,-11.03)) ;
#121955=CARTESIAN_POINT('',(6.94309644062712,-0.156903559372885,-11.5161928812542)) ;
#121956=CARTESIAN_POINT('Origin',(7.,-0.1,-11.03)) ;
#121957=CARTESIAN_POINT('',(7.,-0.0585786437626909,-11.3714213562373)) ;
#121958=CARTESIAN_POINT('',(7.,-0.0585786437626909,-11.4885786437627)) ;
#121959=CARTESIAN_POINT('',(7.,-0.0585786437626909,-11.03)) ;
#121960=CARTESIAN_POINT('',(7.,0.0585786437626909,-11.4885786437627)) ;
#121961=CARTESIAN_POINT('',(7.,-0.1,-11.4885786437627)) ;
#121962=CARTESIAN_POINT('',(7.,0.0585786437626909,-11.3714213562373)) ;
#121963=CARTESIAN_POINT('',(7.,0.0585786437626909,-11.03)) ;
#121964=CARTESIAN_POINT('',(7.,-0.1,-11.3714213562373)) ;
#121965=CARTESIAN_POINT('Origin',(0.6,-0.600000000000001,-11.03)) ;
#121966=CARTESIAN_POINT('',(6.65857864376269,-0.300000000000001,-11.03)) ;
#121967=CARTESIAN_POINT('',(6.65857864376269,0.300000000000002,-11.03)) ;
#121968=CARTESIAN_POINT('',(6.65857864376269,-0.399999999999999,-11.03)) ;
#121969=CARTESIAN_POINT('',(2.4,0.3,-11.03)) ;
#121970=CARTESIAN_POINT('',(6.65857864376269,-0.300000000000001,-11.03)) ;
#121971=CARTESIAN_POINT('Origin',(0.6,-0.600000000000001,-11.83)) ;
#121972=CARTESIAN_POINT('',(6.65857864376269,0.300000000000002,-11.83)) ;
#121973=CARTESIAN_POINT('',(0.6,0.299999999999999,-11.83)) ;
#121974=CARTESIAN_POINT('',(6.65857864376269,-0.300000000000001,-11.83)) ;
#121975=CARTESIAN_POINT('',(6.65857864376269,-0.6,-11.83)) ;
#121976=CARTESIAN_POINT('',(0.6,-0.3,-11.83)) ;
#121977=CARTESIAN_POINT('Origin',(-0.4,-0.600000000000001,-14.84)) ;
#121978=CARTESIAN_POINT('',(-0.4,-0.600000000000001,-14.94)) ;
#121979=CARTESIAN_POINT('',(-0.4,-0.600000000000001,-15.54)) ;
#121980=CARTESIAN_POINT('',(-0.4,-0.600000000000001,-14.84)) ;
#121981=CARTESIAN_POINT('',(-0.4,-6.05857864376269,-15.54)) ;
#121982=CARTESIAN_POINT('',(-0.4,-0.600000000000001,-15.54)) ;
#121983=CARTESIAN_POINT('',(-0.4,-6.05857864376269,-14.94)) ;
#121984=CARTESIAN_POINT('',(-0.4,-6.05857864376269,-14.84)) ;
#121985=CARTESIAN_POINT('',(-0.4,-0.600000000000001,-14.94)) ;
#121986=CARTESIAN_POINT('Origin',(-0.4,-6.1,-14.84)) ;
#121987=CARTESIAN_POINT('',(-0.129289321881346,-6.37071067811866,-15.2985786437627)) ;
#121988=CARTESIAN_POINT('',(-0.129289321881346,-6.37071067811866,-15.1814213562373)) ;
#121989=CARTESIAN_POINT('',(-0.129289321881346,-6.37071067811866,-14.84)) ;
#121990=CARTESIAN_POINT('',(-0.370710678118655,-6.12928932188134,-14.94)) ;
#121991=CARTESIAN_POINT('',(-0.423570226039552,-6.07642977396045,-14.8871404520791)) ;
#121992=CARTESIAN_POINT('',(-0.370710678118655,-6.12928932188134,-15.54)) ;
#121993=CARTESIAN_POINT('',(-0.370710678118655,-6.12928932188134,-14.84)) ;
#121994=CARTESIAN_POINT('',(-0.156903559372884,-6.34309644062712,-15.3261928812542)) ;
#121995=CARTESIAN_POINT('Origin',(-0.1,-6.4,-14.84)) ;
#121996=CARTESIAN_POINT('',(0.0585786437626908,-6.4,-15.2985786437627)) ;
#121997=CARTESIAN_POINT('',(0.0585786437626908,-6.4,-15.1814213562373)) ;
#121998=CARTESIAN_POINT('',(0.0585786437626908,-6.4,-14.84)) ;
#121999=CARTESIAN_POINT('',(-0.0585786437626908,-6.4,-15.1814213562373)) ;
#122000=CARTESIAN_POINT('',(-0.1,-6.4,-15.1814213562373)) ;
#122001=CARTESIAN_POINT('',(-0.0585786437626908,-6.4,-15.2985786437627)) ;
#122002=CARTESIAN_POINT('',(-0.0585786437626908,-6.4,-14.84)) ;
#122003=CARTESIAN_POINT('',(-0.1,-6.4,-15.2985786437627)) ;
#122004=CARTESIAN_POINT('Origin',(0.1,-6.4,-14.84)) ;
#122005=CARTESIAN_POINT('',(0.370710678118655,-6.12928932188134,-15.54)) ;
#122006=CARTESIAN_POINT('',(0.370710678118655,-6.12928932188134,-14.94)) ;
#122007=CARTESIAN_POINT('',(0.370710678118655,-6.12928932188134,-14.84)) ;
#122008=CARTESIAN_POINT('',(0.129289321881346,-6.37071067811866,-15.1814213562373)) ;
#122009=CARTESIAN_POINT('',(0.223570226039553,-6.27642977396045,-15.0871404520791)) ;
#122010=CARTESIAN_POINT('',(0.129289321881346,-6.37071067811866,-15.2985786437627)) ;
#122011=CARTESIAN_POINT('',(0.129289321881346,-6.37071067811866,-14.84)) ;
#122012=CARTESIAN_POINT('',(-0.0430964406271151,-6.54309644062712,-15.1261928812542)) ;
#122013=CARTESIAN_POINT('Origin',(0.4,-6.1,-14.84)) ;
#122014=CARTESIAN_POINT('',(0.4,-6.05857864376269,-14.94)) ;
#122015=CARTESIAN_POINT('',(0.4,-6.05857864376269,-15.54)) ;
#122016=CARTESIAN_POINT('',(0.4,-6.05857864376269,-14.84)) ;
#122017=CARTESIAN_POINT('',(0.4,-0.6,-15.54)) ;
#122018=CARTESIAN_POINT('',(0.4,-6.1,-15.54)) ;
#122019=CARTESIAN_POINT('',(0.4,-0.6,-14.94)) ;
#122020=CARTESIAN_POINT('',(0.4,-0.6,-14.84)) ;
#122021=CARTESIAN_POINT('',(0.4,-6.05857864376269,-14.94)) ;
#122022=CARTESIAN_POINT('Origin',(0.6,-0.600000000000001,-14.84)) ;
#122023=CARTESIAN_POINT('',(0.3,-6.05857864376269,-14.84)) ;
#122024=CARTESIAN_POINT('',(0.3,-0.6,-14.84)) ;
#122025=CARTESIAN_POINT('',(0.3,-0.6,-14.84)) ;
#122026=CARTESIAN_POINT('Origin',(0.6,-0.6,-14.84)) ;
#122027=CARTESIAN_POINT('',(-0.3,-0.600000000000001,-14.84)) ;
#122028=CARTESIAN_POINT('Origin',(0.6,-0.600000000000001,-14.84)) ;
#122029=CARTESIAN_POINT('',(-0.300000000000001,-6.05857864376269,-14.84)) ;
#122030=CARTESIAN_POINT('',(-0.3,-0.600000000000001,-14.84)) ;
#122031=CARTESIAN_POINT('',(0.4,-6.05857864376269,-14.84)) ;
#122032=CARTESIAN_POINT('Origin',(0.6,-0.600000000000001,-15.64)) ;
#122033=CARTESIAN_POINT('',(-0.299999999999999,-6.05857864376269,-15.64)) ;
#122034=CARTESIAN_POINT('',(-0.3,-0.600000000000001,-15.64)) ;
#122035=CARTESIAN_POINT('',(-0.3,-0.600000000000001,-15.64)) ;
#122036=CARTESIAN_POINT('Origin',(0.6,-0.600000000000001,-15.64)) ;
#122037=CARTESIAN_POINT('',(0.3,-0.6,-15.64)) ;
#122038=CARTESIAN_POINT('Origin',(0.6,-0.6,-15.64)) ;
#122039=CARTESIAN_POINT('',(0.3,-6.05857864376269,-15.64)) ;
#122040=CARTESIAN_POINT('',(0.3,-0.600000000000001,-15.64)) ;
#122041=CARTESIAN_POINT('',(0.6,-6.05857864376269,-15.64)) ;
#122042=CARTESIAN_POINT('Origin',(0.6,-0.600000000000001,-14.84)) ;
#122043=CARTESIAN_POINT('Origin',(0.6,-0.600000000000001,-15.54)) ;
#122044=CARTESIAN_POINT('Origin',(0.6,-0.600000000000001,-14.94)) ;
#122045=CARTESIAN_POINT('Origin',(0.6,-0.6,-14.84)) ;
#122046=CARTESIAN_POINT('Origin',(0.6,-0.6,-15.54)) ;
#122047=CARTESIAN_POINT('Origin',(0.6,-0.6,-14.94)) ;
#122048=CARTESIAN_POINT('Origin',(7.,0.1,-14.84)) ;
#122049=CARTESIAN_POINT('',(6.72928932188135,0.370710678118655,-15.54)) ;
#122050=CARTESIAN_POINT('',(6.72928932188135,0.370710678118655,-14.94)) ;
#122051=CARTESIAN_POINT('',(6.72928932188135,0.370710678118655,-14.84)) ;
#122052=CARTESIAN_POINT('',(6.97071067811866,0.129289321881346,-15.1814213562373)) ;
#122053=CARTESIAN_POINT('',(6.87642977396045,0.223570226039552,-15.0871404520791)) ;
#122054=CARTESIAN_POINT('',(6.97071067811866,0.129289321881346,-15.2985786437627)) ;
#122055=CARTESIAN_POINT('',(6.97071067811866,0.129289321881346,-14.84)) ;
#122056=CARTESIAN_POINT('',(7.14309644062712,-0.0430964406271147,-15.1261928812542)) ;
#122057=CARTESIAN_POINT('Origin',(6.7,0.400000000000001,-14.84)) ;
#122058=CARTESIAN_POINT('',(6.65857864376269,0.400000000000001,-14.94)) ;
#122059=CARTESIAN_POINT('',(6.65857864376269,0.400000000000001,-15.54)) ;
#122060=CARTESIAN_POINT('',(6.65857864376269,0.400000000000001,-14.84)) ;
#122061=CARTESIAN_POINT('',(6.7,0.400000000000001,-15.54)) ;
#122062=CARTESIAN_POINT('',(6.65857864376269,0.400000000000001,-14.94)) ;
#122063=CARTESIAN_POINT('Origin',(0.6,-0.4,-14.84)) ;
#122064=CARTESIAN_POINT('',(6.65857864376269,-0.400000000000001,-15.54)) ;
#122065=CARTESIAN_POINT('',(0.6,-0.4,-15.54)) ;
#122066=CARTESIAN_POINT('',(6.65857864376269,-0.400000000000001,-14.94)) ;
#122067=CARTESIAN_POINT('',(6.65857864376269,-0.400000000000001,-14.84)) ;
#122068=CARTESIAN_POINT('',(2.4,-0.4,-14.94)) ;
#122069=CARTESIAN_POINT('Origin',(6.7,-0.400000000000001,-14.84)) ;
#122070=CARTESIAN_POINT('',(6.97071067811866,-0.129289321881346,-15.2985786437627)) ;
#122071=CARTESIAN_POINT('',(6.97071067811866,-0.129289321881346,-15.1814213562373)) ;
#122072=CARTESIAN_POINT('',(6.97071067811866,-0.129289321881346,-14.84)) ;
#122073=CARTESIAN_POINT('',(6.72928932188135,-0.370710678118655,-14.94)) ;
#122074=CARTESIAN_POINT('',(6.67642977396045,-0.423570226039552,-14.8871404520791)) ;
#122075=CARTESIAN_POINT('',(6.72928932188135,-0.370710678118655,-15.54)) ;
#122076=CARTESIAN_POINT('',(6.72928932188135,-0.370710678118655,-14.84)) ;
#122077=CARTESIAN_POINT('',(6.94309644062712,-0.156903559372885,-15.3261928812542)) ;
#122078=CARTESIAN_POINT('Origin',(7.,-0.1,-14.84)) ;
#122079=CARTESIAN_POINT('',(7.,-0.0585786437626909,-15.1814213562373)) ;
#122080=CARTESIAN_POINT('',(7.,-0.0585786437626909,-15.2985786437627)) ;
#122081=CARTESIAN_POINT('',(7.,-0.0585786437626909,-14.84)) ;
#122082=CARTESIAN_POINT('',(7.,0.0585786437626909,-15.2985786437627)) ;
#122083=CARTESIAN_POINT('',(7.,-0.1,-15.2985786437627)) ;
#122084=CARTESIAN_POINT('',(7.,0.0585786437626909,-15.1814213562373)) ;
#122085=CARTESIAN_POINT('',(7.,0.0585786437626909,-14.84)) ;
#122086=CARTESIAN_POINT('',(7.,-0.1,-15.1814213562373)) ;
#122087=CARTESIAN_POINT('Origin',(0.6,-0.600000000000001,-14.84)) ;
#122088=CARTESIAN_POINT('',(6.65857864376269,-0.300000000000001,-14.84)) ;
#122089=CARTESIAN_POINT('',(6.65857864376269,0.3,-14.84)) ;
#122090=CARTESIAN_POINT('',(6.65857864376269,-0.399999999999999,-14.84)) ;
#122091=CARTESIAN_POINT('',(2.4,0.3,-14.84)) ;
#122092=CARTESIAN_POINT('',(6.65857864376269,-0.300000000000001,-14.84)) ;
#122093=CARTESIAN_POINT('Origin',(0.6,-0.600000000000001,-15.64)) ;
#122094=CARTESIAN_POINT('',(6.65857864376269,0.300000000000003,-15.64)) ;
#122095=CARTESIAN_POINT('',(0.6,0.299999999999999,-15.64)) ;
#122096=CARTESIAN_POINT('',(6.65857864376269,-0.300000000000001,-15.64)) ;
#122097=CARTESIAN_POINT('',(6.65857864376269,-0.6,-15.64)) ;
#122098=CARTESIAN_POINT('',(0.6,-0.3,-15.64)) ;
#122099=CARTESIAN_POINT('Origin',(-0.4,-0.600000000000001,-18.65)) ;
#122100=CARTESIAN_POINT('',(-0.4,-0.600000000000001,-18.75)) ;
#122101=CARTESIAN_POINT('',(-0.4,-0.600000000000001,-19.35)) ;
#122102=CARTESIAN_POINT('',(-0.4,-0.600000000000001,-18.65)) ;
#122103=CARTESIAN_POINT('',(-0.4,-6.05857864376269,-19.35)) ;
#122104=CARTESIAN_POINT('',(-0.4,-0.600000000000001,-19.35)) ;
#122105=CARTESIAN_POINT('',(-0.4,-6.05857864376269,-18.75)) ;
#122106=CARTESIAN_POINT('',(-0.4,-6.05857864376269,-18.65)) ;
#122107=CARTESIAN_POINT('',(-0.4,-0.600000000000001,-18.75)) ;
#122108=CARTESIAN_POINT('Origin',(-0.4,-6.1,-18.65)) ;
#122109=CARTESIAN_POINT('',(-0.129289321881345,-6.37071067811866,-19.1085786437627)) ;
#122110=CARTESIAN_POINT('',(-0.129289321881346,-6.37071067811866,-18.9914213562373)) ;
#122111=CARTESIAN_POINT('',(-0.129289321881346,-6.37071067811866,-18.65)) ;
#122112=CARTESIAN_POINT('',(-0.370710678118655,-6.12928932188134,-18.75)) ;
#122113=CARTESIAN_POINT('',(-0.423570226039551,-6.07642977396045,-18.6971404520791)) ;
#122114=CARTESIAN_POINT('',(-0.370710678118655,-6.12928932188134,-19.35)) ;
#122115=CARTESIAN_POINT('',(-0.370710678118655,-6.12928932188134,-18.65)) ;
#122116=CARTESIAN_POINT('',(-0.156903559372884,-6.34309644062712,-19.1361928812542)) ;
#122117=CARTESIAN_POINT('Origin',(-0.1,-6.4,-18.65)) ;
#122118=CARTESIAN_POINT('',(0.0585786437626908,-6.4,-19.1085786437627)) ;
#122119=CARTESIAN_POINT('',(0.0585786437626908,-6.4,-18.9914213562373)) ;
#122120=CARTESIAN_POINT('',(0.0585786437626908,-6.4,-18.65)) ;
#122121=CARTESIAN_POINT('',(-0.0585786437626908,-6.4,-18.9914213562373)) ;
#122122=CARTESIAN_POINT('',(-0.1,-6.4,-18.9914213562373)) ;
#122123=CARTESIAN_POINT('',(-0.0585786437626908,-6.4,-19.1085786437627)) ;
#122124=CARTESIAN_POINT('',(-0.0585786437626908,-6.4,-18.65)) ;
#122125=CARTESIAN_POINT('',(-0.1,-6.4,-19.1085786437627)) ;
#122126=CARTESIAN_POINT('Origin',(0.1,-6.4,-18.65)) ;
#122127=CARTESIAN_POINT('',(0.370710678118654,-6.12928932188135,-19.35)) ;
#122128=CARTESIAN_POINT('',(0.370710678118655,-6.12928932188134,-18.75)) ;
#122129=CARTESIAN_POINT('',(0.370710678118655,-6.12928932188134,-18.65)) ;
#122130=CARTESIAN_POINT('',(0.129289321881346,-6.37071067811866,-18.9914213562373)) ;
#122131=CARTESIAN_POINT('',(0.223570226039551,-6.27642977396045,-18.8971404520791)) ;
#122132=CARTESIAN_POINT('',(0.129289321881346,-6.37071067811866,-19.1085786437627)) ;
#122133=CARTESIAN_POINT('',(0.129289321881346,-6.37071067811866,-18.65)) ;
#122134=CARTESIAN_POINT('',(-0.0430964406271139,-6.54309644062711,-18.9361928812542)) ;
#122135=CARTESIAN_POINT('Origin',(0.4,-6.1,-18.65)) ;
#122136=CARTESIAN_POINT('',(0.4,-6.05857864376269,-18.75)) ;
#122137=CARTESIAN_POINT('',(0.4,-6.05857864376269,-19.35)) ;
#122138=CARTESIAN_POINT('',(0.4,-6.05857864376269,-18.65)) ;
#122139=CARTESIAN_POINT('',(0.4,-0.6,-19.35)) ;
#122140=CARTESIAN_POINT('',(0.4,-6.1,-19.35)) ;
#122141=CARTESIAN_POINT('',(0.4,-0.6,-18.75)) ;
#122142=CARTESIAN_POINT('',(0.4,-0.6,-18.65)) ;
#122143=CARTESIAN_POINT('',(0.4,-6.05857864376269,-18.75)) ;
#122144=CARTESIAN_POINT('Origin',(0.6,-0.600000000000001,-18.65)) ;
#122145=CARTESIAN_POINT('',(0.3,-6.05857864376269,-18.65)) ;
#122146=CARTESIAN_POINT('',(0.3,-0.6,-18.65)) ;
#122147=CARTESIAN_POINT('',(0.3,-0.6,-18.65)) ;
#122148=CARTESIAN_POINT('Origin',(0.6,-0.6,-18.65)) ;
#122149=CARTESIAN_POINT('',(-0.3,-0.600000000000001,-18.65)) ;
#122150=CARTESIAN_POINT('Origin',(0.6,-0.600000000000001,-18.65)) ;
#122151=CARTESIAN_POINT('',(-0.299999999999994,-6.0585786437627,-18.65)) ;
#122152=CARTESIAN_POINT('',(-0.3,-0.600000000000001,-18.65)) ;
#122153=CARTESIAN_POINT('',(0.4,-6.0585786437627,-18.65)) ;
#122154=CARTESIAN_POINT('Origin',(0.6,-0.600000000000001,-19.45)) ;
#122155=CARTESIAN_POINT('',(-0.299999999999994,-6.0585786437627,-19.45)) ;
#122156=CARTESIAN_POINT('',(-0.3,-0.600000000000001,-19.45)) ;
#122157=CARTESIAN_POINT('',(-0.3,-0.600000000000001,-19.45)) ;
#122158=CARTESIAN_POINT('Origin',(0.6,-0.600000000000001,-19.45)) ;
#122159=CARTESIAN_POINT('',(0.3,-0.6,-19.45)) ;
#122160=CARTESIAN_POINT('Origin',(0.6,-0.6,-19.45)) ;
#122161=CARTESIAN_POINT('',(0.3,-6.05857864376269,-19.45)) ;
#122162=CARTESIAN_POINT('',(0.3,-0.600000000000001,-19.45)) ;
#122163=CARTESIAN_POINT('',(0.6,-6.05857864376269,-19.45)) ;
#122164=CARTESIAN_POINT('Origin',(0.6,-0.600000000000001,-18.65)) ;
#122165=CARTESIAN_POINT('Origin',(0.6,-0.600000000000001,-19.35)) ;
#122166=CARTESIAN_POINT('Origin',(0.6,-0.600000000000001,-18.75)) ;
#122167=CARTESIAN_POINT('Origin',(0.6,-0.6,-18.65)) ;
#122168=CARTESIAN_POINT('Origin',(0.6,-0.6,-19.35)) ;
#122169=CARTESIAN_POINT('Origin',(0.6,-0.6,-18.75)) ;
#122170=CARTESIAN_POINT('Origin',(7.,0.1,-18.65)) ;
#122171=CARTESIAN_POINT('',(6.72928932188135,0.370710678118656,-19.35)) ;
#122172=CARTESIAN_POINT('',(6.72928932188135,0.370710678118655,-18.75)) ;
#122173=CARTESIAN_POINT('',(6.72928932188135,0.370710678118655,-18.65)) ;
#122174=CARTESIAN_POINT('',(6.97071067811866,0.129289321881346,-18.9914213562373)) ;
#122175=CARTESIAN_POINT('',(6.87642977396045,0.22357022603955,-18.8971404520791)) ;
#122176=CARTESIAN_POINT('',(6.97071067811866,0.129289321881346,-19.1085786437627)) ;
#122177=CARTESIAN_POINT('',(6.97071067811866,0.129289321881346,-18.65)) ;
#122178=CARTESIAN_POINT('',(7.14309644062712,-0.0430964406271155,-18.9361928812542)) ;
#122179=CARTESIAN_POINT('Origin',(6.7,0.400000000000001,-18.65)) ;
#122180=CARTESIAN_POINT('',(6.65857864376269,0.400000000000001,-18.75)) ;
#122181=CARTESIAN_POINT('',(6.65857864376269,0.400000000000001,-19.35)) ;
#122182=CARTESIAN_POINT('',(6.65857864376269,0.400000000000001,-18.65)) ;
#122183=CARTESIAN_POINT('',(6.7,0.400000000000001,-19.35)) ;
#122184=CARTESIAN_POINT('',(6.65857864376269,0.400000000000001,-18.75)) ;
#122185=CARTESIAN_POINT('Origin',(0.6,-0.4,-18.65)) ;
#122186=CARTESIAN_POINT('',(6.65857864376269,-0.400000000000001,-19.35)) ;
#122187=CARTESIAN_POINT('',(0.6,-0.4,-19.35)) ;
#122188=CARTESIAN_POINT('',(6.65857864376269,-0.400000000000001,-18.75)) ;
#122189=CARTESIAN_POINT('',(6.65857864376269,-0.400000000000001,-18.65)) ;
#122190=CARTESIAN_POINT('',(2.4,-0.4,-18.75)) ;
#122191=CARTESIAN_POINT('Origin',(6.7,-0.400000000000001,-18.65)) ;
#122192=CARTESIAN_POINT('',(6.97071067811866,-0.129289321881345,-19.1085786437627)) ;
#122193=CARTESIAN_POINT('',(6.97071067811866,-0.129289321881346,-18.9914213562373)) ;
#122194=CARTESIAN_POINT('',(6.97071067811866,-0.129289321881346,-18.65)) ;
#122195=CARTESIAN_POINT('',(6.72928932188135,-0.370710678118655,-18.75)) ;
#122196=CARTESIAN_POINT('',(6.67642977396045,-0.423570226039551,-18.6971404520791)) ;
#122197=CARTESIAN_POINT('',(6.72928932188135,-0.370710678118655,-19.35)) ;
#122198=CARTESIAN_POINT('',(6.72928932188135,-0.370710678118655,-18.65)) ;
#122199=CARTESIAN_POINT('',(6.94309644062712,-0.156903559372885,-19.1361928812542)) ;
#122200=CARTESIAN_POINT('Origin',(7.,-0.1,-18.65)) ;
#122201=CARTESIAN_POINT('',(7.,-0.0585786437626909,-18.9914213562373)) ;
#122202=CARTESIAN_POINT('',(7.,-0.0585786437626909,-19.1085786437627)) ;
#122203=CARTESIAN_POINT('',(7.,-0.0585786437626909,-18.65)) ;
#122204=CARTESIAN_POINT('',(7.,0.0585786437626909,-19.1085786437627)) ;
#122205=CARTESIAN_POINT('',(7.,-0.1,-19.1085786437627)) ;
#122206=CARTESIAN_POINT('',(7.,0.0585786437626909,-18.9914213562373)) ;
#122207=CARTESIAN_POINT('',(7.,0.0585786437626909,-18.65)) ;
#122208=CARTESIAN_POINT('',(7.,-0.1,-18.9914213562373)) ;
#122209=CARTESIAN_POINT('Origin',(0.6,-0.600000000000001,-18.65)) ;
#122210=CARTESIAN_POINT('',(6.65857864376269,-0.300000000000001,-18.65)) ;
#122211=CARTESIAN_POINT('',(6.6585786437627,0.299999999999992,-18.65)) ;
#122212=CARTESIAN_POINT('',(6.6585786437627,-0.399999999999999,-18.65)) ;
#122213=CARTESIAN_POINT('',(2.4,0.3,-18.65)) ;
#122214=CARTESIAN_POINT('',(6.65857864376269,-0.300000000000001,-18.65)) ;
#122215=CARTESIAN_POINT('Origin',(0.6,-0.600000000000001,-19.45)) ;
#122216=CARTESIAN_POINT('',(6.65857864376269,0.299999999999998,-19.45)) ;
#122217=CARTESIAN_POINT('',(0.6,0.299999999999999,-19.45)) ;
#122218=CARTESIAN_POINT('',(6.65857864376269,-0.300000000000001,-19.45)) ;
#122219=CARTESIAN_POINT('',(6.65857864376269,-0.6,-19.45)) ;
#122220=CARTESIAN_POINT('',(0.6,-0.3,-19.45)) ;
#122221=CARTESIAN_POINT('Origin',(-0.4,-0.600000000000001,-22.46)) ;
#122222=CARTESIAN_POINT('',(-0.4,-0.600000000000001,-22.56)) ;
#122223=CARTESIAN_POINT('',(-0.4,-0.600000000000001,-23.16)) ;
#122224=CARTESIAN_POINT('',(-0.4,-0.600000000000001,-22.46)) ;
#122225=CARTESIAN_POINT('',(-0.4,-6.05857864376269,-23.16)) ;
#122226=CARTESIAN_POINT('',(-0.4,-0.600000000000001,-23.16)) ;
#122227=CARTESIAN_POINT('',(-0.4,-6.05857864376269,-22.56)) ;
#122228=CARTESIAN_POINT('',(-0.4,-6.05857864376269,-22.46)) ;
#122229=CARTESIAN_POINT('',(-0.4,-0.600000000000001,-22.56)) ;
#122230=CARTESIAN_POINT('Origin',(-0.4,-6.1,-22.46)) ;
#122231=CARTESIAN_POINT('',(-0.129289321881345,-6.37071067811866,-22.9185786437627)) ;
#122232=CARTESIAN_POINT('',(-0.129289321881346,-6.37071067811866,-22.8014213562373)) ;
#122233=CARTESIAN_POINT('',(-0.129289321881346,-6.37071067811866,-22.46)) ;
#122234=CARTESIAN_POINT('',(-0.370710678118655,-6.12928932188134,-22.56)) ;
#122235=CARTESIAN_POINT('',(-0.423570226039551,-6.07642977396045,-22.5071404520791)) ;
#122236=CARTESIAN_POINT('',(-0.370710678118655,-6.12928932188134,-23.16)) ;
#122237=CARTESIAN_POINT('',(-0.370710678118655,-6.12928932188134,-22.46)) ;
#122238=CARTESIAN_POINT('',(-0.156903559372884,-6.34309644062712,-22.9461928812542)) ;
#122239=CARTESIAN_POINT('Origin',(-0.1,-6.4,-22.46)) ;
#122240=CARTESIAN_POINT('',(0.0585786437626908,-6.4,-22.9185786437627)) ;
#122241=CARTESIAN_POINT('',(0.0585786437626908,-6.4,-22.8014213562373)) ;
#122242=CARTESIAN_POINT('',(0.0585786437626908,-6.4,-22.46)) ;
#122243=CARTESIAN_POINT('',(-0.0585786437626908,-6.4,-22.8014213562373)) ;
#122244=CARTESIAN_POINT('',(-0.1,-6.4,-22.8014213562373)) ;
#122245=CARTESIAN_POINT('',(-0.0585786437626908,-6.4,-22.9185786437627)) ;
#122246=CARTESIAN_POINT('',(-0.0585786437626908,-6.4,-22.46)) ;
#122247=CARTESIAN_POINT('',(-0.1,-6.4,-22.9185786437627)) ;
#122248=CARTESIAN_POINT('Origin',(0.1,-6.4,-22.46)) ;
#122249=CARTESIAN_POINT('',(0.370710678118654,-6.12928932188135,-23.16)) ;
#122250=CARTESIAN_POINT('',(0.370710678118655,-6.12928932188134,-22.56)) ;
#122251=CARTESIAN_POINT('',(0.370710678118655,-6.12928932188134,-22.46)) ;
#122252=CARTESIAN_POINT('',(0.129289321881346,-6.37071067811866,-22.8014213562373)) ;
#122253=CARTESIAN_POINT('',(0.223570226039551,-6.27642977396045,-22.7071404520791)) ;
#122254=CARTESIAN_POINT('',(0.129289321881346,-6.37071067811866,-22.9185786437627)) ;
#122255=CARTESIAN_POINT('',(0.129289321881346,-6.37071067811866,-22.46)) ;
#122256=CARTESIAN_POINT('',(-0.0430964406271139,-6.54309644062711,-22.7461928812542)) ;
#122257=CARTESIAN_POINT('Origin',(0.4,-6.1,-22.46)) ;
#122258=CARTESIAN_POINT('',(0.4,-6.05857864376269,-22.56)) ;
#122259=CARTESIAN_POINT('',(0.4,-6.05857864376269,-23.16)) ;
#122260=CARTESIAN_POINT('',(0.4,-6.05857864376269,-22.46)) ;
#122261=CARTESIAN_POINT('',(0.4,-0.6,-23.16)) ;
#122262=CARTESIAN_POINT('',(0.4,-6.1,-23.16)) ;
#122263=CARTESIAN_POINT('',(0.4,-0.6,-22.56)) ;
#122264=CARTESIAN_POINT('',(0.4,-0.6,-22.46)) ;
#122265=CARTESIAN_POINT('',(0.4,-6.05857864376269,-22.56)) ;
#122266=CARTESIAN_POINT('Origin',(0.6,-0.600000000000001,-22.46)) ;
#122267=CARTESIAN_POINT('',(0.3,-6.05857864376269,-22.46)) ;
#122268=CARTESIAN_POINT('',(0.3,-0.6,-22.46)) ;
#122269=CARTESIAN_POINT('',(0.3,-0.6,-22.46)) ;
#122270=CARTESIAN_POINT('Origin',(0.6,-0.6,-22.46)) ;
#122271=CARTESIAN_POINT('',(-0.3,-0.600000000000001,-22.46)) ;
#122272=CARTESIAN_POINT('Origin',(0.6,-0.600000000000001,-22.46)) ;
#122273=CARTESIAN_POINT('',(-0.299999999999994,-6.0585786437627,-22.46)) ;
#122274=CARTESIAN_POINT('',(-0.3,-0.600000000000001,-22.46)) ;
#122275=CARTESIAN_POINT('',(0.4,-6.0585786437627,-22.46)) ;
#122276=CARTESIAN_POINT('Origin',(0.6,-0.600000000000001,-23.26)) ;
#122277=CARTESIAN_POINT('',(-0.299999999999994,-6.0585786437627,-23.26)) ;
#122278=CARTESIAN_POINT('',(-0.3,-0.600000000000001,-23.26)) ;
#122279=CARTESIAN_POINT('',(-0.3,-0.600000000000001,-23.26)) ;
#122280=CARTESIAN_POINT('Origin',(0.6,-0.600000000000001,-23.26)) ;
#122281=CARTESIAN_POINT('',(0.3,-0.6,-23.26)) ;
#122282=CARTESIAN_POINT('Origin',(0.6,-0.6,-23.26)) ;
#122283=CARTESIAN_POINT('',(0.3,-6.05857864376269,-23.26)) ;
#122284=CARTESIAN_POINT('',(0.3,-0.600000000000001,-23.26)) ;
#122285=CARTESIAN_POINT('',(0.6,-6.05857864376269,-23.26)) ;
#122286=CARTESIAN_POINT('Origin',(0.6,-0.600000000000001,-22.46)) ;
#122287=CARTESIAN_POINT('Origin',(0.6,-0.600000000000001,-23.16)) ;
#122288=CARTESIAN_POINT('Origin',(0.6,-0.600000000000001,-22.56)) ;
#122289=CARTESIAN_POINT('Origin',(0.6,-0.6,-22.46)) ;
#122290=CARTESIAN_POINT('Origin',(0.6,-0.6,-23.16)) ;
#122291=CARTESIAN_POINT('Origin',(0.6,-0.6,-22.56)) ;
#122292=CARTESIAN_POINT('Origin',(7.,0.1,-22.46)) ;
#122293=CARTESIAN_POINT('',(6.72928932188135,0.370710678118656,-23.16)) ;
#122294=CARTESIAN_POINT('',(6.72928932188135,0.370710678118655,-22.56)) ;
#122295=CARTESIAN_POINT('',(6.72928932188135,0.370710678118655,-22.46)) ;
#122296=CARTESIAN_POINT('',(6.97071067811866,0.129289321881346,-22.8014213562373)) ;
#122297=CARTESIAN_POINT('',(6.87642977396045,0.22357022603955,-22.7071404520791)) ;
#122298=CARTESIAN_POINT('',(6.97071067811866,0.129289321881346,-22.9185786437627)) ;
#122299=CARTESIAN_POINT('',(6.97071067811866,0.129289321881346,-22.46)) ;
#122300=CARTESIAN_POINT('',(7.14309644062712,-0.0430964406271155,-22.7461928812542)) ;
#122301=CARTESIAN_POINT('Origin',(6.7,0.400000000000001,-22.46)) ;
#122302=CARTESIAN_POINT('',(6.65857864376269,0.400000000000001,-22.56)) ;
#122303=CARTESIAN_POINT('',(6.65857864376269,0.400000000000001,-23.16)) ;
#122304=CARTESIAN_POINT('',(6.65857864376269,0.400000000000001,-22.46)) ;
#122305=CARTESIAN_POINT('',(6.7,0.400000000000001,-23.16)) ;
#122306=CARTESIAN_POINT('',(6.65857864376269,0.400000000000001,-22.56)) ;
#122307=CARTESIAN_POINT('Origin',(0.6,-0.4,-22.46)) ;
#122308=CARTESIAN_POINT('',(6.65857864376269,-0.400000000000001,-23.16)) ;
#122309=CARTESIAN_POINT('',(0.6,-0.4,-23.16)) ;
#122310=CARTESIAN_POINT('',(6.65857864376269,-0.400000000000001,-22.56)) ;
#122311=CARTESIAN_POINT('',(6.65857864376269,-0.400000000000001,-22.46)) ;
#122312=CARTESIAN_POINT('',(2.4,-0.4,-22.56)) ;
#122313=CARTESIAN_POINT('Origin',(6.7,-0.400000000000001,-22.46)) ;
#122314=CARTESIAN_POINT('',(6.97071067811866,-0.129289321881345,-22.9185786437627)) ;
#122315=CARTESIAN_POINT('',(6.97071067811866,-0.129289321881346,-22.8014213562373)) ;
#122316=CARTESIAN_POINT('',(6.97071067811866,-0.129289321881346,-22.46)) ;
#122317=CARTESIAN_POINT('',(6.72928932188135,-0.370710678118655,-22.56)) ;
#122318=CARTESIAN_POINT('',(6.67642977396045,-0.423570226039551,-22.5071404520791)) ;
#122319=CARTESIAN_POINT('',(6.72928932188135,-0.370710678118655,-23.16)) ;
#122320=CARTESIAN_POINT('',(6.72928932188135,-0.370710678118655,-22.46)) ;
#122321=CARTESIAN_POINT('',(6.94309644062712,-0.156903559372885,-22.9461928812542)) ;
#122322=CARTESIAN_POINT('Origin',(7.,-0.1,-22.46)) ;
#122323=CARTESIAN_POINT('',(7.,-0.0585786437626909,-22.8014213562373)) ;
#122324=CARTESIAN_POINT('',(7.,-0.0585786437626909,-22.9185786437627)) ;
#122325=CARTESIAN_POINT('',(7.,-0.0585786437626909,-22.46)) ;
#122326=CARTESIAN_POINT('',(7.,0.0585786437626909,-22.9185786437627)) ;
#122327=CARTESIAN_POINT('',(7.,-0.1,-22.9185786437627)) ;
#122328=CARTESIAN_POINT('',(7.,0.0585786437626909,-22.8014213562373)) ;
#122329=CARTESIAN_POINT('',(7.,0.0585786437626909,-22.46)) ;
#122330=CARTESIAN_POINT('',(7.,-0.1,-22.8014213562373)) ;
#122331=CARTESIAN_POINT('Origin',(0.6,-0.600000000000001,-22.46)) ;
#122332=CARTESIAN_POINT('',(6.65857864376269,-0.300000000000001,-22.46)) ;
#122333=CARTESIAN_POINT('',(6.6585786437627,0.299999999999994,-22.46)) ;
#122334=CARTESIAN_POINT('',(6.6585786437627,-0.399999999999999,-22.46)) ;
#122335=CARTESIAN_POINT('',(2.4,0.3,-22.46)) ;
#122336=CARTESIAN_POINT('',(6.65857864376269,-0.300000000000001,-22.46)) ;
#122337=CARTESIAN_POINT('Origin',(0.6,-0.600000000000001,-23.26)) ;
#122338=CARTESIAN_POINT('',(6.65857864376269,0.299999999999998,-23.26)) ;
#122339=CARTESIAN_POINT('',(0.6,0.299999999999999,-23.26)) ;
#122340=CARTESIAN_POINT('',(6.65857864376269,-0.300000000000001,-23.26)) ;
#122341=CARTESIAN_POINT('',(6.65857864376269,-0.6,-23.26)) ;
#122342=CARTESIAN_POINT('',(0.6,-0.3,-23.26)) ;
#122343=CARTESIAN_POINT('Origin',(-0.4,-0.600000000000001,-26.27)) ;
#122344=CARTESIAN_POINT('',(-0.4,-0.600000000000001,-26.37)) ;
#122345=CARTESIAN_POINT('',(-0.4,-0.600000000000001,-26.97)) ;
#122346=CARTESIAN_POINT('',(-0.4,-0.600000000000001,-26.27)) ;
#122347=CARTESIAN_POINT('',(-0.4,-6.05857864376269,-26.97)) ;
#122348=CARTESIAN_POINT('',(-0.4,-0.600000000000001,-26.97)) ;
#122349=CARTESIAN_POINT('',(-0.4,-6.05857864376269,-26.37)) ;
#122350=CARTESIAN_POINT('',(-0.4,-6.05857864376269,-26.27)) ;
#122351=CARTESIAN_POINT('',(-0.4,-0.600000000000001,-26.37)) ;
#122352=CARTESIAN_POINT('Origin',(-0.4,-6.1,-26.27)) ;
#122353=CARTESIAN_POINT('',(-0.129289321881345,-6.37071067811866,-26.7285786437627)) ;
#122354=CARTESIAN_POINT('',(-0.129289321881346,-6.37071067811866,-26.6114213562373)) ;
#122355=CARTESIAN_POINT('',(-0.129289321881346,-6.37071067811866,-26.27)) ;
#122356=CARTESIAN_POINT('',(-0.370710678118655,-6.12928932188134,-26.37)) ;
#122357=CARTESIAN_POINT('',(-0.423570226039551,-6.07642977396045,-26.3171404520791)) ;
#122358=CARTESIAN_POINT('',(-0.370710678118655,-6.12928932188134,-26.97)) ;
#122359=CARTESIAN_POINT('',(-0.370710678118655,-6.12928932188134,-26.27)) ;
#122360=CARTESIAN_POINT('',(-0.156903559372884,-6.34309644062712,-26.7561928812542)) ;
#122361=CARTESIAN_POINT('Origin',(-0.1,-6.4,-26.27)) ;
#122362=CARTESIAN_POINT('',(0.0585786437626908,-6.4,-26.7285786437627)) ;
#122363=CARTESIAN_POINT('',(0.0585786437626908,-6.4,-26.6114213562373)) ;
#122364=CARTESIAN_POINT('',(0.0585786437626908,-6.4,-26.27)) ;
#122365=CARTESIAN_POINT('',(-0.0585786437626908,-6.4,-26.6114213562373)) ;
#122366=CARTESIAN_POINT('',(-0.1,-6.4,-26.6114213562373)) ;
#122367=CARTESIAN_POINT('',(-0.0585786437626908,-6.4,-26.7285786437627)) ;
#122368=CARTESIAN_POINT('',(-0.0585786437626908,-6.4,-26.27)) ;
#122369=CARTESIAN_POINT('',(-0.1,-6.4,-26.7285786437627)) ;
#122370=CARTESIAN_POINT('Origin',(0.1,-6.4,-26.27)) ;
#122371=CARTESIAN_POINT('',(0.370710678118654,-6.12928932188135,-26.97)) ;
#122372=CARTESIAN_POINT('',(0.370710678118655,-6.12928932188134,-26.37)) ;
#122373=CARTESIAN_POINT('',(0.370710678118655,-6.12928932188134,-26.27)) ;
#122374=CARTESIAN_POINT('',(0.129289321881346,-6.37071067811866,-26.6114213562373)) ;
#122375=CARTESIAN_POINT('',(0.223570226039551,-6.27642977396045,-26.5171404520791)) ;
#122376=CARTESIAN_POINT('',(0.129289321881346,-6.37071067811866,-26.7285786437627)) ;
#122377=CARTESIAN_POINT('',(0.129289321881346,-6.37071067811866,-26.27)) ;
#122378=CARTESIAN_POINT('',(-0.0430964406271139,-6.54309644062711,-26.5561928812542)) ;
#122379=CARTESIAN_POINT('Origin',(0.4,-6.1,-26.27)) ;
#122380=CARTESIAN_POINT('',(0.4,-6.05857864376269,-26.37)) ;
#122381=CARTESIAN_POINT('',(0.4,-6.05857864376269,-26.97)) ;
#122382=CARTESIAN_POINT('',(0.4,-6.05857864376269,-26.27)) ;
#122383=CARTESIAN_POINT('',(0.4,-0.6,-26.97)) ;
#122384=CARTESIAN_POINT('',(0.4,-6.1,-26.97)) ;
#122385=CARTESIAN_POINT('',(0.4,-0.6,-26.37)) ;
#122386=CARTESIAN_POINT('',(0.4,-0.6,-26.27)) ;
#122387=CARTESIAN_POINT('',(0.4,-6.05857864376269,-26.37)) ;
#122388=CARTESIAN_POINT('Origin',(0.6,-0.600000000000001,-26.27)) ;
#122389=CARTESIAN_POINT('',(0.3,-6.05857864376269,-26.27)) ;
#122390=CARTESIAN_POINT('',(0.3,-0.6,-26.27)) ;
#122391=CARTESIAN_POINT('',(0.3,-0.6,-26.27)) ;
#122392=CARTESIAN_POINT('Origin',(0.6,-0.6,-26.27)) ;
#122393=CARTESIAN_POINT('',(-0.3,-0.600000000000001,-26.27)) ;
#122394=CARTESIAN_POINT('Origin',(0.6,-0.600000000000001,-26.27)) ;
#122395=CARTESIAN_POINT('',(-0.299999999999994,-6.0585786437627,-26.27)) ;
#122396=CARTESIAN_POINT('',(-0.3,-0.600000000000001,-26.27)) ;
#122397=CARTESIAN_POINT('',(0.4,-6.0585786437627,-26.27)) ;
#122398=CARTESIAN_POINT('Origin',(0.6,-0.600000000000001,-27.07)) ;
#122399=CARTESIAN_POINT('',(-0.299999999999994,-6.0585786437627,-27.07)) ;
#122400=CARTESIAN_POINT('',(-0.3,-0.600000000000001,-27.07)) ;
#122401=CARTESIAN_POINT('',(-0.3,-0.600000000000001,-27.07)) ;
#122402=CARTESIAN_POINT('Origin',(0.6,-0.600000000000001,-27.07)) ;
#122403=CARTESIAN_POINT('',(0.3,-0.6,-27.07)) ;
#122404=CARTESIAN_POINT('Origin',(0.6,-0.6,-27.07)) ;
#122405=CARTESIAN_POINT('',(0.3,-6.05857864376269,-27.07)) ;
#122406=CARTESIAN_POINT('',(0.3,-0.600000000000001,-27.07)) ;
#122407=CARTESIAN_POINT('',(0.6,-6.05857864376269,-27.07)) ;
#122408=CARTESIAN_POINT('Origin',(0.6,-0.600000000000001,-26.27)) ;
#122409=CARTESIAN_POINT('Origin',(0.6,-0.600000000000001,-26.97)) ;
#122410=CARTESIAN_POINT('Origin',(0.6,-0.600000000000001,-26.37)) ;
#122411=CARTESIAN_POINT('Origin',(0.6,-0.6,-26.27)) ;
#122412=CARTESIAN_POINT('Origin',(0.6,-0.6,-26.97)) ;
#122413=CARTESIAN_POINT('Origin',(0.6,-0.6,-26.37)) ;
#122414=CARTESIAN_POINT('Origin',(7.,0.1,-26.27)) ;
#122415=CARTESIAN_POINT('',(6.72928932188135,0.370710678118656,-26.97)) ;
#122416=CARTESIAN_POINT('',(6.72928932188135,0.370710678118655,-26.37)) ;
#122417=CARTESIAN_POINT('',(6.72928932188135,0.370710678118655,-26.27)) ;
#122418=CARTESIAN_POINT('',(6.97071067811866,0.129289321881346,-26.6114213562373)) ;
#122419=CARTESIAN_POINT('',(6.87642977396045,0.22357022603955,-26.5171404520791)) ;
#122420=CARTESIAN_POINT('',(6.97071067811866,0.129289321881346,-26.7285786437627)) ;
#122421=CARTESIAN_POINT('',(6.97071067811866,0.129289321881346,-26.27)) ;
#122422=CARTESIAN_POINT('',(7.14309644062712,-0.0430964406271155,-26.5561928812542)) ;
#122423=CARTESIAN_POINT('Origin',(6.7,0.400000000000001,-26.27)) ;
#122424=CARTESIAN_POINT('',(6.65857864376269,0.400000000000001,-26.37)) ;
#122425=CARTESIAN_POINT('',(6.65857864376269,0.400000000000001,-26.97)) ;
#122426=CARTESIAN_POINT('',(6.65857864376269,0.400000000000001,-26.27)) ;
#122427=CARTESIAN_POINT('',(6.7,0.400000000000001,-26.97)) ;
#122428=CARTESIAN_POINT('',(6.65857864376269,0.400000000000001,-26.37)) ;
#122429=CARTESIAN_POINT('Origin',(0.6,-0.4,-26.27)) ;
#122430=CARTESIAN_POINT('',(6.65857864376269,-0.400000000000001,-26.97)) ;
#122431=CARTESIAN_POINT('',(0.6,-0.4,-26.97)) ;
#122432=CARTESIAN_POINT('',(6.65857864376269,-0.400000000000001,-26.37)) ;
#122433=CARTESIAN_POINT('',(6.65857864376269,-0.400000000000001,-26.27)) ;
#122434=CARTESIAN_POINT('',(2.4,-0.4,-26.37)) ;
#122435=CARTESIAN_POINT('Origin',(6.7,-0.400000000000001,-26.27)) ;
#122436=CARTESIAN_POINT('',(6.97071067811866,-0.129289321881345,-26.7285786437627)) ;
#122437=CARTESIAN_POINT('',(6.97071067811866,-0.129289321881346,-26.6114213562373)) ;
#122438=CARTESIAN_POINT('',(6.97071067811866,-0.129289321881346,-26.27)) ;
#122439=CARTESIAN_POINT('',(6.72928932188135,-0.370710678118655,-26.37)) ;
#122440=CARTESIAN_POINT('',(6.67642977396045,-0.423570226039551,-26.3171404520791)) ;
#122441=CARTESIAN_POINT('',(6.72928932188135,-0.370710678118655,-26.97)) ;
#122442=CARTESIAN_POINT('',(6.72928932188135,-0.370710678118655,-26.27)) ;
#122443=CARTESIAN_POINT('',(6.94309644062712,-0.156903559372885,-26.7561928812542)) ;
#122444=CARTESIAN_POINT('Origin',(7.,-0.1,-26.27)) ;
#122445=CARTESIAN_POINT('',(7.,-0.0585786437626909,-26.6114213562373)) ;
#122446=CARTESIAN_POINT('',(7.,-0.0585786437626909,-26.7285786437627)) ;
#122447=CARTESIAN_POINT('',(7.,-0.0585786437626909,-26.27)) ;
#122448=CARTESIAN_POINT('',(7.,0.0585786437626909,-26.7285786437627)) ;
#122449=CARTESIAN_POINT('',(7.,-0.1,-26.7285786437627)) ;
#122450=CARTESIAN_POINT('',(7.,0.0585786437626909,-26.6114213562373)) ;
#122451=CARTESIAN_POINT('',(7.,0.0585786437626909,-26.27)) ;
#122452=CARTESIAN_POINT('',(7.,-0.1,-26.6114213562373)) ;
#122453=CARTESIAN_POINT('Origin',(0.6,-0.600000000000001,-26.27)) ;
#122454=CARTESIAN_POINT('',(6.65857864376269,-0.300000000000001,-26.27)) ;
#122455=CARTESIAN_POINT('',(6.6585786437627,0.299999999999994,-26.27)) ;
#122456=CARTESIAN_POINT('',(6.6585786437627,-0.399999999999999,-26.27)) ;
#122457=CARTESIAN_POINT('',(2.4,0.3,-26.27)) ;
#122458=CARTESIAN_POINT('',(6.65857864376269,-0.300000000000001,-26.27)) ;
#122459=CARTESIAN_POINT('Origin',(0.6,-0.600000000000001,-27.07)) ;
#122460=CARTESIAN_POINT('',(6.65857864376269,0.299999999999998,-27.07)) ;
#122461=CARTESIAN_POINT('',(0.6,0.299999999999999,-27.07)) ;
#122462=CARTESIAN_POINT('',(6.65857864376269,-0.300000000000001,-27.07)) ;
#122463=CARTESIAN_POINT('',(6.65857864376269,-0.6,-27.07)) ;
#122464=CARTESIAN_POINT('',(0.6,-0.3,-27.07)) ;
#122465=CARTESIAN_POINT('Origin',(-0.4,-0.600000000000001,-30.08)) ;
#122466=CARTESIAN_POINT('',(-0.4,-0.600000000000001,-30.18)) ;
#122467=CARTESIAN_POINT('',(-0.4,-0.600000000000001,-30.78)) ;
#122468=CARTESIAN_POINT('',(-0.4,-0.600000000000001,-30.08)) ;
#122469=CARTESIAN_POINT('',(-0.4,-6.05857864376269,-30.78)) ;
#122470=CARTESIAN_POINT('',(-0.4,-0.600000000000001,-30.78)) ;
#122471=CARTESIAN_POINT('',(-0.4,-6.05857864376269,-30.18)) ;
#122472=CARTESIAN_POINT('',(-0.4,-6.05857864376269,-30.08)) ;
#122473=CARTESIAN_POINT('',(-0.4,-0.600000000000001,-30.18)) ;
#122474=CARTESIAN_POINT('Origin',(-0.4,-6.1,-30.08)) ;
#122475=CARTESIAN_POINT('',(-0.129289321881345,-6.37071067811866,-30.5385786437627)) ;
#122476=CARTESIAN_POINT('',(-0.129289321881346,-6.37071067811866,-30.4214213562373)) ;
#122477=CARTESIAN_POINT('',(-0.129289321881346,-6.37071067811866,-30.08)) ;
#122478=CARTESIAN_POINT('',(-0.370710678118655,-6.12928932188134,-30.18)) ;
#122479=CARTESIAN_POINT('',(-0.423570226039551,-6.07642977396045,-30.1271404520791)) ;
#122480=CARTESIAN_POINT('',(-0.370710678118655,-6.12928932188134,-30.78)) ;
#122481=CARTESIAN_POINT('',(-0.370710678118655,-6.12928932188134,-30.08)) ;
#122482=CARTESIAN_POINT('',(-0.156903559372884,-6.34309644062712,-30.5661928812542)) ;
#122483=CARTESIAN_POINT('Origin',(-0.1,-6.4,-30.08)) ;
#122484=CARTESIAN_POINT('',(0.0585786437626908,-6.4,-30.5385786437627)) ;
#122485=CARTESIAN_POINT('',(0.0585786437626908,-6.4,-30.4214213562373)) ;
#122486=CARTESIAN_POINT('',(0.0585786437626908,-6.4,-30.08)) ;
#122487=CARTESIAN_POINT('',(-0.0585786437626908,-6.4,-30.4214213562373)) ;
#122488=CARTESIAN_POINT('',(-0.1,-6.4,-30.4214213562373)) ;
#122489=CARTESIAN_POINT('',(-0.0585786437626908,-6.4,-30.5385786437627)) ;
#122490=CARTESIAN_POINT('',(-0.0585786437626908,-6.4,-30.08)) ;
#122491=CARTESIAN_POINT('',(-0.1,-6.4,-30.5385786437627)) ;
#122492=CARTESIAN_POINT('Origin',(0.1,-6.4,-30.08)) ;
#122493=CARTESIAN_POINT('',(0.370710678118654,-6.12928932188135,-30.78)) ;
#122494=CARTESIAN_POINT('',(0.370710678118655,-6.12928932188134,-30.18)) ;
#122495=CARTESIAN_POINT('',(0.370710678118655,-6.12928932188134,-30.08)) ;
#122496=CARTESIAN_POINT('',(0.129289321881346,-6.37071067811866,-30.4214213562373)) ;
#122497=CARTESIAN_POINT('',(0.223570226039551,-6.27642977396045,-30.3271404520791)) ;
#122498=CARTESIAN_POINT('',(0.129289321881346,-6.37071067811866,-30.5385786437627)) ;
#122499=CARTESIAN_POINT('',(0.129289321881346,-6.37071067811866,-30.08)) ;
#122500=CARTESIAN_POINT('',(-0.0430964406271139,-6.54309644062711,-30.3661928812542)) ;
#122501=CARTESIAN_POINT('Origin',(0.4,-6.1,-30.08)) ;
#122502=CARTESIAN_POINT('',(0.4,-6.05857864376269,-30.18)) ;
#122503=CARTESIAN_POINT('',(0.4,-6.05857864376269,-30.78)) ;
#122504=CARTESIAN_POINT('',(0.4,-6.05857864376269,-30.08)) ;
#122505=CARTESIAN_POINT('',(0.4,-0.6,-30.78)) ;
#122506=CARTESIAN_POINT('',(0.4,-6.1,-30.78)) ;
#122507=CARTESIAN_POINT('',(0.4,-0.6,-30.18)) ;
#122508=CARTESIAN_POINT('',(0.4,-0.6,-30.08)) ;
#122509=CARTESIAN_POINT('',(0.4,-6.05857864376269,-30.18)) ;
#122510=CARTESIAN_POINT('Origin',(0.6,-0.600000000000001,-30.08)) ;
#122511=CARTESIAN_POINT('',(0.3,-6.05857864376269,-30.08)) ;
#122512=CARTESIAN_POINT('',(0.3,-0.6,-30.08)) ;
#122513=CARTESIAN_POINT('',(0.3,-0.6,-30.08)) ;
#122514=CARTESIAN_POINT('Origin',(0.6,-0.6,-30.08)) ;
#122515=CARTESIAN_POINT('',(-0.3,-0.600000000000001,-30.08)) ;
#122516=CARTESIAN_POINT('Origin',(0.6,-0.600000000000001,-30.08)) ;
#122517=CARTESIAN_POINT('',(-0.299999999999994,-6.0585786437627,-30.08)) ;
#122518=CARTESIAN_POINT('',(-0.3,-0.600000000000001,-30.08)) ;
#122519=CARTESIAN_POINT('',(0.4,-6.0585786437627,-30.08)) ;
#122520=CARTESIAN_POINT('Origin',(0.6,-0.600000000000001,-30.88)) ;
#122521=CARTESIAN_POINT('',(-0.299999999999994,-6.0585786437627,-30.88)) ;
#122522=CARTESIAN_POINT('',(-0.3,-0.600000000000001,-30.88)) ;
#122523=CARTESIAN_POINT('',(-0.3,-0.600000000000001,-30.88)) ;
#122524=CARTESIAN_POINT('Origin',(0.6,-0.600000000000001,-30.88)) ;
#122525=CARTESIAN_POINT('',(0.3,-0.6,-30.88)) ;
#122526=CARTESIAN_POINT('Origin',(0.6,-0.6,-30.88)) ;
#122527=CARTESIAN_POINT('',(0.3,-6.05857864376269,-30.88)) ;
#122528=CARTESIAN_POINT('',(0.3,-0.600000000000001,-30.88)) ;
#122529=CARTESIAN_POINT('',(0.6,-6.05857864376269,-30.88)) ;
#122530=CARTESIAN_POINT('Origin',(0.6,-0.600000000000001,-30.08)) ;
#122531=CARTESIAN_POINT('Origin',(0.6,-0.600000000000001,-30.78)) ;
#122532=CARTESIAN_POINT('Origin',(0.6,-0.600000000000001,-30.18)) ;
#122533=CARTESIAN_POINT('Origin',(0.6,-0.6,-30.08)) ;
#122534=CARTESIAN_POINT('Origin',(0.6,-0.6,-30.78)) ;
#122535=CARTESIAN_POINT('Origin',(0.6,-0.6,-30.18)) ;
#122536=CARTESIAN_POINT('Origin',(7.,0.1,-30.08)) ;
#122537=CARTESIAN_POINT('',(6.72928932188135,0.370710678118656,-30.78)) ;
#122538=CARTESIAN_POINT('',(6.72928932188135,0.370710678118655,-30.18)) ;
#122539=CARTESIAN_POINT('',(6.72928932188135,0.370710678118655,-30.08)) ;
#122540=CARTESIAN_POINT('',(6.97071067811866,0.129289321881346,-30.4214213562373)) ;
#122541=CARTESIAN_POINT('',(6.87642977396045,0.22357022603955,-30.3271404520791)) ;
#122542=CARTESIAN_POINT('',(6.97071067811866,0.129289321881346,-30.5385786437627)) ;
#122543=CARTESIAN_POINT('',(6.97071067811866,0.129289321881346,-30.08)) ;
#122544=CARTESIAN_POINT('',(7.14309644062712,-0.0430964406271155,-30.3661928812542)) ;
#122545=CARTESIAN_POINT('Origin',(6.7,0.400000000000001,-30.08)) ;
#122546=CARTESIAN_POINT('',(6.65857864376269,0.400000000000001,-30.18)) ;
#122547=CARTESIAN_POINT('',(6.65857864376269,0.400000000000001,-30.78)) ;
#122548=CARTESIAN_POINT('',(6.65857864376269,0.400000000000001,-30.08)) ;
#122549=CARTESIAN_POINT('',(6.7,0.400000000000001,-30.78)) ;
#122550=CARTESIAN_POINT('',(6.65857864376269,0.400000000000001,-30.18)) ;
#122551=CARTESIAN_POINT('Origin',(0.6,-0.4,-30.08)) ;
#122552=CARTESIAN_POINT('',(6.65857864376269,-0.400000000000001,-30.78)) ;
#122553=CARTESIAN_POINT('',(0.6,-0.4,-30.78)) ;
#122554=CARTESIAN_POINT('',(6.65857864376269,-0.400000000000001,-30.18)) ;
#122555=CARTESIAN_POINT('',(6.65857864376269,-0.400000000000001,-30.08)) ;
#122556=CARTESIAN_POINT('',(2.4,-0.4,-30.18)) ;
#122557=CARTESIAN_POINT('Origin',(6.7,-0.400000000000001,-30.08)) ;
#122558=CARTESIAN_POINT('',(6.97071067811866,-0.129289321881345,-30.5385786437627)) ;
#122559=CARTESIAN_POINT('',(6.97071067811866,-0.129289321881346,-30.4214213562373)) ;
#122560=CARTESIAN_POINT('',(6.97071067811866,-0.129289321881346,-30.08)) ;
#122561=CARTESIAN_POINT('',(6.72928932188135,-0.370710678118655,-30.18)) ;
#122562=CARTESIAN_POINT('',(6.67642977396045,-0.423570226039551,-30.1271404520791)) ;
#122563=CARTESIAN_POINT('',(6.72928932188135,-0.370710678118655,-30.78)) ;
#122564=CARTESIAN_POINT('',(6.72928932188135,-0.370710678118655,-30.08)) ;
#122565=CARTESIAN_POINT('',(6.94309644062712,-0.156903559372885,-30.5661928812542)) ;
#122566=CARTESIAN_POINT('Origin',(7.,-0.1,-30.08)) ;
#122567=CARTESIAN_POINT('',(7.,-0.0585786437626909,-30.4214213562373)) ;
#122568=CARTESIAN_POINT('',(7.,-0.0585786437626909,-30.5385786437627)) ;
#122569=CARTESIAN_POINT('',(7.,-0.0585786437626909,-30.08)) ;
#122570=CARTESIAN_POINT('',(7.,0.0585786437626909,-30.5385786437627)) ;
#122571=CARTESIAN_POINT('',(7.,-0.1,-30.5385786437627)) ;
#122572=CARTESIAN_POINT('',(7.,0.0585786437626909,-30.4214213562373)) ;
#122573=CARTESIAN_POINT('',(7.,0.0585786437626909,-30.08)) ;
#122574=CARTESIAN_POINT('',(7.,-0.1,-30.4214213562373)) ;
#122575=CARTESIAN_POINT('Origin',(0.6,-0.600000000000001,-30.08)) ;
#122576=CARTESIAN_POINT('',(6.65857864376269,-0.300000000000001,-30.08)) ;
#122577=CARTESIAN_POINT('',(6.6585786437627,0.299999999999994,-30.08)) ;
#122578=CARTESIAN_POINT('',(6.6585786437627,-0.399999999999999,-30.08)) ;
#122579=CARTESIAN_POINT('',(2.4,0.3,-30.08)) ;
#122580=CARTESIAN_POINT('',(6.65857864376269,-0.300000000000001,-30.08)) ;
#122581=CARTESIAN_POINT('Origin',(0.6,-0.600000000000001,-30.88)) ;
#122582=CARTESIAN_POINT('',(6.65857864376269,0.299999999999998,-30.88)) ;
#122583=CARTESIAN_POINT('',(0.6,0.299999999999999,-30.88)) ;
#122584=CARTESIAN_POINT('',(6.65857864376269,-0.300000000000001,-30.88)) ;
#122585=CARTESIAN_POINT('',(6.65857864376269,-0.6,-30.88)) ;
#122586=CARTESIAN_POINT('',(0.6,-0.3,-30.88)) ;
#122587=CARTESIAN_POINT('Origin',(-0.4,-0.600000000000001,-33.89)) ;
#122588=CARTESIAN_POINT('',(-0.4,-0.600000000000001,-33.99)) ;
#122589=CARTESIAN_POINT('',(-0.4,-0.600000000000001,-34.59)) ;
#122590=CARTESIAN_POINT('',(-0.4,-0.600000000000001,-33.89)) ;
#122591=CARTESIAN_POINT('',(-0.4,-6.05857864376269,-34.59)) ;
#122592=CARTESIAN_POINT('',(-0.4,-0.600000000000001,-34.59)) ;
#122593=CARTESIAN_POINT('',(-0.4,-6.05857864376269,-33.99)) ;
#122594=CARTESIAN_POINT('',(-0.4,-6.05857864376269,-33.89)) ;
#122595=CARTESIAN_POINT('',(-0.4,-0.600000000000001,-33.99)) ;
#122596=CARTESIAN_POINT('Origin',(-0.4,-6.1,-33.89)) ;
#122597=CARTESIAN_POINT('',(-0.129289321881345,-6.37071067811866,-34.3485786437627)) ;
#122598=CARTESIAN_POINT('',(-0.129289321881346,-6.37071067811866,-34.2314213562373)) ;
#122599=CARTESIAN_POINT('',(-0.129289321881346,-6.37071067811866,-33.89)) ;
#122600=CARTESIAN_POINT('',(-0.370710678118655,-6.12928932188134,-33.99)) ;
#122601=CARTESIAN_POINT('',(-0.423570226039552,-6.07642977396045,-33.9371404520791)) ;
#122602=CARTESIAN_POINT('',(-0.370710678118655,-6.12928932188134,-34.59)) ;
#122603=CARTESIAN_POINT('',(-0.370710678118655,-6.12928932188134,-33.89)) ;
#122604=CARTESIAN_POINT('',(-0.156903559372882,-6.34309644062712,-34.3761928812542)) ;
#122605=CARTESIAN_POINT('Origin',(-0.1,-6.4,-33.89)) ;
#122606=CARTESIAN_POINT('',(0.0585786437626908,-6.4,-34.3485786437627)) ;
#122607=CARTESIAN_POINT('',(0.0585786437626908,-6.4,-34.2314213562373)) ;
#122608=CARTESIAN_POINT('',(0.0585786437626908,-6.4,-33.89)) ;
#122609=CARTESIAN_POINT('',(-0.0585786437626908,-6.4,-34.2314213562373)) ;
#122610=CARTESIAN_POINT('',(-0.1,-6.4,-34.2314213562373)) ;
#122611=CARTESIAN_POINT('',(-0.0585786437626908,-6.4,-34.3485786437627)) ;
#122612=CARTESIAN_POINT('',(-0.0585786437626908,-6.4,-33.89)) ;
#122613=CARTESIAN_POINT('',(-0.1,-6.4,-34.3485786437627)) ;
#122614=CARTESIAN_POINT('Origin',(0.1,-6.4,-33.89)) ;
#122615=CARTESIAN_POINT('',(0.370710678118654,-6.12928932188135,-34.59)) ;
#122616=CARTESIAN_POINT('',(0.370710678118655,-6.12928932188134,-33.99)) ;
#122617=CARTESIAN_POINT('',(0.370710678118655,-6.12928932188134,-33.89)) ;
#122618=CARTESIAN_POINT('',(0.129289321881346,-6.37071067811866,-34.2314213562373)) ;
#122619=CARTESIAN_POINT('',(0.223570226039555,-6.27642977396044,-34.1371404520791)) ;
#122620=CARTESIAN_POINT('',(0.129289321881346,-6.37071067811866,-34.3485786437627)) ;
#122621=CARTESIAN_POINT('',(0.129289321881346,-6.37071067811866,-33.89)) ;
#122622=CARTESIAN_POINT('',(-0.0430964406271177,-6.54309644062712,-34.1761928812542)) ;
#122623=CARTESIAN_POINT('Origin',(0.4,-6.1,-33.89)) ;
#122624=CARTESIAN_POINT('',(0.4,-6.05857864376269,-33.99)) ;
#122625=CARTESIAN_POINT('',(0.4,-6.05857864376269,-34.59)) ;
#122626=CARTESIAN_POINT('',(0.4,-6.05857864376269,-33.89)) ;
#122627=CARTESIAN_POINT('',(0.4,-0.6,-34.59)) ;
#122628=CARTESIAN_POINT('',(0.4,-6.1,-34.59)) ;
#122629=CARTESIAN_POINT('',(0.4,-0.6,-33.99)) ;
#122630=CARTESIAN_POINT('',(0.4,-0.6,-33.89)) ;
#122631=CARTESIAN_POINT('',(0.4,-6.05857864376269,-33.99)) ;
#122632=CARTESIAN_POINT('Origin',(0.6,-0.600000000000001,-33.89)) ;
#122633=CARTESIAN_POINT('',(0.3,-6.05857864376269,-33.89)) ;
#122634=CARTESIAN_POINT('',(0.3,-0.6,-33.89)) ;
#122635=CARTESIAN_POINT('',(0.3,-0.6,-33.89)) ;
#122636=CARTESIAN_POINT('Origin',(0.6,-0.6,-33.89)) ;
#122637=CARTESIAN_POINT('',(-0.3,-0.600000000000001,-33.89)) ;
#122638=CARTESIAN_POINT('Origin',(0.6,-0.600000000000001,-33.89)) ;
#122639=CARTESIAN_POINT('',(-0.300000000000006,-6.05857864376268,-33.89)) ;
#122640=CARTESIAN_POINT('',(-0.3,-0.600000000000001,-33.89)) ;
#122641=CARTESIAN_POINT('',(0.4,-6.05857864376269,-33.89)) ;
#122642=CARTESIAN_POINT('Origin',(0.6,-0.600000000000001,-34.69)) ;
#122643=CARTESIAN_POINT('',(-0.299999999999998,-6.05857864376269,-34.69)) ;
#122644=CARTESIAN_POINT('',(-0.3,-0.600000000000001,-34.69)) ;
#122645=CARTESIAN_POINT('',(-0.3,-0.600000000000001,-34.69)) ;
#122646=CARTESIAN_POINT('Origin',(0.6,-0.600000000000001,-34.69)) ;
#122647=CARTESIAN_POINT('',(0.3,-0.6,-34.69)) ;
#122648=CARTESIAN_POINT('Origin',(0.6,-0.6,-34.69)) ;
#122649=CARTESIAN_POINT('',(0.3,-6.05857864376269,-34.69)) ;
#122650=CARTESIAN_POINT('',(0.3,-0.600000000000001,-34.69)) ;
#122651=CARTESIAN_POINT('',(0.6,-6.05857864376269,-34.69)) ;
#122652=CARTESIAN_POINT('Origin',(0.6,-0.600000000000001,-33.89)) ;
#122653=CARTESIAN_POINT('Origin',(0.6,-0.600000000000001,-34.59)) ;
#122654=CARTESIAN_POINT('Origin',(0.6,-0.600000000000001,-33.99)) ;
#122655=CARTESIAN_POINT('Origin',(0.6,-0.6,-33.89)) ;
#122656=CARTESIAN_POINT('Origin',(0.6,-0.6,-34.59)) ;
#122657=CARTESIAN_POINT('Origin',(0.6,-0.6,-33.99)) ;
#122658=CARTESIAN_POINT('Origin',(7.,0.1,-33.89)) ;
#122659=CARTESIAN_POINT('',(6.72928932188135,0.370710678118655,-34.59)) ;
#122660=CARTESIAN_POINT('',(6.72928932188135,0.370710678118655,-33.99)) ;
#122661=CARTESIAN_POINT('',(6.72928932188135,0.370710678118655,-33.89)) ;
#122662=CARTESIAN_POINT('',(6.97071067811866,0.129289321881346,-34.2314213562373)) ;
#122663=CARTESIAN_POINT('',(6.87642977396044,0.223570226039555,-34.1371404520791)) ;
#122664=CARTESIAN_POINT('',(6.97071067811866,0.129289321881346,-34.3485786437627)) ;
#122665=CARTESIAN_POINT('',(6.97071067811866,0.129289321881346,-33.89)) ;
#122666=CARTESIAN_POINT('',(7.14309644062712,-0.0430964406271179,-34.1761928812542)) ;
#122667=CARTESIAN_POINT('Origin',(6.7,0.400000000000001,-33.89)) ;
#122668=CARTESIAN_POINT('',(6.65857864376269,0.400000000000001,-33.99)) ;
#122669=CARTESIAN_POINT('',(6.65857864376269,0.400000000000001,-34.59)) ;
#122670=CARTESIAN_POINT('',(6.65857864376269,0.400000000000001,-33.89)) ;
#122671=CARTESIAN_POINT('',(6.7,0.400000000000001,-34.59)) ;
#122672=CARTESIAN_POINT('',(6.65857864376269,0.400000000000001,-33.99)) ;
#122673=CARTESIAN_POINT('Origin',(0.6,-0.4,-33.89)) ;
#122674=CARTESIAN_POINT('',(6.65857864376269,-0.400000000000001,-34.59)) ;
#122675=CARTESIAN_POINT('',(0.6,-0.4,-34.59)) ;
#122676=CARTESIAN_POINT('',(6.65857864376269,-0.400000000000001,-33.99)) ;
#122677=CARTESIAN_POINT('',(6.65857864376269,-0.400000000000001,-33.89)) ;
#122678=CARTESIAN_POINT('',(2.4,-0.4,-33.99)) ;
#122679=CARTESIAN_POINT('Origin',(6.7,-0.400000000000001,-33.89)) ;
#122680=CARTESIAN_POINT('',(6.97071067811866,-0.129289321881345,-34.3485786437627)) ;
#122681=CARTESIAN_POINT('',(6.97071067811866,-0.129289321881346,-34.2314213562373)) ;
#122682=CARTESIAN_POINT('',(6.97071067811866,-0.129289321881346,-33.89)) ;
#122683=CARTESIAN_POINT('',(6.72928932188135,-0.370710678118655,-33.99)) ;
#122684=CARTESIAN_POINT('',(6.67642977396045,-0.423570226039555,-33.9371404520791)) ;
#122685=CARTESIAN_POINT('',(6.72928932188135,-0.370710678118655,-34.59)) ;
#122686=CARTESIAN_POINT('',(6.72928932188135,-0.370710678118655,-33.89)) ;
#122687=CARTESIAN_POINT('',(6.94309644062712,-0.156903559372885,-34.3761928812542)) ;
#122688=CARTESIAN_POINT('Origin',(7.,-0.1,-33.89)) ;
#122689=CARTESIAN_POINT('',(7.,-0.0585786437626909,-34.2314213562373)) ;
#122690=CARTESIAN_POINT('',(7.,-0.0585786437626909,-34.3485786437627)) ;
#122691=CARTESIAN_POINT('',(7.,-0.0585786437626909,-33.89)) ;
#122692=CARTESIAN_POINT('',(7.,0.0585786437626909,-34.3485786437627)) ;
#122693=CARTESIAN_POINT('',(7.,-0.1,-34.3485786437627)) ;
#122694=CARTESIAN_POINT('',(7.,0.0585786437626909,-34.2314213562373)) ;
#122695=CARTESIAN_POINT('',(7.,0.0585786437626909,-33.89)) ;
#122696=CARTESIAN_POINT('',(7.,-0.1,-34.2314213562373)) ;
#122697=CARTESIAN_POINT('Origin',(0.6,-0.600000000000001,-33.89)) ;
#122698=CARTESIAN_POINT('',(6.65857864376269,-0.300000000000001,-33.89)) ;
#122699=CARTESIAN_POINT('',(6.65857864376269,0.300000000000007,-33.89)) ;
#122700=CARTESIAN_POINT('',(6.65857864376269,-0.399999999999999,-33.89)) ;
#122701=CARTESIAN_POINT('',(2.4,0.3,-33.89)) ;
#122702=CARTESIAN_POINT('',(6.65857864376269,-0.300000000000001,-33.89)) ;
#122703=CARTESIAN_POINT('Origin',(0.6,-0.600000000000001,-34.69)) ;
#122704=CARTESIAN_POINT('',(6.65857864376269,0.3,-34.69)) ;
#122705=CARTESIAN_POINT('',(0.6,0.299999999999999,-34.69)) ;
#122706=CARTESIAN_POINT('',(6.65857864376269,-0.300000000000001,-34.69)) ;
#122707=CARTESIAN_POINT('',(6.6585786437627,-0.6,-34.69)) ;
#122708=CARTESIAN_POINT('',(0.6,-0.3,-34.69)) ;
#122709=CARTESIAN_POINT('Origin',(0.4,-6.4,-34.39)) ;
#122710=CARTESIAN_POINT('',(-0.0585786437626895,-6.37071067811866,-34.4192893218813)) ;
#122711=CARTESIAN_POINT('',(-0.299999999999997,-6.12928932188135,-34.6607106781186)) ;
#122712=CARTESIAN_POINT('',(0.113807118745769,-6.54309644062712,-34.2469035593729)) ;
#122713=CARTESIAN_POINT('',(0.299999999999999,-6.12928932188134,-34.6607106781187)) ;
#122714=CARTESIAN_POINT('',(0.4,-6.12928932188135,-34.6607106781186)) ;
#122715=CARTESIAN_POINT('',(0.0585786437626844,-6.37071067811866,-34.4192893218813)) ;
#122716=CARTESIAN_POINT('',(0.152859547920894,-6.27642977396045,-34.5135702260395)) ;
#122717=CARTESIAN_POINT('',(0.4,-6.37071067811866,-34.4192893218813)) ;
#122718=CARTESIAN_POINT('Origin',(0.4,-6.1,-33.89)) ;
#122719=CARTESIAN_POINT('',(0.058578643762689,-6.37071067811866,-34.1607106781187)) ;
#122720=CARTESIAN_POINT('',(0.300000000000011,-6.12928932188133,-33.9192893218813)) ;
#122721=CARTESIAN_POINT('',(0.352859547920897,-6.07642977396045,-33.8664297739605)) ;
#122722=CARTESIAN_POINT('',(-0.300000000000007,-6.12928932188133,-33.9192893218813)) ;
#122723=CARTESIAN_POINT('',(0.4,-6.12928932188134,-33.9192893218814)) ;
#122724=CARTESIAN_POINT('',(-0.0585786437626846,-6.37071067811866,-34.1607106781187)) ;
#122725=CARTESIAN_POINT('',(-0.0861928812542284,-6.34309644062711,-34.1330964406271)) ;
#122726=CARTESIAN_POINT('',(0.4,-6.37071067811866,-34.1607106781187)) ;
#122727=CARTESIAN_POINT('Origin',(0.4,-6.4,-30.58)) ;
#122728=CARTESIAN_POINT('',(-0.0585786437626899,-6.37071067811865,-30.6092893218813)) ;
#122729=CARTESIAN_POINT('',(-0.299999999999994,-6.12928932188135,-30.8507106781187)) ;
#122730=CARTESIAN_POINT('',(0.11380711874577,-6.54309644062711,-30.4369035593729)) ;
#122731=CARTESIAN_POINT('',(0.299999999999999,-6.12928932188135,-30.8507106781187)) ;
#122732=CARTESIAN_POINT('',(0.4,-6.12928932188134,-30.8507106781187)) ;
#122733=CARTESIAN_POINT('',(0.058578643762692,-6.37071067811865,-30.6092893218813)) ;
#122734=CARTESIAN_POINT('',(0.152859547920897,-6.27642977396045,-30.7035702260396)) ;
#122735=CARTESIAN_POINT('',(0.4,-6.37071067811865,-30.6092893218813)) ;
#122736=CARTESIAN_POINT('Origin',(0.4,-6.1,-30.08)) ;
#122737=CARTESIAN_POINT('',(0.0585786437626916,-6.37071067811865,-30.3507106781187)) ;
#122738=CARTESIAN_POINT('',(0.299999999999992,-6.12928932188135,-30.1092893218814)) ;
#122739=CARTESIAN_POINT('',(0.352859547920897,-6.07642977396045,-30.0564297739604)) ;
#122740=CARTESIAN_POINT('',(-0.299999999999994,-6.12928932188135,-30.1092893218814)) ;
#122741=CARTESIAN_POINT('',(0.4,-6.12928932188135,-30.1092893218813)) ;
#122742=CARTESIAN_POINT('',(-0.0585786437626909,-6.37071067811865,-30.3507106781187)) ;
#122743=CARTESIAN_POINT('',(-0.0861928812542305,-6.34309644062712,-30.3230964406271)) ;
#122744=CARTESIAN_POINT('',(0.4,-6.37071067811865,-30.3507106781187)) ;
#122745=CARTESIAN_POINT('Origin',(0.4,-6.4,-26.77)) ;
#122746=CARTESIAN_POINT('',(-0.0585786437626899,-6.37071067811865,-26.7992893218813)) ;
#122747=CARTESIAN_POINT('',(-0.299999999999994,-6.12928932188135,-27.0407106781187)) ;
#122748=CARTESIAN_POINT('',(0.11380711874577,-6.54309644062711,-26.6269035593729)) ;
#122749=CARTESIAN_POINT('',(0.299999999999999,-6.12928932188135,-27.0407106781187)) ;
#122750=CARTESIAN_POINT('',(0.4,-6.12928932188134,-27.0407106781187)) ;
#122751=CARTESIAN_POINT('',(0.058578643762692,-6.37071067811865,-26.7992893218813)) ;
#122752=CARTESIAN_POINT('',(0.152859547920897,-6.27642977396045,-26.8935702260396)) ;
#122753=CARTESIAN_POINT('',(0.4,-6.37071067811865,-26.7992893218813)) ;
#122754=CARTESIAN_POINT('Origin',(0.4,-6.1,-26.27)) ;
#122755=CARTESIAN_POINT('',(0.0585786437626916,-6.37071067811865,-26.5407106781187)) ;
#122756=CARTESIAN_POINT('',(0.299999999999992,-6.12928932188135,-26.2992893218814)) ;
#122757=CARTESIAN_POINT('',(0.352859547920897,-6.07642977396045,-26.2464297739604)) ;
#122758=CARTESIAN_POINT('',(-0.299999999999994,-6.12928932188135,-26.2992893218814)) ;
#122759=CARTESIAN_POINT('',(0.4,-6.12928932188135,-26.2992893218813)) ;
#122760=CARTESIAN_POINT('',(-0.0585786437626909,-6.37071067811865,-26.5407106781187)) ;
#122761=CARTESIAN_POINT('',(-0.0861928812542305,-6.34309644062712,-26.5130964406271)) ;
#122762=CARTESIAN_POINT('',(0.4,-6.37071067811865,-26.5407106781187)) ;
#122763=CARTESIAN_POINT('Origin',(0.4,-6.4,-22.96)) ;
#122764=CARTESIAN_POINT('',(-0.0585786437626899,-6.37071067811865,-22.9892893218813)) ;
#122765=CARTESIAN_POINT('',(-0.299999999999994,-6.12928932188135,-23.2307106781187)) ;
#122766=CARTESIAN_POINT('',(0.11380711874577,-6.54309644062711,-22.8169035593729)) ;
#122767=CARTESIAN_POINT('',(0.299999999999999,-6.12928932188135,-23.2307106781187)) ;
#122768=CARTESIAN_POINT('',(0.4,-6.12928932188134,-23.2307106781187)) ;
#122769=CARTESIAN_POINT('',(0.058578643762692,-6.37071067811865,-22.9892893218813)) ;
#122770=CARTESIAN_POINT('',(0.152859547920897,-6.27642977396045,-23.0835702260395)) ;
#122771=CARTESIAN_POINT('',(0.4,-6.37071067811865,-22.9892893218813)) ;
#122772=CARTESIAN_POINT('Origin',(0.4,-6.1,-22.46)) ;
#122773=CARTESIAN_POINT('',(0.0585786437626916,-6.37071067811865,-22.7307106781187)) ;
#122774=CARTESIAN_POINT('',(0.299999999999992,-6.12928932188135,-22.4892893218814)) ;
#122775=CARTESIAN_POINT('',(0.352859547920897,-6.07642977396045,-22.4364297739604)) ;
#122776=CARTESIAN_POINT('',(-0.299999999999994,-6.12928932188135,-22.4892893218814)) ;
#122777=CARTESIAN_POINT('',(0.4,-6.12928932188135,-22.4892893218814)) ;
#122778=CARTESIAN_POINT('',(-0.0585786437626909,-6.37071067811865,-22.7307106781187)) ;
#122779=CARTESIAN_POINT('',(-0.0861928812542305,-6.34309644062712,-22.7030964406271)) ;
#122780=CARTESIAN_POINT('',(0.4,-6.37071067811865,-22.7307106781187)) ;
#122781=CARTESIAN_POINT('Origin',(0.4,-6.4,-19.15)) ;
#122782=CARTESIAN_POINT('',(-0.0585786437626899,-6.37071067811865,-19.1792893218813)) ;
#122783=CARTESIAN_POINT('',(-0.299999999999994,-6.12928932188135,-19.4207106781187)) ;
#122784=CARTESIAN_POINT('',(0.11380711874577,-6.54309644062711,-19.0069035593729)) ;
#122785=CARTESIAN_POINT('',(0.299999999999999,-6.12928932188135,-19.4207106781187)) ;
#122786=CARTESIAN_POINT('',(0.4,-6.12928932188134,-19.4207106781187)) ;
#122787=CARTESIAN_POINT('',(0.058578643762692,-6.37071067811865,-19.1792893218813)) ;
#122788=CARTESIAN_POINT('',(0.152859547920897,-6.27642977396045,-19.2735702260396)) ;
#122789=CARTESIAN_POINT('',(0.4,-6.37071067811865,-19.1792893218813)) ;
#122790=CARTESIAN_POINT('Origin',(0.4,-6.1,-18.65)) ;
#122791=CARTESIAN_POINT('',(0.0585786437626916,-6.37071067811865,-18.9207106781187)) ;
#122792=CARTESIAN_POINT('',(0.299999999999992,-6.12928932188135,-18.6792893218814)) ;
#122793=CARTESIAN_POINT('',(0.352859547920897,-6.07642977396045,-18.6264297739605)) ;
#122794=CARTESIAN_POINT('',(-0.299999999999994,-6.12928932188135,-18.6792893218814)) ;
#122795=CARTESIAN_POINT('',(0.4,-6.12928932188135,-18.6792893218813)) ;
#122796=CARTESIAN_POINT('',(-0.0585786437626909,-6.37071067811865,-18.9207106781187)) ;
#122797=CARTESIAN_POINT('',(-0.0861928812542305,-6.34309644062712,-18.8930964406271)) ;
#122798=CARTESIAN_POINT('',(0.4,-6.37071067811865,-18.9207106781187)) ;
#122799=CARTESIAN_POINT('Origin',(0.4,-6.4,-15.34)) ;
#122800=CARTESIAN_POINT('',(-0.0585786437626904,-6.37071067811866,-15.3692893218813)) ;
#122801=CARTESIAN_POINT('',(-0.299999999999999,-6.12928932188134,-15.6107106781187)) ;
#122802=CARTESIAN_POINT('',(0.11380711874577,-6.54309644062711,-15.1969035593729)) ;
#122803=CARTESIAN_POINT('',(0.3,-6.12928932188134,-15.6107106781187)) ;
#122804=CARTESIAN_POINT('',(0.4,-6.12928932188134,-15.6107106781187)) ;
#122805=CARTESIAN_POINT('',(0.0585786437626911,-6.37071067811866,-15.3692893218813)) ;
#122806=CARTESIAN_POINT('',(0.152859547920897,-6.27642977396045,-15.4635702260396)) ;
#122807=CARTESIAN_POINT('',(0.4,-6.37071067811866,-15.3692893218813)) ;
#122808=CARTESIAN_POINT('Origin',(0.4,-6.1,-14.84)) ;
#122809=CARTESIAN_POINT('',(0.0585786437626904,-6.37071067811866,-15.1107106781187)) ;
#122810=CARTESIAN_POINT('',(0.299999999999999,-6.12928932188135,-14.8692893218813)) ;
#122811=CARTESIAN_POINT('',(0.352859547920896,-6.07642977396045,-14.8164297739604)) ;
#122812=CARTESIAN_POINT('',(-0.300000000000001,-6.12928932188134,-14.8692893218813)) ;
#122813=CARTESIAN_POINT('',(0.4,-6.12928932188134,-14.8692893218813)) ;
#122814=CARTESIAN_POINT('',(-0.0585786437626914,-6.37071067811866,-15.1107106781187)) ;
#122815=CARTESIAN_POINT('',(-0.0861928812542312,-6.34309644062712,-15.0830964406271)) ;
#122816=CARTESIAN_POINT('',(0.4,-6.37071067811866,-15.1107106781187)) ;
#122817=CARTESIAN_POINT('Origin',(0.4,-6.4,-11.53)) ;
#122818=CARTESIAN_POINT('',(-0.0585786437626916,-6.37071067811866,-11.5592893218813)) ;
#122819=CARTESIAN_POINT('',(-0.3,-6.12928932188135,-11.8007106781187)) ;
#122820=CARTESIAN_POINT('',(0.113807118745769,-6.54309644062712,-11.3869035593729)) ;
#122821=CARTESIAN_POINT('',(0.299999999999998,-6.12928932188135,-11.8007106781187)) ;
#122822=CARTESIAN_POINT('',(0.4,-6.12928932188134,-11.8007106781187)) ;
#122823=CARTESIAN_POINT('',(0.0585786437626907,-6.37071067811866,-11.5592893218813)) ;
#122824=CARTESIAN_POINT('',(0.152859547920896,-6.27642977396045,-11.6535702260396)) ;
#122825=CARTESIAN_POINT('',(0.4,-6.37071067811866,-11.5592893218813)) ;
#122826=CARTESIAN_POINT('Origin',(0.4,-6.1,-11.03)) ;
#122827=CARTESIAN_POINT('',(0.0585786437626913,-6.37071067811866,-11.3007106781187)) ;
#122828=CARTESIAN_POINT('',(0.300000000000001,-6.12928932188134,-11.0592893218813)) ;
#122829=CARTESIAN_POINT('',(0.352859547920897,-6.07642977396045,-11.0064297739604)) ;
#122830=CARTESIAN_POINT('',(-0.300000000000003,-6.12928932188134,-11.0592893218813)) ;
#122831=CARTESIAN_POINT('',(0.4,-6.12928932188134,-11.0592893218813)) ;
#122832=CARTESIAN_POINT('',(-0.0585786437626915,-6.37071067811866,-11.3007106781187)) ;
#122833=CARTESIAN_POINT('',(-0.0861928812542312,-6.34309644062712,-11.2730964406271)) ;
#122834=CARTESIAN_POINT('',(0.4,-6.37071067811866,-11.3007106781187)) ;
#122835=CARTESIAN_POINT('Origin',(0.4,-6.4,-7.72)) ;
#122836=CARTESIAN_POINT('',(-0.0585786437626906,-6.37071067811866,-7.74928932188134)) ;
#122837=CARTESIAN_POINT('',(-0.299999999999999,-6.12928932188134,-7.99071067811865)) ;
#122838=CARTESIAN_POINT('',(0.113807118745769,-6.54309644062711,-7.57690355937288)) ;
#122839=CARTESIAN_POINT('',(0.3,-6.12928932188134,-7.99071067811865)) ;
#122840=CARTESIAN_POINT('',(0.4,-6.12928932188134,-7.99071067811866)) ;
#122841=CARTESIAN_POINT('',(0.0585786437626912,-6.37071067811866,-7.74928932188134)) ;
#122842=CARTESIAN_POINT('',(0.152859547920897,-6.27642977396045,-7.84357022603955)) ;
#122843=CARTESIAN_POINT('',(0.4,-6.37071067811866,-7.74928932188134)) ;
#122844=CARTESIAN_POINT('Origin',(0.4,-6.1,-7.22)) ;
#122845=CARTESIAN_POINT('',(0.0585786437626908,-6.37071067811866,-7.49071067811866)) ;
#122846=CARTESIAN_POINT('',(0.300000000000002,-6.12928932188134,-7.24928932188134)) ;
#122847=CARTESIAN_POINT('',(0.352859547920897,-6.07642977396045,-7.19642977396045)) ;
#122848=CARTESIAN_POINT('',(-0.300000000000001,-6.12928932188134,-7.24928932188134)) ;
#122849=CARTESIAN_POINT('',(0.4,-6.12928932188134,-7.24928932188134)) ;
#122850=CARTESIAN_POINT('',(-0.0585786437626907,-6.37071067811866,-7.49071067811866)) ;
#122851=CARTESIAN_POINT('',(-0.0861928812542307,-6.34309644062712,-7.46309644062712)) ;
#122852=CARTESIAN_POINT('',(0.4,-6.37071067811866,-7.49071067811866)) ;
#122853=CARTESIAN_POINT('Origin',(0.4,-6.4,-3.91)) ;
#122854=CARTESIAN_POINT('',(-0.0585786437626904,-6.37071067811866,-3.93928932188134)) ;
#122855=CARTESIAN_POINT('',(-0.300000000000001,-6.12928932188134,-4.18071067811866)) ;
#122856=CARTESIAN_POINT('',(0.11380711874577,-6.54309644062711,-3.76690355937288)) ;
#122857=CARTESIAN_POINT('',(0.300000000000001,-6.12928932188134,-4.18071067811866)) ;
#122858=CARTESIAN_POINT('',(0.4,-6.12928932188134,-4.18071067811865)) ;
#122859=CARTESIAN_POINT('',(0.0585786437626911,-6.37071067811866,-3.93928932188134)) ;
#122860=CARTESIAN_POINT('',(0.152859547920897,-6.27642977396045,-4.03357022603955)) ;
#122861=CARTESIAN_POINT('',(0.4,-6.37071067811866,-3.93928932188134)) ;
#122862=CARTESIAN_POINT('Origin',(0.4,-6.1,-3.41)) ;
#122863=CARTESIAN_POINT('',(0.0585786437626907,-6.37071067811866,-3.68071067811866)) ;
#122864=CARTESIAN_POINT('',(0.299999999999999,-6.12928932188135,-3.43928932188135)) ;
#122865=CARTESIAN_POINT('',(0.352859547920897,-6.07642977396045,-3.38642977396045)) ;
#122866=CARTESIAN_POINT('',(-0.299999999999999,-6.12928932188135,-3.43928932188135)) ;
#122867=CARTESIAN_POINT('',(0.4,-6.12928932188134,-3.43928932188135)) ;
#122868=CARTESIAN_POINT('',(-0.0585786437626909,-6.37071067811866,-3.68071067811866)) ;
#122869=CARTESIAN_POINT('',(-0.086192881254231,-6.34309644062712,-3.65309644062712)) ;
#122870=CARTESIAN_POINT('',(0.4,-6.37071067811866,-3.68071067811866)) ;
#122871=CARTESIAN_POINT('Origin',(6.7,-0.399999999999999,-34.69)) ;
#122872=CARTESIAN_POINT('',(6.97071067811865,-0.0585786437626952,-34.4192893218813)) ;
#122873=CARTESIAN_POINT('',(6.72928932188135,-0.300000000000001,-34.6607106781186)) ;
#122874=CARTESIAN_POINT('',(6.67642977396045,-0.352859547920898,-34.7135702260396)) ;
#122875=CARTESIAN_POINT('',(6.72928932188134,0.3,-34.6607106781187)) ;
#122876=CARTESIAN_POINT('',(6.72928932188135,-0.399999999999999,-34.6607106781186)) ;
#122877=CARTESIAN_POINT('',(6.97071067811865,0.0585786437626901,-34.4192893218813)) ;
#122878=CARTESIAN_POINT('',(6.94309644062711,0.0861928812542281,-34.4469035593729)) ;
#122879=CARTESIAN_POINT('',(6.97071067811865,-0.4,-34.4192893218813)) ;
#122880=CARTESIAN_POINT('Origin',(7.,-0.399999999999999,-34.19)) ;
#122881=CARTESIAN_POINT('',(6.97071067811866,0.0585786437626919,-34.1607106781187)) ;
#122882=CARTESIAN_POINT('',(6.72928932188134,0.300000000000006,-33.9192893218814)) ;
#122883=CARTESIAN_POINT('',(7.14309644062712,-0.113807118745768,-34.3330964406271)) ;
#122884=CARTESIAN_POINT('',(6.72928932188134,-0.300000000000007,-33.9192893218813)) ;
#122885=CARTESIAN_POINT('',(6.72928932188134,-0.399999999999999,-33.9192893218814)) ;
#122886=CARTESIAN_POINT('',(6.97071067811866,-0.058578643762684,-34.1607106781187)) ;
#122887=CARTESIAN_POINT('',(6.87642977396045,-0.152859547920894,-34.0664297739605)) ;
#122888=CARTESIAN_POINT('',(6.97071067811866,-0.399999999999999,-34.1607106781187)) ;
#122889=CARTESIAN_POINT('Origin',(6.7,-0.399999999999999,-30.88)) ;
#122890=CARTESIAN_POINT('',(6.97071067811866,-0.0585786437626901,-30.6092893218813)) ;
#122891=CARTESIAN_POINT('',(6.72928932188135,-0.299999999999997,-30.8507106781187)) ;
#122892=CARTESIAN_POINT('',(6.67642977396045,-0.352859547920897,-30.9035702260396)) ;
#122893=CARTESIAN_POINT('',(6.72928932188135,0.299999999999998,-30.8507106781187)) ;
#122894=CARTESIAN_POINT('',(6.72928932188135,-0.399999999999999,-30.8507106781187)) ;
#122895=CARTESIAN_POINT('',(6.97071067811866,0.0585786437626903,-30.6092893218813)) ;
#122896=CARTESIAN_POINT('',(6.94309644062712,0.0861928812542301,-30.6369035593729)) ;
#122897=CARTESIAN_POINT('',(6.97071067811866,-0.4,-30.6092893218813)) ;
#122898=CARTESIAN_POINT('Origin',(7.,-0.399999999999999,-30.38)) ;
#122899=CARTESIAN_POINT('',(6.97071067811865,0.058578643762691,-30.3507106781187)) ;
#122900=CARTESIAN_POINT('',(6.72928932188135,0.299999999999994,-30.1092893218813)) ;
#122901=CARTESIAN_POINT('',(7.14309644062712,-0.11380711874577,-30.5230964406271)) ;
#122902=CARTESIAN_POINT('',(6.72928932188135,-0.299999999999999,-30.1092893218813)) ;
#122903=CARTESIAN_POINT('',(6.72928932188135,-0.399999999999999,-30.1092893218813)) ;
#122904=CARTESIAN_POINT('',(6.97071067811865,-0.0585786437626907,-30.3507106781187)) ;
#122905=CARTESIAN_POINT('',(6.87642977396045,-0.152859547920896,-30.2564297739604)) ;
#122906=CARTESIAN_POINT('',(6.97071067811865,-0.399999999999999,-30.3507106781187)) ;
#122907=CARTESIAN_POINT('Origin',(6.7,-0.399999999999999,-27.07)) ;
#122908=CARTESIAN_POINT('',(6.97071067811866,-0.0585786437626901,-26.7992893218813)) ;
#122909=CARTESIAN_POINT('',(6.72928932188135,-0.299999999999997,-27.0407106781187)) ;
#122910=CARTESIAN_POINT('',(6.67642977396045,-0.352859547920897,-27.0935702260396)) ;
#122911=CARTESIAN_POINT('',(6.72928932188135,0.299999999999998,-27.0407106781187)) ;
#122912=CARTESIAN_POINT('',(6.72928932188135,-0.399999999999999,-27.0407106781187)) ;
#122913=CARTESIAN_POINT('',(6.97071067811866,0.0585786437626903,-26.7992893218813)) ;
#122914=CARTESIAN_POINT('',(6.94309644062712,0.0861928812542301,-26.8269035593729)) ;
#122915=CARTESIAN_POINT('',(6.97071067811866,-0.4,-26.7992893218813)) ;
#122916=CARTESIAN_POINT('Origin',(7.,-0.399999999999999,-26.57)) ;
#122917=CARTESIAN_POINT('',(6.97071067811865,0.058578643762691,-26.5407106781187)) ;
#122918=CARTESIAN_POINT('',(6.72928932188135,0.299999999999994,-26.2992893218813)) ;
#122919=CARTESIAN_POINT('',(7.14309644062712,-0.11380711874577,-26.7130964406271)) ;
#122920=CARTESIAN_POINT('',(6.72928932188135,-0.299999999999999,-26.2992893218813)) ;
#122921=CARTESIAN_POINT('',(6.72928932188135,-0.399999999999999,-26.2992893218813)) ;
#122922=CARTESIAN_POINT('',(6.97071067811865,-0.0585786437626907,-26.5407106781187)) ;
#122923=CARTESIAN_POINT('',(6.87642977396045,-0.152859547920896,-26.4464297739605)) ;
#122924=CARTESIAN_POINT('',(6.97071067811865,-0.399999999999999,-26.5407106781187)) ;
#122925=CARTESIAN_POINT('Origin',(6.7,-0.399999999999999,-23.26)) ;
#122926=CARTESIAN_POINT('',(6.97071067811866,-0.0585786437626901,-22.9892893218813)) ;
#122927=CARTESIAN_POINT('',(6.72928932188135,-0.299999999999997,-23.2307106781187)) ;
#122928=CARTESIAN_POINT('',(6.67642977396045,-0.352859547920897,-23.2835702260396)) ;
#122929=CARTESIAN_POINT('',(6.72928932188135,0.299999999999998,-23.2307106781187)) ;
#122930=CARTESIAN_POINT('',(6.72928932188135,-0.399999999999999,-23.2307106781187)) ;
#122931=CARTESIAN_POINT('',(6.97071067811866,0.0585786437626903,-22.9892893218813)) ;
#122932=CARTESIAN_POINT('',(6.94309644062712,0.0861928812542301,-23.0169035593729)) ;
#122933=CARTESIAN_POINT('',(6.97071067811866,-0.4,-22.9892893218813)) ;
#122934=CARTESIAN_POINT('Origin',(7.,-0.399999999999999,-22.76)) ;
#122935=CARTESIAN_POINT('',(6.97071067811865,0.058578643762691,-22.7307106781187)) ;
#122936=CARTESIAN_POINT('',(6.72928932188135,0.299999999999994,-22.4892893218814)) ;
#122937=CARTESIAN_POINT('',(7.14309644062712,-0.11380711874577,-22.9030964406271)) ;
#122938=CARTESIAN_POINT('',(6.72928932188135,-0.299999999999999,-22.4892893218813)) ;
#122939=CARTESIAN_POINT('',(6.72928932188135,-0.399999999999999,-22.4892893218814)) ;
#122940=CARTESIAN_POINT('',(6.97071067811865,-0.0585786437626907,-22.7307106781187)) ;
#122941=CARTESIAN_POINT('',(6.87642977396045,-0.152859547920896,-22.6364297739605)) ;
#122942=CARTESIAN_POINT('',(6.97071067811865,-0.399999999999999,-22.7307106781187)) ;
#122943=CARTESIAN_POINT('Origin',(6.7,-0.399999999999999,-19.45)) ;
#122944=CARTESIAN_POINT('',(6.97071067811866,-0.0585786437626901,-19.1792893218813)) ;
#122945=CARTESIAN_POINT('',(6.72928932188135,-0.299999999999997,-19.4207106781187)) ;
#122946=CARTESIAN_POINT('',(6.67642977396045,-0.352859547920897,-19.4735702260396)) ;
#122947=CARTESIAN_POINT('',(6.72928932188135,0.299999999999998,-19.4207106781187)) ;
#122948=CARTESIAN_POINT('',(6.72928932188135,-0.399999999999999,-19.4207106781187)) ;
#122949=CARTESIAN_POINT('',(6.97071067811866,0.0585786437626903,-19.1792893218813)) ;
#122950=CARTESIAN_POINT('',(6.94309644062712,0.0861928812542301,-19.2069035593729)) ;
#122951=CARTESIAN_POINT('',(6.97071067811866,-0.4,-19.1792893218813)) ;
#122952=CARTESIAN_POINT('Origin',(7.,-0.399999999999999,-18.95)) ;
#122953=CARTESIAN_POINT('',(6.97071067811865,0.058578643762691,-18.9207106781187)) ;
#122954=CARTESIAN_POINT('',(6.72928932188135,0.299999999999992,-18.6792893218814)) ;
#122955=CARTESIAN_POINT('',(7.14309644062712,-0.11380711874577,-19.0930964406271)) ;
#122956=CARTESIAN_POINT('',(6.72928932188135,-0.299999999999999,-18.6792893218813)) ;
#122957=CARTESIAN_POINT('',(6.72928932188135,-0.399999999999999,-18.6792893218813)) ;
#122958=CARTESIAN_POINT('',(6.97071067811865,-0.0585786437626907,-18.9207106781187)) ;
#122959=CARTESIAN_POINT('',(6.87642977396045,-0.152859547920896,-18.8264297739604)) ;
#122960=CARTESIAN_POINT('',(6.97071067811865,-0.399999999999999,-18.9207106781187)) ;
#122961=CARTESIAN_POINT('Origin',(6.7,-0.399999999999999,-15.64)) ;
#122962=CARTESIAN_POINT('',(6.97071067811866,-0.058578643762691,-15.3692893218813)) ;
#122963=CARTESIAN_POINT('',(6.72928932188135,-0.299999999999999,-15.6107106781187)) ;
#122964=CARTESIAN_POINT('',(6.67642977396045,-0.352859547920897,-15.6635702260396)) ;
#122965=CARTESIAN_POINT('',(6.72928932188134,0.300000000000003,-15.6107106781187)) ;
#122966=CARTESIAN_POINT('',(6.72928932188135,-0.399999999999999,-15.6107106781187)) ;
#122967=CARTESIAN_POINT('',(6.97071067811866,0.0585786437626913,-15.3692893218813)) ;
#122968=CARTESIAN_POINT('',(6.94309644062712,0.086192881254231,-15.3969035593729)) ;
#122969=CARTESIAN_POINT('',(6.97071067811866,-0.4,-15.3692893218813)) ;
#122970=CARTESIAN_POINT('Origin',(7.,-0.399999999999999,-15.14)) ;
#122971=CARTESIAN_POINT('',(6.97071067811865,0.0585786437626917,-15.1107106781187)) ;
#122972=CARTESIAN_POINT('',(6.72928932188135,0.3,-14.8692893218813)) ;
#122973=CARTESIAN_POINT('',(7.14309644062712,-0.11380711874577,-15.2830964406271)) ;
#122974=CARTESIAN_POINT('',(6.72928932188135,-0.299999999999999,-14.8692893218813)) ;
#122975=CARTESIAN_POINT('',(6.72928932188135,-0.399999999999999,-14.8692893218813)) ;
#122976=CARTESIAN_POINT('',(6.97071067811865,-0.0585786437626915,-15.1107106781187)) ;
#122977=CARTESIAN_POINT('',(6.87642977396045,-0.152859547920897,-15.0164297739605)) ;
#122978=CARTESIAN_POINT('',(6.97071067811865,-0.399999999999999,-15.1107106781187)) ;
#122979=CARTESIAN_POINT('Origin',(6.7,-0.399999999999999,-11.83)) ;
#122980=CARTESIAN_POINT('',(6.97071067811866,-0.058578643762691,-11.5592893218813)) ;
#122981=CARTESIAN_POINT('',(6.72928932188134,-0.300000000000002,-11.8007106781187)) ;
#122982=CARTESIAN_POINT('',(6.67642977396045,-0.352859547920897,-11.8535702260395)) ;
#122983=CARTESIAN_POINT('',(6.72928932188135,0.300000000000002,-11.8007106781187)) ;
#122984=CARTESIAN_POINT('',(6.72928932188135,-0.399999999999999,-11.8007106781187)) ;
#122985=CARTESIAN_POINT('',(6.97071067811866,0.0585786437626919,-11.5592893218813)) ;
#122986=CARTESIAN_POINT('',(6.94309644062712,0.0861928812542313,-11.5869035593729)) ;
#122987=CARTESIAN_POINT('',(6.97071067811866,-0.4,-11.5592893218813)) ;
#122988=CARTESIAN_POINT('Origin',(7.,-0.399999999999999,-11.33)) ;
#122989=CARTESIAN_POINT('',(6.97071067811865,0.0585786437626923,-11.3007106781187)) ;
#122990=CARTESIAN_POINT('',(6.72928932188135,0.300000000000001,-11.0592893218813)) ;
#122991=CARTESIAN_POINT('',(7.14309644062712,-0.113807118745769,-11.4730964406271)) ;
#122992=CARTESIAN_POINT('',(6.72928932188135,-0.300000000000002,-11.0592893218813)) ;
#122993=CARTESIAN_POINT('',(6.72928932188134,-0.399999999999999,-11.0592893218813)) ;
#122994=CARTESIAN_POINT('',(6.97071067811865,-0.0585786437626925,-11.3007106781187)) ;
#122995=CARTESIAN_POINT('',(6.87642977396045,-0.152859547920897,-11.2064297739604)) ;
#122996=CARTESIAN_POINT('',(6.97071067811865,-0.399999999999999,-11.3007106781187)) ;
#122997=CARTESIAN_POINT('Origin',(6.7,-0.399999999999999,-8.02)) ;
#122998=CARTESIAN_POINT('',(6.97071067811866,-0.0585786437626908,-7.74928932188134)) ;
#122999=CARTESIAN_POINT('',(6.72928932188134,-0.300000000000002,-7.99071067811866)) ;
#123000=CARTESIAN_POINT('',(6.67642977396045,-0.352859547920897,-8.04357022603955)) ;
#123001=CARTESIAN_POINT('',(6.72928932188135,0.300000000000002,-7.99071067811866)) ;
#123002=CARTESIAN_POINT('',(6.72928932188135,-0.399999999999999,-7.99071067811866)) ;
#123003=CARTESIAN_POINT('',(6.97071067811866,0.0585786437626916,-7.74928932188134)) ;
#123004=CARTESIAN_POINT('',(6.94309644062712,0.0861928812542312,-7.77690355937288)) ;
#123005=CARTESIAN_POINT('',(6.97071067811866,-0.4,-7.74928932188134)) ;
#123006=CARTESIAN_POINT('Origin',(7.,-0.399999999999999,-7.52)) ;
#123007=CARTESIAN_POINT('',(6.97071067811866,0.0585786437626905,-7.49071067811866)) ;
#123008=CARTESIAN_POINT('',(6.72928932188134,0.300000000000002,-7.24928932188134)) ;
#123009=CARTESIAN_POINT('',(7.14309644062712,-0.11380711874577,-7.66309644062712)) ;
#123010=CARTESIAN_POINT('',(6.72928932188135,-0.300000000000002,-7.24928932188134)) ;
#123011=CARTESIAN_POINT('',(6.72928932188135,-0.399999999999999,-7.24928932188134)) ;
#123012=CARTESIAN_POINT('',(6.97071067811866,-0.058578643762691,-7.49071067811866)) ;
#123013=CARTESIAN_POINT('',(6.87642977396045,-0.152859547920897,-7.39642977396045)) ;
#123014=CARTESIAN_POINT('',(6.97071067811866,-0.399999999999999,-7.49071067811866)) ;
#123015=CARTESIAN_POINT('Origin',(6.7,-0.399999999999999,-4.21)) ;
#123016=CARTESIAN_POINT('',(6.97071067811866,-0.058578643762691,-3.93928932188135)) ;
#123017=CARTESIAN_POINT('',(6.72928932188135,-0.300000000000001,-4.18071067811866)) ;
#123018=CARTESIAN_POINT('',(6.67642977396045,-0.352859547920897,-4.23357022603955)) ;
#123019=CARTESIAN_POINT('',(6.72928932188135,0.300000000000001,-4.18071067811866)) ;
#123020=CARTESIAN_POINT('',(6.72928932188135,-0.399999999999999,-4.18071067811866)) ;
#123021=CARTESIAN_POINT('',(6.97071067811866,0.0585786437626911,-3.93928932188135)) ;
#123022=CARTESIAN_POINT('',(6.94309644062712,0.0861928812542308,-3.96690355937289)) ;
#123023=CARTESIAN_POINT('',(6.97071067811866,-0.4,-3.93928932188135)) ;
#123024=CARTESIAN_POINT('Origin',(7.,-0.399999999999999,-3.71)) ;
#123025=CARTESIAN_POINT('',(6.97071067811866,0.058578643762691,-3.68071067811866)) ;
#123026=CARTESIAN_POINT('',(6.72928932188135,0.3,-3.43928932188135)) ;
#123027=CARTESIAN_POINT('',(7.14309644062712,-0.11380711874577,-3.85309644062712)) ;
#123028=CARTESIAN_POINT('',(6.72928932188135,-0.3,-3.43928932188135)) ;
#123029=CARTESIAN_POINT('',(6.72928932188135,-0.399999999999999,-3.43928932188135)) ;
#123030=CARTESIAN_POINT('',(6.97071067811866,-0.0585786437626913,-3.68071067811866)) ;
#123031=CARTESIAN_POINT('',(6.87642977396045,-0.152859547920897,-3.58642977396045)) ;
#123032=CARTESIAN_POINT('',(6.97071067811866,-0.399999999999999,-3.68071067811866)) ;
#123033=CARTESIAN_POINT('Origin',(-0.113807118745769,-6.47238576250846,
-3.69619288125423)) ;
#123034=CARTESIAN_POINT('Origin',(0.3,-6.05857864376269,-4.11)) ;
#123035=CARTESIAN_POINT('Origin',(0.0585786437626911,-6.3,-3.86857864376269)) ;
#123036=CARTESIAN_POINT('Origin',(0.3,-6.05857864376269,-3.41)) ;
#123037=CARTESIAN_POINT('Origin',(0.3,-6.05857864376269,-4.11)) ;
#123038=CARTESIAN_POINT('Origin',(0.3,-6.05857864376269,-3.51)) ;
#123039=CARTESIAN_POINT('Origin',(0.0585786437626908,-6.3,-3.86857864376269)) ;
#123040=CARTESIAN_POINT('Origin',(0.0585786437626908,-6.3,-3.86857864376269)) ;
#123041=CARTESIAN_POINT('Origin',(0.0585786437626908,-6.3,-3.86857864376269)) ;
#123042=CARTESIAN_POINT('Origin',(0.152859547920897,-6.20571909584179,-3.6571404520791)) ;
#123043=CARTESIAN_POINT('Origin',(0.3,-6.05857864376269,-3.51)) ;
#123044=CARTESIAN_POINT('Origin',(0.0585786437626908,-6.3,-3.75142135623731)) ;
#123045=CARTESIAN_POINT('Origin',(0.0585786437626908,-6.3,-3.41)) ;
#123046=CARTESIAN_POINT('Origin',(0.0585786437626908,-6.3,-3.75142135623731)) ;
#123047=CARTESIAN_POINT('Origin',(0.4,-6.3,-3.86857864376269)) ;
#123048=CARTESIAN_POINT('Origin',(-0.0585786437626904,-6.3,-3.86857864376269)) ;
#123049=CARTESIAN_POINT('Origin',(0.0585786437626908,-6.3,-3.75142135623731)) ;
#123050=CARTESIAN_POINT('Origin',(0.0585786437626907,-6.3,-3.75142135623731)) ;
#123051=CARTESIAN_POINT('Origin',(-0.0585786437626908,-6.3,-3.86857864376269)) ;
#123052=CARTESIAN_POINT('Origin',(-0.0585786437626908,-6.3,-3.86857864376269)) ;
#123053=CARTESIAN_POINT('Origin',(-0.0585786437626908,-6.3,-3.86857864376269)) ;
#123054=CARTESIAN_POINT('Origin',(-0.1,-6.3,-3.75142135623731)) ;
#123055=CARTESIAN_POINT('Origin',(-0.0585786437626908,-6.3,-3.75142135623731)) ;
#123056=CARTESIAN_POINT('Origin',(-0.0585786437626908,-6.3,-3.41)) ;
#123057=CARTESIAN_POINT('Origin',(-0.0585786437626908,-6.3,-3.75142135623731)) ;
#123058=CARTESIAN_POINT('Origin',(-0.0861928812542299,-6.27238576250846,
-3.89619288125423)) ;
#123059=CARTESIAN_POINT('Origin',(-0.3,-6.05857864376269,-4.11)) ;
#123060=CARTESIAN_POINT('Origin',(-0.0585786437626908,-6.3,-3.75142135623731)) ;
#123061=CARTESIAN_POINT('Origin',(-0.0585786437626909,-6.3,-3.75142135623731)) ;
#123062=CARTESIAN_POINT('Origin',(-0.3,-6.05857864376269,-3.41)) ;
#123063=CARTESIAN_POINT('Origin',(-0.3,-6.05857864376269,-4.11)) ;
#123064=CARTESIAN_POINT('Origin',(-0.3,-6.05857864376269,-3.51)) ;
#123065=CARTESIAN_POINT('Origin',(-0.352859547920897,-6.00571909584179,
-3.4571404520791)) ;
#123066=CARTESIAN_POINT('Origin',(-0.3,-6.05857864376269,-3.51)) ;
#123067=CARTESIAN_POINT('Origin',(7.07238576250846,-0.11380711874577,-3.69619288125423)) ;
#123068=CARTESIAN_POINT('Origin',(6.65857864376269,0.300000000000001,-4.11)) ;
#123069=CARTESIAN_POINT('Origin',(6.9,0.0585786437626911,-3.86857864376269)) ;
#123070=CARTESIAN_POINT('Origin',(6.65857864376269,0.300000000000001,-3.41)) ;
#123071=CARTESIAN_POINT('Origin',(6.65857864376269,0.300000000000001,-4.11)) ;
#123072=CARTESIAN_POINT('Origin',(6.65857864376269,0.300000000000001,-3.51)) ;
#123073=CARTESIAN_POINT('Origin',(6.9,0.0585786437626909,-3.86857864376269)) ;
#123074=CARTESIAN_POINT('Origin',(6.9,0.0585786437626909,-3.86857864376269)) ;
#123075=CARTESIAN_POINT('Origin',(6.9,0.0585786437626909,-3.86857864376269)) ;
#123076=CARTESIAN_POINT('Origin',(6.80571909584179,0.152859547920897,-3.6571404520791)) ;
#123077=CARTESIAN_POINT('Origin',(6.65857864376269,0.300000000000001,-3.51)) ;
#123078=CARTESIAN_POINT('Origin',(6.9,0.0585786437626909,-3.75142135623731)) ;
#123079=CARTESIAN_POINT('Origin',(6.9,0.0585786437626909,-3.41)) ;
#123080=CARTESIAN_POINT('Origin',(6.9,0.0585786437626909,-3.75142135623731)) ;
#123081=CARTESIAN_POINT('Origin',(6.9,-0.1,-3.86857864376269)) ;
#123082=CARTESIAN_POINT('Origin',(6.9,-0.058578643762691,-3.86857864376269)) ;
#123083=CARTESIAN_POINT('Origin',(6.9,0.0585786437626909,-3.75142135623731)) ;
#123084=CARTESIAN_POINT('Origin',(6.9,0.058578643762691,-3.75142135623731)) ;
#123085=CARTESIAN_POINT('Origin',(6.9,-0.0585786437626909,-3.86857864376269)) ;
#123086=CARTESIAN_POINT('Origin',(6.9,-0.0585786437626909,-3.86857864376269)) ;
#123087=CARTESIAN_POINT('Origin',(6.9,-0.0585786437626909,-3.86857864376269)) ;
#123088=CARTESIAN_POINT('Origin',(6.9,-0.399999999999999,-3.75142135623731)) ;
#123089=CARTESIAN_POINT('Origin',(6.9,-0.0585786437626909,-3.75142135623731)) ;
#123090=CARTESIAN_POINT('Origin',(6.9,-0.0585786437626909,-3.41)) ;
#123091=CARTESIAN_POINT('Origin',(6.9,-0.0585786437626909,-3.75142135623731)) ;
#123092=CARTESIAN_POINT('Origin',(6.87238576250846,-0.0861928812542305,
-3.89619288125423)) ;
#123093=CARTESIAN_POINT('Origin',(6.65857864376269,-0.3,-4.11)) ;
#123094=CARTESIAN_POINT('Origin',(6.9,-0.0585786437626909,-3.75142135623731)) ;
#123095=CARTESIAN_POINT('Origin',(6.9,-0.0585786437626913,-3.75142135623731)) ;
#123096=CARTESIAN_POINT('Origin',(6.65857864376269,-0.300000000000001,-3.41)) ;
#123097=CARTESIAN_POINT('Origin',(6.65857864376269,-0.300000000000001,-4.11)) ;
#123098=CARTESIAN_POINT('Origin',(6.65857864376269,-0.300000000000001,-3.51)) ;
#123099=CARTESIAN_POINT('Origin',(6.60571909584179,-0.352859547920897,-3.4571404520791)) ;
#123100=CARTESIAN_POINT('Origin',(6.65857864376269,-0.300000000000001,-3.51)) ;
#123101=CARTESIAN_POINT('Origin',(-0.11380711874577,-6.47238576250846,-7.50619288125423)) ;
#123102=CARTESIAN_POINT('Origin',(0.300000000000001,-6.05857864376269,-7.92)) ;
#123103=CARTESIAN_POINT('Origin',(0.0585786437626912,-6.3,-7.67857864376269)) ;
#123104=CARTESIAN_POINT('Origin',(0.3,-6.05857864376269,-7.22)) ;
#123105=CARTESIAN_POINT('Origin',(0.3,-6.05857864376269,-7.92)) ;
#123106=CARTESIAN_POINT('Origin',(0.3,-6.05857864376269,-7.32)) ;
#123107=CARTESIAN_POINT('Origin',(0.0585786437626908,-6.3,-7.67857864376269)) ;
#123108=CARTESIAN_POINT('Origin',(0.0585786437626908,-6.3,-7.67857864376269)) ;
#123109=CARTESIAN_POINT('Origin',(0.0585786437626908,-6.3,-7.67857864376269)) ;
#123110=CARTESIAN_POINT('Origin',(0.152859547920898,-6.20571909584179,-7.4671404520791)) ;
#123111=CARTESIAN_POINT('Origin',(0.300000000000001,-6.05857864376269,-7.32)) ;
#123112=CARTESIAN_POINT('Origin',(0.0585786437626908,-6.3,-7.56142135623731)) ;
#123113=CARTESIAN_POINT('Origin',(0.0585786437626908,-6.3,-7.22)) ;
#123114=CARTESIAN_POINT('Origin',(0.0585786437626908,-6.3,-7.56142135623731)) ;
#123115=CARTESIAN_POINT('Origin',(0.4,-6.3,-7.67857864376269)) ;
#123116=CARTESIAN_POINT('Origin',(-0.0585786437626906,-6.3,-7.67857864376269)) ;
#123117=CARTESIAN_POINT('Origin',(0.0585786437626908,-6.3,-7.56142135623731)) ;
#123118=CARTESIAN_POINT('Origin',(0.0585786437626908,-6.3,-7.56142135623731)) ;
#123119=CARTESIAN_POINT('Origin',(-0.0585786437626908,-6.3,-7.67857864376269)) ;
#123120=CARTESIAN_POINT('Origin',(-0.0585786437626907,-6.3,-7.67857864376269)) ;
#123121=CARTESIAN_POINT('Origin',(-0.0585786437626908,-6.3,-7.67857864376269)) ;
#123122=CARTESIAN_POINT('Origin',(-0.1,-6.3,-7.56142135623731)) ;
#123123=CARTESIAN_POINT('Origin',(-0.0585786437626908,-6.3,-7.56142135623731)) ;
#123124=CARTESIAN_POINT('Origin',(-0.0585786437626908,-6.3,-7.22)) ;
#123125=CARTESIAN_POINT('Origin',(-0.0585786437626908,-6.3,-7.56142135623731)) ;
#123126=CARTESIAN_POINT('Origin',(-0.0861928812542296,-6.27238576250846,
-7.70619288125423)) ;
#123127=CARTESIAN_POINT('Origin',(-0.3,-6.05857864376269,-7.92)) ;
#123128=CARTESIAN_POINT('Origin',(-0.0585786437626908,-6.3,-7.56142135623731)) ;
#123129=CARTESIAN_POINT('Origin',(-0.0585786437626907,-6.3,-7.56142135623731)) ;
#123130=CARTESIAN_POINT('Origin',(-0.3,-6.05857864376269,-7.22)) ;
#123131=CARTESIAN_POINT('Origin',(-0.3,-6.05857864376269,-7.92)) ;
#123132=CARTESIAN_POINT('Origin',(-0.3,-6.05857864376269,-7.32)) ;
#123133=CARTESIAN_POINT('Origin',(-0.352859547920897,-6.00571909584179,
-7.2671404520791)) ;
#123134=CARTESIAN_POINT('Origin',(-0.300000000000001,-6.05857864376269,
-7.32)) ;
#123135=CARTESIAN_POINT('Origin',(7.07238576250846,-0.11380711874577,-7.50619288125423)) ;
#123136=CARTESIAN_POINT('Origin',(6.65857864376269,0.300000000000002,-7.92)) ;
#123137=CARTESIAN_POINT('Origin',(6.9,0.0585786437626916,-7.67857864376269)) ;
#123138=CARTESIAN_POINT('Origin',(6.65857864376269,0.300000000000001,-7.22)) ;
#123139=CARTESIAN_POINT('Origin',(6.65857864376269,0.300000000000001,-7.92)) ;
#123140=CARTESIAN_POINT('Origin',(6.65857864376269,0.300000000000001,-7.32)) ;
#123141=CARTESIAN_POINT('Origin',(6.9,0.0585786437626909,-7.67857864376269)) ;
#123142=CARTESIAN_POINT('Origin',(6.9,0.0585786437626909,-7.67857864376269)) ;
#123143=CARTESIAN_POINT('Origin',(6.9,0.0585786437626909,-7.67857864376269)) ;
#123144=CARTESIAN_POINT('Origin',(6.80571909584179,0.152859547920898,-7.4671404520791)) ;
#123145=CARTESIAN_POINT('Origin',(6.65857864376269,0.300000000000002,-7.32)) ;
#123146=CARTESIAN_POINT('Origin',(6.9,0.0585786437626908,-7.56142135623731)) ;
#123147=CARTESIAN_POINT('Origin',(6.9,0.0585786437626909,-7.22)) ;
#123148=CARTESIAN_POINT('Origin',(6.9,0.0585786437626909,-7.56142135623731)) ;
#123149=CARTESIAN_POINT('Origin',(6.9,-0.1,-7.67857864376269)) ;
#123150=CARTESIAN_POINT('Origin',(6.9,-0.0585786437626908,-7.67857864376269)) ;
#123151=CARTESIAN_POINT('Origin',(6.9,0.0585786437626909,-7.56142135623731)) ;
#123152=CARTESIAN_POINT('Origin',(6.9,0.0585786437626905,-7.56142135623731)) ;
#123153=CARTESIAN_POINT('Origin',(6.9,-0.058578643762691,-7.67857864376269)) ;
#123154=CARTESIAN_POINT('Origin',(6.9,-0.058578643762691,-7.67857864376269)) ;
#123155=CARTESIAN_POINT('Origin',(6.9,-0.0585786437626909,-7.67857864376269)) ;
#123156=CARTESIAN_POINT('Origin',(6.9,-0.399999999999999,-7.56142135623731)) ;
#123157=CARTESIAN_POINT('Origin',(6.9,-0.0585786437626909,-7.56142135623731)) ;
#123158=CARTESIAN_POINT('Origin',(6.9,-0.0585786437626909,-7.22)) ;
#123159=CARTESIAN_POINT('Origin',(6.9,-0.0585786437626909,-7.56142135623731)) ;
#123160=CARTESIAN_POINT('Origin',(6.87238576250846,-0.0861928812542304,
-7.70619288125423)) ;
#123161=CARTESIAN_POINT('Origin',(6.65857864376269,-0.300000000000001,-7.92)) ;
#123162=CARTESIAN_POINT('Origin',(6.9,-0.058578643762691,-7.56142135623731)) ;
#123163=CARTESIAN_POINT('Origin',(6.9,-0.058578643762691,-7.56142135623731)) ;
#123164=CARTESIAN_POINT('Origin',(6.65857864376269,-0.300000000000001,-7.22)) ;
#123165=CARTESIAN_POINT('Origin',(6.65857864376269,-0.300000000000001,-7.92)) ;
#123166=CARTESIAN_POINT('Origin',(6.65857864376269,-0.300000000000001,-7.32)) ;
#123167=CARTESIAN_POINT('Origin',(6.60571909584179,-0.352859547920898,-7.2671404520791)) ;
#123168=CARTESIAN_POINT('Origin',(6.65857864376269,-0.300000000000001,-7.32)) ;
#123169=CARTESIAN_POINT('Origin',(-0.11380711874577,-6.47238576250846,-11.3161928812542)) ;
#123170=CARTESIAN_POINT('Origin',(0.299999999999999,-6.05857864376269,-11.73)) ;
#123171=CARTESIAN_POINT('Origin',(0.0585786437626907,-6.3,-11.4885786437627)) ;
#123172=CARTESIAN_POINT('Origin',(0.3,-6.05857864376269,-11.03)) ;
#123173=CARTESIAN_POINT('Origin',(0.3,-6.05857864376269,-11.73)) ;
#123174=CARTESIAN_POINT('Origin',(0.3,-6.05857864376269,-11.13)) ;
#123175=CARTESIAN_POINT('Origin',(0.0585786437626908,-6.3,-11.4885786437627)) ;
#123176=CARTESIAN_POINT('Origin',(0.0585786437626908,-6.3,-11.4885786437627)) ;
#123177=CARTESIAN_POINT('Origin',(0.0585786437626908,-6.3,-11.4885786437627)) ;
#123178=CARTESIAN_POINT('Origin',(0.152859547920898,-6.20571909584179,-11.2771404520791)) ;
#123179=CARTESIAN_POINT('Origin',(0.300000000000003,-6.05857864376269,-11.13)) ;
#123180=CARTESIAN_POINT('Origin',(0.0585786437626905,-6.3,-11.3714213562373)) ;
#123181=CARTESIAN_POINT('Origin',(0.0585786437626908,-6.3,-11.03)) ;
#123182=CARTESIAN_POINT('Origin',(0.0585786437626908,-6.3,-11.3714213562373)) ;
#123183=CARTESIAN_POINT('Origin',(0.4,-6.3,-11.4885786437627)) ;
#123184=CARTESIAN_POINT('Origin',(-0.0585786437626916,-6.3,-11.4885786437627)) ;
#123185=CARTESIAN_POINT('Origin',(0.0585786437626908,-6.3,-11.3714213562373)) ;
#123186=CARTESIAN_POINT('Origin',(0.0585786437626913,-6.3,-11.3714213562373)) ;
#123187=CARTESIAN_POINT('Origin',(-0.0585786437626908,-6.3,-11.4885786437627)) ;
#123188=CARTESIAN_POINT('Origin',(-0.0585786437626908,-6.3,-11.4885786437627)) ;
#123189=CARTESIAN_POINT('Origin',(-0.0585786437626908,-6.3,-11.4885786437627)) ;
#123190=CARTESIAN_POINT('Origin',(-0.1,-6.3,-11.3714213562373)) ;
#123191=CARTESIAN_POINT('Origin',(-0.0585786437626908,-6.3,-11.3714213562373)) ;
#123192=CARTESIAN_POINT('Origin',(-0.0585786437626908,-6.3,-11.03)) ;
#123193=CARTESIAN_POINT('Origin',(-0.0585786437626908,-6.3,-11.3714213562373)) ;
#123194=CARTESIAN_POINT('Origin',(-0.0861928812542293,-6.27238576250846,
-11.5161928812542)) ;
#123195=CARTESIAN_POINT('Origin',(-0.3,-6.05857864376269,-11.73)) ;
#123196=CARTESIAN_POINT('Origin',(-0.0585786437626908,-6.3,-11.3714213562373)) ;
#123197=CARTESIAN_POINT('Origin',(-0.0585786437626915,-6.3,-11.3714213562373)) ;
#123198=CARTESIAN_POINT('Origin',(-0.3,-6.05857864376269,-11.03)) ;
#123199=CARTESIAN_POINT('Origin',(-0.3,-6.05857864376269,-11.73)) ;
#123200=CARTESIAN_POINT('Origin',(-0.3,-6.05857864376269,-11.13)) ;
#123201=CARTESIAN_POINT('Origin',(-0.352859547920898,-6.00571909584179,
-11.0771404520791)) ;
#123202=CARTESIAN_POINT('Origin',(-0.300000000000003,-6.05857864376269,
-11.13)) ;
#123203=CARTESIAN_POINT('Origin',(7.07238576250846,-0.11380711874577,-11.3161928812542)) ;
#123204=CARTESIAN_POINT('Origin',(6.65857864376269,0.300000000000003,-11.73)) ;
#123205=CARTESIAN_POINT('Origin',(6.9,0.0585786437626919,-11.4885786437627)) ;
#123206=CARTESIAN_POINT('Origin',(6.65857864376269,0.300000000000001,-11.03)) ;
#123207=CARTESIAN_POINT('Origin',(6.65857864376269,0.300000000000001,-11.73)) ;
#123208=CARTESIAN_POINT('Origin',(6.65857864376269,0.300000000000001,-11.13)) ;
#123209=CARTESIAN_POINT('Origin',(6.9,0.0585786437626909,-11.4885786437627)) ;
#123210=CARTESIAN_POINT('Origin',(6.9,0.0585786437626909,-11.4885786437627)) ;
#123211=CARTESIAN_POINT('Origin',(6.9,0.0585786437626909,-11.4885786437627)) ;
#123212=CARTESIAN_POINT('Origin',(6.80571909584179,0.152859547920898,-11.2771404520791)) ;
#123213=CARTESIAN_POINT('Origin',(6.65857864376269,0.300000000000003,-11.13)) ;
#123214=CARTESIAN_POINT('Origin',(6.9,0.0585786437626911,-11.3714213562373)) ;
#123215=CARTESIAN_POINT('Origin',(6.9,0.0585786437626909,-11.03)) ;
#123216=CARTESIAN_POINT('Origin',(6.9,0.0585786437626909,-11.3714213562373)) ;
#123217=CARTESIAN_POINT('Origin',(6.9,-0.1,-11.4885786437627)) ;
#123218=CARTESIAN_POINT('Origin',(6.9,-0.058578643762691,-11.4885786437627)) ;
#123219=CARTESIAN_POINT('Origin',(6.9,0.0585786437626909,-11.3714213562373)) ;
#123220=CARTESIAN_POINT('Origin',(6.9,0.0585786437626923,-11.3714213562373)) ;
#123221=CARTESIAN_POINT('Origin',(6.9,-0.058578643762691,-11.4885786437627)) ;
#123222=CARTESIAN_POINT('Origin',(6.9,-0.0585786437626912,-11.4885786437627)) ;
#123223=CARTESIAN_POINT('Origin',(6.9,-0.0585786437626909,-11.4885786437627)) ;
#123224=CARTESIAN_POINT('Origin',(6.9,-0.399999999999999,-11.3714213562373)) ;
#123225=CARTESIAN_POINT('Origin',(6.9,-0.0585786437626909,-11.3714213562373)) ;
#123226=CARTESIAN_POINT('Origin',(6.9,-0.0585786437626909,-11.03)) ;
#123227=CARTESIAN_POINT('Origin',(6.9,-0.0585786437626909,-11.3714213562373)) ;
#123228=CARTESIAN_POINT('Origin',(6.87238576250846,-0.0861928812542304,
-11.5161928812542)) ;
#123229=CARTESIAN_POINT('Origin',(6.65857864376269,-0.300000000000002,-11.73)) ;
#123230=CARTESIAN_POINT('Origin',(6.9,-0.058578643762691,-11.3714213562373)) ;
#123231=CARTESIAN_POINT('Origin',(6.9,-0.0585786437626925,-11.3714213562373)) ;
#123232=CARTESIAN_POINT('Origin',(6.65857864376269,-0.300000000000001,-11.03)) ;
#123233=CARTESIAN_POINT('Origin',(6.65857864376269,-0.300000000000001,-11.73)) ;
#123234=CARTESIAN_POINT('Origin',(6.65857864376269,-0.300000000000001,-11.13)) ;
#123235=CARTESIAN_POINT('Origin',(6.60571909584179,-0.352859547920898,-11.0771404520791)) ;
#123236=CARTESIAN_POINT('Origin',(6.65857864376269,-0.300000000000003,-11.13)) ;
#123237=CARTESIAN_POINT('Origin',(-0.113807118745769,-6.47238576250846,
-15.1261928812542)) ;
#123238=CARTESIAN_POINT('Origin',(0.300000000000001,-6.05857864376269,-15.54)) ;
#123239=CARTESIAN_POINT('Origin',(0.0585786437626911,-6.3,-15.2985786437627)) ;
#123240=CARTESIAN_POINT('Origin',(0.3,-6.05857864376269,-14.84)) ;
#123241=CARTESIAN_POINT('Origin',(0.3,-6.05857864376269,-15.54)) ;
#123242=CARTESIAN_POINT('Origin',(0.3,-6.05857864376269,-14.94)) ;
#123243=CARTESIAN_POINT('Origin',(0.0585786437626908,-6.3,-15.2985786437627)) ;
#123244=CARTESIAN_POINT('Origin',(0.0585786437626908,-6.3,-15.2985786437627)) ;
#123245=CARTESIAN_POINT('Origin',(0.0585786437626908,-6.3,-15.2985786437627)) ;
#123246=CARTESIAN_POINT('Origin',(0.152859547920898,-6.20571909584179,-15.0871404520791)) ;
#123247=CARTESIAN_POINT('Origin',(0.300000000000001,-6.05857864376269,-14.94)) ;
#123248=CARTESIAN_POINT('Origin',(0.0585786437626911,-6.3,-15.1814213562373)) ;
#123249=CARTESIAN_POINT('Origin',(0.0585786437626908,-6.3,-14.84)) ;
#123250=CARTESIAN_POINT('Origin',(0.0585786437626908,-6.3,-15.1814213562373)) ;
#123251=CARTESIAN_POINT('Origin',(0.4,-6.3,-15.2985786437627)) ;
#123252=CARTESIAN_POINT('Origin',(-0.0585786437626904,-6.3,-15.2985786437627)) ;
#123253=CARTESIAN_POINT('Origin',(0.0585786437626908,-6.3,-15.1814213562373)) ;
#123254=CARTESIAN_POINT('Origin',(0.0585786437626904,-6.3,-15.1814213562373)) ;
#123255=CARTESIAN_POINT('Origin',(-0.0585786437626908,-6.3,-15.2985786437627)) ;
#123256=CARTESIAN_POINT('Origin',(-0.0585786437626908,-6.3,-15.2985786437627)) ;
#123257=CARTESIAN_POINT('Origin',(-0.0585786437626908,-6.3,-15.2985786437627)) ;
#123258=CARTESIAN_POINT('Origin',(-0.1,-6.3,-15.1814213562373)) ;
#123259=CARTESIAN_POINT('Origin',(-0.0585786437626908,-6.3,-15.1814213562373)) ;
#123260=CARTESIAN_POINT('Origin',(-0.0585786437626908,-6.3,-14.84)) ;
#123261=CARTESIAN_POINT('Origin',(-0.0585786437626908,-6.3,-15.1814213562373)) ;
#123262=CARTESIAN_POINT('Origin',(-0.0861928812542299,-6.27238576250846,
-15.3261928812542)) ;
#123263=CARTESIAN_POINT('Origin',(-0.300000000000001,-6.05857864376269,
-15.54)) ;
#123264=CARTESIAN_POINT('Origin',(-0.0585786437626908,-6.3,-15.1814213562373)) ;
#123265=CARTESIAN_POINT('Origin',(-0.0585786437626914,-6.3,-15.1814213562373)) ;
#123266=CARTESIAN_POINT('Origin',(-0.3,-6.05857864376269,-14.84)) ;
#123267=CARTESIAN_POINT('Origin',(-0.3,-6.05857864376269,-15.54)) ;
#123268=CARTESIAN_POINT('Origin',(-0.3,-6.05857864376269,-14.94)) ;
#123269=CARTESIAN_POINT('Origin',(-0.352859547920897,-6.00571909584179,
-14.8871404520791)) ;
#123270=CARTESIAN_POINT('Origin',(-0.3,-6.05857864376269,-14.94)) ;
#123271=CARTESIAN_POINT('Origin',(7.07238576250846,-0.11380711874577,-15.1261928812542)) ;
#123272=CARTESIAN_POINT('Origin',(6.65857864376269,0.300000000000003,-15.54)) ;
#123273=CARTESIAN_POINT('Origin',(6.9,0.0585786437626913,-15.2985786437627)) ;
#123274=CARTESIAN_POINT('Origin',(6.65857864376269,0.300000000000001,-14.84)) ;
#123275=CARTESIAN_POINT('Origin',(6.65857864376269,0.300000000000001,-15.54)) ;
#123276=CARTESIAN_POINT('Origin',(6.65857864376269,0.300000000000001,-14.94)) ;
#123277=CARTESIAN_POINT('Origin',(6.9,0.0585786437626909,-15.2985786437627)) ;
#123278=CARTESIAN_POINT('Origin',(6.9,0.0585786437626909,-15.2985786437627)) ;
#123279=CARTESIAN_POINT('Origin',(6.9,0.0585786437626909,-15.2985786437627)) ;
#123280=CARTESIAN_POINT('Origin',(6.80571909584179,0.152859547920897,-15.0871404520791)) ;
#123281=CARTESIAN_POINT('Origin',(6.65857864376269,0.300000000000001,-14.94)) ;
#123282=CARTESIAN_POINT('Origin',(6.9,0.0585786437626909,-15.1814213562373)) ;
#123283=CARTESIAN_POINT('Origin',(6.9,0.0585786437626909,-14.84)) ;
#123284=CARTESIAN_POINT('Origin',(6.9,0.0585786437626909,-15.1814213562373)) ;
#123285=CARTESIAN_POINT('Origin',(6.9,-0.1,-15.2985786437627)) ;
#123286=CARTESIAN_POINT('Origin',(6.9,-0.058578643762691,-15.2985786437627)) ;
#123287=CARTESIAN_POINT('Origin',(6.9,0.0585786437626909,-15.1814213562373)) ;
#123288=CARTESIAN_POINT('Origin',(6.9,0.0585786437626917,-15.1814213562373)) ;
#123289=CARTESIAN_POINT('Origin',(6.9,-0.0585786437626909,-15.2985786437627)) ;
#123290=CARTESIAN_POINT('Origin',(6.9,-0.058578643762691,-15.2985786437627)) ;
#123291=CARTESIAN_POINT('Origin',(6.9,-0.0585786437626909,-15.2985786437627)) ;
#123292=CARTESIAN_POINT('Origin',(6.9,-0.399999999999999,-15.1814213562373)) ;
#123293=CARTESIAN_POINT('Origin',(6.9,-0.0585786437626909,-15.1814213562373)) ;
#123294=CARTESIAN_POINT('Origin',(6.9,-0.0585786437626909,-14.84)) ;
#123295=CARTESIAN_POINT('Origin',(6.9,-0.0585786437626909,-15.1814213562373)) ;
#123296=CARTESIAN_POINT('Origin',(6.87238576250846,-0.0861928812542304,
-15.3261928812542)) ;
#123297=CARTESIAN_POINT('Origin',(6.65857864376269,-0.300000000000002,-15.54)) ;
#123298=CARTESIAN_POINT('Origin',(6.9,-0.058578643762691,-15.1814213562373)) ;
#123299=CARTESIAN_POINT('Origin',(6.9,-0.0585786437626915,-15.1814213562373)) ;
#123300=CARTESIAN_POINT('Origin',(6.65857864376269,-0.300000000000001,-14.84)) ;
#123301=CARTESIAN_POINT('Origin',(6.65857864376269,-0.300000000000001,-15.54)) ;
#123302=CARTESIAN_POINT('Origin',(6.65857864376269,-0.300000000000001,-14.94)) ;
#123303=CARTESIAN_POINT('Origin',(6.60571909584179,-0.352859547920897,-14.8871404520791)) ;
#123304=CARTESIAN_POINT('Origin',(6.65857864376269,-0.300000000000001,-14.94)) ;
#123305=CARTESIAN_POINT('Origin',(-0.113807118745769,-6.47238576250846,
-18.9361928812542)) ;
#123306=CARTESIAN_POINT('Origin',(0.300000000000001,-6.05857864376269,-19.35)) ;
#123307=CARTESIAN_POINT('Origin',(0.058578643762692,-6.3,-19.1085786437627)) ;
#123308=CARTESIAN_POINT('Origin',(0.3,-6.05857864376269,-18.65)) ;
#123309=CARTESIAN_POINT('Origin',(0.3,-6.05857864376269,-19.35)) ;
#123310=CARTESIAN_POINT('Origin',(0.3,-6.05857864376269,-18.75)) ;
#123311=CARTESIAN_POINT('Origin',(0.0585786437626908,-6.3,-19.1085786437627)) ;
#123312=CARTESIAN_POINT('Origin',(0.0585786437626908,-6.3,-19.1085786437627)) ;
#123313=CARTESIAN_POINT('Origin',(0.0585786437626908,-6.3,-19.1085786437627)) ;
#123314=CARTESIAN_POINT('Origin',(0.152859547920896,-6.2057190958418,-18.8971404520791)) ;
#123315=CARTESIAN_POINT('Origin',(0.299999999999995,-6.0585786437627,-18.75)) ;
#123316=CARTESIAN_POINT('Origin',(0.0585786437626908,-6.3,-18.9914213562373)) ;
#123317=CARTESIAN_POINT('Origin',(0.0585786437626908,-6.3,-18.65)) ;
#123318=CARTESIAN_POINT('Origin',(0.0585786437626908,-6.3,-18.9914213562373)) ;
#123319=CARTESIAN_POINT('Origin',(0.4,-6.3,-19.1085786437627)) ;
#123320=CARTESIAN_POINT('Origin',(-0.0585786437626899,-6.3,-19.1085786437627)) ;
#123321=CARTESIAN_POINT('Origin',(0.0585786437626908,-6.3,-18.9914213562373)) ;
#123322=CARTESIAN_POINT('Origin',(0.0585786437626916,-6.3,-18.9914213562373)) ;
#123323=CARTESIAN_POINT('Origin',(-0.0585786437626908,-6.3,-19.1085786437627)) ;
#123324=CARTESIAN_POINT('Origin',(-0.0585786437626905,-6.3,-19.1085786437627)) ;
#123325=CARTESIAN_POINT('Origin',(-0.0585786437626908,-6.3,-19.1085786437627)) ;
#123326=CARTESIAN_POINT('Origin',(-0.1,-6.3,-18.9914213562373)) ;
#123327=CARTESIAN_POINT('Origin',(-0.0585786437626908,-6.3,-18.9914213562373)) ;
#123328=CARTESIAN_POINT('Origin',(-0.0585786437626908,-6.3,-18.65)) ;
#123329=CARTESIAN_POINT('Origin',(-0.0585786437626908,-6.3,-18.9914213562373)) ;
#123330=CARTESIAN_POINT('Origin',(-0.0861928812542299,-6.27238576250846,
-19.1361928812542)) ;
#123331=CARTESIAN_POINT('Origin',(-0.299999999999999,-6.05857864376269,
-19.35)) ;
#123332=CARTESIAN_POINT('Origin',(-0.0585786437626908,-6.3,-18.9914213562373)) ;
#123333=CARTESIAN_POINT('Origin',(-0.0585786437626909,-6.3,-18.9914213562373)) ;
#123334=CARTESIAN_POINT('Origin',(-0.3,-6.05857864376269,-18.65)) ;
#123335=CARTESIAN_POINT('Origin',(-0.3,-6.05857864376269,-19.35)) ;
#123336=CARTESIAN_POINT('Origin',(-0.3,-6.05857864376269,-18.75)) ;
#123337=CARTESIAN_POINT('Origin',(-0.352859547920895,-6.00571909584179,
-18.6971404520791)) ;
#123338=CARTESIAN_POINT('Origin',(-0.299999999999997,-6.05857864376269,
-18.75)) ;
#123339=CARTESIAN_POINT('Origin',(7.07238576250846,-0.11380711874577,-18.9361928812542)) ;
#123340=CARTESIAN_POINT('Origin',(6.65857864376269,0.299999999999999,-19.35)) ;
#123341=CARTESIAN_POINT('Origin',(6.9,0.0585786437626903,-19.1085786437627)) ;
#123342=CARTESIAN_POINT('Origin',(6.65857864376269,0.300000000000001,-18.65)) ;
#123343=CARTESIAN_POINT('Origin',(6.65857864376269,0.300000000000001,-19.35)) ;
#123344=CARTESIAN_POINT('Origin',(6.65857864376269,0.300000000000001,-18.75)) ;
#123345=CARTESIAN_POINT('Origin',(6.9,0.0585786437626909,-19.1085786437627)) ;
#123346=CARTESIAN_POINT('Origin',(6.9,0.0585786437626909,-19.1085786437627)) ;
#123347=CARTESIAN_POINT('Origin',(6.9,0.0585786437626909,-19.1085786437627)) ;
#123348=CARTESIAN_POINT('Origin',(6.8057190958418,0.152859547920896,-18.8971404520791)) ;
#123349=CARTESIAN_POINT('Origin',(6.6585786437627,0.299999999999996,-18.75)) ;
#123350=CARTESIAN_POINT('Origin',(6.9,0.0585786437626908,-18.9914213562373)) ;
#123351=CARTESIAN_POINT('Origin',(6.9,0.0585786437626909,-18.65)) ;
#123352=CARTESIAN_POINT('Origin',(6.9,0.0585786437626909,-18.9914213562373)) ;
#123353=CARTESIAN_POINT('Origin',(6.9,-0.1,-19.1085786437627)) ;
#123354=CARTESIAN_POINT('Origin',(6.9,-0.0585786437626902,-19.1085786437627)) ;
#123355=CARTESIAN_POINT('Origin',(6.9,0.0585786437626909,-18.9914213562373)) ;
#123356=CARTESIAN_POINT('Origin',(6.9,0.058578643762691,-18.9914213562373)) ;
#123357=CARTESIAN_POINT('Origin',(6.9,-0.0585786437626909,-19.1085786437627)) ;
#123358=CARTESIAN_POINT('Origin',(6.9,-0.0585786437626907,-19.1085786437627)) ;
#123359=CARTESIAN_POINT('Origin',(6.9,-0.0585786437626909,-19.1085786437627)) ;
#123360=CARTESIAN_POINT('Origin',(6.9,-0.399999999999999,-18.9914213562373)) ;
#123361=CARTESIAN_POINT('Origin',(6.9,-0.0585786437626909,-18.9914213562373)) ;
#123362=CARTESIAN_POINT('Origin',(6.9,-0.0585786437626909,-18.65)) ;
#123363=CARTESIAN_POINT('Origin',(6.9,-0.058578643762691,-18.9914213562373)) ;
#123364=CARTESIAN_POINT('Origin',(6.87238576250846,-0.0861928812542304,
-19.1361928812542)) ;
#123365=CARTESIAN_POINT('Origin',(6.65857864376269,-0.3,-19.35)) ;
#123366=CARTESIAN_POINT('Origin',(6.9,-0.0585786437626909,-18.9914213562373)) ;
#123367=CARTESIAN_POINT('Origin',(6.9,-0.0585786437626907,-18.9914213562373)) ;
#123368=CARTESIAN_POINT('Origin',(6.65857864376269,-0.300000000000001,-18.65)) ;
#123369=CARTESIAN_POINT('Origin',(6.65857864376269,-0.300000000000001,-19.35)) ;
#123370=CARTESIAN_POINT('Origin',(6.65857864376269,-0.300000000000001,-18.75)) ;
#123371=CARTESIAN_POINT('Origin',(6.6057190958418,-0.352859547920896,-18.6971404520791)) ;
#123372=CARTESIAN_POINT('Origin',(6.65857864376269,-0.299999999999998,-18.75)) ;
#123373=CARTESIAN_POINT('Origin',(-0.113807118745769,-6.47238576250846,
-22.7461928812542)) ;
#123374=CARTESIAN_POINT('Origin',(0.300000000000001,-6.05857864376269,-23.16)) ;
#123375=CARTESIAN_POINT('Origin',(0.058578643762692,-6.3,-22.9185786437627)) ;
#123376=CARTESIAN_POINT('Origin',(0.3,-6.05857864376269,-22.46)) ;
#123377=CARTESIAN_POINT('Origin',(0.3,-6.05857864376269,-23.16)) ;
#123378=CARTESIAN_POINT('Origin',(0.3,-6.05857864376269,-22.56)) ;
#123379=CARTESIAN_POINT('Origin',(0.0585786437626908,-6.3,-22.9185786437627)) ;
#123380=CARTESIAN_POINT('Origin',(0.0585786437626908,-6.3,-22.9185786437627)) ;
#123381=CARTESIAN_POINT('Origin',(0.0585786437626908,-6.3,-22.9185786437627)) ;
#123382=CARTESIAN_POINT('Origin',(0.152859547920896,-6.2057190958418,-22.7071404520791)) ;
#123383=CARTESIAN_POINT('Origin',(0.299999999999995,-6.0585786437627,-22.56)) ;
#123384=CARTESIAN_POINT('Origin',(0.0585786437626908,-6.3,-22.8014213562373)) ;
#123385=CARTESIAN_POINT('Origin',(0.0585786437626908,-6.3,-22.46)) ;
#123386=CARTESIAN_POINT('Origin',(0.0585786437626908,-6.3,-22.8014213562373)) ;
#123387=CARTESIAN_POINT('Origin',(0.4,-6.3,-22.9185786437627)) ;
#123388=CARTESIAN_POINT('Origin',(-0.0585786437626899,-6.3,-22.9185786437627)) ;
#123389=CARTESIAN_POINT('Origin',(0.0585786437626908,-6.3,-22.8014213562373)) ;
#123390=CARTESIAN_POINT('Origin',(0.0585786437626916,-6.3,-22.8014213562373)) ;
#123391=CARTESIAN_POINT('Origin',(-0.0585786437626908,-6.3,-22.9185786437627)) ;
#123392=CARTESIAN_POINT('Origin',(-0.0585786437626905,-6.3,-22.9185786437627)) ;
#123393=CARTESIAN_POINT('Origin',(-0.0585786437626908,-6.3,-22.9185786437627)) ;
#123394=CARTESIAN_POINT('Origin',(-0.1,-6.3,-22.8014213562373)) ;
#123395=CARTESIAN_POINT('Origin',(-0.0585786437626908,-6.3,-22.8014213562373)) ;
#123396=CARTESIAN_POINT('Origin',(-0.0585786437626908,-6.3,-22.46)) ;
#123397=CARTESIAN_POINT('Origin',(-0.0585786437626908,-6.3,-22.8014213562373)) ;
#123398=CARTESIAN_POINT('Origin',(-0.0861928812542299,-6.27238576250846,
-22.9461928812542)) ;
#123399=CARTESIAN_POINT('Origin',(-0.299999999999999,-6.05857864376269,
-23.16)) ;
#123400=CARTESIAN_POINT('Origin',(-0.0585786437626908,-6.3,-22.8014213562373)) ;
#123401=CARTESIAN_POINT('Origin',(-0.0585786437626909,-6.3,-22.8014213562373)) ;
#123402=CARTESIAN_POINT('Origin',(-0.3,-6.05857864376269,-22.46)) ;
#123403=CARTESIAN_POINT('Origin',(-0.3,-6.05857864376269,-23.16)) ;
#123404=CARTESIAN_POINT('Origin',(-0.3,-6.05857864376269,-22.56)) ;
#123405=CARTESIAN_POINT('Origin',(-0.352859547920895,-6.00571909584179,
-22.5071404520791)) ;
#123406=CARTESIAN_POINT('Origin',(-0.299999999999997,-6.05857864376269,
-22.56)) ;
#123407=CARTESIAN_POINT('Origin',(7.07238576250846,-0.11380711874577,-22.7461928812542)) ;
#123408=CARTESIAN_POINT('Origin',(6.65857864376269,0.299999999999999,-23.16)) ;
#123409=CARTESIAN_POINT('Origin',(6.9,0.0585786437626903,-22.9185786437627)) ;
#123410=CARTESIAN_POINT('Origin',(6.65857864376269,0.300000000000001,-22.46)) ;
#123411=CARTESIAN_POINT('Origin',(6.65857864376269,0.300000000000001,-23.16)) ;
#123412=CARTESIAN_POINT('Origin',(6.65857864376269,0.300000000000001,-22.56)) ;
#123413=CARTESIAN_POINT('Origin',(6.9,0.0585786437626909,-22.9185786437627)) ;
#123414=CARTESIAN_POINT('Origin',(6.9,0.0585786437626909,-22.9185786437627)) ;
#123415=CARTESIAN_POINT('Origin',(6.9,0.0585786437626909,-22.9185786437627)) ;
#123416=CARTESIAN_POINT('Origin',(6.8057190958418,0.152859547920896,-22.7071404520791)) ;
#123417=CARTESIAN_POINT('Origin',(6.6585786437627,0.299999999999996,-22.56)) ;
#123418=CARTESIAN_POINT('Origin',(6.9,0.0585786437626908,-22.8014213562373)) ;
#123419=CARTESIAN_POINT('Origin',(6.9,0.0585786437626909,-22.46)) ;
#123420=CARTESIAN_POINT('Origin',(6.9,0.0585786437626909,-22.8014213562373)) ;
#123421=CARTESIAN_POINT('Origin',(6.9,-0.1,-22.9185786437627)) ;
#123422=CARTESIAN_POINT('Origin',(6.9,-0.0585786437626902,-22.9185786437627)) ;
#123423=CARTESIAN_POINT('Origin',(6.9,0.0585786437626909,-22.8014213562373)) ;
#123424=CARTESIAN_POINT('Origin',(6.9,0.058578643762691,-22.8014213562373)) ;
#123425=CARTESIAN_POINT('Origin',(6.9,-0.0585786437626909,-22.9185786437627)) ;
#123426=CARTESIAN_POINT('Origin',(6.9,-0.0585786437626907,-22.9185786437627)) ;
#123427=CARTESIAN_POINT('Origin',(6.9,-0.0585786437626909,-22.9185786437627)) ;
#123428=CARTESIAN_POINT('Origin',(6.9,-0.399999999999999,-22.8014213562373)) ;
#123429=CARTESIAN_POINT('Origin',(6.9,-0.0585786437626909,-22.8014213562373)) ;
#123430=CARTESIAN_POINT('Origin',(6.9,-0.0585786437626909,-22.46)) ;
#123431=CARTESIAN_POINT('Origin',(6.9,-0.058578643762691,-22.8014213562373)) ;
#123432=CARTESIAN_POINT('Origin',(6.87238576250846,-0.0861928812542304,
-22.9461928812542)) ;
#123433=CARTESIAN_POINT('Origin',(6.65857864376269,-0.3,-23.16)) ;
#123434=CARTESIAN_POINT('Origin',(6.9,-0.0585786437626909,-22.8014213562373)) ;
#123435=CARTESIAN_POINT('Origin',(6.9,-0.0585786437626907,-22.8014213562373)) ;
#123436=CARTESIAN_POINT('Origin',(6.65857864376269,-0.300000000000001,-22.46)) ;
#123437=CARTESIAN_POINT('Origin',(6.65857864376269,-0.300000000000001,-23.16)) ;
#123438=CARTESIAN_POINT('Origin',(6.65857864376269,-0.300000000000001,-22.56)) ;
#123439=CARTESIAN_POINT('Origin',(6.6057190958418,-0.352859547920896,-22.5071404520791)) ;
#123440=CARTESIAN_POINT('Origin',(6.65857864376269,-0.299999999999998,-22.56)) ;
#123441=CARTESIAN_POINT('Origin',(-0.113807118745769,-6.47238576250846,
-26.5561928812542)) ;
#123442=CARTESIAN_POINT('Origin',(0.300000000000001,-6.05857864376269,-26.97)) ;
#123443=CARTESIAN_POINT('Origin',(0.058578643762692,-6.3,-26.7285786437627)) ;
#123444=CARTESIAN_POINT('Origin',(0.3,-6.05857864376269,-26.27)) ;
#123445=CARTESIAN_POINT('Origin',(0.3,-6.05857864376269,-26.97)) ;
#123446=CARTESIAN_POINT('Origin',(0.3,-6.05857864376269,-26.37)) ;
#123447=CARTESIAN_POINT('Origin',(0.0585786437626908,-6.3,-26.7285786437627)) ;
#123448=CARTESIAN_POINT('Origin',(0.0585786437626908,-6.3,-26.7285786437627)) ;
#123449=CARTESIAN_POINT('Origin',(0.0585786437626908,-6.3,-26.7285786437627)) ;
#123450=CARTESIAN_POINT('Origin',(0.152859547920896,-6.2057190958418,-26.5171404520791)) ;
#123451=CARTESIAN_POINT('Origin',(0.299999999999995,-6.0585786437627,-26.37)) ;
#123452=CARTESIAN_POINT('Origin',(0.0585786437626908,-6.3,-26.6114213562373)) ;
#123453=CARTESIAN_POINT('Origin',(0.0585786437626908,-6.3,-26.27)) ;
#123454=CARTESIAN_POINT('Origin',(0.0585786437626908,-6.3,-26.6114213562373)) ;
#123455=CARTESIAN_POINT('Origin',(0.4,-6.3,-26.7285786437627)) ;
#123456=CARTESIAN_POINT('Origin',(-0.0585786437626899,-6.3,-26.7285786437627)) ;
#123457=CARTESIAN_POINT('Origin',(0.0585786437626908,-6.3,-26.6114213562373)) ;
#123458=CARTESIAN_POINT('Origin',(0.0585786437626916,-6.3,-26.6114213562373)) ;
#123459=CARTESIAN_POINT('Origin',(-0.0585786437626908,-6.3,-26.7285786437627)) ;
#123460=CARTESIAN_POINT('Origin',(-0.0585786437626905,-6.3,-26.7285786437627)) ;
#123461=CARTESIAN_POINT('Origin',(-0.0585786437626908,-6.3,-26.7285786437627)) ;
#123462=CARTESIAN_POINT('Origin',(-0.1,-6.3,-26.6114213562373)) ;
#123463=CARTESIAN_POINT('Origin',(-0.0585786437626908,-6.3,-26.6114213562373)) ;
#123464=CARTESIAN_POINT('Origin',(-0.0585786437626908,-6.3,-26.27)) ;
#123465=CARTESIAN_POINT('Origin',(-0.0585786437626908,-6.3,-26.6114213562373)) ;
#123466=CARTESIAN_POINT('Origin',(-0.0861928812542299,-6.27238576250846,
-26.7561928812542)) ;
#123467=CARTESIAN_POINT('Origin',(-0.299999999999999,-6.05857864376269,
-26.97)) ;
#123468=CARTESIAN_POINT('Origin',(-0.0585786437626908,-6.3,-26.6114213562373)) ;
#123469=CARTESIAN_POINT('Origin',(-0.0585786437626909,-6.3,-26.6114213562373)) ;
#123470=CARTESIAN_POINT('Origin',(-0.3,-6.05857864376269,-26.27)) ;
#123471=CARTESIAN_POINT('Origin',(-0.3,-6.05857864376269,-26.97)) ;
#123472=CARTESIAN_POINT('Origin',(-0.3,-6.05857864376269,-26.37)) ;
#123473=CARTESIAN_POINT('Origin',(-0.352859547920895,-6.00571909584179,
-26.3171404520791)) ;
#123474=CARTESIAN_POINT('Origin',(-0.299999999999997,-6.05857864376269,
-26.37)) ;
#123475=CARTESIAN_POINT('Origin',(7.07238576250846,-0.11380711874577,-26.5561928812542)) ;
#123476=CARTESIAN_POINT('Origin',(6.65857864376269,0.299999999999999,-26.97)) ;
#123477=CARTESIAN_POINT('Origin',(6.9,0.0585786437626903,-26.7285786437627)) ;
#123478=CARTESIAN_POINT('Origin',(6.65857864376269,0.300000000000001,-26.27)) ;
#123479=CARTESIAN_POINT('Origin',(6.65857864376269,0.300000000000001,-26.97)) ;
#123480=CARTESIAN_POINT('Origin',(6.65857864376269,0.300000000000001,-26.37)) ;
#123481=CARTESIAN_POINT('Origin',(6.9,0.0585786437626909,-26.7285786437627)) ;
#123482=CARTESIAN_POINT('Origin',(6.9,0.0585786437626909,-26.7285786437627)) ;
#123483=CARTESIAN_POINT('Origin',(6.9,0.0585786437626909,-26.7285786437627)) ;
#123484=CARTESIAN_POINT('Origin',(6.8057190958418,0.152859547920896,-26.5171404520791)) ;
#123485=CARTESIAN_POINT('Origin',(6.6585786437627,0.299999999999996,-26.37)) ;
#123486=CARTESIAN_POINT('Origin',(6.9,0.0585786437626908,-26.6114213562373)) ;
#123487=CARTESIAN_POINT('Origin',(6.9,0.0585786437626909,-26.27)) ;
#123488=CARTESIAN_POINT('Origin',(6.9,0.0585786437626909,-26.6114213562373)) ;
#123489=CARTESIAN_POINT('Origin',(6.9,-0.1,-26.7285786437627)) ;
#123490=CARTESIAN_POINT('Origin',(6.9,-0.0585786437626902,-26.7285786437627)) ;
#123491=CARTESIAN_POINT('Origin',(6.9,0.0585786437626909,-26.6114213562373)) ;
#123492=CARTESIAN_POINT('Origin',(6.9,0.058578643762691,-26.6114213562373)) ;
#123493=CARTESIAN_POINT('Origin',(6.9,-0.0585786437626909,-26.7285786437627)) ;
#123494=CARTESIAN_POINT('Origin',(6.9,-0.0585786437626907,-26.7285786437627)) ;
#123495=CARTESIAN_POINT('Origin',(6.9,-0.0585786437626909,-26.7285786437627)) ;
#123496=CARTESIAN_POINT('Origin',(6.9,-0.399999999999999,-26.6114213562373)) ;
#123497=CARTESIAN_POINT('Origin',(6.9,-0.0585786437626909,-26.6114213562373)) ;
#123498=CARTESIAN_POINT('Origin',(6.9,-0.0585786437626909,-26.27)) ;
#123499=CARTESIAN_POINT('Origin',(6.9,-0.058578643762691,-26.6114213562373)) ;
#123500=CARTESIAN_POINT('Origin',(6.87238576250846,-0.0861928812542304,
-26.7561928812542)) ;
#123501=CARTESIAN_POINT('Origin',(6.65857864376269,-0.3,-26.97)) ;
#123502=CARTESIAN_POINT('Origin',(6.9,-0.0585786437626909,-26.6114213562373)) ;
#123503=CARTESIAN_POINT('Origin',(6.9,-0.0585786437626907,-26.6114213562373)) ;
#123504=CARTESIAN_POINT('Origin',(6.65857864376269,-0.300000000000001,-26.27)) ;
#123505=CARTESIAN_POINT('Origin',(6.65857864376269,-0.300000000000001,-26.97)) ;
#123506=CARTESIAN_POINT('Origin',(6.65857864376269,-0.300000000000001,-26.37)) ;
#123507=CARTESIAN_POINT('Origin',(6.6057190958418,-0.352859547920896,-26.3171404520791)) ;
#123508=CARTESIAN_POINT('Origin',(6.65857864376269,-0.299999999999998,-26.37)) ;
#123509=CARTESIAN_POINT('Origin',(-0.113807118745769,-6.47238576250846,
-30.3661928812542)) ;
#123510=CARTESIAN_POINT('Origin',(0.300000000000001,-6.05857864376269,-30.78)) ;
#123511=CARTESIAN_POINT('Origin',(0.058578643762692,-6.3,-30.5385786437627)) ;
#123512=CARTESIAN_POINT('Origin',(0.3,-6.05857864376269,-30.08)) ;
#123513=CARTESIAN_POINT('Origin',(0.3,-6.05857864376269,-30.78)) ;
#123514=CARTESIAN_POINT('Origin',(0.3,-6.05857864376269,-30.18)) ;
#123515=CARTESIAN_POINT('Origin',(0.0585786437626908,-6.3,-30.5385786437627)) ;
#123516=CARTESIAN_POINT('Origin',(0.0585786437626908,-6.3,-30.5385786437627)) ;
#123517=CARTESIAN_POINT('Origin',(0.0585786437626908,-6.3,-30.5385786437627)) ;
#123518=CARTESIAN_POINT('Origin',(0.152859547920896,-6.2057190958418,-30.3271404520791)) ;
#123519=CARTESIAN_POINT('Origin',(0.299999999999995,-6.0585786437627,-30.18)) ;
#123520=CARTESIAN_POINT('Origin',(0.0585786437626908,-6.3,-30.4214213562373)) ;
#123521=CARTESIAN_POINT('Origin',(0.0585786437626908,-6.3,-30.08)) ;
#123522=CARTESIAN_POINT('Origin',(0.0585786437626908,-6.3,-30.4214213562373)) ;
#123523=CARTESIAN_POINT('Origin',(0.4,-6.3,-30.5385786437627)) ;
#123524=CARTESIAN_POINT('Origin',(-0.0585786437626899,-6.3,-30.5385786437627)) ;
#123525=CARTESIAN_POINT('Origin',(0.0585786437626908,-6.3,-30.4214213562373)) ;
#123526=CARTESIAN_POINT('Origin',(0.0585786437626916,-6.3,-30.4214213562373)) ;
#123527=CARTESIAN_POINT('Origin',(-0.0585786437626908,-6.3,-30.5385786437627)) ;
#123528=CARTESIAN_POINT('Origin',(-0.0585786437626905,-6.3,-30.5385786437627)) ;
#123529=CARTESIAN_POINT('Origin',(-0.0585786437626908,-6.3,-30.5385786437627)) ;
#123530=CARTESIAN_POINT('Origin',(-0.1,-6.3,-30.4214213562373)) ;
#123531=CARTESIAN_POINT('Origin',(-0.0585786437626908,-6.3,-30.4214213562373)) ;
#123532=CARTESIAN_POINT('Origin',(-0.0585786437626908,-6.3,-30.08)) ;
#123533=CARTESIAN_POINT('Origin',(-0.0585786437626908,-6.3,-30.4214213562373)) ;
#123534=CARTESIAN_POINT('Origin',(-0.0861928812542299,-6.27238576250846,
-30.5661928812542)) ;
#123535=CARTESIAN_POINT('Origin',(-0.299999999999999,-6.05857864376269,
-30.78)) ;
#123536=CARTESIAN_POINT('Origin',(-0.0585786437626908,-6.3,-30.4214213562373)) ;
#123537=CARTESIAN_POINT('Origin',(-0.0585786437626909,-6.3,-30.4214213562373)) ;
#123538=CARTESIAN_POINT('Origin',(-0.3,-6.05857864376269,-30.08)) ;
#123539=CARTESIAN_POINT('Origin',(-0.3,-6.05857864376269,-30.78)) ;
#123540=CARTESIAN_POINT('Origin',(-0.3,-6.05857864376269,-30.18)) ;
#123541=CARTESIAN_POINT('Origin',(-0.352859547920895,-6.00571909584179,
-30.1271404520791)) ;
#123542=CARTESIAN_POINT('Origin',(-0.299999999999997,-6.05857864376269,
-30.18)) ;
#123543=CARTESIAN_POINT('Origin',(7.07238576250846,-0.11380711874577,-30.3661928812542)) ;
#123544=CARTESIAN_POINT('Origin',(6.65857864376269,0.299999999999999,-30.78)) ;
#123545=CARTESIAN_POINT('Origin',(6.9,0.0585786437626903,-30.5385786437627)) ;
#123546=CARTESIAN_POINT('Origin',(6.65857864376269,0.300000000000001,-30.08)) ;
#123547=CARTESIAN_POINT('Origin',(6.65857864376269,0.300000000000001,-30.78)) ;
#123548=CARTESIAN_POINT('Origin',(6.65857864376269,0.300000000000001,-30.18)) ;
#123549=CARTESIAN_POINT('Origin',(6.9,0.0585786437626909,-30.5385786437627)) ;
#123550=CARTESIAN_POINT('Origin',(6.9,0.0585786437626909,-30.5385786437627)) ;
#123551=CARTESIAN_POINT('Origin',(6.9,0.0585786437626909,-30.5385786437627)) ;
#123552=CARTESIAN_POINT('Origin',(6.8057190958418,0.152859547920896,-30.3271404520791)) ;
#123553=CARTESIAN_POINT('Origin',(6.6585786437627,0.299999999999996,-30.18)) ;
#123554=CARTESIAN_POINT('Origin',(6.9,0.0585786437626908,-30.4214213562373)) ;
#123555=CARTESIAN_POINT('Origin',(6.9,0.0585786437626909,-30.08)) ;
#123556=CARTESIAN_POINT('Origin',(6.9,0.0585786437626909,-30.4214213562373)) ;
#123557=CARTESIAN_POINT('Origin',(6.9,-0.1,-30.5385786437627)) ;
#123558=CARTESIAN_POINT('Origin',(6.9,-0.0585786437626902,-30.5385786437627)) ;
#123559=CARTESIAN_POINT('Origin',(6.9,0.0585786437626909,-30.4214213562373)) ;
#123560=CARTESIAN_POINT('Origin',(6.9,0.058578643762691,-30.4214213562373)) ;
#123561=CARTESIAN_POINT('Origin',(6.9,-0.0585786437626909,-30.5385786437627)) ;
#123562=CARTESIAN_POINT('Origin',(6.9,-0.0585786437626907,-30.5385786437627)) ;
#123563=CARTESIAN_POINT('Origin',(6.9,-0.0585786437626909,-30.5385786437627)) ;
#123564=CARTESIAN_POINT('Origin',(6.9,-0.399999999999999,-30.4214213562373)) ;
#123565=CARTESIAN_POINT('Origin',(6.9,-0.0585786437626909,-30.4214213562373)) ;
#123566=CARTESIAN_POINT('Origin',(6.9,-0.0585786437626909,-30.08)) ;
#123567=CARTESIAN_POINT('Origin',(6.9,-0.058578643762691,-30.4214213562373)) ;
#123568=CARTESIAN_POINT('Origin',(6.87238576250846,-0.0861928812542304,
-30.5661928812542)) ;
#123569=CARTESIAN_POINT('Origin',(6.65857864376269,-0.3,-30.78)) ;
#123570=CARTESIAN_POINT('Origin',(6.9,-0.0585786437626909,-30.4214213562373)) ;
#123571=CARTESIAN_POINT('Origin',(6.9,-0.0585786437626907,-30.4214213562373)) ;
#123572=CARTESIAN_POINT('Origin',(6.65857864376269,-0.300000000000001,-30.08)) ;
#123573=CARTESIAN_POINT('Origin',(6.65857864376269,-0.300000000000001,-30.78)) ;
#123574=CARTESIAN_POINT('Origin',(6.65857864376269,-0.300000000000001,-30.18)) ;
#123575=CARTESIAN_POINT('Origin',(6.6057190958418,-0.352859547920896,-30.1271404520791)) ;
#123576=CARTESIAN_POINT('Origin',(6.65857864376269,-0.299999999999998,-30.18)) ;
#123577=CARTESIAN_POINT('Origin',(-0.113807118745771,-6.47238576250846,
-34.1761928812542)) ;
#123578=CARTESIAN_POINT('Origin',(0.299999999999993,-6.0585786437627,-34.59)) ;
#123579=CARTESIAN_POINT('Origin',(0.0585786437626844,-6.3,-34.3485786437627)) ;
#123580=CARTESIAN_POINT('Origin',(0.3,-6.05857864376269,-33.89)) ;
#123581=CARTESIAN_POINT('Origin',(0.3,-6.05857864376269,-34.59)) ;
#123582=CARTESIAN_POINT('Origin',(0.3,-6.05857864376269,-33.99)) ;
#123583=CARTESIAN_POINT('Origin',(0.0585786437626887,-6.3,-34.3485786437627)) ;
#123584=CARTESIAN_POINT('Origin',(0.0585786437626908,-6.3,-34.3485786437627)) ;
#123585=CARTESIAN_POINT('Origin',(0.0585786437626908,-6.3,-34.3485786437627)) ;
#123586=CARTESIAN_POINT('Origin',(0.152859547920899,-6.20571909584179,-34.1371404520791)) ;
#123587=CARTESIAN_POINT('Origin',(0.300000000000006,-6.05857864376268,-33.99)) ;
#123588=CARTESIAN_POINT('Origin',(0.0585786437626911,-6.3,-34.2314213562373)) ;
#123589=CARTESIAN_POINT('Origin',(0.0585786437626908,-6.3,-33.89)) ;
#123590=CARTESIAN_POINT('Origin',(0.0585786437626908,-6.3,-34.2314213562373)) ;
#123591=CARTESIAN_POINT('Origin',(0.4,-6.3,-34.3485786437627)) ;
#123592=CARTESIAN_POINT('Origin',(-0.0585786437626895,-6.3,-34.3485786437627)) ;
#123593=CARTESIAN_POINT('Origin',(0.0585786437626903,-6.3,-34.2314213562373)) ;
#123594=CARTESIAN_POINT('Origin',(0.058578643762689,-6.3,-34.2314213562373)) ;
#123595=CARTESIAN_POINT('Origin',(-0.0585786437626902,-6.3,-34.3485786437627)) ;
#123596=CARTESIAN_POINT('Origin',(-0.0585786437626905,-6.3,-34.3485786437627)) ;
#123597=CARTESIAN_POINT('Origin',(-0.0585786437626908,-6.3,-34.3485786437627)) ;
#123598=CARTESIAN_POINT('Origin',(-0.1,-6.3,-34.2314213562373)) ;
#123599=CARTESIAN_POINT('Origin',(-0.0585786437626908,-6.3,-34.2314213562373)) ;
#123600=CARTESIAN_POINT('Origin',(-0.0585786437626908,-6.3,-33.89)) ;
#123601=CARTESIAN_POINT('Origin',(-0.0585786437626908,-6.3,-34.2314213562373)) ;
#123602=CARTESIAN_POINT('Origin',(-0.0861928812542287,-6.27238576250846,
-34.3761928812542)) ;
#123603=CARTESIAN_POINT('Origin',(-0.299999999999994,-6.0585786437627,-34.59)) ;
#123604=CARTESIAN_POINT('Origin',(-0.0585786437626908,-6.3,-34.2314213562373)) ;
#123605=CARTESIAN_POINT('Origin',(-0.0585786437626846,-6.3,-34.2314213562373)) ;
#123606=CARTESIAN_POINT('Origin',(-0.3,-6.05857864376269,-33.89)) ;
#123607=CARTESIAN_POINT('Origin',(-0.3,-6.05857864376269,-34.59)) ;
#123608=CARTESIAN_POINT('Origin',(-0.3,-6.05857864376269,-33.99)) ;
#123609=CARTESIAN_POINT('Origin',(-0.352859547920899,-6.00571909584179,
-33.9371404520791)) ;
#123610=CARTESIAN_POINT('Origin',(-0.3,-6.05857864376269,-33.99)) ;
#123611=CARTESIAN_POINT('Origin',(7.07238576250846,-0.113807118745771,-34.1761928812542)) ;
#123612=CARTESIAN_POINT('Origin',(6.6585786437627,0.299999999999994,-34.59)) ;
#123613=CARTESIAN_POINT('Origin',(6.9,0.0585786437626901,-34.3485786437627)) ;
#123614=CARTESIAN_POINT('Origin',(6.65857864376269,0.300000000000001,-33.89)) ;
#123615=CARTESIAN_POINT('Origin',(6.65857864376269,0.300000000000001,-34.59)) ;
#123616=CARTESIAN_POINT('Origin',(6.65857864376269,0.300000000000001,-33.99)) ;
#123617=CARTESIAN_POINT('Origin',(6.9,0.0585786437626906,-34.3485786437627)) ;
#123618=CARTESIAN_POINT('Origin',(6.9,0.0585786437626909,-34.3485786437627)) ;
#123619=CARTESIAN_POINT('Origin',(6.9,0.0585786437626909,-34.3485786437627)) ;
#123620=CARTESIAN_POINT('Origin',(6.80571909584179,0.1528595479209,-34.1371404520791)) ;
#123621=CARTESIAN_POINT('Origin',(6.65857864376268,0.300000000000007,-33.99)) ;
#123622=CARTESIAN_POINT('Origin',(6.9,0.0585786437626911,-34.2314213562373)) ;
#123623=CARTESIAN_POINT('Origin',(6.9,0.0585786437626909,-33.89)) ;
#123624=CARTESIAN_POINT('Origin',(6.9,0.0585786437626909,-34.2314213562373)) ;
#123625=CARTESIAN_POINT('Origin',(6.9,-0.1,-34.3485786437627)) ;
#123626=CARTESIAN_POINT('Origin',(6.9,-0.0585786437626952,-34.3485786437627)) ;
#123627=CARTESIAN_POINT('Origin',(6.9,0.0585786437626913,-34.2314213562373)) ;
#123628=CARTESIAN_POINT('Origin',(6.9,0.0585786437626919,-34.2314213562373)) ;
#123629=CARTESIAN_POINT('Origin',(6.9,-0.0585786437626923,-34.3485786437627)) ;
#123630=CARTESIAN_POINT('Origin',(6.9,-0.0585786437626907,-34.3485786437627)) ;
#123631=CARTESIAN_POINT('Origin',(6.9,-0.0585786437626909,-34.3485786437627)) ;
#123632=CARTESIAN_POINT('Origin',(6.9,-0.399999999999999,-34.2314213562373)) ;
#123633=CARTESIAN_POINT('Origin',(6.9,-0.0585786437626909,-34.2314213562373)) ;
#123634=CARTESIAN_POINT('Origin',(6.9,-0.0585786437626909,-33.89)) ;
#123635=CARTESIAN_POINT('Origin',(6.9,-0.058578643762691,-34.2314213562373)) ;
#123636=CARTESIAN_POINT('Origin',(6.87238576250846,-0.0861928812542292,
-34.3761928812542)) ;
#123637=CARTESIAN_POINT('Origin',(6.6585786437627,-0.299999999999995,-34.59)) ;
#123638=CARTESIAN_POINT('Origin',(6.9,-0.0585786437626886,-34.2314213562373)) ;
#123639=CARTESIAN_POINT('Origin',(6.9,-0.058578643762684,-34.2314213562373)) ;
#123640=CARTESIAN_POINT('Origin',(6.65857864376269,-0.300000000000001,-33.89)) ;
#123641=CARTESIAN_POINT('Origin',(6.65857864376269,-0.300000000000001,-34.59)) ;
#123642=CARTESIAN_POINT('Origin',(6.65857864376269,-0.300000000000001,-33.99)) ;
#123643=CARTESIAN_POINT('Origin',(6.60571909584179,-0.3528595479209,-33.9371404520791)) ;
#123644=CARTESIAN_POINT('Origin',(6.65857864376269,-0.300000000000001,-33.99)) ;
#123645=CARTESIAN_POINT('Origin',(0.6,-0.6,-4.11)) ;
#123646=CARTESIAN_POINT('Origin',(0.3,-0.6,-4.11)) ;
#123647=CARTESIAN_POINT('Origin',(0.3,-6.1,-4.11)) ;
#123648=CARTESIAN_POINT('Origin',(0.3,-6.05857864376269,-4.11)) ;
#123649=CARTESIAN_POINT('Origin',(0.3,-6.05857864376269,-4.11)) ;
#123650=CARTESIAN_POINT('Origin',(0.3,-6.05857864376269,-4.11)) ;
#123651=CARTESIAN_POINT('Origin',(0.4,-6.05857864376269,-4.11)) ;
#123652=CARTESIAN_POINT('Origin',(-0.300000000000001,-6.05857864376269,
-4.11)) ;
#123653=CARTESIAN_POINT('Origin',(-0.3,-6.05857864376269,-4.11)) ;
#123654=CARTESIAN_POINT('Origin',(-0.3,-6.05857864376269,-4.11)) ;
#123655=CARTESIAN_POINT('Origin',(-0.3,-0.600000000000001,-4.11)) ;
#123656=CARTESIAN_POINT('Origin',(-0.3,-0.600000000000001,-4.11)) ;
#123657=CARTESIAN_POINT('Origin',(0.6,-0.600000000000001,-4.11)) ;
#123658=CARTESIAN_POINT('Origin',(0.6,-0.600000000000001,-3.51)) ;
#123659=CARTESIAN_POINT('Origin',(-0.3,-0.600000000000001,-3.51)) ;
#123660=CARTESIAN_POINT('Origin',(-0.3,-0.600000000000001,-3.51)) ;
#123661=CARTESIAN_POINT('Origin',(-0.3,-6.05857864376269,-3.51)) ;
#123662=CARTESIAN_POINT('Origin',(-0.3,-6.05857864376269,-3.51)) ;
#123663=CARTESIAN_POINT('Origin',(-0.299999999999999,-6.05857864376269,
-3.51)) ;
#123664=CARTESIAN_POINT('Origin',(0.4,-6.05857864376269,-3.51)) ;
#123665=CARTESIAN_POINT('Origin',(0.299999999999999,-6.05857864376269,-3.51)) ;
#123666=CARTESIAN_POINT('Origin',(0.3,-6.05857864376269,-3.51)) ;
#123667=CARTESIAN_POINT('Origin',(0.3,-6.05857864376269,-3.51)) ;
#123668=CARTESIAN_POINT('Origin',(0.3,-0.600000000000001,-3.51)) ;
#123669=CARTESIAN_POINT('Origin',(0.3,-0.6,-3.51)) ;
#123670=CARTESIAN_POINT('Origin',(0.6,-0.6,-3.51)) ;
#123671=CARTESIAN_POINT('Origin',(6.7,0.300000000000001,-4.11)) ;
#123672=CARTESIAN_POINT('Origin',(6.65857864376269,0.300000000000001,-4.11)) ;
#123673=CARTESIAN_POINT('Origin',(6.65857864376269,0.300000000000001,-4.11)) ;
#123674=CARTESIAN_POINT('Origin',(6.65857864376269,0.300000000000001,-4.11)) ;
#123675=CARTESIAN_POINT('Origin',(6.65857864376269,-0.399999999999999,-4.11)) ;
#123676=CARTESIAN_POINT('Origin',(6.65857864376269,-0.300000000000001,-4.11)) ;
#123677=CARTESIAN_POINT('Origin',(6.65857864376269,-0.3,-4.11)) ;
#123678=CARTESIAN_POINT('Origin',(6.65857864376269,-0.300000000000001,-4.11)) ;
#123679=CARTESIAN_POINT('Origin',(0.6,-0.3,-4.11)) ;
#123680=CARTESIAN_POINT('Origin',(0.6,0.299999999999999,-3.51)) ;
#123681=CARTESIAN_POINT('Origin',(6.65857864376269,0.300000000000001,-3.51)) ;
#123682=CARTESIAN_POINT('Origin',(6.65857864376269,0.300000000000001,-3.51)) ;
#123683=CARTESIAN_POINT('Origin',(6.65857864376269,0.3,-3.51)) ;
#123684=CARTESIAN_POINT('Origin',(6.65857864376269,-0.399999999999999,-3.51)) ;
#123685=CARTESIAN_POINT('Origin',(6.65857864376269,-0.3,-3.51)) ;
#123686=CARTESIAN_POINT('Origin',(0.6,-0.3,-3.51)) ;
#123687=CARTESIAN_POINT('Origin',(6.65857864376269,-0.300000000000001,-3.51)) ;
#123688=CARTESIAN_POINT('Origin',(6.65857864376269,-0.300000000000001,-3.51)) ;
#123689=CARTESIAN_POINT('Origin',(0.6,-0.6,-7.92)) ;
#123690=CARTESIAN_POINT('Origin',(0.3,-0.6,-7.92)) ;
#123691=CARTESIAN_POINT('Origin',(0.3,-6.1,-7.92)) ;
#123692=CARTESIAN_POINT('Origin',(0.3,-6.05857864376269,-7.92)) ;
#123693=CARTESIAN_POINT('Origin',(0.3,-6.05857864376269,-7.92)) ;
#123694=CARTESIAN_POINT('Origin',(0.3,-6.05857864376269,-7.92)) ;
#123695=CARTESIAN_POINT('Origin',(0.4,-6.05857864376269,-7.92)) ;
#123696=CARTESIAN_POINT('Origin',(-0.299999999999999,-6.05857864376269,
-7.92)) ;
#123697=CARTESIAN_POINT('Origin',(-0.3,-6.05857864376269,-7.92)) ;
#123698=CARTESIAN_POINT('Origin',(-0.3,-6.05857864376269,-7.92)) ;
#123699=CARTESIAN_POINT('Origin',(-0.3,-0.600000000000001,-7.92)) ;
#123700=CARTESIAN_POINT('Origin',(-0.3,-0.600000000000001,-7.92)) ;
#123701=CARTESIAN_POINT('Origin',(0.6,-0.600000000000001,-7.92)) ;
#123702=CARTESIAN_POINT('Origin',(0.6,-0.600000000000001,-7.32)) ;
#123703=CARTESIAN_POINT('Origin',(-0.3,-0.600000000000001,-7.32)) ;
#123704=CARTESIAN_POINT('Origin',(-0.3,-0.600000000000001,-7.32)) ;
#123705=CARTESIAN_POINT('Origin',(-0.3,-6.05857864376269,-7.32)) ;
#123706=CARTESIAN_POINT('Origin',(-0.3,-6.05857864376269,-7.32)) ;
#123707=CARTESIAN_POINT('Origin',(-0.300000000000001,-6.05857864376269,
-7.32)) ;
#123708=CARTESIAN_POINT('Origin',(0.4,-6.05857864376269,-7.32)) ;
#123709=CARTESIAN_POINT('Origin',(0.300000000000002,-6.05857864376269,-7.32)) ;
#123710=CARTESIAN_POINT('Origin',(0.300000000000001,-6.05857864376269,-7.32)) ;
#123711=CARTESIAN_POINT('Origin',(0.3,-6.05857864376269,-7.32)) ;
#123712=CARTESIAN_POINT('Origin',(0.3,-0.600000000000001,-7.32)) ;
#123713=CARTESIAN_POINT('Origin',(0.3,-0.6,-7.32)) ;
#123714=CARTESIAN_POINT('Origin',(0.6,-0.6,-7.32)) ;
#123715=CARTESIAN_POINT('Origin',(6.7,0.300000000000001,-7.92)) ;
#123716=CARTESIAN_POINT('Origin',(6.65857864376269,0.300000000000001,-7.92)) ;
#123717=CARTESIAN_POINT('Origin',(6.65857864376269,0.300000000000001,-7.92)) ;
#123718=CARTESIAN_POINT('Origin',(6.65857864376269,0.300000000000002,-7.92)) ;
#123719=CARTESIAN_POINT('Origin',(6.65857864376269,-0.399999999999999,-7.92)) ;
#123720=CARTESIAN_POINT('Origin',(6.65857864376269,-0.300000000000002,-7.92)) ;
#123721=CARTESIAN_POINT('Origin',(6.65857864376269,-0.300000000000001,-7.92)) ;
#123722=CARTESIAN_POINT('Origin',(6.65857864376269,-0.300000000000001,-7.92)) ;
#123723=CARTESIAN_POINT('Origin',(0.6,-0.3,-7.92)) ;
#123724=CARTESIAN_POINT('Origin',(0.6,0.299999999999999,-7.32)) ;
#123725=CARTESIAN_POINT('Origin',(6.65857864376269,0.300000000000001,-7.32)) ;
#123726=CARTESIAN_POINT('Origin',(6.65857864376269,0.300000000000001,-7.32)) ;
#123727=CARTESIAN_POINT('Origin',(6.65857864376269,0.300000000000002,-7.32)) ;
#123728=CARTESIAN_POINT('Origin',(6.65857864376269,-0.399999999999999,-7.32)) ;
#123729=CARTESIAN_POINT('Origin',(6.65857864376269,-0.300000000000002,-7.32)) ;
#123730=CARTESIAN_POINT('Origin',(0.6,-0.3,-7.32)) ;
#123731=CARTESIAN_POINT('Origin',(6.65857864376269,-0.300000000000001,-7.32)) ;
#123732=CARTESIAN_POINT('Origin',(6.65857864376269,-0.300000000000001,-7.32)) ;
#123733=CARTESIAN_POINT('Origin',(0.6,-0.6,-11.73)) ;
#123734=CARTESIAN_POINT('Origin',(0.3,-0.6,-11.73)) ;
#123735=CARTESIAN_POINT('Origin',(0.3,-6.1,-11.73)) ;
#123736=CARTESIAN_POINT('Origin',(0.3,-6.05857864376269,-11.73)) ;
#123737=CARTESIAN_POINT('Origin',(0.3,-6.05857864376269,-11.73)) ;
#123738=CARTESIAN_POINT('Origin',(0.299999999999998,-6.05857864376269,-11.73)) ;
#123739=CARTESIAN_POINT('Origin',(0.4,-6.05857864376269,-11.73)) ;
#123740=CARTESIAN_POINT('Origin',(-0.299999999999999,-6.05857864376269,
-11.73)) ;
#123741=CARTESIAN_POINT('Origin',(-0.3,-6.05857864376269,-11.73)) ;
#123742=CARTESIAN_POINT('Origin',(-0.3,-6.05857864376269,-11.73)) ;
#123743=CARTESIAN_POINT('Origin',(-0.3,-0.600000000000001,-11.73)) ;
#123744=CARTESIAN_POINT('Origin',(-0.3,-0.600000000000001,-11.73)) ;
#123745=CARTESIAN_POINT('Origin',(0.6,-0.600000000000001,-11.73)) ;
#123746=CARTESIAN_POINT('Origin',(0.6,-0.600000000000001,-11.13)) ;
#123747=CARTESIAN_POINT('Origin',(-0.3,-0.600000000000001,-11.13)) ;
#123748=CARTESIAN_POINT('Origin',(-0.3,-0.600000000000001,-11.13)) ;
#123749=CARTESIAN_POINT('Origin',(-0.3,-6.05857864376269,-11.13)) ;
#123750=CARTESIAN_POINT('Origin',(-0.3,-6.05857864376269,-11.13)) ;
#123751=CARTESIAN_POINT('Origin',(-0.300000000000002,-6.05857864376269,
-11.13)) ;
#123752=CARTESIAN_POINT('Origin',(0.4,-6.05857864376269,-11.13)) ;
#123753=CARTESIAN_POINT('Origin',(0.300000000000001,-6.05857864376269,-11.13)) ;
#123754=CARTESIAN_POINT('Origin',(0.300000000000003,-6.05857864376269,-11.13)) ;
#123755=CARTESIAN_POINT('Origin',(0.3,-6.05857864376269,-11.13)) ;
#123756=CARTESIAN_POINT('Origin',(0.3,-0.600000000000001,-11.13)) ;
#123757=CARTESIAN_POINT('Origin',(0.3,-0.6,-11.13)) ;
#123758=CARTESIAN_POINT('Origin',(0.6,-0.6,-11.13)) ;
#123759=CARTESIAN_POINT('Origin',(6.7,0.300000000000001,-11.73)) ;
#123760=CARTESIAN_POINT('Origin',(6.65857864376269,0.300000000000001,-11.73)) ;
#123761=CARTESIAN_POINT('Origin',(6.65857864376269,0.300000000000001,-11.73)) ;
#123762=CARTESIAN_POINT('Origin',(6.65857864376269,0.300000000000001,-11.73)) ;
#123763=CARTESIAN_POINT('Origin',(6.65857864376269,-0.399999999999999,-11.73)) ;
#123764=CARTESIAN_POINT('Origin',(6.65857864376269,-0.300000000000002,-11.73)) ;
#123765=CARTESIAN_POINT('Origin',(6.65857864376269,-0.300000000000002,-11.73)) ;
#123766=CARTESIAN_POINT('Origin',(6.65857864376269,-0.300000000000001,-11.73)) ;
#123767=CARTESIAN_POINT('Origin',(0.6,-0.3,-11.73)) ;
#123768=CARTESIAN_POINT('Origin',(0.6,0.299999999999999,-11.13)) ;
#123769=CARTESIAN_POINT('Origin',(6.65857864376269,0.300000000000001,-11.13)) ;
#123770=CARTESIAN_POINT('Origin',(6.65857864376269,0.300000000000001,-11.13)) ;
#123771=CARTESIAN_POINT('Origin',(6.65857864376269,0.300000000000001,-11.13)) ;
#123772=CARTESIAN_POINT('Origin',(6.65857864376269,-0.399999999999999,-11.13)) ;
#123773=CARTESIAN_POINT('Origin',(6.65857864376269,-0.300000000000002,-11.13)) ;
#123774=CARTESIAN_POINT('Origin',(0.6,-0.3,-11.13)) ;
#123775=CARTESIAN_POINT('Origin',(6.65857864376269,-0.300000000000001,-11.13)) ;
#123776=CARTESIAN_POINT('Origin',(6.65857864376269,-0.300000000000003,-11.13)) ;
#123777=CARTESIAN_POINT('Origin',(0.6,-0.6,-15.54)) ;
#123778=CARTESIAN_POINT('Origin',(0.3,-0.6,-15.54)) ;
#123779=CARTESIAN_POINT('Origin',(0.3,-6.1,-15.54)) ;
#123780=CARTESIAN_POINT('Origin',(0.3,-6.05857864376269,-15.54)) ;
#123781=CARTESIAN_POINT('Origin',(0.3,-6.05857864376269,-15.54)) ;
#123782=CARTESIAN_POINT('Origin',(0.3,-6.05857864376269,-15.54)) ;
#123783=CARTESIAN_POINT('Origin',(0.4,-6.05857864376269,-15.54)) ;
#123784=CARTESIAN_POINT('Origin',(-0.299999999999999,-6.05857864376269,
-15.54)) ;
#123785=CARTESIAN_POINT('Origin',(-0.300000000000001,-6.05857864376269,
-15.54)) ;
#123786=CARTESIAN_POINT('Origin',(-0.3,-6.05857864376269,-15.54)) ;
#123787=CARTESIAN_POINT('Origin',(-0.3,-0.600000000000001,-15.54)) ;
#123788=CARTESIAN_POINT('Origin',(-0.3,-0.600000000000001,-15.54)) ;
#123789=CARTESIAN_POINT('Origin',(0.6,-0.600000000000001,-15.54)) ;
#123790=CARTESIAN_POINT('Origin',(0.6,-0.600000000000001,-14.94)) ;
#123791=CARTESIAN_POINT('Origin',(-0.3,-0.600000000000001,-14.94)) ;
#123792=CARTESIAN_POINT('Origin',(-0.3,-0.600000000000001,-14.94)) ;
#123793=CARTESIAN_POINT('Origin',(-0.3,-6.05857864376269,-14.94)) ;
#123794=CARTESIAN_POINT('Origin',(-0.3,-6.05857864376269,-14.94)) ;
#123795=CARTESIAN_POINT('Origin',(-0.3,-6.05857864376269,-14.94)) ;
#123796=CARTESIAN_POINT('Origin',(0.4,-6.05857864376269,-14.94)) ;
#123797=CARTESIAN_POINT('Origin',(0.299999999999999,-6.05857864376269,-14.94)) ;
#123798=CARTESIAN_POINT('Origin',(0.300000000000001,-6.05857864376269,-14.94)) ;
#123799=CARTESIAN_POINT('Origin',(0.3,-6.05857864376269,-14.94)) ;
#123800=CARTESIAN_POINT('Origin',(0.3,-0.600000000000001,-14.94)) ;
#123801=CARTESIAN_POINT('Origin',(0.3,-0.6,-14.94)) ;
#123802=CARTESIAN_POINT('Origin',(0.6,-0.6,-14.94)) ;
#123803=CARTESIAN_POINT('Origin',(6.7,0.300000000000001,-15.54)) ;
#123804=CARTESIAN_POINT('Origin',(6.65857864376269,0.300000000000001,-15.54)) ;
#123805=CARTESIAN_POINT('Origin',(6.65857864376269,0.300000000000001,-15.54)) ;
#123806=CARTESIAN_POINT('Origin',(6.65857864376269,0.300000000000003,-15.54)) ;
#123807=CARTESIAN_POINT('Origin',(6.65857864376269,-0.399999999999999,-15.54)) ;
#123808=CARTESIAN_POINT('Origin',(6.65857864376269,-0.3,-15.54)) ;
#123809=CARTESIAN_POINT('Origin',(6.65857864376269,-0.300000000000002,-15.54)) ;
#123810=CARTESIAN_POINT('Origin',(6.65857864376269,-0.300000000000001,-15.54)) ;
#123811=CARTESIAN_POINT('Origin',(0.6,-0.3,-15.54)) ;
#123812=CARTESIAN_POINT('Origin',(0.6,0.299999999999999,-14.94)) ;
#123813=CARTESIAN_POINT('Origin',(6.65857864376269,0.300000000000001,-14.94)) ;
#123814=CARTESIAN_POINT('Origin',(6.65857864376269,0.300000000000001,-14.94)) ;
#123815=CARTESIAN_POINT('Origin',(6.65857864376269,0.3,-14.94)) ;
#123816=CARTESIAN_POINT('Origin',(6.65857864376269,-0.399999999999999,-14.94)) ;
#123817=CARTESIAN_POINT('Origin',(6.65857864376269,-0.299999999999999,-14.94)) ;
#123818=CARTESIAN_POINT('Origin',(0.6,-0.3,-14.94)) ;
#123819=CARTESIAN_POINT('Origin',(6.65857864376269,-0.300000000000001,-14.94)) ;
#123820=CARTESIAN_POINT('Origin',(6.65857864376269,-0.300000000000001,-14.94)) ;
#123821=CARTESIAN_POINT('Origin',(0.6,-0.6,-19.35)) ;
#123822=CARTESIAN_POINT('Origin',(0.3,-0.6,-19.35)) ;
#123823=CARTESIAN_POINT('Origin',(0.3,-6.1,-19.35)) ;
#123824=CARTESIAN_POINT('Origin',(0.3,-6.05857864376269,-19.35)) ;
#123825=CARTESIAN_POINT('Origin',(0.3,-6.05857864376269,-19.35)) ;
#123826=CARTESIAN_POINT('Origin',(0.299999999999999,-6.05857864376269,-19.35)) ;
#123827=CARTESIAN_POINT('Origin',(0.4,-6.05857864376269,-19.35)) ;
#123828=CARTESIAN_POINT('Origin',(-0.299999999999994,-6.0585786437627,-19.35)) ;
#123829=CARTESIAN_POINT('Origin',(-0.299999999999999,-6.05857864376269,
-19.35)) ;
#123830=CARTESIAN_POINT('Origin',(-0.3,-6.05857864376269,-19.35)) ;
#123831=CARTESIAN_POINT('Origin',(-0.3,-0.600000000000001,-19.35)) ;
#123832=CARTESIAN_POINT('Origin',(-0.3,-0.600000000000001,-19.35)) ;
#123833=CARTESIAN_POINT('Origin',(0.6,-0.600000000000001,-19.35)) ;
#123834=CARTESIAN_POINT('Origin',(0.6,-0.600000000000001,-18.75)) ;
#123835=CARTESIAN_POINT('Origin',(-0.3,-0.600000000000001,-18.75)) ;
#123836=CARTESIAN_POINT('Origin',(-0.3,-0.600000000000001,-18.75)) ;
#123837=CARTESIAN_POINT('Origin',(-0.3,-6.05857864376269,-18.75)) ;
#123838=CARTESIAN_POINT('Origin',(-0.3,-6.05857864376269,-18.75)) ;
#123839=CARTESIAN_POINT('Origin',(-0.299999999999994,-6.0585786437627,-18.75)) ;
#123840=CARTESIAN_POINT('Origin',(0.4,-6.0585786437627,-18.75)) ;
#123841=CARTESIAN_POINT('Origin',(0.299999999999993,-6.0585786437627,-18.75)) ;
#123842=CARTESIAN_POINT('Origin',(0.299999999999996,-6.0585786437627,-18.75)) ;
#123843=CARTESIAN_POINT('Origin',(0.3,-6.05857864376269,-18.75)) ;
#123844=CARTESIAN_POINT('Origin',(0.3,-0.600000000000001,-18.75)) ;
#123845=CARTESIAN_POINT('Origin',(0.3,-0.6,-18.75)) ;
#123846=CARTESIAN_POINT('Origin',(0.6,-0.6,-18.75)) ;
#123847=CARTESIAN_POINT('Origin',(6.7,0.300000000000001,-19.35)) ;
#123848=CARTESIAN_POINT('Origin',(6.65857864376269,0.300000000000001,-19.35)) ;
#123849=CARTESIAN_POINT('Origin',(6.65857864376269,0.300000000000001,-19.35)) ;
#123850=CARTESIAN_POINT('Origin',(6.65857864376269,0.299999999999997,-19.35)) ;
#123851=CARTESIAN_POINT('Origin',(6.65857864376269,-0.399999999999999,-19.35)) ;
#123852=CARTESIAN_POINT('Origin',(6.65857864376269,-0.299999999999997,-19.35)) ;
#123853=CARTESIAN_POINT('Origin',(6.65857864376269,-0.3,-19.35)) ;
#123854=CARTESIAN_POINT('Origin',(6.65857864376269,-0.300000000000001,-19.35)) ;
#123855=CARTESIAN_POINT('Origin',(0.6,-0.3,-19.35)) ;
#123856=CARTESIAN_POINT('Origin',(0.6,0.299999999999999,-18.75)) ;
#123857=CARTESIAN_POINT('Origin',(6.65857864376269,0.300000000000001,-18.75)) ;
#123858=CARTESIAN_POINT('Origin',(6.65857864376269,0.300000000000001,-18.75)) ;
#123859=CARTESIAN_POINT('Origin',(6.6585786437627,0.299999999999995,-18.75)) ;
#123860=CARTESIAN_POINT('Origin',(6.6585786437627,-0.399999999999999,-18.75)) ;
#123861=CARTESIAN_POINT('Origin',(6.6585786437627,-0.299999999999994,-18.75)) ;
#123862=CARTESIAN_POINT('Origin',(0.6,-0.3,-18.75)) ;
#123863=CARTESIAN_POINT('Origin',(6.65857864376269,-0.300000000000001,-18.75)) ;
#123864=CARTESIAN_POINT('Origin',(6.65857864376269,-0.299999999999998,-18.75)) ;
#123865=CARTESIAN_POINT('Origin',(0.6,-0.6,-23.16)) ;
#123866=CARTESIAN_POINT('Origin',(0.3,-0.6,-23.16)) ;
#123867=CARTESIAN_POINT('Origin',(0.3,-6.1,-23.16)) ;
#123868=CARTESIAN_POINT('Origin',(0.3,-6.05857864376269,-23.16)) ;
#123869=CARTESIAN_POINT('Origin',(0.3,-6.05857864376269,-23.16)) ;
#123870=CARTESIAN_POINT('Origin',(0.299999999999999,-6.05857864376269,-23.16)) ;
#123871=CARTESIAN_POINT('Origin',(0.4,-6.05857864376269,-23.16)) ;
#123872=CARTESIAN_POINT('Origin',(-0.299999999999994,-6.0585786437627,-23.16)) ;
#123873=CARTESIAN_POINT('Origin',(-0.299999999999999,-6.05857864376269,
-23.16)) ;
#123874=CARTESIAN_POINT('Origin',(-0.3,-6.05857864376269,-23.16)) ;
#123875=CARTESIAN_POINT('Origin',(-0.3,-0.600000000000001,-23.16)) ;
#123876=CARTESIAN_POINT('Origin',(-0.3,-0.600000000000001,-23.16)) ;
#123877=CARTESIAN_POINT('Origin',(0.6,-0.600000000000001,-23.16)) ;
#123878=CARTESIAN_POINT('Origin',(0.6,-0.600000000000001,-22.56)) ;
#123879=CARTESIAN_POINT('Origin',(-0.3,-0.600000000000001,-22.56)) ;
#123880=CARTESIAN_POINT('Origin',(-0.3,-0.600000000000001,-22.56)) ;
#123881=CARTESIAN_POINT('Origin',(-0.3,-6.05857864376269,-22.56)) ;
#123882=CARTESIAN_POINT('Origin',(-0.3,-6.05857864376269,-22.56)) ;
#123883=CARTESIAN_POINT('Origin',(-0.299999999999994,-6.0585786437627,-22.56)) ;
#123884=CARTESIAN_POINT('Origin',(0.4,-6.0585786437627,-22.56)) ;
#123885=CARTESIAN_POINT('Origin',(0.299999999999993,-6.0585786437627,-22.56)) ;
#123886=CARTESIAN_POINT('Origin',(0.299999999999996,-6.0585786437627,-22.56)) ;
#123887=CARTESIAN_POINT('Origin',(0.3,-6.05857864376269,-22.56)) ;
#123888=CARTESIAN_POINT('Origin',(0.3,-0.600000000000001,-22.56)) ;
#123889=CARTESIAN_POINT('Origin',(0.3,-0.6,-22.56)) ;
#123890=CARTESIAN_POINT('Origin',(0.6,-0.6,-22.56)) ;
#123891=CARTESIAN_POINT('Origin',(6.7,0.300000000000001,-23.16)) ;
#123892=CARTESIAN_POINT('Origin',(6.65857864376269,0.300000000000001,-23.16)) ;
#123893=CARTESIAN_POINT('Origin',(6.65857864376269,0.300000000000001,-23.16)) ;
#123894=CARTESIAN_POINT('Origin',(6.65857864376269,0.299999999999997,-23.16)) ;
#123895=CARTESIAN_POINT('Origin',(6.65857864376269,-0.399999999999999,-23.16)) ;
#123896=CARTESIAN_POINT('Origin',(6.65857864376269,-0.299999999999997,-23.16)) ;
#123897=CARTESIAN_POINT('Origin',(6.65857864376269,-0.3,-23.16)) ;
#123898=CARTESIAN_POINT('Origin',(6.65857864376269,-0.300000000000001,-23.16)) ;
#123899=CARTESIAN_POINT('Origin',(0.6,-0.3,-23.16)) ;
#123900=CARTESIAN_POINT('Origin',(0.6,0.299999999999999,-22.56)) ;
#123901=CARTESIAN_POINT('Origin',(6.65857864376269,0.300000000000001,-22.56)) ;
#123902=CARTESIAN_POINT('Origin',(6.65857864376269,0.300000000000001,-22.56)) ;
#123903=CARTESIAN_POINT('Origin',(6.6585786437627,0.299999999999995,-22.56)) ;
#123904=CARTESIAN_POINT('Origin',(6.6585786437627,-0.399999999999999,-22.56)) ;
#123905=CARTESIAN_POINT('Origin',(6.6585786437627,-0.299999999999994,-22.56)) ;
#123906=CARTESIAN_POINT('Origin',(0.6,-0.3,-22.56)) ;
#123907=CARTESIAN_POINT('Origin',(6.65857864376269,-0.300000000000001,-22.56)) ;
#123908=CARTESIAN_POINT('Origin',(6.65857864376269,-0.299999999999998,-22.56)) ;
#123909=CARTESIAN_POINT('Origin',(0.6,-0.6,-26.97)) ;
#123910=CARTESIAN_POINT('Origin',(0.3,-0.6,-26.97)) ;
#123911=CARTESIAN_POINT('Origin',(0.3,-6.1,-26.97)) ;
#123912=CARTESIAN_POINT('Origin',(0.3,-6.05857864376269,-26.97)) ;
#123913=CARTESIAN_POINT('Origin',(0.3,-6.05857864376269,-26.97)) ;
#123914=CARTESIAN_POINT('Origin',(0.299999999999999,-6.05857864376269,-26.97)) ;
#123915=CARTESIAN_POINT('Origin',(0.4,-6.05857864376269,-26.97)) ;
#123916=CARTESIAN_POINT('Origin',(-0.299999999999994,-6.0585786437627,-26.97)) ;
#123917=CARTESIAN_POINT('Origin',(-0.299999999999999,-6.05857864376269,
-26.97)) ;
#123918=CARTESIAN_POINT('Origin',(-0.3,-6.05857864376269,-26.97)) ;
#123919=CARTESIAN_POINT('Origin',(-0.3,-0.600000000000001,-26.97)) ;
#123920=CARTESIAN_POINT('Origin',(-0.3,-0.600000000000001,-26.97)) ;
#123921=CARTESIAN_POINT('Origin',(0.6,-0.600000000000001,-26.97)) ;
#123922=CARTESIAN_POINT('Origin',(0.6,-0.600000000000001,-26.37)) ;
#123923=CARTESIAN_POINT('Origin',(-0.3,-0.600000000000001,-26.37)) ;
#123924=CARTESIAN_POINT('Origin',(-0.3,-0.600000000000001,-26.37)) ;
#123925=CARTESIAN_POINT('Origin',(-0.3,-6.05857864376269,-26.37)) ;
#123926=CARTESIAN_POINT('Origin',(-0.3,-6.05857864376269,-26.37)) ;
#123927=CARTESIAN_POINT('Origin',(-0.299999999999994,-6.0585786437627,-26.37)) ;
#123928=CARTESIAN_POINT('Origin',(0.4,-6.0585786437627,-26.37)) ;
#123929=CARTESIAN_POINT('Origin',(0.299999999999993,-6.0585786437627,-26.37)) ;
#123930=CARTESIAN_POINT('Origin',(0.299999999999996,-6.0585786437627,-26.37)) ;
#123931=CARTESIAN_POINT('Origin',(0.3,-6.05857864376269,-26.37)) ;
#123932=CARTESIAN_POINT('Origin',(0.3,-0.600000000000001,-26.37)) ;
#123933=CARTESIAN_POINT('Origin',(0.3,-0.6,-26.37)) ;
#123934=CARTESIAN_POINT('Origin',(0.6,-0.6,-26.37)) ;
#123935=CARTESIAN_POINT('Origin',(6.7,0.300000000000001,-26.97)) ;
#123936=CARTESIAN_POINT('Origin',(6.65857864376269,0.300000000000001,-26.97)) ;
#123937=CARTESIAN_POINT('Origin',(6.65857864376269,0.300000000000001,-26.97)) ;
#123938=CARTESIAN_POINT('Origin',(6.65857864376269,0.299999999999997,-26.97)) ;
#123939=CARTESIAN_POINT('Origin',(6.65857864376269,-0.399999999999999,-26.97)) ;
#123940=CARTESIAN_POINT('Origin',(6.65857864376269,-0.299999999999997,-26.97)) ;
#123941=CARTESIAN_POINT('Origin',(6.65857864376269,-0.3,-26.97)) ;
#123942=CARTESIAN_POINT('Origin',(6.65857864376269,-0.300000000000001,-26.97)) ;
#123943=CARTESIAN_POINT('Origin',(0.6,-0.3,-26.97)) ;
#123944=CARTESIAN_POINT('Origin',(0.6,0.299999999999999,-26.37)) ;
#123945=CARTESIAN_POINT('Origin',(6.65857864376269,0.300000000000001,-26.37)) ;
#123946=CARTESIAN_POINT('Origin',(6.65857864376269,0.300000000000001,-26.37)) ;
#123947=CARTESIAN_POINT('Origin',(6.6585786437627,0.299999999999995,-26.37)) ;
#123948=CARTESIAN_POINT('Origin',(6.6585786437627,-0.399999999999999,-26.37)) ;
#123949=CARTESIAN_POINT('Origin',(6.6585786437627,-0.299999999999994,-26.37)) ;
#123950=CARTESIAN_POINT('Origin',(0.6,-0.3,-26.37)) ;
#123951=CARTESIAN_POINT('Origin',(6.65857864376269,-0.300000000000001,-26.37)) ;
#123952=CARTESIAN_POINT('Origin',(6.65857864376269,-0.299999999999998,-26.37)) ;
#123953=CARTESIAN_POINT('Origin',(0.6,-0.6,-30.78)) ;
#123954=CARTESIAN_POINT('Origin',(0.3,-0.6,-30.78)) ;
#123955=CARTESIAN_POINT('Origin',(0.3,-6.1,-30.78)) ;
#123956=CARTESIAN_POINT('Origin',(0.3,-6.05857864376269,-30.78)) ;
#123957=CARTESIAN_POINT('Origin',(0.3,-6.05857864376269,-30.78)) ;
#123958=CARTESIAN_POINT('Origin',(0.299999999999999,-6.05857864376269,-30.78)) ;
#123959=CARTESIAN_POINT('Origin',(0.4,-6.05857864376269,-30.78)) ;
#123960=CARTESIAN_POINT('Origin',(-0.299999999999994,-6.0585786437627,-30.78)) ;
#123961=CARTESIAN_POINT('Origin',(-0.299999999999999,-6.05857864376269,
-30.78)) ;
#123962=CARTESIAN_POINT('Origin',(-0.3,-6.05857864376269,-30.78)) ;
#123963=CARTESIAN_POINT('Origin',(-0.3,-0.600000000000001,-30.78)) ;
#123964=CARTESIAN_POINT('Origin',(-0.3,-0.600000000000001,-30.78)) ;
#123965=CARTESIAN_POINT('Origin',(0.6,-0.600000000000001,-30.78)) ;
#123966=CARTESIAN_POINT('Origin',(0.6,-0.600000000000001,-30.18)) ;
#123967=CARTESIAN_POINT('Origin',(-0.3,-0.600000000000001,-30.18)) ;
#123968=CARTESIAN_POINT('Origin',(-0.3,-0.600000000000001,-30.18)) ;
#123969=CARTESIAN_POINT('Origin',(-0.3,-6.05857864376269,-30.18)) ;
#123970=CARTESIAN_POINT('Origin',(-0.3,-6.05857864376269,-30.18)) ;
#123971=CARTESIAN_POINT('Origin',(-0.299999999999994,-6.0585786437627,-30.18)) ;
#123972=CARTESIAN_POINT('Origin',(0.4,-6.0585786437627,-30.18)) ;
#123973=CARTESIAN_POINT('Origin',(0.299999999999993,-6.0585786437627,-30.18)) ;
#123974=CARTESIAN_POINT('Origin',(0.299999999999996,-6.0585786437627,-30.18)) ;
#123975=CARTESIAN_POINT('Origin',(0.3,-6.05857864376269,-30.18)) ;
#123976=CARTESIAN_POINT('Origin',(0.3,-0.600000000000001,-30.18)) ;
#123977=CARTESIAN_POINT('Origin',(0.3,-0.6,-30.18)) ;
#123978=CARTESIAN_POINT('Origin',(0.6,-0.6,-30.18)) ;
#123979=CARTESIAN_POINT('Origin',(6.7,0.300000000000001,-30.78)) ;
#123980=CARTESIAN_POINT('Origin',(6.65857864376269,0.300000000000001,-30.78)) ;
#123981=CARTESIAN_POINT('Origin',(6.65857864376269,0.300000000000001,-30.78)) ;
#123982=CARTESIAN_POINT('Origin',(6.65857864376269,0.299999999999997,-30.78)) ;
#123983=CARTESIAN_POINT('Origin',(6.65857864376269,-0.399999999999999,-30.78)) ;
#123984=CARTESIAN_POINT('Origin',(6.65857864376269,-0.299999999999997,-30.78)) ;
#123985=CARTESIAN_POINT('Origin',(6.65857864376269,-0.3,-30.78)) ;
#123986=CARTESIAN_POINT('Origin',(6.65857864376269,-0.300000000000001,-30.78)) ;
#123987=CARTESIAN_POINT('Origin',(0.6,-0.3,-30.78)) ;
#123988=CARTESIAN_POINT('Origin',(0.6,0.299999999999999,-30.18)) ;
#123989=CARTESIAN_POINT('Origin',(6.65857864376269,0.300000000000001,-30.18)) ;
#123990=CARTESIAN_POINT('Origin',(6.65857864376269,0.300000000000001,-30.18)) ;
#123991=CARTESIAN_POINT('Origin',(6.6585786437627,0.299999999999995,-30.18)) ;
#123992=CARTESIAN_POINT('Origin',(6.6585786437627,-0.399999999999999,-30.18)) ;
#123993=CARTESIAN_POINT('Origin',(6.6585786437627,-0.299999999999994,-30.18)) ;
#123994=CARTESIAN_POINT('Origin',(0.6,-0.3,-30.18)) ;
#123995=CARTESIAN_POINT('Origin',(6.65857864376269,-0.300000000000001,-30.18)) ;
#123996=CARTESIAN_POINT('Origin',(6.65857864376269,-0.299999999999998,-30.18)) ;
#123997=CARTESIAN_POINT('Origin',(0.6,-0.6,-34.59)) ;
#123998=CARTESIAN_POINT('Origin',(0.3,-0.6,-34.59)) ;
#123999=CARTESIAN_POINT('Origin',(0.3,-6.1,-34.59)) ;
#124000=CARTESIAN_POINT('Origin',(0.3,-6.05857864376269,-34.59)) ;
#124001=CARTESIAN_POINT('Origin',(0.3,-6.05857864376269,-34.59)) ;
#124002=CARTESIAN_POINT('Origin',(0.3,-6.05857864376269,-34.59)) ;
#124003=CARTESIAN_POINT('Origin',(0.4,-6.05857864376269,-34.59)) ;
#124004=CARTESIAN_POINT('Origin',(-0.299999999999998,-6.05857864376269,
-34.59)) ;
#124005=CARTESIAN_POINT('Origin',(-0.299999999999994,-6.0585786437627,-34.59)) ;
#124006=CARTESIAN_POINT('Origin',(-0.3,-6.05857864376269,-34.59)) ;
#124007=CARTESIAN_POINT('Origin',(-0.3,-0.600000000000001,-34.59)) ;
#124008=CARTESIAN_POINT('Origin',(-0.3,-0.600000000000001,-34.59)) ;
#124009=CARTESIAN_POINT('Origin',(0.6,-0.600000000000001,-34.59)) ;
#124010=CARTESIAN_POINT('Origin',(0.6,-0.600000000000001,-33.99)) ;
#124011=CARTESIAN_POINT('Origin',(-0.3,-0.600000000000001,-33.99)) ;
#124012=CARTESIAN_POINT('Origin',(-0.3,-0.600000000000001,-33.99)) ;
#124013=CARTESIAN_POINT('Origin',(-0.3,-6.05857864376269,-33.99)) ;
#124014=CARTESIAN_POINT('Origin',(-0.3,-6.05857864376269,-33.99)) ;
#124015=CARTESIAN_POINT('Origin',(-0.300000000000007,-6.05857864376268,
-33.99)) ;
#124016=CARTESIAN_POINT('Origin',(0.4,-6.05857864376269,-33.99)) ;
#124017=CARTESIAN_POINT('Origin',(0.30000000000001,-6.05857864376268,-33.99)) ;
#124018=CARTESIAN_POINT('Origin',(0.300000000000006,-6.05857864376268,-33.99)) ;
#124019=CARTESIAN_POINT('Origin',(0.3,-6.05857864376269,-33.99)) ;
#124020=CARTESIAN_POINT('Origin',(0.3,-0.600000000000001,-33.99)) ;
#124021=CARTESIAN_POINT('Origin',(0.3,-0.6,-33.99)) ;
#124022=CARTESIAN_POINT('Origin',(0.6,-0.6,-33.99)) ;
#124023=CARTESIAN_POINT('Origin',(6.7,0.300000000000001,-34.59)) ;
#124024=CARTESIAN_POINT('Origin',(6.65857864376269,0.300000000000001,-34.59)) ;
#124025=CARTESIAN_POINT('Origin',(6.65857864376269,0.300000000000001,-34.59)) ;
#124026=CARTESIAN_POINT('Origin',(6.65857864376269,0.300000000000001,-34.59)) ;
#124027=CARTESIAN_POINT('Origin',(6.6585786437627,-0.399999999999999,-34.59)) ;
#124028=CARTESIAN_POINT('Origin',(6.65857864376269,-0.300000000000002,-34.59)) ;
#124029=CARTESIAN_POINT('Origin',(6.6585786437627,-0.299999999999996,-34.59)) ;
#124030=CARTESIAN_POINT('Origin',(6.65857864376269,-0.300000000000001,-34.59)) ;
#124031=CARTESIAN_POINT('Origin',(0.6,-0.3,-34.59)) ;
#124032=CARTESIAN_POINT('Origin',(0.6,0.299999999999999,-33.99)) ;
#124033=CARTESIAN_POINT('Origin',(6.65857864376269,0.300000000000001,-33.99)) ;
#124034=CARTESIAN_POINT('Origin',(6.65857864376269,0.300000000000001,-33.99)) ;
#124035=CARTESIAN_POINT('Origin',(6.65857864376269,0.300000000000005,-33.99)) ;
#124036=CARTESIAN_POINT('Origin',(6.65857864376269,-0.399999999999999,-33.99)) ;
#124037=CARTESIAN_POINT('Origin',(6.65857864376268,-0.300000000000006,-33.99)) ;
#124038=CARTESIAN_POINT('Origin',(0.6,-0.3,-33.99)) ;
#124039=CARTESIAN_POINT('Origin',(6.65857864376269,-0.300000000000001,-33.99)) ;
#124040=CARTESIAN_POINT('Origin',(6.65857864376269,-0.300000000000001,-33.99)) ;
#126560=UNCERTAINTY_MEASURE_WITH_UNIT(LENGTH_MEASURE(0.01),#126572,
'DISTANCE_ACCURACY_VALUE',
'Maximum model space distance between geometric entities at asserted c
onnectivities') ;
#126563=UNCERTAINTY_MEASURE_WITH_UNIT(LENGTH_MEASURE(0.01),#126572,
'DISTANCE_ACCURACY_VALUE',
'Maximum model space distance between geometric entities at asserted c
onnectivities') ;
#126568=(
GEOMETRIC_REPRESENTATION_CONTEXT(3)
GLOBAL_UNCERTAINTY_ASSIGNED_CONTEXT((#126560))
GLOBAL_UNIT_ASSIGNED_CONTEXT((#126572,#126574,#126575))
REPRESENTATION_CONTEXT('','3D')
) ;
#126571=(
GEOMETRIC_REPRESENTATION_CONTEXT(3)
GLOBAL_UNCERTAINTY_ASSIGNED_CONTEXT((#126563))
GLOBAL_UNIT_ASSIGNED_CONTEXT((#126572,#126574,#126575))
REPRESENTATION_CONTEXT('','3D')
) ;
#126572=(
LENGTH_UNIT()
NAMED_UNIT(*)
SI_UNIT(.MILLI.,.METRE.)
) ;
#126574=(
NAMED_UNIT(*)
PLANE_ANGLE_UNIT()
SI_UNIT($,.RADIAN.)
) ;
#126575=(
NAMED_UNIT(*)
SI_UNIT($,.STERADIAN.)
SOLID_ANGLE_UNIT()
) ;
#126580=SHAPE_DEFINITION_REPRESENTATION(#126587,#126602) ;
#126587=PRODUCT_DEFINITION_SHAPE('',$,#126610) ;
#126602=SHAPE_REPRESENTATION('',(#71866),#126568) ;
#126605=PRODUCT_DEFINITION_CONTEXT('part definition',#126628,'design') ;
#126610=PRODUCT_DEFINITION('Header_3.81mm_N10','Header_3.81mm_N10',#126617,
#126605) ;
#126617=PRODUCT_DEFINITION_FORMATION('',$,#126634) ;
#126628=APPLICATION_CONTEXT(
'Core Data for Automotive Mechanical Design Process') ;
#126629=PRODUCT_CONTEXT('part definition',#126628,'mechanical') ;
#126634=PRODUCT('Header_3.81mm_N10','Header_3.81mm_N10',$,(#126629)) ;
#126639=PRESENTATION_STYLE_ASSIGNMENT((#126648)) ;
#126640=PRESENTATION_STYLE_ASSIGNMENT((#126649)) ;
#126641=PRESENTATION_STYLE_ASSIGNMENT((#126650)) ;
#126648=SURFACE_STYLE_USAGE(.BOTH.,#126657) ;
#126649=SURFACE_STYLE_USAGE(.BOTH.,#126658) ;
#126650=SURFACE_STYLE_USAGE(.BOTH.,#126659) ;
#126657=SURFACE_SIDE_STYLE('',(#126666)) ;
#126658=SURFACE_SIDE_STYLE('',(#126667)) ;
#126659=SURFACE_SIDE_STYLE('',(#126668)) ;
#126666=SURFACE_STYLE_FILL_AREA(#126675) ;
#126667=SURFACE_STYLE_FILL_AREA(#126676) ;
#126668=SURFACE_STYLE_FILL_AREA(#126677) ;
#126675=FILL_AREA_STYLE('Opaque(202,209,238)',(#126684)) ;
#126676=FILL_AREA_STYLE('Opaque(128,255,128)',(#126685)) ;
#126677=FILL_AREA_STYLE('Opaque(204,207,204)',(#126686)) ;
#126684=FILL_AREA_STYLE_COLOUR('Opaque(202,209,238)',#126693) ;
#126685=FILL_AREA_STYLE_COLOUR('Opaque(128,255,128)',#126694) ;
#126686=FILL_AREA_STYLE_COLOUR('Opaque(204,207,204)',#126695) ;
#126693=COLOUR_RGB('Opaque(202,209,238)', 0.66274510, 0.83137255, 0.94901961) ;
#126694=COLOUR_RGB('Opaque(128,255,128)', 0.66274510, 0.83137255, 0.94901961) ;
#126695=COLOUR_RGB('Opaque(204,207,204)', 0.40784314, 0.44705882, 0.49803922) ;
ENDSEC;
END-ISO-10303-21;
